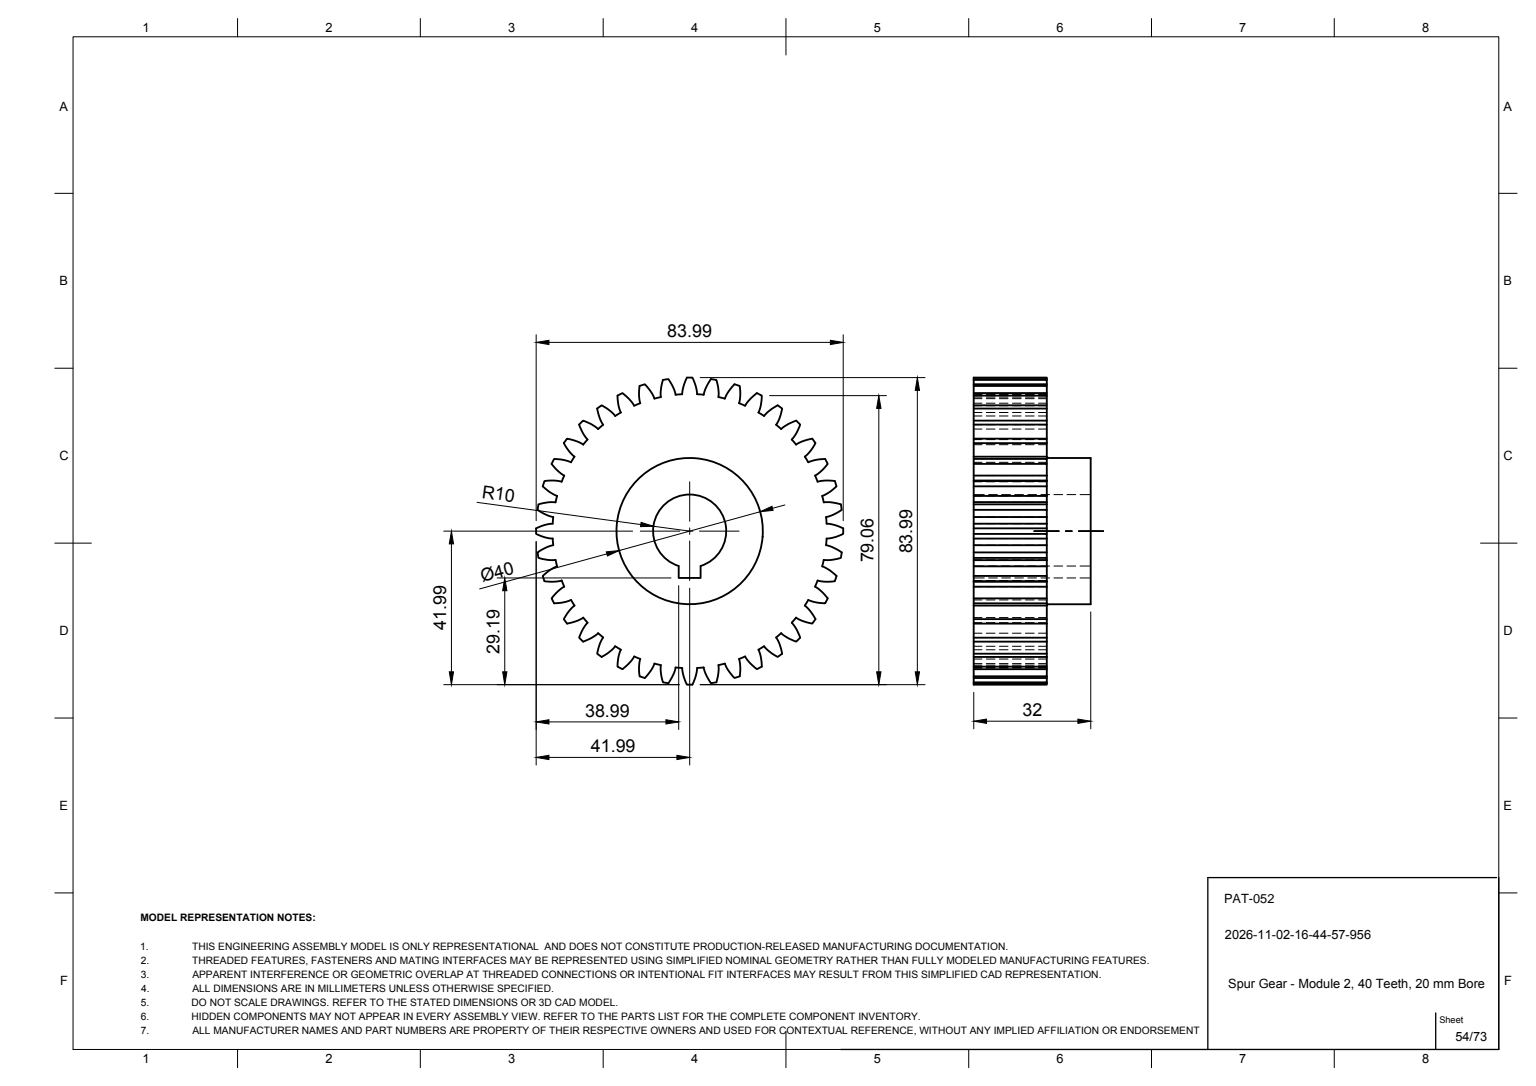
ISO-10303-21;
HEADER;
/* Generated by software containing ST-Developer
 * from STEP Tools, Inc. (www.steptools.com) 
 */

FILE_DESCRIPTION(
/* description */ ('Hand-crank gear train demonstrator'),
/* implementation_level */ '2;1');

FILE_NAME(
/* name */ 'Spur Gear - Module 2, 40 Teeth, 20 mm Bore.step',
/* time_stamp */ '2026-10-28T03:22:13-07:00',
/* author */ (''),
/* organization */ (''),
/* preprocessor_version */ 'ST-DEVELOPER v20.2',
/* originating_system */ 'Autodesk Translation Framework v15.17.0.0',
/* authorisation */ '');

FILE_SCHEMA (('AUTOMOTIVE_DESIGN { 1 0 10303 214 3 1 1 }'));
ENDSEC;

DATA;
#10=MECHANICAL_DESIGN_GEOMETRIC_PRESENTATION_REPRESENTATION('',(#1263),#62758);
#51=(
BOUNDED_SURFACE()
B_SPLINE_SURFACE(5,1,((#44627,#44628),(#44629,#44630),(#44631,#44632),(#44633,
#44634),(#44635,#44636),(#44637,#44638),(#44639,#44640),(#44641,#44642),
(#44643,#44644),(#44645,#44646),(#44647,#44648),(#44649,#44650),(#44651,
#44652),(#44653,#44654),(#44655,#44656),(#44657,#44658),(#44659,#44660),
(#44661,#44662),(#44663,#44664),(#44665,#44666),(#44667,#44668),(#44669,
#44670),(#44671,#44672),(#44673,#44674),(#44675,#44676),(#44677,#44678),
(#44679,#44680),(#44681,#44682),(#44683,#44684),(#44685,#44686),(#44687,
#44688),(#44689,#44690),(#44691,#44692),(#44693,#44694),(#44695,#44696),
(#44697,#44698),(#44699,#44700),(#44701,#44702),(#44703,#44704),(#44705,
#44706),(#44707,#44708),(#44709,#44710),(#44711,#44712),(#44713,#44714),
(#44715,#44716),(#44717,#44718),(#44719,#44720),(#44721,#44722),(#44723,
#44724),(#44725,#44726),(#44727,#44728),(#44729,#44730),(#44731,#44732),
(#44733,#44734),(#44735,#44736),(#44737,#44738),(#44739,#44740),(#44741,
#44742),(#44743,#44744),(#44745,#44746),(#44747,#44748),(#44749,#44750),
(#44751,#44752),(#44753,#44754),(#44755,#44756),(#44757,#44758),(#44759,
#44760),(#44761,#44762),(#44763,#44764),(#44765,#44766)),.UNSPECIFIED.,
 .F.,.F.,.F.)
B_SPLINE_SURFACE_WITH_KNOTS((6,1,1,1,1,1,1,1,1,1,1,1,1,1,1,1,1,1,1,1,1,
1,1,1,1,1,1,1,1,1,1,1,1,1,1,1,1,1,1,1,1,1,1,1,1,1,1,1,1,1,1,1,1,1,1,1,1,
1,1,1,1,1,1,1,1,6),(2,2),(-1.,-0.984615384615383,-0.969230769230768,-0.953846153846152,
-0.938461538461537,-0.923076923076922,-0.907692307692306,-0.892307692307691,
-0.876923076923076,-0.86153846153846,-0.846153846153845,-0.83076923076923,
-0.815384615384614,-0.799999999999999,-0.784615384615384,-0.769230769230768,
-0.753846153846153,-0.738461538461538,-0.723076923076922,-0.707692307692307,
-0.692307692307692,-0.676923076923076,-0.661538461538461,-0.646153846153846,
-0.63076923076923,-0.615384615384615,-0.6,-0.584615384615384,-0.569230769230769,
-0.553846153846154,-0.538461538461538,-0.523076923076923,-0.507692307692308,
-0.492307692307692,-0.476923076923077,-0.461538461538462,-0.446153846153846,
-0.430769230769231,-0.415384615384615,-0.4,-0.384615384615385,-0.369230769230769,
-0.353846153846154,-0.338461538461538,-0.323076923076923,-0.307692307692308,
-0.292307692307692,-0.276923076923077,-0.261538461538462,-0.246153846153846,
-0.230769230769231,-0.215384615384615,-0.2,-0.184615384615385,-0.169230769230769,
-0.153846153846154,-0.138461538461538,-0.123076923076923,-0.107692307692308,
-0.0923076923076923,-0.0769230769230769,-0.0615384615384615,-0.0461538461538462,
-0.0307692307692308,-0.0153846153846154,0.),(-1.,1.),.UNSPECIFIED.)
GEOMETRIC_REPRESENTATION_ITEM()
RATIONAL_B_SPLINE_SURFACE(((1.,1.),(1.,1.),(1.,1.),(1.,1.),(1.,1.),(1.,
1.),(1.,1.),(1.,1.),(1.,1.),(1.,1.),(1.,1.),(1.,1.),(1.,1.),(1.,1.),(1.,
1.),(1.,1.),(1.,1.),(1.,1.),(1.,1.),(1.,1.),(1.,1.),(1.,1.),(1.,1.),(1.,
1.),(1.,1.),(1.,1.),(1.,1.),(1.,1.),(1.,1.),(1.,1.),(1.,1.),(1.,1.),(1.,
1.),(1.,1.),(1.,1.),(1.,1.),(1.,1.),(1.,1.),(1.,1.),(1.,1.),(1.,1.),(1.,
1.),(1.,1.),(1.,1.),(1.,1.),(1.,1.),(1.,1.),(1.,1.),(1.,1.),(1.,1.),(1.,
1.),(1.,1.),(1.,1.),(1.,1.),(1.,1.),(1.,1.),(1.,1.),(1.,1.),(1.,1.),(1.,
1.),(1.,1.),(1.,1.),(1.,1.),(1.,1.),(1.,1.),(1.,1.),(1.,1.),(1.,1.),(1.,
1.),(1.,1.)))
REPRESENTATION_ITEM('')
SURFACE()
);
#52=(
BOUNDED_SURFACE()
B_SPLINE_SURFACE(5,1,((#44846,#44847),(#44848,#44849),(#44850,#44851),(#44852,
#44853),(#44854,#44855),(#44856,#44857),(#44858,#44859),(#44860,#44861),
(#44862,#44863),(#44864,#44865),(#44866,#44867),(#44868,#44869),(#44870,
#44871),(#44872,#44873),(#44874,#44875),(#44876,#44877),(#44878,#44879),
(#44880,#44881),(#44882,#44883),(#44884,#44885),(#44886,#44887),(#44888,
#44889),(#44890,#44891),(#44892,#44893),(#44894,#44895),(#44896,#44897),
(#44898,#44899),(#44900,#44901),(#44902,#44903),(#44904,#44905),(#44906,
#44907),(#44908,#44909),(#44910,#44911),(#44912,#44913),(#44914,#44915),
(#44916,#44917),(#44918,#44919),(#44920,#44921),(#44922,#44923),(#44924,
#44925),(#44926,#44927),(#44928,#44929),(#44930,#44931),(#44932,#44933),
(#44934,#44935),(#44936,#44937),(#44938,#44939),(#44940,#44941),(#44942,
#44943),(#44944,#44945),(#44946,#44947),(#44948,#44949),(#44950,#44951),
(#44952,#44953),(#44954,#44955),(#44956,#44957),(#44958,#44959),(#44960,
#44961),(#44962,#44963),(#44964,#44965),(#44966,#44967),(#44968,#44969),
(#44970,#44971),(#44972,#44973),(#44974,#44975),(#44976,#44977),(#44978,
#44979),(#44980,#44981),(#44982,#44983),(#44984,#44985)),.UNSPECIFIED.,
 .F.,.F.,.F.)
B_SPLINE_SURFACE_WITH_KNOTS((6,1,1,1,1,1,1,1,1,1,1,1,1,1,1,1,1,1,1,1,1,
1,1,1,1,1,1,1,1,1,1,1,1,1,1,1,1,1,1,1,1,1,1,1,1,1,1,1,1,1,1,1,1,1,1,1,1,
1,1,1,1,1,1,1,1,6),(2,2),(-1.,-0.984615384615383,-0.969230769230768,-0.953846153846152,
-0.938461538461537,-0.923076923076922,-0.907692307692306,-0.892307692307691,
-0.876923076923076,-0.86153846153846,-0.846153846153845,-0.83076923076923,
-0.815384615384614,-0.799999999999999,-0.784615384615384,-0.769230769230768,
-0.753846153846153,-0.738461538461538,-0.723076923076922,-0.707692307692307,
-0.692307692307692,-0.676923076923076,-0.661538461538461,-0.646153846153846,
-0.63076923076923,-0.615384615384615,-0.6,-0.584615384615384,-0.569230769230769,
-0.553846153846154,-0.538461538461538,-0.523076923076923,-0.507692307692308,
-0.492307692307692,-0.476923076923077,-0.461538461538462,-0.446153846153846,
-0.430769230769231,-0.415384615384615,-0.4,-0.384615384615385,-0.369230769230769,
-0.353846153846154,-0.338461538461538,-0.323076923076923,-0.307692307692308,
-0.292307692307692,-0.276923076923077,-0.261538461538462,-0.246153846153846,
-0.230769230769231,-0.215384615384615,-0.2,-0.184615384615385,-0.169230769230769,
-0.153846153846154,-0.138461538461538,-0.123076923076923,-0.107692307692308,
-0.0923076923076923,-0.0769230769230769,-0.0615384615384615,-0.0461538461538462,
-0.0307692307692308,-0.0153846153846154,0.),(-1.,1.),.UNSPECIFIED.)
GEOMETRIC_REPRESENTATION_ITEM()
RATIONAL_B_SPLINE_SURFACE(((1.,1.),(1.,1.),(1.,1.),(1.,1.),(1.,1.),(1.,
1.),(1.,1.),(1.,1.),(1.,1.),(1.,1.),(1.,1.),(1.,1.),(1.,1.),(1.,1.),(1.,
1.),(1.,1.),(1.,1.),(1.,1.),(1.,1.),(1.,1.),(1.,1.),(1.,1.),(1.,1.),(1.,
1.),(1.,1.),(1.,1.),(1.,1.),(1.,1.),(1.,1.),(1.,1.),(1.,1.),(1.,1.),(1.,
1.),(1.,1.),(1.,1.),(1.,1.),(1.,1.),(1.,1.),(1.,1.),(1.,1.),(1.,1.),(1.,
1.),(1.,1.),(1.,1.),(1.,1.),(1.,1.),(1.,1.),(1.,1.),(1.,1.),(1.,1.),(1.,
1.),(1.,1.),(1.,1.),(1.,1.),(1.,1.),(1.,1.),(1.,1.),(1.,1.),(1.,1.),(1.,
1.),(1.,1.),(1.,1.),(1.,1.),(1.,1.),(1.,1.),(1.,1.),(1.,1.),(1.,1.),(1.,
1.),(1.,1.)))
REPRESENTATION_ITEM('')
SURFACE()
);
#53=(
BOUNDED_SURFACE()
B_SPLINE_SURFACE(5,1,((#45076,#45077),(#45078,#45079),(#45080,#45081),(#45082,
#45083),(#45084,#45085),(#45086,#45087),(#45088,#45089),(#45090,#45091),
(#45092,#45093),(#45094,#45095),(#45096,#45097),(#45098,#45099),(#45100,
#45101),(#45102,#45103),(#45104,#45105),(#45106,#45107),(#45108,#45109),
(#45110,#45111),(#45112,#45113),(#45114,#45115),(#45116,#45117),(#45118,
#45119),(#45120,#45121),(#45122,#45123),(#45124,#45125),(#45126,#45127),
(#45128,#45129),(#45130,#45131),(#45132,#45133),(#45134,#45135),(#45136,
#45137),(#45138,#45139),(#45140,#45141),(#45142,#45143),(#45144,#45145),
(#45146,#45147),(#45148,#45149),(#45150,#45151),(#45152,#45153),(#45154,
#45155),(#45156,#45157),(#45158,#45159),(#45160,#45161),(#45162,#45163),
(#45164,#45165),(#45166,#45167),(#45168,#45169),(#45170,#45171),(#45172,
#45173),(#45174,#45175),(#45176,#45177),(#45178,#45179),(#45180,#45181),
(#45182,#45183),(#45184,#45185),(#45186,#45187),(#45188,#45189),(#45190,
#45191),(#45192,#45193),(#45194,#45195),(#45196,#45197),(#45198,#45199),
(#45200,#45201),(#45202,#45203),(#45204,#45205),(#45206,#45207),(#45208,
#45209),(#45210,#45211),(#45212,#45213),(#45214,#45215)),.UNSPECIFIED.,
 .F.,.F.,.F.)
B_SPLINE_SURFACE_WITH_KNOTS((6,1,1,1,1,1,1,1,1,1,1,1,1,1,1,1,1,1,1,1,1,
1,1,1,1,1,1,1,1,1,1,1,1,1,1,1,1,1,1,1,1,1,1,1,1,1,1,1,1,1,1,1,1,1,1,1,1,
1,1,1,1,1,1,1,1,6),(2,2),(-1.,-0.984615384615383,-0.969230769230768,-0.953846153846152,
-0.938461538461537,-0.923076923076922,-0.907692307692306,-0.892307692307691,
-0.876923076923076,-0.86153846153846,-0.846153846153845,-0.83076923076923,
-0.815384615384614,-0.799999999999999,-0.784615384615384,-0.769230769230768,
-0.753846153846153,-0.738461538461538,-0.723076923076922,-0.707692307692307,
-0.692307692307692,-0.676923076923076,-0.661538461538461,-0.646153846153846,
-0.63076923076923,-0.615384615384615,-0.6,-0.584615384615384,-0.569230769230769,
-0.553846153846154,-0.538461538461538,-0.523076923076923,-0.507692307692308,
-0.492307692307692,-0.476923076923077,-0.461538461538462,-0.446153846153846,
-0.430769230769231,-0.415384615384615,-0.4,-0.384615384615385,-0.369230769230769,
-0.353846153846154,-0.338461538461538,-0.323076923076923,-0.307692307692308,
-0.292307692307692,-0.276923076923077,-0.261538461538462,-0.246153846153846,
-0.230769230769231,-0.215384615384615,-0.2,-0.184615384615385,-0.169230769230769,
-0.153846153846154,-0.138461538461538,-0.123076923076923,-0.107692307692308,
-0.0923076923076923,-0.0769230769230769,-0.0615384615384615,-0.0461538461538462,
-0.0307692307692308,-0.0153846153846154,0.),(-1.,1.),.UNSPECIFIED.)
GEOMETRIC_REPRESENTATION_ITEM()
RATIONAL_B_SPLINE_SURFACE(((1.,1.),(1.,1.),(1.,1.),(1.,1.),(1.,1.),(1.,
1.),(1.,1.),(1.,1.),(1.,1.),(1.,1.),(1.,1.),(1.,1.),(1.,1.),(1.,1.),(1.,
1.),(1.,1.),(1.,1.),(1.,1.),(1.,1.),(1.,1.),(1.,1.),(1.,1.),(1.,1.),(1.,
1.),(1.,1.),(1.,1.),(1.,1.),(1.,1.),(1.,1.),(1.,1.),(1.,1.),(1.,1.),(1.,
1.),(1.,1.),(1.,1.),(1.,1.),(1.,1.),(1.,1.),(1.,1.),(1.,1.),(1.,1.),(1.,
1.),(1.,1.),(1.,1.),(1.,1.),(1.,1.),(1.,1.),(1.,1.),(1.,1.),(1.,1.),(1.,
1.),(1.,1.),(1.,1.),(1.,1.),(1.,1.),(1.,1.),(1.,1.),(1.,1.),(1.,1.),(1.,
1.),(1.,1.),(1.,1.),(1.,1.),(1.,1.),(1.,1.),(1.,1.),(1.,1.),(1.,1.),(1.,
1.),(1.,1.)))
REPRESENTATION_ITEM('')
SURFACE()
);
#54=(
BOUNDED_SURFACE()
B_SPLINE_SURFACE(5,1,((#45288,#45289),(#45290,#45291),(#45292,#45293),(#45294,
#45295),(#45296,#45297),(#45298,#45299),(#45300,#45301),(#45302,#45303),
(#45304,#45305),(#45306,#45307),(#45308,#45309),(#45310,#45311),(#45312,
#45313),(#45314,#45315),(#45316,#45317),(#45318,#45319),(#45320,#45321),
(#45322,#45323),(#45324,#45325),(#45326,#45327),(#45328,#45329),(#45330,
#45331),(#45332,#45333),(#45334,#45335),(#45336,#45337),(#45338,#45339),
(#45340,#45341),(#45342,#45343),(#45344,#45345),(#45346,#45347),(#45348,
#45349),(#45350,#45351),(#45352,#45353),(#45354,#45355),(#45356,#45357),
(#45358,#45359),(#45360,#45361),(#45362,#45363),(#45364,#45365),(#45366,
#45367),(#45368,#45369),(#45370,#45371),(#45372,#45373),(#45374,#45375),
(#45376,#45377),(#45378,#45379),(#45380,#45381),(#45382,#45383),(#45384,
#45385),(#45386,#45387),(#45388,#45389),(#45390,#45391),(#45392,#45393),
(#45394,#45395),(#45396,#45397),(#45398,#45399),(#45400,#45401),(#45402,
#45403),(#45404,#45405),(#45406,#45407),(#45408,#45409),(#45410,#45411),
(#45412,#45413),(#45414,#45415),(#45416,#45417),(#45418,#45419),(#45420,
#45421),(#45422,#45423),(#45424,#45425),(#45426,#45427)),.UNSPECIFIED.,
 .F.,.F.,.F.)
B_SPLINE_SURFACE_WITH_KNOTS((6,1,1,1,1,1,1,1,1,1,1,1,1,1,1,1,1,1,1,1,1,
1,1,1,1,1,1,1,1,1,1,1,1,1,1,1,1,1,1,1,1,1,1,1,1,1,1,1,1,1,1,1,1,1,1,1,1,
1,1,1,1,1,1,1,1,6),(2,2),(-1.,-0.984615384615383,-0.969230769230768,-0.953846153846152,
-0.938461538461537,-0.923076923076922,-0.907692307692306,-0.892307692307691,
-0.876923076923076,-0.86153846153846,-0.846153846153845,-0.83076923076923,
-0.815384615384614,-0.799999999999999,-0.784615384615384,-0.769230769230768,
-0.753846153846153,-0.738461538461538,-0.723076923076922,-0.707692307692307,
-0.692307692307692,-0.676923076923076,-0.661538461538461,-0.646153846153846,
-0.63076923076923,-0.615384615384615,-0.6,-0.584615384615384,-0.569230769230769,
-0.553846153846154,-0.538461538461538,-0.523076923076923,-0.507692307692308,
-0.492307692307692,-0.476923076923077,-0.461538461538462,-0.446153846153846,
-0.430769230769231,-0.415384615384615,-0.4,-0.384615384615385,-0.369230769230769,
-0.353846153846154,-0.338461538461538,-0.323076923076923,-0.307692307692308,
-0.292307692307692,-0.276923076923077,-0.261538461538462,-0.246153846153846,
-0.230769230769231,-0.215384615384615,-0.2,-0.184615384615385,-0.169230769230769,
-0.153846153846154,-0.138461538461538,-0.123076923076923,-0.107692307692308,
-0.0923076923076923,-0.0769230769230769,-0.0615384615384615,-0.0461538461538462,
-0.0307692307692308,-0.0153846153846154,0.),(-1.,1.),.UNSPECIFIED.)
GEOMETRIC_REPRESENTATION_ITEM()
RATIONAL_B_SPLINE_SURFACE(((1.,1.),(1.,1.),(1.,1.),(1.,1.),(1.,1.),(1.,
1.),(1.,1.),(1.,1.),(1.,1.),(1.,1.),(1.,1.),(1.,1.),(1.,1.),(1.,1.),(1.,
1.),(1.,1.),(1.,1.),(1.,1.),(1.,1.),(1.,1.),(1.,1.),(1.,1.),(1.,1.),(1.,
1.),(1.,1.),(1.,1.),(1.,1.),(1.,1.),(1.,1.),(1.,1.),(1.,1.),(1.,1.),(1.,
1.),(1.,1.),(1.,1.),(1.,1.),(1.,1.),(1.,1.),(1.,1.),(1.,1.),(1.,1.),(1.,
1.),(1.,1.),(1.,1.),(1.,1.),(1.,1.),(1.,1.),(1.,1.),(1.,1.),(1.,1.),(1.,
1.),(1.,1.),(1.,1.),(1.,1.),(1.,1.),(1.,1.),(1.,1.),(1.,1.),(1.,1.),(1.,
1.),(1.,1.),(1.,1.),(1.,1.),(1.,1.),(1.,1.),(1.,1.),(1.,1.),(1.,1.),(1.,
1.),(1.,1.)))
REPRESENTATION_ITEM('')
SURFACE()
);
#55=(
BOUNDED_SURFACE()
B_SPLINE_SURFACE(5,1,((#45518,#45519),(#45520,#45521),(#45522,#45523),(#45524,
#45525),(#45526,#45527),(#45528,#45529),(#45530,#45531),(#45532,#45533),
(#45534,#45535),(#45536,#45537),(#45538,#45539),(#45540,#45541),(#45542,
#45543),(#45544,#45545),(#45546,#45547),(#45548,#45549),(#45550,#45551),
(#45552,#45553),(#45554,#45555),(#45556,#45557),(#45558,#45559),(#45560,
#45561),(#45562,#45563),(#45564,#45565),(#45566,#45567),(#45568,#45569),
(#45570,#45571),(#45572,#45573),(#45574,#45575),(#45576,#45577),(#45578,
#45579),(#45580,#45581),(#45582,#45583),(#45584,#45585),(#45586,#45587),
(#45588,#45589),(#45590,#45591),(#45592,#45593),(#45594,#45595),(#45596,
#45597),(#45598,#45599),(#45600,#45601),(#45602,#45603),(#45604,#45605),
(#45606,#45607),(#45608,#45609),(#45610,#45611),(#45612,#45613),(#45614,
#45615),(#45616,#45617),(#45618,#45619),(#45620,#45621),(#45622,#45623),
(#45624,#45625),(#45626,#45627),(#45628,#45629),(#45630,#45631),(#45632,
#45633),(#45634,#45635),(#45636,#45637),(#45638,#45639),(#45640,#45641),
(#45642,#45643),(#45644,#45645),(#45646,#45647),(#45648,#45649),(#45650,
#45651),(#45652,#45653),(#45654,#45655),(#45656,#45657)),.UNSPECIFIED.,
 .F.,.F.,.F.)
B_SPLINE_SURFACE_WITH_KNOTS((6,1,1,1,1,1,1,1,1,1,1,1,1,1,1,1,1,1,1,1,1,
1,1,1,1,1,1,1,1,1,1,1,1,1,1,1,1,1,1,1,1,1,1,1,1,1,1,1,1,1,1,1,1,1,1,1,1,
1,1,1,1,1,1,1,1,6),(2,2),(-1.,-0.984615384615383,-0.969230769230768,-0.953846153846152,
-0.938461538461537,-0.923076923076922,-0.907692307692306,-0.892307692307691,
-0.876923076923076,-0.86153846153846,-0.846153846153845,-0.83076923076923,
-0.815384615384614,-0.799999999999999,-0.784615384615384,-0.769230769230768,
-0.753846153846153,-0.738461538461538,-0.723076923076922,-0.707692307692307,
-0.692307692307692,-0.676923076923076,-0.661538461538461,-0.646153846153846,
-0.63076923076923,-0.615384615384615,-0.6,-0.584615384615384,-0.569230769230769,
-0.553846153846154,-0.538461538461538,-0.523076923076923,-0.507692307692308,
-0.492307692307692,-0.476923076923077,-0.461538461538462,-0.446153846153846,
-0.430769230769231,-0.415384615384615,-0.4,-0.384615384615385,-0.369230769230769,
-0.353846153846154,-0.338461538461538,-0.323076923076923,-0.307692307692308,
-0.292307692307692,-0.276923076923077,-0.261538461538462,-0.246153846153846,
-0.230769230769231,-0.215384615384615,-0.2,-0.184615384615385,-0.169230769230769,
-0.153846153846154,-0.138461538461538,-0.123076923076923,-0.107692307692308,
-0.0923076923076923,-0.0769230769230769,-0.0615384615384615,-0.0461538461538462,
-0.0307692307692308,-0.0153846153846154,0.),(-1.,1.),.UNSPECIFIED.)
GEOMETRIC_REPRESENTATION_ITEM()
RATIONAL_B_SPLINE_SURFACE(((1.,1.),(1.,1.),(1.,1.),(1.,1.),(1.,1.),(1.,
1.),(1.,1.),(1.,1.),(1.,1.),(1.,1.),(1.,1.),(1.,1.),(1.,1.),(1.,1.),(1.,
1.),(1.,1.),(1.,1.),(1.,1.),(1.,1.),(1.,1.),(1.,1.),(1.,1.),(1.,1.),(1.,
1.),(1.,1.),(1.,1.),(1.,1.),(1.,1.),(1.,1.),(1.,1.),(1.,1.),(1.,1.),(1.,
1.),(1.,1.),(1.,1.),(1.,1.),(1.,1.),(1.,1.),(1.,1.),(1.,1.),(1.,1.),(1.,
1.),(1.,1.),(1.,1.),(1.,1.),(1.,1.),(1.,1.),(1.,1.),(1.,1.),(1.,1.),(1.,
1.),(1.,1.),(1.,1.),(1.,1.),(1.,1.),(1.,1.),(1.,1.),(1.,1.),(1.,1.),(1.,
1.),(1.,1.),(1.,1.),(1.,1.),(1.,1.),(1.,1.),(1.,1.),(1.,1.),(1.,1.),(1.,
1.),(1.,1.)))
REPRESENTATION_ITEM('')
SURFACE()
);
#56=(
BOUNDED_SURFACE()
B_SPLINE_SURFACE(5,1,((#45730,#45731),(#45732,#45733),(#45734,#45735),(#45736,
#45737),(#45738,#45739),(#45740,#45741),(#45742,#45743),(#45744,#45745),
(#45746,#45747),(#45748,#45749),(#45750,#45751),(#45752,#45753),(#45754,
#45755),(#45756,#45757),(#45758,#45759),(#45760,#45761),(#45762,#45763),
(#45764,#45765),(#45766,#45767),(#45768,#45769),(#45770,#45771),(#45772,
#45773),(#45774,#45775),(#45776,#45777),(#45778,#45779),(#45780,#45781),
(#45782,#45783),(#45784,#45785),(#45786,#45787),(#45788,#45789),(#45790,
#45791),(#45792,#45793),(#45794,#45795),(#45796,#45797),(#45798,#45799),
(#45800,#45801),(#45802,#45803),(#45804,#45805),(#45806,#45807),(#45808,
#45809),(#45810,#45811),(#45812,#45813),(#45814,#45815),(#45816,#45817),
(#45818,#45819),(#45820,#45821),(#45822,#45823),(#45824,#45825),(#45826,
#45827),(#45828,#45829),(#45830,#45831),(#45832,#45833),(#45834,#45835),
(#45836,#45837),(#45838,#45839),(#45840,#45841),(#45842,#45843),(#45844,
#45845),(#45846,#45847),(#45848,#45849),(#45850,#45851),(#45852,#45853),
(#45854,#45855),(#45856,#45857),(#45858,#45859),(#45860,#45861),(#45862,
#45863),(#45864,#45865),(#45866,#45867),(#45868,#45869)),.UNSPECIFIED.,
 .F.,.F.,.F.)
B_SPLINE_SURFACE_WITH_KNOTS((6,1,1,1,1,1,1,1,1,1,1,1,1,1,1,1,1,1,1,1,1,
1,1,1,1,1,1,1,1,1,1,1,1,1,1,1,1,1,1,1,1,1,1,1,1,1,1,1,1,1,1,1,1,1,1,1,1,
1,1,1,1,1,1,1,1,6),(2,2),(-1.,-0.984615384615383,-0.969230769230768,-0.953846153846152,
-0.938461538461537,-0.923076923076922,-0.907692307692306,-0.892307692307691,
-0.876923076923076,-0.86153846153846,-0.846153846153845,-0.83076923076923,
-0.815384615384614,-0.799999999999999,-0.784615384615384,-0.769230769230768,
-0.753846153846153,-0.738461538461538,-0.723076923076922,-0.707692307692307,
-0.692307692307692,-0.676923076923076,-0.661538461538461,-0.646153846153846,
-0.63076923076923,-0.615384615384615,-0.6,-0.584615384615384,-0.569230769230769,
-0.553846153846154,-0.538461538461538,-0.523076923076923,-0.507692307692308,
-0.492307692307692,-0.476923076923077,-0.461538461538462,-0.446153846153846,
-0.430769230769231,-0.415384615384615,-0.4,-0.384615384615385,-0.369230769230769,
-0.353846153846154,-0.338461538461538,-0.323076923076923,-0.307692307692308,
-0.292307692307692,-0.276923076923077,-0.261538461538462,-0.246153846153846,
-0.230769230769231,-0.215384615384615,-0.2,-0.184615384615385,-0.169230769230769,
-0.153846153846154,-0.138461538461538,-0.123076923076923,-0.107692307692308,
-0.0923076923076923,-0.0769230769230769,-0.0615384615384615,-0.0461538461538462,
-0.0307692307692308,-0.0153846153846154,0.),(-1.,1.),.UNSPECIFIED.)
GEOMETRIC_REPRESENTATION_ITEM()
RATIONAL_B_SPLINE_SURFACE(((1.,1.),(1.,1.),(1.,1.),(1.,1.),(1.,1.),(1.,
1.),(1.,1.),(1.,1.),(1.,1.),(1.,1.),(1.,1.),(1.,1.),(1.,1.),(1.,1.),(1.,
1.),(1.,1.),(1.,1.),(1.,1.),(1.,1.),(1.,1.),(1.,1.),(1.,1.),(1.,1.),(1.,
1.),(1.,1.),(1.,1.),(1.,1.),(1.,1.),(1.,1.),(1.,1.),(1.,1.),(1.,1.),(1.,
1.),(1.,1.),(1.,1.),(1.,1.),(1.,1.),(1.,1.),(1.,1.),(1.,1.),(1.,1.),(1.,
1.),(1.,1.),(1.,1.),(1.,1.),(1.,1.),(1.,1.),(1.,1.),(1.,1.),(1.,1.),(1.,
1.),(1.,1.),(1.,1.),(1.,1.),(1.,1.),(1.,1.),(1.,1.),(1.,1.),(1.,1.),(1.,
1.),(1.,1.),(1.,1.),(1.,1.),(1.,1.),(1.,1.),(1.,1.),(1.,1.),(1.,1.),(1.,
1.),(1.,1.)))
REPRESENTATION_ITEM('')
SURFACE()
);
#57=(
BOUNDED_SURFACE()
B_SPLINE_SURFACE(5,1,((#45960,#45961),(#45962,#45963),(#45964,#45965),(#45966,
#45967),(#45968,#45969),(#45970,#45971),(#45972,#45973),(#45974,#45975),
(#45976,#45977),(#45978,#45979),(#45980,#45981),(#45982,#45983),(#45984,
#45985),(#45986,#45987),(#45988,#45989),(#45990,#45991),(#45992,#45993),
(#45994,#45995),(#45996,#45997),(#45998,#45999),(#46000,#46001),(#46002,
#46003),(#46004,#46005),(#46006,#46007),(#46008,#46009),(#46010,#46011),
(#46012,#46013),(#46014,#46015),(#46016,#46017),(#46018,#46019),(#46020,
#46021),(#46022,#46023),(#46024,#46025),(#46026,#46027),(#46028,#46029),
(#46030,#46031),(#46032,#46033),(#46034,#46035),(#46036,#46037),(#46038,
#46039),(#46040,#46041),(#46042,#46043),(#46044,#46045),(#46046,#46047),
(#46048,#46049),(#46050,#46051),(#46052,#46053),(#46054,#46055),(#46056,
#46057),(#46058,#46059),(#46060,#46061),(#46062,#46063),(#46064,#46065),
(#46066,#46067),(#46068,#46069),(#46070,#46071),(#46072,#46073),(#46074,
#46075),(#46076,#46077),(#46078,#46079),(#46080,#46081),(#46082,#46083),
(#46084,#46085),(#46086,#46087),(#46088,#46089),(#46090,#46091),(#46092,
#46093),(#46094,#46095),(#46096,#46097),(#46098,#46099)),.UNSPECIFIED.,
 .F.,.F.,.F.)
B_SPLINE_SURFACE_WITH_KNOTS((6,1,1,1,1,1,1,1,1,1,1,1,1,1,1,1,1,1,1,1,1,
1,1,1,1,1,1,1,1,1,1,1,1,1,1,1,1,1,1,1,1,1,1,1,1,1,1,1,1,1,1,1,1,1,1,1,1,
1,1,1,1,1,1,1,1,6),(2,2),(-1.,-0.984615384615383,-0.969230769230768,-0.953846153846152,
-0.938461538461537,-0.923076923076922,-0.907692307692306,-0.892307692307691,
-0.876923076923076,-0.86153846153846,-0.846153846153845,-0.83076923076923,
-0.815384615384614,-0.799999999999999,-0.784615384615384,-0.769230769230768,
-0.753846153846153,-0.738461538461538,-0.723076923076922,-0.707692307692307,
-0.692307692307692,-0.676923076923076,-0.661538461538461,-0.646153846153846,
-0.63076923076923,-0.615384615384615,-0.6,-0.584615384615384,-0.569230769230769,
-0.553846153846154,-0.538461538461538,-0.523076923076923,-0.507692307692308,
-0.492307692307692,-0.476923076923077,-0.461538461538462,-0.446153846153846,
-0.430769230769231,-0.415384615384615,-0.4,-0.384615384615385,-0.369230769230769,
-0.353846153846154,-0.338461538461538,-0.323076923076923,-0.307692307692308,
-0.292307692307692,-0.276923076923077,-0.261538461538462,-0.246153846153846,
-0.230769230769231,-0.215384615384615,-0.2,-0.184615384615385,-0.169230769230769,
-0.153846153846154,-0.138461538461538,-0.123076923076923,-0.107692307692308,
-0.0923076923076923,-0.0769230769230769,-0.0615384615384615,-0.0461538461538462,
-0.0307692307692308,-0.0153846153846154,0.),(-1.,1.),.UNSPECIFIED.)
GEOMETRIC_REPRESENTATION_ITEM()
RATIONAL_B_SPLINE_SURFACE(((1.,1.),(1.,1.),(1.,1.),(1.,1.),(1.,1.),(1.,
1.),(1.,1.),(1.,1.),(1.,1.),(1.,1.),(1.,1.),(1.,1.),(1.,1.),(1.,1.),(1.,
1.),(1.,1.),(1.,1.),(1.,1.),(1.,1.),(1.,1.),(1.,1.),(1.,1.),(1.,1.),(1.,
1.),(1.,1.),(1.,1.),(1.,1.),(1.,1.),(1.,1.),(1.,1.),(1.,1.),(1.,1.),(1.,
1.),(1.,1.),(1.,1.),(1.,1.),(1.,1.),(1.,1.),(1.,1.),(1.,1.),(1.,1.),(1.,
1.),(1.,1.),(1.,1.),(1.,1.),(1.,1.),(1.,1.),(1.,1.),(1.,1.),(1.,1.),(1.,
1.),(1.,1.),(1.,1.),(1.,1.),(1.,1.),(1.,1.),(1.,1.),(1.,1.),(1.,1.),(1.,
1.),(1.,1.),(1.,1.),(1.,1.),(1.,1.),(1.,1.),(1.,1.),(1.,1.),(1.,1.),(1.,
1.),(1.,1.)))
REPRESENTATION_ITEM('')
SURFACE()
);
#58=(
BOUNDED_SURFACE()
B_SPLINE_SURFACE(5,1,((#46172,#46173),(#46174,#46175),(#46176,#46177),(#46178,
#46179),(#46180,#46181),(#46182,#46183),(#46184,#46185),(#46186,#46187),
(#46188,#46189),(#46190,#46191),(#46192,#46193),(#46194,#46195),(#46196,
#46197),(#46198,#46199),(#46200,#46201),(#46202,#46203),(#46204,#46205),
(#46206,#46207),(#46208,#46209),(#46210,#46211),(#46212,#46213),(#46214,
#46215),(#46216,#46217),(#46218,#46219),(#46220,#46221),(#46222,#46223),
(#46224,#46225),(#46226,#46227),(#46228,#46229),(#46230,#46231),(#46232,
#46233),(#46234,#46235),(#46236,#46237),(#46238,#46239),(#46240,#46241),
(#46242,#46243),(#46244,#46245),(#46246,#46247),(#46248,#46249),(#46250,
#46251),(#46252,#46253),(#46254,#46255),(#46256,#46257),(#46258,#46259),
(#46260,#46261),(#46262,#46263),(#46264,#46265),(#46266,#46267),(#46268,
#46269),(#46270,#46271),(#46272,#46273),(#46274,#46275),(#46276,#46277),
(#46278,#46279),(#46280,#46281),(#46282,#46283),(#46284,#46285),(#46286,
#46287),(#46288,#46289),(#46290,#46291),(#46292,#46293),(#46294,#46295),
(#46296,#46297),(#46298,#46299),(#46300,#46301),(#46302,#46303),(#46304,
#46305),(#46306,#46307),(#46308,#46309),(#46310,#46311)),.UNSPECIFIED.,
 .F.,.F.,.F.)
B_SPLINE_SURFACE_WITH_KNOTS((6,1,1,1,1,1,1,1,1,1,1,1,1,1,1,1,1,1,1,1,1,
1,1,1,1,1,1,1,1,1,1,1,1,1,1,1,1,1,1,1,1,1,1,1,1,1,1,1,1,1,1,1,1,1,1,1,1,
1,1,1,1,1,1,1,1,6),(2,2),(-1.,-0.984615384615383,-0.969230769230768,-0.953846153846152,
-0.938461538461537,-0.923076923076922,-0.907692307692306,-0.892307692307691,
-0.876923076923076,-0.86153846153846,-0.846153846153845,-0.83076923076923,
-0.815384615384614,-0.799999999999999,-0.784615384615384,-0.769230769230768,
-0.753846153846153,-0.738461538461538,-0.723076923076922,-0.707692307692307,
-0.692307692307692,-0.676923076923076,-0.661538461538461,-0.646153846153846,
-0.63076923076923,-0.615384615384615,-0.6,-0.584615384615384,-0.569230769230769,
-0.553846153846154,-0.538461538461538,-0.523076923076923,-0.507692307692308,
-0.492307692307692,-0.476923076923077,-0.461538461538462,-0.446153846153846,
-0.430769230769231,-0.415384615384615,-0.4,-0.384615384615385,-0.369230769230769,
-0.353846153846154,-0.338461538461538,-0.323076923076923,-0.307692307692308,
-0.292307692307692,-0.276923076923077,-0.261538461538462,-0.246153846153846,
-0.230769230769231,-0.215384615384615,-0.2,-0.184615384615385,-0.169230769230769,
-0.153846153846154,-0.138461538461538,-0.123076923076923,-0.107692307692308,
-0.0923076923076923,-0.0769230769230769,-0.0615384615384615,-0.0461538461538462,
-0.0307692307692308,-0.0153846153846154,0.),(-1.,1.),.UNSPECIFIED.)
GEOMETRIC_REPRESENTATION_ITEM()
RATIONAL_B_SPLINE_SURFACE(((1.,1.),(1.,1.),(1.,1.),(1.,1.),(1.,1.),(1.,
1.),(1.,1.),(1.,1.),(1.,1.),(1.,1.),(1.,1.),(1.,1.),(1.,1.),(1.,1.),(1.,
1.),(1.,1.),(1.,1.),(1.,1.),(1.,1.),(1.,1.),(1.,1.),(1.,1.),(1.,1.),(1.,
1.),(1.,1.),(1.,1.),(1.,1.),(1.,1.),(1.,1.),(1.,1.),(1.,1.),(1.,1.),(1.,
1.),(1.,1.),(1.,1.),(1.,1.),(1.,1.),(1.,1.),(1.,1.),(1.,1.),(1.,1.),(1.,
1.),(1.,1.),(1.,1.),(1.,1.),(1.,1.),(1.,1.),(1.,1.),(1.,1.),(1.,1.),(1.,
1.),(1.,1.),(1.,1.),(1.,1.),(1.,1.),(1.,1.),(1.,1.),(1.,1.),(1.,1.),(1.,
1.),(1.,1.),(1.,1.),(1.,1.),(1.,1.),(1.,1.),(1.,1.),(1.,1.),(1.,1.),(1.,
1.),(1.,1.)))
REPRESENTATION_ITEM('')
SURFACE()
);
#59=(
BOUNDED_SURFACE()
B_SPLINE_SURFACE(5,1,((#46402,#46403),(#46404,#46405),(#46406,#46407),(#46408,
#46409),(#46410,#46411),(#46412,#46413),(#46414,#46415),(#46416,#46417),
(#46418,#46419),(#46420,#46421),(#46422,#46423),(#46424,#46425),(#46426,
#46427),(#46428,#46429),(#46430,#46431),(#46432,#46433),(#46434,#46435),
(#46436,#46437),(#46438,#46439),(#46440,#46441),(#46442,#46443),(#46444,
#46445),(#46446,#46447),(#46448,#46449),(#46450,#46451),(#46452,#46453),
(#46454,#46455),(#46456,#46457),(#46458,#46459),(#46460,#46461),(#46462,
#46463),(#46464,#46465),(#46466,#46467),(#46468,#46469),(#46470,#46471),
(#46472,#46473),(#46474,#46475),(#46476,#46477),(#46478,#46479),(#46480,
#46481),(#46482,#46483),(#46484,#46485),(#46486,#46487),(#46488,#46489),
(#46490,#46491),(#46492,#46493),(#46494,#46495),(#46496,#46497),(#46498,
#46499),(#46500,#46501),(#46502,#46503),(#46504,#46505),(#46506,#46507),
(#46508,#46509),(#46510,#46511),(#46512,#46513),(#46514,#46515),(#46516,
#46517),(#46518,#46519),(#46520,#46521),(#46522,#46523),(#46524,#46525),
(#46526,#46527),(#46528,#46529),(#46530,#46531),(#46532,#46533),(#46534,
#46535),(#46536,#46537),(#46538,#46539),(#46540,#46541)),.UNSPECIFIED.,
 .F.,.F.,.F.)
B_SPLINE_SURFACE_WITH_KNOTS((6,1,1,1,1,1,1,1,1,1,1,1,1,1,1,1,1,1,1,1,1,
1,1,1,1,1,1,1,1,1,1,1,1,1,1,1,1,1,1,1,1,1,1,1,1,1,1,1,1,1,1,1,1,1,1,1,1,
1,1,1,1,1,1,1,1,6),(2,2),(-1.,-0.984615384615383,-0.969230769230768,-0.953846153846152,
-0.938461538461537,-0.923076923076922,-0.907692307692306,-0.892307692307691,
-0.876923076923076,-0.86153846153846,-0.846153846153845,-0.83076923076923,
-0.815384615384614,-0.799999999999999,-0.784615384615384,-0.769230769230768,
-0.753846153846153,-0.738461538461538,-0.723076923076922,-0.707692307692307,
-0.692307692307692,-0.676923076923076,-0.661538461538461,-0.646153846153846,
-0.63076923076923,-0.615384615384615,-0.6,-0.584615384615384,-0.569230769230769,
-0.553846153846154,-0.538461538461538,-0.523076923076923,-0.507692307692308,
-0.492307692307692,-0.476923076923077,-0.461538461538462,-0.446153846153846,
-0.430769230769231,-0.415384615384615,-0.4,-0.384615384615385,-0.369230769230769,
-0.353846153846154,-0.338461538461538,-0.323076923076923,-0.307692307692308,
-0.292307692307692,-0.276923076923077,-0.261538461538462,-0.246153846153846,
-0.230769230769231,-0.215384615384615,-0.2,-0.184615384615385,-0.169230769230769,
-0.153846153846154,-0.138461538461538,-0.123076923076923,-0.107692307692308,
-0.0923076923076923,-0.0769230769230769,-0.0615384615384615,-0.0461538461538462,
-0.0307692307692308,-0.0153846153846154,0.),(-1.,1.),.UNSPECIFIED.)
GEOMETRIC_REPRESENTATION_ITEM()
RATIONAL_B_SPLINE_SURFACE(((1.,1.),(1.,1.),(1.,1.),(1.,1.),(1.,1.),(1.,
1.),(1.,1.),(1.,1.),(1.,1.),(1.,1.),(1.,1.),(1.,1.),(1.,1.),(1.,1.),(1.,
1.),(1.,1.),(1.,1.),(1.,1.),(1.,1.),(1.,1.),(1.,1.),(1.,1.),(1.,1.),(1.,
1.),(1.,1.),(1.,1.),(1.,1.),(1.,1.),(1.,1.),(1.,1.),(1.,1.),(1.,1.),(1.,
1.),(1.,1.),(1.,1.),(1.,1.),(1.,1.),(1.,1.),(1.,1.),(1.,1.),(1.,1.),(1.,
1.),(1.,1.),(1.,1.),(1.,1.),(1.,1.),(1.,1.),(1.,1.),(1.,1.),(1.,1.),(1.,
1.),(1.,1.),(1.,1.),(1.,1.),(1.,1.),(1.,1.),(1.,1.),(1.,1.),(1.,1.),(1.,
1.),(1.,1.),(1.,1.),(1.,1.),(1.,1.),(1.,1.),(1.,1.),(1.,1.),(1.,1.),(1.,
1.),(1.,1.)))
REPRESENTATION_ITEM('')
SURFACE()
);
#60=(
BOUNDED_SURFACE()
B_SPLINE_SURFACE(5,1,((#46614,#46615),(#46616,#46617),(#46618,#46619),(#46620,
#46621),(#46622,#46623),(#46624,#46625),(#46626,#46627),(#46628,#46629),
(#46630,#46631),(#46632,#46633),(#46634,#46635),(#46636,#46637),(#46638,
#46639),(#46640,#46641),(#46642,#46643),(#46644,#46645),(#46646,#46647),
(#46648,#46649),(#46650,#46651),(#46652,#46653),(#46654,#46655),(#46656,
#46657),(#46658,#46659),(#46660,#46661),(#46662,#46663),(#46664,#46665),
(#46666,#46667),(#46668,#46669),(#46670,#46671),(#46672,#46673),(#46674,
#46675),(#46676,#46677),(#46678,#46679),(#46680,#46681),(#46682,#46683),
(#46684,#46685),(#46686,#46687),(#46688,#46689),(#46690,#46691),(#46692,
#46693),(#46694,#46695),(#46696,#46697),(#46698,#46699),(#46700,#46701),
(#46702,#46703),(#46704,#46705),(#46706,#46707),(#46708,#46709),(#46710,
#46711),(#46712,#46713),(#46714,#46715),(#46716,#46717),(#46718,#46719),
(#46720,#46721),(#46722,#46723),(#46724,#46725),(#46726,#46727),(#46728,
#46729),(#46730,#46731),(#46732,#46733),(#46734,#46735),(#46736,#46737),
(#46738,#46739),(#46740,#46741),(#46742,#46743),(#46744,#46745),(#46746,
#46747),(#46748,#46749),(#46750,#46751),(#46752,#46753)),.UNSPECIFIED.,
 .F.,.F.,.F.)
B_SPLINE_SURFACE_WITH_KNOTS((6,1,1,1,1,1,1,1,1,1,1,1,1,1,1,1,1,1,1,1,1,
1,1,1,1,1,1,1,1,1,1,1,1,1,1,1,1,1,1,1,1,1,1,1,1,1,1,1,1,1,1,1,1,1,1,1,1,
1,1,1,1,1,1,1,1,6),(2,2),(-1.,-0.984615384615383,-0.969230769230768,-0.953846153846152,
-0.938461538461537,-0.923076923076922,-0.907692307692306,-0.892307692307691,
-0.876923076923076,-0.86153846153846,-0.846153846153845,-0.83076923076923,
-0.815384615384614,-0.799999999999999,-0.784615384615384,-0.769230769230768,
-0.753846153846153,-0.738461538461538,-0.723076923076922,-0.707692307692307,
-0.692307692307692,-0.676923076923076,-0.661538461538461,-0.646153846153846,
-0.63076923076923,-0.615384615384615,-0.6,-0.584615384615384,-0.569230769230769,
-0.553846153846154,-0.538461538461538,-0.523076923076923,-0.507692307692308,
-0.492307692307692,-0.476923076923077,-0.461538461538462,-0.446153846153846,
-0.430769230769231,-0.415384615384615,-0.4,-0.384615384615385,-0.369230769230769,
-0.353846153846154,-0.338461538461538,-0.323076923076923,-0.307692307692308,
-0.292307692307692,-0.276923076923077,-0.261538461538462,-0.246153846153846,
-0.230769230769231,-0.215384615384615,-0.2,-0.184615384615385,-0.169230769230769,
-0.153846153846154,-0.138461538461538,-0.123076923076923,-0.107692307692308,
-0.0923076923076923,-0.0769230769230769,-0.0615384615384615,-0.0461538461538462,
-0.0307692307692308,-0.0153846153846154,0.),(-1.,1.),.UNSPECIFIED.)
GEOMETRIC_REPRESENTATION_ITEM()
RATIONAL_B_SPLINE_SURFACE(((1.,1.),(1.,1.),(1.,1.),(1.,1.),(1.,1.),(1.,
1.),(1.,1.),(1.,1.),(1.,1.),(1.,1.),(1.,1.),(1.,1.),(1.,1.),(1.,1.),(1.,
1.),(1.,1.),(1.,1.),(1.,1.),(1.,1.),(1.,1.),(1.,1.),(1.,1.),(1.,1.),(1.,
1.),(1.,1.),(1.,1.),(1.,1.),(1.,1.),(1.,1.),(1.,1.),(1.,1.),(1.,1.),(1.,
1.),(1.,1.),(1.,1.),(1.,1.),(1.,1.),(1.,1.),(1.,1.),(1.,1.),(1.,1.),(1.,
1.),(1.,1.),(1.,1.),(1.,1.),(1.,1.),(1.,1.),(1.,1.),(1.,1.),(1.,1.),(1.,
1.),(1.,1.),(1.,1.),(1.,1.),(1.,1.),(1.,1.),(1.,1.),(1.,1.),(1.,1.),(1.,
1.),(1.,1.),(1.,1.),(1.,1.),(1.,1.),(1.,1.),(1.,1.),(1.,1.),(1.,1.),(1.,
1.),(1.,1.)))
REPRESENTATION_ITEM('')
SURFACE()
);
#61=(
BOUNDED_SURFACE()
B_SPLINE_SURFACE(5,1,((#46844,#46845),(#46846,#46847),(#46848,#46849),(#46850,
#46851),(#46852,#46853),(#46854,#46855),(#46856,#46857),(#46858,#46859),
(#46860,#46861),(#46862,#46863),(#46864,#46865),(#46866,#46867),(#46868,
#46869),(#46870,#46871),(#46872,#46873),(#46874,#46875),(#46876,#46877),
(#46878,#46879),(#46880,#46881),(#46882,#46883),(#46884,#46885),(#46886,
#46887),(#46888,#46889),(#46890,#46891),(#46892,#46893),(#46894,#46895),
(#46896,#46897),(#46898,#46899),(#46900,#46901),(#46902,#46903),(#46904,
#46905),(#46906,#46907),(#46908,#46909),(#46910,#46911),(#46912,#46913),
(#46914,#46915),(#46916,#46917),(#46918,#46919),(#46920,#46921),(#46922,
#46923),(#46924,#46925),(#46926,#46927),(#46928,#46929),(#46930,#46931),
(#46932,#46933),(#46934,#46935),(#46936,#46937),(#46938,#46939),(#46940,
#46941),(#46942,#46943),(#46944,#46945),(#46946,#46947),(#46948,#46949),
(#46950,#46951),(#46952,#46953),(#46954,#46955),(#46956,#46957),(#46958,
#46959),(#46960,#46961),(#46962,#46963),(#46964,#46965),(#46966,#46967),
(#46968,#46969),(#46970,#46971),(#46972,#46973),(#46974,#46975),(#46976,
#46977),(#46978,#46979),(#46980,#46981),(#46982,#46983)),.UNSPECIFIED.,
 .F.,.F.,.F.)
B_SPLINE_SURFACE_WITH_KNOTS((6,1,1,1,1,1,1,1,1,1,1,1,1,1,1,1,1,1,1,1,1,
1,1,1,1,1,1,1,1,1,1,1,1,1,1,1,1,1,1,1,1,1,1,1,1,1,1,1,1,1,1,1,1,1,1,1,1,
1,1,1,1,1,1,1,1,6),(2,2),(-1.,-0.984615384615383,-0.969230769230768,-0.953846153846152,
-0.938461538461537,-0.923076923076922,-0.907692307692306,-0.892307692307691,
-0.876923076923076,-0.86153846153846,-0.846153846153845,-0.83076923076923,
-0.815384615384614,-0.799999999999999,-0.784615384615384,-0.769230769230768,
-0.753846153846153,-0.738461538461538,-0.723076923076922,-0.707692307692307,
-0.692307692307692,-0.676923076923076,-0.661538461538461,-0.646153846153846,
-0.63076923076923,-0.615384615384615,-0.6,-0.584615384615384,-0.569230769230769,
-0.553846153846154,-0.538461538461538,-0.523076923076923,-0.507692307692308,
-0.492307692307692,-0.476923076923077,-0.461538461538462,-0.446153846153846,
-0.430769230769231,-0.415384615384615,-0.4,-0.384615384615385,-0.369230769230769,
-0.353846153846154,-0.338461538461538,-0.323076923076923,-0.307692307692308,
-0.292307692307692,-0.276923076923077,-0.261538461538462,-0.246153846153846,
-0.230769230769231,-0.215384615384615,-0.2,-0.184615384615385,-0.169230769230769,
-0.153846153846154,-0.138461538461538,-0.123076923076923,-0.107692307692308,
-0.0923076923076923,-0.0769230769230769,-0.0615384615384615,-0.0461538461538462,
-0.0307692307692308,-0.0153846153846154,0.),(-1.,1.),.UNSPECIFIED.)
GEOMETRIC_REPRESENTATION_ITEM()
RATIONAL_B_SPLINE_SURFACE(((1.,1.),(1.,1.),(1.,1.),(1.,1.),(1.,1.),(1.,
1.),(1.,1.),(1.,1.),(1.,1.),(1.,1.),(1.,1.),(1.,1.),(1.,1.),(1.,1.),(1.,
1.),(1.,1.),(1.,1.),(1.,1.),(1.,1.),(1.,1.),(1.,1.),(1.,1.),(1.,1.),(1.,
1.),(1.,1.),(1.,1.),(1.,1.),(1.,1.),(1.,1.),(1.,1.),(1.,1.),(1.,1.),(1.,
1.),(1.,1.),(1.,1.),(1.,1.),(1.,1.),(1.,1.),(1.,1.),(1.,1.),(1.,1.),(1.,
1.),(1.,1.),(1.,1.),(1.,1.),(1.,1.),(1.,1.),(1.,1.),(1.,1.),(1.,1.),(1.,
1.),(1.,1.),(1.,1.),(1.,1.),(1.,1.),(1.,1.),(1.,1.),(1.,1.),(1.,1.),(1.,
1.),(1.,1.),(1.,1.),(1.,1.),(1.,1.),(1.,1.),(1.,1.),(1.,1.),(1.,1.),(1.,
1.),(1.,1.)))
REPRESENTATION_ITEM('')
SURFACE()
);
#62=(
BOUNDED_SURFACE()
B_SPLINE_SURFACE(5,1,((#47056,#47057),(#47058,#47059),(#47060,#47061),(#47062,
#47063),(#47064,#47065),(#47066,#47067),(#47068,#47069),(#47070,#47071),
(#47072,#47073),(#47074,#47075),(#47076,#47077),(#47078,#47079),(#47080,
#47081),(#47082,#47083),(#47084,#47085),(#47086,#47087),(#47088,#47089),
(#47090,#47091),(#47092,#47093),(#47094,#47095),(#47096,#47097),(#47098,
#47099),(#47100,#47101),(#47102,#47103),(#47104,#47105),(#47106,#47107),
(#47108,#47109),(#47110,#47111),(#47112,#47113),(#47114,#47115),(#47116,
#47117),(#47118,#47119),(#47120,#47121),(#47122,#47123),(#47124,#47125),
(#47126,#47127),(#47128,#47129),(#47130,#47131),(#47132,#47133),(#47134,
#47135),(#47136,#47137),(#47138,#47139),(#47140,#47141),(#47142,#47143),
(#47144,#47145),(#47146,#47147),(#47148,#47149),(#47150,#47151),(#47152,
#47153),(#47154,#47155),(#47156,#47157),(#47158,#47159),(#47160,#47161),
(#47162,#47163),(#47164,#47165),(#47166,#47167),(#47168,#47169),(#47170,
#47171),(#47172,#47173),(#47174,#47175),(#47176,#47177),(#47178,#47179),
(#47180,#47181),(#47182,#47183),(#47184,#47185),(#47186,#47187),(#47188,
#47189),(#47190,#47191),(#47192,#47193),(#47194,#47195)),.UNSPECIFIED.,
 .F.,.F.,.F.)
B_SPLINE_SURFACE_WITH_KNOTS((6,1,1,1,1,1,1,1,1,1,1,1,1,1,1,1,1,1,1,1,1,
1,1,1,1,1,1,1,1,1,1,1,1,1,1,1,1,1,1,1,1,1,1,1,1,1,1,1,1,1,1,1,1,1,1,1,1,
1,1,1,1,1,1,1,1,6),(2,2),(-1.,-0.984615384615383,-0.969230769230768,-0.953846153846152,
-0.938461538461537,-0.923076923076922,-0.907692307692306,-0.892307692307691,
-0.876923076923076,-0.86153846153846,-0.846153846153845,-0.83076923076923,
-0.815384615384614,-0.799999999999999,-0.784615384615384,-0.769230769230768,
-0.753846153846153,-0.738461538461538,-0.723076923076922,-0.707692307692307,
-0.692307692307692,-0.676923076923076,-0.661538461538461,-0.646153846153846,
-0.63076923076923,-0.615384615384615,-0.6,-0.584615384615384,-0.569230769230769,
-0.553846153846154,-0.538461538461538,-0.523076923076923,-0.507692307692308,
-0.492307692307692,-0.476923076923077,-0.461538461538462,-0.446153846153846,
-0.430769230769231,-0.415384615384615,-0.4,-0.384615384615385,-0.369230769230769,
-0.353846153846154,-0.338461538461538,-0.323076923076923,-0.307692307692308,
-0.292307692307692,-0.276923076923077,-0.261538461538462,-0.246153846153846,
-0.230769230769231,-0.215384615384615,-0.2,-0.184615384615385,-0.169230769230769,
-0.153846153846154,-0.138461538461538,-0.123076923076923,-0.107692307692308,
-0.0923076923076923,-0.0769230769230769,-0.0615384615384615,-0.0461538461538462,
-0.0307692307692308,-0.0153846153846154,0.),(-1.,1.),.UNSPECIFIED.)
GEOMETRIC_REPRESENTATION_ITEM()
RATIONAL_B_SPLINE_SURFACE(((1.,1.),(1.,1.),(1.,1.),(1.,1.),(1.,1.),(1.,
1.),(1.,1.),(1.,1.),(1.,1.),(1.,1.),(1.,1.),(1.,1.),(1.,1.),(1.,1.),(1.,
1.),(1.,1.),(1.,1.),(1.,1.),(1.,1.),(1.,1.),(1.,1.),(1.,1.),(1.,1.),(1.,
1.),(1.,1.),(1.,1.),(1.,1.),(1.,1.),(1.,1.),(1.,1.),(1.,1.),(1.,1.),(1.,
1.),(1.,1.),(1.,1.),(1.,1.),(1.,1.),(1.,1.),(1.,1.),(1.,1.),(1.,1.),(1.,
1.),(1.,1.),(1.,1.),(1.,1.),(1.,1.),(1.,1.),(1.,1.),(1.,1.),(1.,1.),(1.,
1.),(1.,1.),(1.,1.),(1.,1.),(1.,1.),(1.,1.),(1.,1.),(1.,1.),(1.,1.),(1.,
1.),(1.,1.),(1.,1.),(1.,1.),(1.,1.),(1.,1.),(1.,1.),(1.,1.),(1.,1.),(1.,
1.),(1.,1.)))
REPRESENTATION_ITEM('')
SURFACE()
);
#63=(
BOUNDED_SURFACE()
B_SPLINE_SURFACE(5,1,((#47286,#47287),(#47288,#47289),(#47290,#47291),(#47292,
#47293),(#47294,#47295),(#47296,#47297),(#47298,#47299),(#47300,#47301),
(#47302,#47303),(#47304,#47305),(#47306,#47307),(#47308,#47309),(#47310,
#47311),(#47312,#47313),(#47314,#47315),(#47316,#47317),(#47318,#47319),
(#47320,#47321),(#47322,#47323),(#47324,#47325),(#47326,#47327),(#47328,
#47329),(#47330,#47331),(#47332,#47333),(#47334,#47335),(#47336,#47337),
(#47338,#47339),(#47340,#47341),(#47342,#47343),(#47344,#47345),(#47346,
#47347),(#47348,#47349),(#47350,#47351),(#47352,#47353),(#47354,#47355),
(#47356,#47357),(#47358,#47359),(#47360,#47361),(#47362,#47363),(#47364,
#47365),(#47366,#47367),(#47368,#47369),(#47370,#47371),(#47372,#47373),
(#47374,#47375),(#47376,#47377),(#47378,#47379),(#47380,#47381),(#47382,
#47383),(#47384,#47385),(#47386,#47387),(#47388,#47389),(#47390,#47391),
(#47392,#47393),(#47394,#47395),(#47396,#47397),(#47398,#47399),(#47400,
#47401),(#47402,#47403),(#47404,#47405),(#47406,#47407),(#47408,#47409),
(#47410,#47411),(#47412,#47413),(#47414,#47415),(#47416,#47417),(#47418,
#47419),(#47420,#47421),(#47422,#47423),(#47424,#47425)),.UNSPECIFIED.,
 .F.,.F.,.F.)
B_SPLINE_SURFACE_WITH_KNOTS((6,1,1,1,1,1,1,1,1,1,1,1,1,1,1,1,1,1,1,1,1,
1,1,1,1,1,1,1,1,1,1,1,1,1,1,1,1,1,1,1,1,1,1,1,1,1,1,1,1,1,1,1,1,1,1,1,1,
1,1,1,1,1,1,1,1,6),(2,2),(-1.,-0.984615384615383,-0.969230769230768,-0.953846153846152,
-0.938461538461537,-0.923076923076922,-0.907692307692306,-0.892307692307691,
-0.876923076923076,-0.86153846153846,-0.846153846153845,-0.83076923076923,
-0.815384615384614,-0.799999999999999,-0.784615384615384,-0.769230769230768,
-0.753846153846153,-0.738461538461538,-0.723076923076922,-0.707692307692307,
-0.692307692307692,-0.676923076923076,-0.661538461538461,-0.646153846153846,
-0.63076923076923,-0.615384615384615,-0.6,-0.584615384615384,-0.569230769230769,
-0.553846153846154,-0.538461538461538,-0.523076923076923,-0.507692307692308,
-0.492307692307692,-0.476923076923077,-0.461538461538462,-0.446153846153846,
-0.430769230769231,-0.415384615384615,-0.4,-0.384615384615385,-0.369230769230769,
-0.353846153846154,-0.338461538461538,-0.323076923076923,-0.307692307692308,
-0.292307692307692,-0.276923076923077,-0.261538461538462,-0.246153846153846,
-0.230769230769231,-0.215384615384615,-0.2,-0.184615384615385,-0.169230769230769,
-0.153846153846154,-0.138461538461538,-0.123076923076923,-0.107692307692308,
-0.0923076923076923,-0.0769230769230769,-0.0615384615384615,-0.0461538461538462,
-0.0307692307692308,-0.0153846153846154,0.),(-1.,1.),.UNSPECIFIED.)
GEOMETRIC_REPRESENTATION_ITEM()
RATIONAL_B_SPLINE_SURFACE(((1.,1.),(1.,1.),(1.,1.),(1.,1.),(1.,1.),(1.,
1.),(1.,1.),(1.,1.),(1.,1.),(1.,1.),(1.,1.),(1.,1.),(1.,1.),(1.,1.),(1.,
1.),(1.,1.),(1.,1.),(1.,1.),(1.,1.),(1.,1.),(1.,1.),(1.,1.),(1.,1.),(1.,
1.),(1.,1.),(1.,1.),(1.,1.),(1.,1.),(1.,1.),(1.,1.),(1.,1.),(1.,1.),(1.,
1.),(1.,1.),(1.,1.),(1.,1.),(1.,1.),(1.,1.),(1.,1.),(1.,1.),(1.,1.),(1.,
1.),(1.,1.),(1.,1.),(1.,1.),(1.,1.),(1.,1.),(1.,1.),(1.,1.),(1.,1.),(1.,
1.),(1.,1.),(1.,1.),(1.,1.),(1.,1.),(1.,1.),(1.,1.),(1.,1.),(1.,1.),(1.,
1.),(1.,1.),(1.,1.),(1.,1.),(1.,1.),(1.,1.),(1.,1.),(1.,1.),(1.,1.),(1.,
1.),(1.,1.)))
REPRESENTATION_ITEM('')
SURFACE()
);
#64=(
BOUNDED_SURFACE()
B_SPLINE_SURFACE(5,1,((#47498,#47499),(#47500,#47501),(#47502,#47503),(#47504,
#47505),(#47506,#47507),(#47508,#47509),(#47510,#47511),(#47512,#47513),
(#47514,#47515),(#47516,#47517),(#47518,#47519),(#47520,#47521),(#47522,
#47523),(#47524,#47525),(#47526,#47527),(#47528,#47529),(#47530,#47531),
(#47532,#47533),(#47534,#47535),(#47536,#47537),(#47538,#47539),(#47540,
#47541),(#47542,#47543),(#47544,#47545),(#47546,#47547),(#47548,#47549),
(#47550,#47551),(#47552,#47553),(#47554,#47555),(#47556,#47557),(#47558,
#47559),(#47560,#47561),(#47562,#47563),(#47564,#47565),(#47566,#47567),
(#47568,#47569),(#47570,#47571),(#47572,#47573),(#47574,#47575),(#47576,
#47577),(#47578,#47579),(#47580,#47581),(#47582,#47583),(#47584,#47585),
(#47586,#47587),(#47588,#47589),(#47590,#47591),(#47592,#47593),(#47594,
#47595),(#47596,#47597),(#47598,#47599),(#47600,#47601),(#47602,#47603),
(#47604,#47605),(#47606,#47607),(#47608,#47609),(#47610,#47611),(#47612,
#47613),(#47614,#47615),(#47616,#47617),(#47618,#47619),(#47620,#47621),
(#47622,#47623),(#47624,#47625),(#47626,#47627),(#47628,#47629),(#47630,
#47631),(#47632,#47633),(#47634,#47635),(#47636,#47637)),.UNSPECIFIED.,
 .F.,.F.,.F.)
B_SPLINE_SURFACE_WITH_KNOTS((6,1,1,1,1,1,1,1,1,1,1,1,1,1,1,1,1,1,1,1,1,
1,1,1,1,1,1,1,1,1,1,1,1,1,1,1,1,1,1,1,1,1,1,1,1,1,1,1,1,1,1,1,1,1,1,1,1,
1,1,1,1,1,1,1,1,6),(2,2),(-1.,-0.984615384615383,-0.969230769230768,-0.953846153846152,
-0.938461538461537,-0.923076923076922,-0.907692307692306,-0.892307692307691,
-0.876923076923076,-0.86153846153846,-0.846153846153845,-0.83076923076923,
-0.815384615384614,-0.799999999999999,-0.784615384615384,-0.769230769230768,
-0.753846153846153,-0.738461538461538,-0.723076923076922,-0.707692307692307,
-0.692307692307692,-0.676923076923076,-0.661538461538461,-0.646153846153846,
-0.63076923076923,-0.615384615384615,-0.6,-0.584615384615384,-0.569230769230769,
-0.553846153846154,-0.538461538461538,-0.523076923076923,-0.507692307692308,
-0.492307692307692,-0.476923076923077,-0.461538461538462,-0.446153846153846,
-0.430769230769231,-0.415384615384615,-0.4,-0.384615384615385,-0.369230769230769,
-0.353846153846154,-0.338461538461538,-0.323076923076923,-0.307692307692308,
-0.292307692307692,-0.276923076923077,-0.261538461538462,-0.246153846153846,
-0.230769230769231,-0.215384615384615,-0.2,-0.184615384615385,-0.169230769230769,
-0.153846153846154,-0.138461538461538,-0.123076923076923,-0.107692307692308,
-0.0923076923076923,-0.0769230769230769,-0.0615384615384615,-0.0461538461538462,
-0.0307692307692308,-0.0153846153846154,0.),(-1.,1.),.UNSPECIFIED.)
GEOMETRIC_REPRESENTATION_ITEM()
RATIONAL_B_SPLINE_SURFACE(((1.,1.),(1.,1.),(1.,1.),(1.,1.),(1.,1.),(1.,
1.),(1.,1.),(1.,1.),(1.,1.),(1.,1.),(1.,1.),(1.,1.),(1.,1.),(1.,1.),(1.,
1.),(1.,1.),(1.,1.),(1.,1.),(1.,1.),(1.,1.),(1.,1.),(1.,1.),(1.,1.),(1.,
1.),(1.,1.),(1.,1.),(1.,1.),(1.,1.),(1.,1.),(1.,1.),(1.,1.),(1.,1.),(1.,
1.),(1.,1.),(1.,1.),(1.,1.),(1.,1.),(1.,1.),(1.,1.),(1.,1.),(1.,1.),(1.,
1.),(1.,1.),(1.,1.),(1.,1.),(1.,1.),(1.,1.),(1.,1.),(1.,1.),(1.,1.),(1.,
1.),(1.,1.),(1.,1.),(1.,1.),(1.,1.),(1.,1.),(1.,1.),(1.,1.),(1.,1.),(1.,
1.),(1.,1.),(1.,1.),(1.,1.),(1.,1.),(1.,1.),(1.,1.),(1.,1.),(1.,1.),(1.,
1.),(1.,1.)))
REPRESENTATION_ITEM('')
SURFACE()
);
#65=(
BOUNDED_SURFACE()
B_SPLINE_SURFACE(5,1,((#47728,#47729),(#47730,#47731),(#47732,#47733),(#47734,
#47735),(#47736,#47737),(#47738,#47739),(#47740,#47741),(#47742,#47743),
(#47744,#47745),(#47746,#47747),(#47748,#47749),(#47750,#47751),(#47752,
#47753),(#47754,#47755),(#47756,#47757),(#47758,#47759),(#47760,#47761),
(#47762,#47763),(#47764,#47765),(#47766,#47767),(#47768,#47769),(#47770,
#47771),(#47772,#47773),(#47774,#47775),(#47776,#47777),(#47778,#47779),
(#47780,#47781),(#47782,#47783),(#47784,#47785),(#47786,#47787),(#47788,
#47789),(#47790,#47791),(#47792,#47793),(#47794,#47795),(#47796,#47797),
(#47798,#47799),(#47800,#47801),(#47802,#47803),(#47804,#47805),(#47806,
#47807),(#47808,#47809),(#47810,#47811),(#47812,#47813),(#47814,#47815),
(#47816,#47817),(#47818,#47819),(#47820,#47821),(#47822,#47823),(#47824,
#47825),(#47826,#47827),(#47828,#47829),(#47830,#47831),(#47832,#47833),
(#47834,#47835),(#47836,#47837),(#47838,#47839),(#47840,#47841),(#47842,
#47843),(#47844,#47845),(#47846,#47847),(#47848,#47849),(#47850,#47851),
(#47852,#47853),(#47854,#47855),(#47856,#47857),(#47858,#47859),(#47860,
#47861),(#47862,#47863),(#47864,#47865),(#47866,#47867)),.UNSPECIFIED.,
 .F.,.F.,.F.)
B_SPLINE_SURFACE_WITH_KNOTS((6,1,1,1,1,1,1,1,1,1,1,1,1,1,1,1,1,1,1,1,1,
1,1,1,1,1,1,1,1,1,1,1,1,1,1,1,1,1,1,1,1,1,1,1,1,1,1,1,1,1,1,1,1,1,1,1,1,
1,1,1,1,1,1,1,1,6),(2,2),(-1.,-0.984615384615383,-0.969230769230768,-0.953846153846152,
-0.938461538461537,-0.923076923076922,-0.907692307692306,-0.892307692307691,
-0.876923076923076,-0.86153846153846,-0.846153846153845,-0.83076923076923,
-0.815384615384614,-0.799999999999999,-0.784615384615384,-0.769230769230768,
-0.753846153846153,-0.738461538461538,-0.723076923076922,-0.707692307692307,
-0.692307692307692,-0.676923076923076,-0.661538461538461,-0.646153846153846,
-0.63076923076923,-0.615384615384615,-0.6,-0.584615384615384,-0.569230769230769,
-0.553846153846154,-0.538461538461538,-0.523076923076923,-0.507692307692308,
-0.492307692307692,-0.476923076923077,-0.461538461538462,-0.446153846153846,
-0.430769230769231,-0.415384615384615,-0.4,-0.384615384615385,-0.369230769230769,
-0.353846153846154,-0.338461538461538,-0.323076923076923,-0.307692307692308,
-0.292307692307692,-0.276923076923077,-0.261538461538462,-0.246153846153846,
-0.230769230769231,-0.215384615384615,-0.2,-0.184615384615385,-0.169230769230769,
-0.153846153846154,-0.138461538461538,-0.123076923076923,-0.107692307692308,
-0.0923076923076923,-0.0769230769230769,-0.0615384615384615,-0.0461538461538462,
-0.0307692307692308,-0.0153846153846154,0.),(-1.,1.),.UNSPECIFIED.)
GEOMETRIC_REPRESENTATION_ITEM()
RATIONAL_B_SPLINE_SURFACE(((1.,1.),(1.,1.),(1.,1.),(1.,1.),(1.,1.),(1.,
1.),(1.,1.),(1.,1.),(1.,1.),(1.,1.),(1.,1.),(1.,1.),(1.,1.),(1.,1.),(1.,
1.),(1.,1.),(1.,1.),(1.,1.),(1.,1.),(1.,1.),(1.,1.),(1.,1.),(1.,1.),(1.,
1.),(1.,1.),(1.,1.),(1.,1.),(1.,1.),(1.,1.),(1.,1.),(1.,1.),(1.,1.),(1.,
1.),(1.,1.),(1.,1.),(1.,1.),(1.,1.),(1.,1.),(1.,1.),(1.,1.),(1.,1.),(1.,
1.),(1.,1.),(1.,1.),(1.,1.),(1.,1.),(1.,1.),(1.,1.),(1.,1.),(1.,1.),(1.,
1.),(1.,1.),(1.,1.),(1.,1.),(1.,1.),(1.,1.),(1.,1.),(1.,1.),(1.,1.),(1.,
1.),(1.,1.),(1.,1.),(1.,1.),(1.,1.),(1.,1.),(1.,1.),(1.,1.),(1.,1.),(1.,
1.),(1.,1.)))
REPRESENTATION_ITEM('')
SURFACE()
);
#66=(
BOUNDED_SURFACE()
B_SPLINE_SURFACE(5,1,((#47940,#47941),(#47942,#47943),(#47944,#47945),(#47946,
#47947),(#47948,#47949),(#47950,#47951),(#47952,#47953),(#47954,#47955),
(#47956,#47957),(#47958,#47959),(#47960,#47961),(#47962,#47963),(#47964,
#47965),(#47966,#47967),(#47968,#47969),(#47970,#47971),(#47972,#47973),
(#47974,#47975),(#47976,#47977),(#47978,#47979),(#47980,#47981),(#47982,
#47983),(#47984,#47985),(#47986,#47987),(#47988,#47989),(#47990,#47991),
(#47992,#47993),(#47994,#47995),(#47996,#47997),(#47998,#47999),(#48000,
#48001),(#48002,#48003),(#48004,#48005),(#48006,#48007),(#48008,#48009),
(#48010,#48011),(#48012,#48013),(#48014,#48015),(#48016,#48017),(#48018,
#48019),(#48020,#48021),(#48022,#48023),(#48024,#48025),(#48026,#48027),
(#48028,#48029),(#48030,#48031),(#48032,#48033),(#48034,#48035),(#48036,
#48037),(#48038,#48039),(#48040,#48041),(#48042,#48043),(#48044,#48045),
(#48046,#48047),(#48048,#48049),(#48050,#48051),(#48052,#48053),(#48054,
#48055),(#48056,#48057),(#48058,#48059),(#48060,#48061),(#48062,#48063),
(#48064,#48065),(#48066,#48067),(#48068,#48069),(#48070,#48071),(#48072,
#48073),(#48074,#48075),(#48076,#48077),(#48078,#48079)),.UNSPECIFIED.,
 .F.,.F.,.F.)
B_SPLINE_SURFACE_WITH_KNOTS((6,1,1,1,1,1,1,1,1,1,1,1,1,1,1,1,1,1,1,1,1,
1,1,1,1,1,1,1,1,1,1,1,1,1,1,1,1,1,1,1,1,1,1,1,1,1,1,1,1,1,1,1,1,1,1,1,1,
1,1,1,1,1,1,1,1,6),(2,2),(-1.,-0.984615384615383,-0.969230769230768,-0.953846153846152,
-0.938461538461537,-0.923076923076922,-0.907692307692306,-0.892307692307691,
-0.876923076923076,-0.86153846153846,-0.846153846153845,-0.83076923076923,
-0.815384615384614,-0.799999999999999,-0.784615384615384,-0.769230769230768,
-0.753846153846153,-0.738461538461538,-0.723076923076922,-0.707692307692307,
-0.692307692307692,-0.676923076923076,-0.661538461538461,-0.646153846153846,
-0.63076923076923,-0.615384615384615,-0.6,-0.584615384615384,-0.569230769230769,
-0.553846153846154,-0.538461538461538,-0.523076923076923,-0.507692307692308,
-0.492307692307692,-0.476923076923077,-0.461538461538462,-0.446153846153846,
-0.430769230769231,-0.415384615384615,-0.4,-0.384615384615385,-0.369230769230769,
-0.353846153846154,-0.338461538461538,-0.323076923076923,-0.307692307692308,
-0.292307692307692,-0.276923076923077,-0.261538461538462,-0.246153846153846,
-0.230769230769231,-0.215384615384615,-0.2,-0.184615384615385,-0.169230769230769,
-0.153846153846154,-0.138461538461538,-0.123076923076923,-0.107692307692308,
-0.0923076923076923,-0.0769230769230769,-0.0615384615384615,-0.0461538461538462,
-0.0307692307692308,-0.0153846153846154,0.),(-1.,1.),.UNSPECIFIED.)
GEOMETRIC_REPRESENTATION_ITEM()
RATIONAL_B_SPLINE_SURFACE(((1.,1.),(1.,1.),(1.,1.),(1.,1.),(1.,1.),(1.,
1.),(1.,1.),(1.,1.),(1.,1.),(1.,1.),(1.,1.),(1.,1.),(1.,1.),(1.,1.),(1.,
1.),(1.,1.),(1.,1.),(1.,1.),(1.,1.),(1.,1.),(1.,1.),(1.,1.),(1.,1.),(1.,
1.),(1.,1.),(1.,1.),(1.,1.),(1.,1.),(1.,1.),(1.,1.),(1.,1.),(1.,1.),(1.,
1.),(1.,1.),(1.,1.),(1.,1.),(1.,1.),(1.,1.),(1.,1.),(1.,1.),(1.,1.),(1.,
1.),(1.,1.),(1.,1.),(1.,1.),(1.,1.),(1.,1.),(1.,1.),(1.,1.),(1.,1.),(1.,
1.),(1.,1.),(1.,1.),(1.,1.),(1.,1.),(1.,1.),(1.,1.),(1.,1.),(1.,1.),(1.,
1.),(1.,1.),(1.,1.),(1.,1.),(1.,1.),(1.,1.),(1.,1.),(1.,1.),(1.,1.),(1.,
1.),(1.,1.)))
REPRESENTATION_ITEM('')
SURFACE()
);
#67=(
BOUNDED_SURFACE()
B_SPLINE_SURFACE(5,1,((#48170,#48171),(#48172,#48173),(#48174,#48175),(#48176,
#48177),(#48178,#48179),(#48180,#48181),(#48182,#48183),(#48184,#48185),
(#48186,#48187),(#48188,#48189),(#48190,#48191),(#48192,#48193),(#48194,
#48195),(#48196,#48197),(#48198,#48199),(#48200,#48201),(#48202,#48203),
(#48204,#48205),(#48206,#48207),(#48208,#48209),(#48210,#48211),(#48212,
#48213),(#48214,#48215),(#48216,#48217),(#48218,#48219),(#48220,#48221),
(#48222,#48223),(#48224,#48225),(#48226,#48227),(#48228,#48229),(#48230,
#48231),(#48232,#48233),(#48234,#48235),(#48236,#48237),(#48238,#48239),
(#48240,#48241),(#48242,#48243),(#48244,#48245),(#48246,#48247),(#48248,
#48249),(#48250,#48251),(#48252,#48253),(#48254,#48255),(#48256,#48257),
(#48258,#48259),(#48260,#48261),(#48262,#48263),(#48264,#48265),(#48266,
#48267),(#48268,#48269),(#48270,#48271),(#48272,#48273),(#48274,#48275),
(#48276,#48277),(#48278,#48279),(#48280,#48281),(#48282,#48283),(#48284,
#48285),(#48286,#48287),(#48288,#48289),(#48290,#48291),(#48292,#48293),
(#48294,#48295),(#48296,#48297),(#48298,#48299),(#48300,#48301),(#48302,
#48303),(#48304,#48305),(#48306,#48307),(#48308,#48309)),.UNSPECIFIED.,
 .F.,.F.,.F.)
B_SPLINE_SURFACE_WITH_KNOTS((6,1,1,1,1,1,1,1,1,1,1,1,1,1,1,1,1,1,1,1,1,
1,1,1,1,1,1,1,1,1,1,1,1,1,1,1,1,1,1,1,1,1,1,1,1,1,1,1,1,1,1,1,1,1,1,1,1,
1,1,1,1,1,1,1,1,6),(2,2),(-1.,-0.984615384615383,-0.969230769230768,-0.953846153846152,
-0.938461538461537,-0.923076923076922,-0.907692307692306,-0.892307692307691,
-0.876923076923076,-0.86153846153846,-0.846153846153845,-0.83076923076923,
-0.815384615384614,-0.799999999999999,-0.784615384615384,-0.769230769230768,
-0.753846153846153,-0.738461538461538,-0.723076923076922,-0.707692307692307,
-0.692307692307692,-0.676923076923076,-0.661538461538461,-0.646153846153846,
-0.63076923076923,-0.615384615384615,-0.6,-0.584615384615384,-0.569230769230769,
-0.553846153846154,-0.538461538461538,-0.523076923076923,-0.507692307692308,
-0.492307692307692,-0.476923076923077,-0.461538461538462,-0.446153846153846,
-0.430769230769231,-0.415384615384615,-0.4,-0.384615384615385,-0.369230769230769,
-0.353846153846154,-0.338461538461538,-0.323076923076923,-0.307692307692308,
-0.292307692307692,-0.276923076923077,-0.261538461538462,-0.246153846153846,
-0.230769230769231,-0.215384615384615,-0.2,-0.184615384615385,-0.169230769230769,
-0.153846153846154,-0.138461538461538,-0.123076923076923,-0.107692307692308,
-0.0923076923076923,-0.0769230769230769,-0.0615384615384615,-0.0461538461538462,
-0.0307692307692308,-0.0153846153846154,0.),(-1.,1.),.UNSPECIFIED.)
GEOMETRIC_REPRESENTATION_ITEM()
RATIONAL_B_SPLINE_SURFACE(((1.,1.),(1.,1.),(1.,1.),(1.,1.),(1.,1.),(1.,
1.),(1.,1.),(1.,1.),(1.,1.),(1.,1.),(1.,1.),(1.,1.),(1.,1.),(1.,1.),(1.,
1.),(1.,1.),(1.,1.),(1.,1.),(1.,1.),(1.,1.),(1.,1.),(1.,1.),(1.,1.),(1.,
1.),(1.,1.),(1.,1.),(1.,1.),(1.,1.),(1.,1.),(1.,1.),(1.,1.),(1.,1.),(1.,
1.),(1.,1.),(1.,1.),(1.,1.),(1.,1.),(1.,1.),(1.,1.),(1.,1.),(1.,1.),(1.,
1.),(1.,1.),(1.,1.),(1.,1.),(1.,1.),(1.,1.),(1.,1.),(1.,1.),(1.,1.),(1.,
1.),(1.,1.),(1.,1.),(1.,1.),(1.,1.),(1.,1.),(1.,1.),(1.,1.),(1.,1.),(1.,
1.),(1.,1.),(1.,1.),(1.,1.),(1.,1.),(1.,1.),(1.,1.),(1.,1.),(1.,1.),(1.,
1.),(1.,1.)))
REPRESENTATION_ITEM('')
SURFACE()
);
#68=(
BOUNDED_SURFACE()
B_SPLINE_SURFACE(5,1,((#48382,#48383),(#48384,#48385),(#48386,#48387),(#48388,
#48389),(#48390,#48391),(#48392,#48393),(#48394,#48395),(#48396,#48397),
(#48398,#48399),(#48400,#48401),(#48402,#48403),(#48404,#48405),(#48406,
#48407),(#48408,#48409),(#48410,#48411),(#48412,#48413),(#48414,#48415),
(#48416,#48417),(#48418,#48419),(#48420,#48421),(#48422,#48423),(#48424,
#48425),(#48426,#48427),(#48428,#48429),(#48430,#48431),(#48432,#48433),
(#48434,#48435),(#48436,#48437),(#48438,#48439),(#48440,#48441),(#48442,
#48443),(#48444,#48445),(#48446,#48447),(#48448,#48449),(#48450,#48451),
(#48452,#48453),(#48454,#48455),(#48456,#48457),(#48458,#48459),(#48460,
#48461),(#48462,#48463),(#48464,#48465),(#48466,#48467),(#48468,#48469),
(#48470,#48471),(#48472,#48473),(#48474,#48475),(#48476,#48477),(#48478,
#48479),(#48480,#48481),(#48482,#48483),(#48484,#48485),(#48486,#48487),
(#48488,#48489),(#48490,#48491),(#48492,#48493),(#48494,#48495),(#48496,
#48497),(#48498,#48499),(#48500,#48501),(#48502,#48503),(#48504,#48505),
(#48506,#48507),(#48508,#48509),(#48510,#48511),(#48512,#48513),(#48514,
#48515),(#48516,#48517),(#48518,#48519),(#48520,#48521)),.UNSPECIFIED.,
 .F.,.F.,.F.)
B_SPLINE_SURFACE_WITH_KNOTS((6,1,1,1,1,1,1,1,1,1,1,1,1,1,1,1,1,1,1,1,1,
1,1,1,1,1,1,1,1,1,1,1,1,1,1,1,1,1,1,1,1,1,1,1,1,1,1,1,1,1,1,1,1,1,1,1,1,
1,1,1,1,1,1,1,1,6),(2,2),(-1.,-0.984615384615383,-0.969230769230768,-0.953846153846152,
-0.938461538461537,-0.923076923076922,-0.907692307692306,-0.892307692307691,
-0.876923076923076,-0.86153846153846,-0.846153846153845,-0.83076923076923,
-0.815384615384614,-0.799999999999999,-0.784615384615384,-0.769230769230768,
-0.753846153846153,-0.738461538461538,-0.723076923076922,-0.707692307692307,
-0.692307692307692,-0.676923076923076,-0.661538461538461,-0.646153846153846,
-0.63076923076923,-0.615384615384615,-0.6,-0.584615384615384,-0.569230769230769,
-0.553846153846154,-0.538461538461538,-0.523076923076923,-0.507692307692308,
-0.492307692307692,-0.476923076923077,-0.461538461538462,-0.446153846153846,
-0.430769230769231,-0.415384615384615,-0.4,-0.384615384615385,-0.369230769230769,
-0.353846153846154,-0.338461538461538,-0.323076923076923,-0.307692307692308,
-0.292307692307692,-0.276923076923077,-0.261538461538462,-0.246153846153846,
-0.230769230769231,-0.215384615384615,-0.2,-0.184615384615385,-0.169230769230769,
-0.153846153846154,-0.138461538461538,-0.123076923076923,-0.107692307692308,
-0.0923076923076923,-0.0769230769230769,-0.0615384615384615,-0.0461538461538462,
-0.0307692307692308,-0.0153846153846154,0.),(-1.,1.),.UNSPECIFIED.)
GEOMETRIC_REPRESENTATION_ITEM()
RATIONAL_B_SPLINE_SURFACE(((1.,1.),(1.,1.),(1.,1.),(1.,1.),(1.,1.),(1.,
1.),(1.,1.),(1.,1.),(1.,1.),(1.,1.),(1.,1.),(1.,1.),(1.,1.),(1.,1.),(1.,
1.),(1.,1.),(1.,1.),(1.,1.),(1.,1.),(1.,1.),(1.,1.),(1.,1.),(1.,1.),(1.,
1.),(1.,1.),(1.,1.),(1.,1.),(1.,1.),(1.,1.),(1.,1.),(1.,1.),(1.,1.),(1.,
1.),(1.,1.),(1.,1.),(1.,1.),(1.,1.),(1.,1.),(1.,1.),(1.,1.),(1.,1.),(1.,
1.),(1.,1.),(1.,1.),(1.,1.),(1.,1.),(1.,1.),(1.,1.),(1.,1.),(1.,1.),(1.,
1.),(1.,1.),(1.,1.),(1.,1.),(1.,1.),(1.,1.),(1.,1.),(1.,1.),(1.,1.),(1.,
1.),(1.,1.),(1.,1.),(1.,1.),(1.,1.),(1.,1.),(1.,1.),(1.,1.),(1.,1.),(1.,
1.),(1.,1.)))
REPRESENTATION_ITEM('')
SURFACE()
);
#69=(
BOUNDED_SURFACE()
B_SPLINE_SURFACE(5,1,((#48612,#48613),(#48614,#48615),(#48616,#48617),(#48618,
#48619),(#48620,#48621),(#48622,#48623),(#48624,#48625),(#48626,#48627),
(#48628,#48629),(#48630,#48631),(#48632,#48633),(#48634,#48635),(#48636,
#48637),(#48638,#48639),(#48640,#48641),(#48642,#48643),(#48644,#48645),
(#48646,#48647),(#48648,#48649),(#48650,#48651),(#48652,#48653),(#48654,
#48655),(#48656,#48657),(#48658,#48659),(#48660,#48661),(#48662,#48663),
(#48664,#48665),(#48666,#48667),(#48668,#48669),(#48670,#48671),(#48672,
#48673),(#48674,#48675),(#48676,#48677),(#48678,#48679),(#48680,#48681),
(#48682,#48683),(#48684,#48685),(#48686,#48687),(#48688,#48689),(#48690,
#48691),(#48692,#48693),(#48694,#48695),(#48696,#48697),(#48698,#48699),
(#48700,#48701),(#48702,#48703),(#48704,#48705),(#48706,#48707),(#48708,
#48709),(#48710,#48711),(#48712,#48713),(#48714,#48715),(#48716,#48717),
(#48718,#48719),(#48720,#48721),(#48722,#48723),(#48724,#48725),(#48726,
#48727),(#48728,#48729),(#48730,#48731),(#48732,#48733),(#48734,#48735),
(#48736,#48737),(#48738,#48739),(#48740,#48741),(#48742,#48743),(#48744,
#48745),(#48746,#48747),(#48748,#48749),(#48750,#48751)),.UNSPECIFIED.,
 .F.,.F.,.F.)
B_SPLINE_SURFACE_WITH_KNOTS((6,1,1,1,1,1,1,1,1,1,1,1,1,1,1,1,1,1,1,1,1,
1,1,1,1,1,1,1,1,1,1,1,1,1,1,1,1,1,1,1,1,1,1,1,1,1,1,1,1,1,1,1,1,1,1,1,1,
1,1,1,1,1,1,1,1,6),(2,2),(-1.,-0.984615384615383,-0.969230769230768,-0.953846153846152,
-0.938461538461537,-0.923076923076922,-0.907692307692306,-0.892307692307691,
-0.876923076923076,-0.86153846153846,-0.846153846153845,-0.83076923076923,
-0.815384615384614,-0.799999999999999,-0.784615384615384,-0.769230769230768,
-0.753846153846153,-0.738461538461538,-0.723076923076922,-0.707692307692307,
-0.692307692307692,-0.676923076923076,-0.661538461538461,-0.646153846153846,
-0.63076923076923,-0.615384615384615,-0.6,-0.584615384615384,-0.569230769230769,
-0.553846153846154,-0.538461538461538,-0.523076923076923,-0.507692307692308,
-0.492307692307692,-0.476923076923077,-0.461538461538462,-0.446153846153846,
-0.430769230769231,-0.415384615384615,-0.4,-0.384615384615385,-0.369230769230769,
-0.353846153846154,-0.338461538461538,-0.323076923076923,-0.307692307692308,
-0.292307692307692,-0.276923076923077,-0.261538461538462,-0.246153846153846,
-0.230769230769231,-0.215384615384615,-0.2,-0.184615384615385,-0.169230769230769,
-0.153846153846154,-0.138461538461538,-0.123076923076923,-0.107692307692308,
-0.0923076923076923,-0.0769230769230769,-0.0615384615384615,-0.0461538461538462,
-0.0307692307692308,-0.0153846153846154,0.),(-1.,1.),.UNSPECIFIED.)
GEOMETRIC_REPRESENTATION_ITEM()
RATIONAL_B_SPLINE_SURFACE(((1.,1.),(1.,1.),(1.,1.),(1.,1.),(1.,1.),(1.,
1.),(1.,1.),(1.,1.),(1.,1.),(1.,1.),(1.,1.),(1.,1.),(1.,1.),(1.,1.),(1.,
1.),(1.,1.),(1.,1.),(1.,1.),(1.,1.),(1.,1.),(1.,1.),(1.,1.),(1.,1.),(1.,
1.),(1.,1.),(1.,1.),(1.,1.),(1.,1.),(1.,1.),(1.,1.),(1.,1.),(1.,1.),(1.,
1.),(1.,1.),(1.,1.),(1.,1.),(1.,1.),(1.,1.),(1.,1.),(1.,1.),(1.,1.),(1.,
1.),(1.,1.),(1.,1.),(1.,1.),(1.,1.),(1.,1.),(1.,1.),(1.,1.),(1.,1.),(1.,
1.),(1.,1.),(1.,1.),(1.,1.),(1.,1.),(1.,1.),(1.,1.),(1.,1.),(1.,1.),(1.,
1.),(1.,1.),(1.,1.),(1.,1.),(1.,1.),(1.,1.),(1.,1.),(1.,1.),(1.,1.),(1.,
1.),(1.,1.)))
REPRESENTATION_ITEM('')
SURFACE()
);
#70=(
BOUNDED_SURFACE()
B_SPLINE_SURFACE(5,1,((#48824,#48825),(#48826,#48827),(#48828,#48829),(#48830,
#48831),(#48832,#48833),(#48834,#48835),(#48836,#48837),(#48838,#48839),
(#48840,#48841),(#48842,#48843),(#48844,#48845),(#48846,#48847),(#48848,
#48849),(#48850,#48851),(#48852,#48853),(#48854,#48855),(#48856,#48857),
(#48858,#48859),(#48860,#48861),(#48862,#48863),(#48864,#48865),(#48866,
#48867),(#48868,#48869),(#48870,#48871),(#48872,#48873),(#48874,#48875),
(#48876,#48877),(#48878,#48879),(#48880,#48881),(#48882,#48883),(#48884,
#48885),(#48886,#48887),(#48888,#48889),(#48890,#48891),(#48892,#48893),
(#48894,#48895),(#48896,#48897),(#48898,#48899),(#48900,#48901),(#48902,
#48903),(#48904,#48905),(#48906,#48907),(#48908,#48909),(#48910,#48911),
(#48912,#48913),(#48914,#48915),(#48916,#48917),(#48918,#48919),(#48920,
#48921),(#48922,#48923),(#48924,#48925),(#48926,#48927),(#48928,#48929),
(#48930,#48931),(#48932,#48933),(#48934,#48935),(#48936,#48937),(#48938,
#48939),(#48940,#48941),(#48942,#48943),(#48944,#48945),(#48946,#48947),
(#48948,#48949),(#48950,#48951),(#48952,#48953),(#48954,#48955),(#48956,
#48957),(#48958,#48959),(#48960,#48961),(#48962,#48963)),.UNSPECIFIED.,
 .F.,.F.,.F.)
B_SPLINE_SURFACE_WITH_KNOTS((6,1,1,1,1,1,1,1,1,1,1,1,1,1,1,1,1,1,1,1,1,
1,1,1,1,1,1,1,1,1,1,1,1,1,1,1,1,1,1,1,1,1,1,1,1,1,1,1,1,1,1,1,1,1,1,1,1,
1,1,1,1,1,1,1,1,6),(2,2),(-1.,-0.984615384615383,-0.969230769230768,-0.953846153846152,
-0.938461538461537,-0.923076923076922,-0.907692307692306,-0.892307692307691,
-0.876923076923076,-0.86153846153846,-0.846153846153845,-0.83076923076923,
-0.815384615384614,-0.799999999999999,-0.784615384615384,-0.769230769230768,
-0.753846153846153,-0.738461538461538,-0.723076923076922,-0.707692307692307,
-0.692307692307692,-0.676923076923076,-0.661538461538461,-0.646153846153846,
-0.63076923076923,-0.615384615384615,-0.6,-0.584615384615384,-0.569230769230769,
-0.553846153846154,-0.538461538461538,-0.523076923076923,-0.507692307692308,
-0.492307692307692,-0.476923076923077,-0.461538461538462,-0.446153846153846,
-0.430769230769231,-0.415384615384615,-0.4,-0.384615384615385,-0.369230769230769,
-0.353846153846154,-0.338461538461538,-0.323076923076923,-0.307692307692308,
-0.292307692307692,-0.276923076923077,-0.261538461538462,-0.246153846153846,
-0.230769230769231,-0.215384615384615,-0.2,-0.184615384615385,-0.169230769230769,
-0.153846153846154,-0.138461538461538,-0.123076923076923,-0.107692307692308,
-0.0923076923076923,-0.0769230769230769,-0.0615384615384615,-0.0461538461538462,
-0.0307692307692308,-0.0153846153846154,0.),(-1.,1.),.UNSPECIFIED.)
GEOMETRIC_REPRESENTATION_ITEM()
RATIONAL_B_SPLINE_SURFACE(((1.,1.),(1.,1.),(1.,1.),(1.,1.),(1.,1.),(1.,
1.),(1.,1.),(1.,1.),(1.,1.),(1.,1.),(1.,1.),(1.,1.),(1.,1.),(1.,1.),(1.,
1.),(1.,1.),(1.,1.),(1.,1.),(1.,1.),(1.,1.),(1.,1.),(1.,1.),(1.,1.),(1.,
1.),(1.,1.),(1.,1.),(1.,1.),(1.,1.),(1.,1.),(1.,1.),(1.,1.),(1.,1.),(1.,
1.),(1.,1.),(1.,1.),(1.,1.),(1.,1.),(1.,1.),(1.,1.),(1.,1.),(1.,1.),(1.,
1.),(1.,1.),(1.,1.),(1.,1.),(1.,1.),(1.,1.),(1.,1.),(1.,1.),(1.,1.),(1.,
1.),(1.,1.),(1.,1.),(1.,1.),(1.,1.),(1.,1.),(1.,1.),(1.,1.),(1.,1.),(1.,
1.),(1.,1.),(1.,1.),(1.,1.),(1.,1.),(1.,1.),(1.,1.),(1.,1.),(1.,1.),(1.,
1.),(1.,1.)))
REPRESENTATION_ITEM('')
SURFACE()
);
#71=(
BOUNDED_SURFACE()
B_SPLINE_SURFACE(5,1,((#49054,#49055),(#49056,#49057),(#49058,#49059),(#49060,
#49061),(#49062,#49063),(#49064,#49065),(#49066,#49067),(#49068,#49069),
(#49070,#49071),(#49072,#49073),(#49074,#49075),(#49076,#49077),(#49078,
#49079),(#49080,#49081),(#49082,#49083),(#49084,#49085),(#49086,#49087),
(#49088,#49089),(#49090,#49091),(#49092,#49093),(#49094,#49095),(#49096,
#49097),(#49098,#49099),(#49100,#49101),(#49102,#49103),(#49104,#49105),
(#49106,#49107),(#49108,#49109),(#49110,#49111),(#49112,#49113),(#49114,
#49115),(#49116,#49117),(#49118,#49119),(#49120,#49121),(#49122,#49123),
(#49124,#49125),(#49126,#49127),(#49128,#49129),(#49130,#49131),(#49132,
#49133),(#49134,#49135),(#49136,#49137),(#49138,#49139),(#49140,#49141),
(#49142,#49143),(#49144,#49145),(#49146,#49147),(#49148,#49149),(#49150,
#49151),(#49152,#49153),(#49154,#49155),(#49156,#49157),(#49158,#49159),
(#49160,#49161),(#49162,#49163),(#49164,#49165),(#49166,#49167),(#49168,
#49169),(#49170,#49171),(#49172,#49173),(#49174,#49175),(#49176,#49177),
(#49178,#49179),(#49180,#49181),(#49182,#49183),(#49184,#49185),(#49186,
#49187),(#49188,#49189),(#49190,#49191),(#49192,#49193)),.UNSPECIFIED.,
 .F.,.F.,.F.)
B_SPLINE_SURFACE_WITH_KNOTS((6,1,1,1,1,1,1,1,1,1,1,1,1,1,1,1,1,1,1,1,1,
1,1,1,1,1,1,1,1,1,1,1,1,1,1,1,1,1,1,1,1,1,1,1,1,1,1,1,1,1,1,1,1,1,1,1,1,
1,1,1,1,1,1,1,1,6),(2,2),(-1.,-0.984615384615383,-0.969230769230768,-0.953846153846152,
-0.938461538461537,-0.923076923076922,-0.907692307692306,-0.892307692307691,
-0.876923076923076,-0.86153846153846,-0.846153846153845,-0.83076923076923,
-0.815384615384614,-0.799999999999999,-0.784615384615384,-0.769230769230768,
-0.753846153846153,-0.738461538461538,-0.723076923076922,-0.707692307692307,
-0.692307692307692,-0.676923076923076,-0.661538461538461,-0.646153846153846,
-0.63076923076923,-0.615384615384615,-0.6,-0.584615384615384,-0.569230769230769,
-0.553846153846154,-0.538461538461538,-0.523076923076923,-0.507692307692308,
-0.492307692307692,-0.476923076923077,-0.461538461538462,-0.446153846153846,
-0.430769230769231,-0.415384615384615,-0.4,-0.384615384615385,-0.369230769230769,
-0.353846153846154,-0.338461538461538,-0.323076923076923,-0.307692307692308,
-0.292307692307692,-0.276923076923077,-0.261538461538462,-0.246153846153846,
-0.230769230769231,-0.215384615384615,-0.2,-0.184615384615385,-0.169230769230769,
-0.153846153846154,-0.138461538461538,-0.123076923076923,-0.107692307692308,
-0.0923076923076923,-0.0769230769230769,-0.0615384615384615,-0.0461538461538462,
-0.0307692307692308,-0.0153846153846154,0.),(-1.,1.),.UNSPECIFIED.)
GEOMETRIC_REPRESENTATION_ITEM()
RATIONAL_B_SPLINE_SURFACE(((1.,1.),(1.,1.),(1.,1.),(1.,1.),(1.,1.),(1.,
1.),(1.,1.),(1.,1.),(1.,1.),(1.,1.),(1.,1.),(1.,1.),(1.,1.),(1.,1.),(1.,
1.),(1.,1.),(1.,1.),(1.,1.),(1.,1.),(1.,1.),(1.,1.),(1.,1.),(1.,1.),(1.,
1.),(1.,1.),(1.,1.),(1.,1.),(1.,1.),(1.,1.),(1.,1.),(1.,1.),(1.,1.),(1.,
1.),(1.,1.),(1.,1.),(1.,1.),(1.,1.),(1.,1.),(1.,1.),(1.,1.),(1.,1.),(1.,
1.),(1.,1.),(1.,1.),(1.,1.),(1.,1.),(1.,1.),(1.,1.),(1.,1.),(1.,1.),(1.,
1.),(1.,1.),(1.,1.),(1.,1.),(1.,1.),(1.,1.),(1.,1.),(1.,1.),(1.,1.),(1.,
1.),(1.,1.),(1.,1.),(1.,1.),(1.,1.),(1.,1.),(1.,1.),(1.,1.),(1.,1.),(1.,
1.),(1.,1.)))
REPRESENTATION_ITEM('')
SURFACE()
);
#72=(
BOUNDED_SURFACE()
B_SPLINE_SURFACE(5,1,((#49266,#49267),(#49268,#49269),(#49270,#49271),(#49272,
#49273),(#49274,#49275),(#49276,#49277),(#49278,#49279),(#49280,#49281),
(#49282,#49283),(#49284,#49285),(#49286,#49287),(#49288,#49289),(#49290,
#49291),(#49292,#49293),(#49294,#49295),(#49296,#49297),(#49298,#49299),
(#49300,#49301),(#49302,#49303),(#49304,#49305),(#49306,#49307),(#49308,
#49309),(#49310,#49311),(#49312,#49313),(#49314,#49315),(#49316,#49317),
(#49318,#49319),(#49320,#49321),(#49322,#49323),(#49324,#49325),(#49326,
#49327),(#49328,#49329),(#49330,#49331),(#49332,#49333),(#49334,#49335),
(#49336,#49337),(#49338,#49339),(#49340,#49341),(#49342,#49343),(#49344,
#49345),(#49346,#49347),(#49348,#49349),(#49350,#49351),(#49352,#49353),
(#49354,#49355),(#49356,#49357),(#49358,#49359),(#49360,#49361),(#49362,
#49363),(#49364,#49365),(#49366,#49367),(#49368,#49369),(#49370,#49371),
(#49372,#49373),(#49374,#49375),(#49376,#49377),(#49378,#49379),(#49380,
#49381),(#49382,#49383),(#49384,#49385),(#49386,#49387),(#49388,#49389),
(#49390,#49391),(#49392,#49393),(#49394,#49395),(#49396,#49397),(#49398,
#49399),(#49400,#49401),(#49402,#49403),(#49404,#49405)),.UNSPECIFIED.,
 .F.,.F.,.F.)
B_SPLINE_SURFACE_WITH_KNOTS((6,1,1,1,1,1,1,1,1,1,1,1,1,1,1,1,1,1,1,1,1,
1,1,1,1,1,1,1,1,1,1,1,1,1,1,1,1,1,1,1,1,1,1,1,1,1,1,1,1,1,1,1,1,1,1,1,1,
1,1,1,1,1,1,1,1,6),(2,2),(-1.,-0.984615384615383,-0.969230769230768,-0.953846153846152,
-0.938461538461537,-0.923076923076922,-0.907692307692306,-0.892307692307691,
-0.876923076923076,-0.86153846153846,-0.846153846153845,-0.83076923076923,
-0.815384615384614,-0.799999999999999,-0.784615384615384,-0.769230769230768,
-0.753846153846153,-0.738461538461538,-0.723076923076922,-0.707692307692307,
-0.692307692307692,-0.676923076923076,-0.661538461538461,-0.646153846153846,
-0.63076923076923,-0.615384615384615,-0.6,-0.584615384615384,-0.569230769230769,
-0.553846153846154,-0.538461538461538,-0.523076923076923,-0.507692307692308,
-0.492307692307692,-0.476923076923077,-0.461538461538462,-0.446153846153846,
-0.430769230769231,-0.415384615384615,-0.4,-0.384615384615385,-0.369230769230769,
-0.353846153846154,-0.338461538461538,-0.323076923076923,-0.307692307692308,
-0.292307692307692,-0.276923076923077,-0.261538461538462,-0.246153846153846,
-0.230769230769231,-0.215384615384615,-0.2,-0.184615384615385,-0.169230769230769,
-0.153846153846154,-0.138461538461538,-0.123076923076923,-0.107692307692308,
-0.0923076923076923,-0.0769230769230769,-0.0615384615384615,-0.0461538461538462,
-0.0307692307692308,-0.0153846153846154,0.),(-1.,1.),.UNSPECIFIED.)
GEOMETRIC_REPRESENTATION_ITEM()
RATIONAL_B_SPLINE_SURFACE(((1.,1.),(1.,1.),(1.,1.),(1.,1.),(1.,1.),(1.,
1.),(1.,1.),(1.,1.),(1.,1.),(1.,1.),(1.,1.),(1.,1.),(1.,1.),(1.,1.),(1.,
1.),(1.,1.),(1.,1.),(1.,1.),(1.,1.),(1.,1.),(1.,1.),(1.,1.),(1.,1.),(1.,
1.),(1.,1.),(1.,1.),(1.,1.),(1.,1.),(1.,1.),(1.,1.),(1.,1.),(1.,1.),(1.,
1.),(1.,1.),(1.,1.),(1.,1.),(1.,1.),(1.,1.),(1.,1.),(1.,1.),(1.,1.),(1.,
1.),(1.,1.),(1.,1.),(1.,1.),(1.,1.),(1.,1.),(1.,1.),(1.,1.),(1.,1.),(1.,
1.),(1.,1.),(1.,1.),(1.,1.),(1.,1.),(1.,1.),(1.,1.),(1.,1.),(1.,1.),(1.,
1.),(1.,1.),(1.,1.),(1.,1.),(1.,1.),(1.,1.),(1.,1.),(1.,1.),(1.,1.),(1.,
1.),(1.,1.)))
REPRESENTATION_ITEM('')
SURFACE()
);
#73=(
BOUNDED_SURFACE()
B_SPLINE_SURFACE(5,1,((#49496,#49497),(#49498,#49499),(#49500,#49501),(#49502,
#49503),(#49504,#49505),(#49506,#49507),(#49508,#49509),(#49510,#49511),
(#49512,#49513),(#49514,#49515),(#49516,#49517),(#49518,#49519),(#49520,
#49521),(#49522,#49523),(#49524,#49525),(#49526,#49527),(#49528,#49529),
(#49530,#49531),(#49532,#49533),(#49534,#49535),(#49536,#49537),(#49538,
#49539),(#49540,#49541),(#49542,#49543),(#49544,#49545),(#49546,#49547),
(#49548,#49549),(#49550,#49551),(#49552,#49553),(#49554,#49555),(#49556,
#49557),(#49558,#49559),(#49560,#49561),(#49562,#49563),(#49564,#49565),
(#49566,#49567),(#49568,#49569),(#49570,#49571),(#49572,#49573),(#49574,
#49575),(#49576,#49577),(#49578,#49579),(#49580,#49581),(#49582,#49583),
(#49584,#49585),(#49586,#49587),(#49588,#49589),(#49590,#49591),(#49592,
#49593),(#49594,#49595),(#49596,#49597),(#49598,#49599),(#49600,#49601),
(#49602,#49603),(#49604,#49605),(#49606,#49607),(#49608,#49609),(#49610,
#49611),(#49612,#49613),(#49614,#49615),(#49616,#49617),(#49618,#49619),
(#49620,#49621),(#49622,#49623),(#49624,#49625),(#49626,#49627),(#49628,
#49629),(#49630,#49631),(#49632,#49633),(#49634,#49635)),.UNSPECIFIED.,
 .F.,.F.,.F.)
B_SPLINE_SURFACE_WITH_KNOTS((6,1,1,1,1,1,1,1,1,1,1,1,1,1,1,1,1,1,1,1,1,
1,1,1,1,1,1,1,1,1,1,1,1,1,1,1,1,1,1,1,1,1,1,1,1,1,1,1,1,1,1,1,1,1,1,1,1,
1,1,1,1,1,1,1,1,6),(2,2),(-1.,-0.984615384615383,-0.969230769230768,-0.953846153846152,
-0.938461538461537,-0.923076923076922,-0.907692307692306,-0.892307692307691,
-0.876923076923076,-0.86153846153846,-0.846153846153845,-0.83076923076923,
-0.815384615384614,-0.799999999999999,-0.784615384615384,-0.769230769230768,
-0.753846153846153,-0.738461538461538,-0.723076923076922,-0.707692307692307,
-0.692307692307692,-0.676923076923076,-0.661538461538461,-0.646153846153846,
-0.63076923076923,-0.615384615384615,-0.6,-0.584615384615384,-0.569230769230769,
-0.553846153846154,-0.538461538461538,-0.523076923076923,-0.507692307692308,
-0.492307692307692,-0.476923076923077,-0.461538461538462,-0.446153846153846,
-0.430769230769231,-0.415384615384615,-0.4,-0.384615384615385,-0.369230769230769,
-0.353846153846154,-0.338461538461538,-0.323076923076923,-0.307692307692308,
-0.292307692307692,-0.276923076923077,-0.261538461538462,-0.246153846153846,
-0.230769230769231,-0.215384615384615,-0.2,-0.184615384615385,-0.169230769230769,
-0.153846153846154,-0.138461538461538,-0.123076923076923,-0.107692307692308,
-0.0923076923076923,-0.0769230769230769,-0.0615384615384615,-0.0461538461538462,
-0.0307692307692308,-0.0153846153846154,0.),(-1.,1.),.UNSPECIFIED.)
GEOMETRIC_REPRESENTATION_ITEM()
RATIONAL_B_SPLINE_SURFACE(((1.,1.),(1.,1.),(1.,1.),(1.,1.),(1.,1.),(1.,
1.),(1.,1.),(1.,1.),(1.,1.),(1.,1.),(1.,1.),(1.,1.),(1.,1.),(1.,1.),(1.,
1.),(1.,1.),(1.,1.),(1.,1.),(1.,1.),(1.,1.),(1.,1.),(1.,1.),(1.,1.),(1.,
1.),(1.,1.),(1.,1.),(1.,1.),(1.,1.),(1.,1.),(1.,1.),(1.,1.),(1.,1.),(1.,
1.),(1.,1.),(1.,1.),(1.,1.),(1.,1.),(1.,1.),(1.,1.),(1.,1.),(1.,1.),(1.,
1.),(1.,1.),(1.,1.),(1.,1.),(1.,1.),(1.,1.),(1.,1.),(1.,1.),(1.,1.),(1.,
1.),(1.,1.),(1.,1.),(1.,1.),(1.,1.),(1.,1.),(1.,1.),(1.,1.),(1.,1.),(1.,
1.),(1.,1.),(1.,1.),(1.,1.),(1.,1.),(1.,1.),(1.,1.),(1.,1.),(1.,1.),(1.,
1.),(1.,1.)))
REPRESENTATION_ITEM('')
SURFACE()
);
#74=(
BOUNDED_SURFACE()
B_SPLINE_SURFACE(5,1,((#49708,#49709),(#49710,#49711),(#49712,#49713),(#49714,
#49715),(#49716,#49717),(#49718,#49719),(#49720,#49721),(#49722,#49723),
(#49724,#49725),(#49726,#49727),(#49728,#49729),(#49730,#49731),(#49732,
#49733),(#49734,#49735),(#49736,#49737),(#49738,#49739),(#49740,#49741),
(#49742,#49743),(#49744,#49745),(#49746,#49747),(#49748,#49749),(#49750,
#49751),(#49752,#49753),(#49754,#49755),(#49756,#49757),(#49758,#49759),
(#49760,#49761),(#49762,#49763),(#49764,#49765),(#49766,#49767),(#49768,
#49769),(#49770,#49771),(#49772,#49773),(#49774,#49775),(#49776,#49777),
(#49778,#49779),(#49780,#49781),(#49782,#49783),(#49784,#49785),(#49786,
#49787),(#49788,#49789),(#49790,#49791),(#49792,#49793),(#49794,#49795),
(#49796,#49797),(#49798,#49799),(#49800,#49801),(#49802,#49803),(#49804,
#49805),(#49806,#49807),(#49808,#49809),(#49810,#49811),(#49812,#49813),
(#49814,#49815),(#49816,#49817),(#49818,#49819),(#49820,#49821),(#49822,
#49823),(#49824,#49825),(#49826,#49827),(#49828,#49829),(#49830,#49831),
(#49832,#49833),(#49834,#49835),(#49836,#49837),(#49838,#49839),(#49840,
#49841),(#49842,#49843),(#49844,#49845),(#49846,#49847)),.UNSPECIFIED.,
 .F.,.F.,.F.)
B_SPLINE_SURFACE_WITH_KNOTS((6,1,1,1,1,1,1,1,1,1,1,1,1,1,1,1,1,1,1,1,1,
1,1,1,1,1,1,1,1,1,1,1,1,1,1,1,1,1,1,1,1,1,1,1,1,1,1,1,1,1,1,1,1,1,1,1,1,
1,1,1,1,1,1,1,1,6),(2,2),(-1.,-0.984615384615383,-0.969230769230768,-0.953846153846152,
-0.938461538461537,-0.923076923076922,-0.907692307692306,-0.892307692307691,
-0.876923076923076,-0.86153846153846,-0.846153846153845,-0.83076923076923,
-0.815384615384614,-0.799999999999999,-0.784615384615384,-0.769230769230768,
-0.753846153846153,-0.738461538461538,-0.723076923076922,-0.707692307692307,
-0.692307692307692,-0.676923076923076,-0.661538461538461,-0.646153846153846,
-0.63076923076923,-0.615384615384615,-0.6,-0.584615384615384,-0.569230769230769,
-0.553846153846154,-0.538461538461538,-0.523076923076923,-0.507692307692308,
-0.492307692307692,-0.476923076923077,-0.461538461538462,-0.446153846153846,
-0.430769230769231,-0.415384615384615,-0.4,-0.384615384615385,-0.369230769230769,
-0.353846153846154,-0.338461538461538,-0.323076923076923,-0.307692307692308,
-0.292307692307692,-0.276923076923077,-0.261538461538462,-0.246153846153846,
-0.230769230769231,-0.215384615384615,-0.2,-0.184615384615385,-0.169230769230769,
-0.153846153846154,-0.138461538461538,-0.123076923076923,-0.107692307692308,
-0.0923076923076923,-0.0769230769230769,-0.0615384615384615,-0.0461538461538462,
-0.0307692307692308,-0.0153846153846154,0.),(-1.,1.),.UNSPECIFIED.)
GEOMETRIC_REPRESENTATION_ITEM()
RATIONAL_B_SPLINE_SURFACE(((1.,1.),(1.,1.),(1.,1.),(1.,1.),(1.,1.),(1.,
1.),(1.,1.),(1.,1.),(1.,1.),(1.,1.),(1.,1.),(1.,1.),(1.,1.),(1.,1.),(1.,
1.),(1.,1.),(1.,1.),(1.,1.),(1.,1.),(1.,1.),(1.,1.),(1.,1.),(1.,1.),(1.,
1.),(1.,1.),(1.,1.),(1.,1.),(1.,1.),(1.,1.),(1.,1.),(1.,1.),(1.,1.),(1.,
1.),(1.,1.),(1.,1.),(1.,1.),(1.,1.),(1.,1.),(1.,1.),(1.,1.),(1.,1.),(1.,
1.),(1.,1.),(1.,1.),(1.,1.),(1.,1.),(1.,1.),(1.,1.),(1.,1.),(1.,1.),(1.,
1.),(1.,1.),(1.,1.),(1.,1.),(1.,1.),(1.,1.),(1.,1.),(1.,1.),(1.,1.),(1.,
1.),(1.,1.),(1.,1.),(1.,1.),(1.,1.),(1.,1.),(1.,1.),(1.,1.),(1.,1.),(1.,
1.),(1.,1.)))
REPRESENTATION_ITEM('')
SURFACE()
);
#75=(
BOUNDED_SURFACE()
B_SPLINE_SURFACE(5,1,((#49938,#49939),(#49940,#49941),(#49942,#49943),(#49944,
#49945),(#49946,#49947),(#49948,#49949),(#49950,#49951),(#49952,#49953),
(#49954,#49955),(#49956,#49957),(#49958,#49959),(#49960,#49961),(#49962,
#49963),(#49964,#49965),(#49966,#49967),(#49968,#49969),(#49970,#49971),
(#49972,#49973),(#49974,#49975),(#49976,#49977),(#49978,#49979),(#49980,
#49981),(#49982,#49983),(#49984,#49985),(#49986,#49987),(#49988,#49989),
(#49990,#49991),(#49992,#49993),(#49994,#49995),(#49996,#49997),(#49998,
#49999),(#50000,#50001),(#50002,#50003),(#50004,#50005),(#50006,#50007),
(#50008,#50009),(#50010,#50011),(#50012,#50013),(#50014,#50015),(#50016,
#50017),(#50018,#50019),(#50020,#50021),(#50022,#50023),(#50024,#50025),
(#50026,#50027),(#50028,#50029),(#50030,#50031),(#50032,#50033),(#50034,
#50035),(#50036,#50037),(#50038,#50039),(#50040,#50041),(#50042,#50043),
(#50044,#50045),(#50046,#50047),(#50048,#50049),(#50050,#50051),(#50052,
#50053),(#50054,#50055),(#50056,#50057),(#50058,#50059),(#50060,#50061),
(#50062,#50063),(#50064,#50065),(#50066,#50067),(#50068,#50069),(#50070,
#50071),(#50072,#50073),(#50074,#50075),(#50076,#50077)),.UNSPECIFIED.,
 .F.,.F.,.F.)
B_SPLINE_SURFACE_WITH_KNOTS((6,1,1,1,1,1,1,1,1,1,1,1,1,1,1,1,1,1,1,1,1,
1,1,1,1,1,1,1,1,1,1,1,1,1,1,1,1,1,1,1,1,1,1,1,1,1,1,1,1,1,1,1,1,1,1,1,1,
1,1,1,1,1,1,1,1,6),(2,2),(-1.,-0.984615384615383,-0.969230769230768,-0.953846153846152,
-0.938461538461537,-0.923076923076922,-0.907692307692306,-0.892307692307691,
-0.876923076923076,-0.86153846153846,-0.846153846153845,-0.83076923076923,
-0.815384615384614,-0.799999999999999,-0.784615384615384,-0.769230769230768,
-0.753846153846153,-0.738461538461538,-0.723076923076922,-0.707692307692307,
-0.692307692307692,-0.676923076923076,-0.661538461538461,-0.646153846153846,
-0.63076923076923,-0.615384615384615,-0.6,-0.584615384615384,-0.569230769230769,
-0.553846153846154,-0.538461538461538,-0.523076923076923,-0.507692307692308,
-0.492307692307692,-0.476923076923077,-0.461538461538462,-0.446153846153846,
-0.430769230769231,-0.415384615384615,-0.4,-0.384615384615385,-0.369230769230769,
-0.353846153846154,-0.338461538461538,-0.323076923076923,-0.307692307692308,
-0.292307692307692,-0.276923076923077,-0.261538461538462,-0.246153846153846,
-0.230769230769231,-0.215384615384615,-0.2,-0.184615384615385,-0.169230769230769,
-0.153846153846154,-0.138461538461538,-0.123076923076923,-0.107692307692308,
-0.0923076923076923,-0.0769230769230769,-0.0615384615384615,-0.0461538461538462,
-0.0307692307692308,-0.0153846153846154,0.),(-1.,1.),.UNSPECIFIED.)
GEOMETRIC_REPRESENTATION_ITEM()
RATIONAL_B_SPLINE_SURFACE(((1.,1.),(1.,1.),(1.,1.),(1.,1.),(1.,1.),(1.,
1.),(1.,1.),(1.,1.),(1.,1.),(1.,1.),(1.,1.),(1.,1.),(1.,1.),(1.,1.),(1.,
1.),(1.,1.),(1.,1.),(1.,1.),(1.,1.),(1.,1.),(1.,1.),(1.,1.),(1.,1.),(1.,
1.),(1.,1.),(1.,1.),(1.,1.),(1.,1.),(1.,1.),(1.,1.),(1.,1.),(1.,1.),(1.,
1.),(1.,1.),(1.,1.),(1.,1.),(1.,1.),(1.,1.),(1.,1.),(1.,1.),(1.,1.),(1.,
1.),(1.,1.),(1.,1.),(1.,1.),(1.,1.),(1.,1.),(1.,1.),(1.,1.),(1.,1.),(1.,
1.),(1.,1.),(1.,1.),(1.,1.),(1.,1.),(1.,1.),(1.,1.),(1.,1.),(1.,1.),(1.,
1.),(1.,1.),(1.,1.),(1.,1.),(1.,1.),(1.,1.),(1.,1.),(1.,1.),(1.,1.),(1.,
1.),(1.,1.)))
REPRESENTATION_ITEM('')
SURFACE()
);
#76=(
BOUNDED_SURFACE()
B_SPLINE_SURFACE(5,1,((#50150,#50151),(#50152,#50153),(#50154,#50155),(#50156,
#50157),(#50158,#50159),(#50160,#50161),(#50162,#50163),(#50164,#50165),
(#50166,#50167),(#50168,#50169),(#50170,#50171),(#50172,#50173),(#50174,
#50175),(#50176,#50177),(#50178,#50179),(#50180,#50181),(#50182,#50183),
(#50184,#50185),(#50186,#50187),(#50188,#50189),(#50190,#50191),(#50192,
#50193),(#50194,#50195),(#50196,#50197),(#50198,#50199),(#50200,#50201),
(#50202,#50203),(#50204,#50205),(#50206,#50207),(#50208,#50209),(#50210,
#50211),(#50212,#50213),(#50214,#50215),(#50216,#50217),(#50218,#50219),
(#50220,#50221),(#50222,#50223),(#50224,#50225),(#50226,#50227),(#50228,
#50229),(#50230,#50231),(#50232,#50233),(#50234,#50235),(#50236,#50237),
(#50238,#50239),(#50240,#50241),(#50242,#50243),(#50244,#50245),(#50246,
#50247),(#50248,#50249),(#50250,#50251),(#50252,#50253),(#50254,#50255),
(#50256,#50257),(#50258,#50259),(#50260,#50261),(#50262,#50263),(#50264,
#50265),(#50266,#50267),(#50268,#50269),(#50270,#50271),(#50272,#50273),
(#50274,#50275),(#50276,#50277),(#50278,#50279),(#50280,#50281),(#50282,
#50283),(#50284,#50285),(#50286,#50287),(#50288,#50289)),.UNSPECIFIED.,
 .F.,.F.,.F.)
B_SPLINE_SURFACE_WITH_KNOTS((6,1,1,1,1,1,1,1,1,1,1,1,1,1,1,1,1,1,1,1,1,
1,1,1,1,1,1,1,1,1,1,1,1,1,1,1,1,1,1,1,1,1,1,1,1,1,1,1,1,1,1,1,1,1,1,1,1,
1,1,1,1,1,1,1,1,6),(2,2),(-1.,-0.984615384615383,-0.969230769230768,-0.953846153846152,
-0.938461538461537,-0.923076923076922,-0.907692307692306,-0.892307692307691,
-0.876923076923076,-0.86153846153846,-0.846153846153845,-0.83076923076923,
-0.815384615384614,-0.799999999999999,-0.784615384615384,-0.769230769230768,
-0.753846153846153,-0.738461538461538,-0.723076923076922,-0.707692307692307,
-0.692307692307692,-0.676923076923076,-0.661538461538461,-0.646153846153846,
-0.63076923076923,-0.615384615384615,-0.6,-0.584615384615384,-0.569230769230769,
-0.553846153846154,-0.538461538461538,-0.523076923076923,-0.507692307692308,
-0.492307692307692,-0.476923076923077,-0.461538461538462,-0.446153846153846,
-0.430769230769231,-0.415384615384615,-0.4,-0.384615384615385,-0.369230769230769,
-0.353846153846154,-0.338461538461538,-0.323076923076923,-0.307692307692308,
-0.292307692307692,-0.276923076923077,-0.261538461538462,-0.246153846153846,
-0.230769230769231,-0.215384615384615,-0.2,-0.184615384615385,-0.169230769230769,
-0.153846153846154,-0.138461538461538,-0.123076923076923,-0.107692307692308,
-0.0923076923076923,-0.0769230769230769,-0.0615384615384615,-0.0461538461538462,
-0.0307692307692308,-0.0153846153846154,0.),(-1.,1.),.UNSPECIFIED.)
GEOMETRIC_REPRESENTATION_ITEM()
RATIONAL_B_SPLINE_SURFACE(((1.,1.),(1.,1.),(1.,1.),(1.,1.),(1.,1.),(1.,
1.),(1.,1.),(1.,1.),(1.,1.),(1.,1.),(1.,1.),(1.,1.),(1.,1.),(1.,1.),(1.,
1.),(1.,1.),(1.,1.),(1.,1.),(1.,1.),(1.,1.),(1.,1.),(1.,1.),(1.,1.),(1.,
1.),(1.,1.),(1.,1.),(1.,1.),(1.,1.),(1.,1.),(1.,1.),(1.,1.),(1.,1.),(1.,
1.),(1.,1.),(1.,1.),(1.,1.),(1.,1.),(1.,1.),(1.,1.),(1.,1.),(1.,1.),(1.,
1.),(1.,1.),(1.,1.),(1.,1.),(1.,1.),(1.,1.),(1.,1.),(1.,1.),(1.,1.),(1.,
1.),(1.,1.),(1.,1.),(1.,1.),(1.,1.),(1.,1.),(1.,1.),(1.,1.),(1.,1.),(1.,
1.),(1.,1.),(1.,1.),(1.,1.),(1.,1.),(1.,1.),(1.,1.),(1.,1.),(1.,1.),(1.,
1.),(1.,1.)))
REPRESENTATION_ITEM('')
SURFACE()
);
#77=(
BOUNDED_SURFACE()
B_SPLINE_SURFACE(5,1,((#50380,#50381),(#50382,#50383),(#50384,#50385),(#50386,
#50387),(#50388,#50389),(#50390,#50391),(#50392,#50393),(#50394,#50395),
(#50396,#50397),(#50398,#50399),(#50400,#50401),(#50402,#50403),(#50404,
#50405),(#50406,#50407),(#50408,#50409),(#50410,#50411),(#50412,#50413),
(#50414,#50415),(#50416,#50417),(#50418,#50419),(#50420,#50421),(#50422,
#50423),(#50424,#50425),(#50426,#50427),(#50428,#50429),(#50430,#50431),
(#50432,#50433),(#50434,#50435),(#50436,#50437),(#50438,#50439),(#50440,
#50441),(#50442,#50443),(#50444,#50445),(#50446,#50447),(#50448,#50449),
(#50450,#50451),(#50452,#50453),(#50454,#50455),(#50456,#50457),(#50458,
#50459),(#50460,#50461),(#50462,#50463),(#50464,#50465),(#50466,#50467),
(#50468,#50469),(#50470,#50471),(#50472,#50473),(#50474,#50475),(#50476,
#50477),(#50478,#50479),(#50480,#50481),(#50482,#50483),(#50484,#50485),
(#50486,#50487),(#50488,#50489),(#50490,#50491),(#50492,#50493),(#50494,
#50495),(#50496,#50497),(#50498,#50499),(#50500,#50501),(#50502,#50503),
(#50504,#50505),(#50506,#50507),(#50508,#50509),(#50510,#50511),(#50512,
#50513),(#50514,#50515),(#50516,#50517),(#50518,#50519)),.UNSPECIFIED.,
 .F.,.F.,.F.)
B_SPLINE_SURFACE_WITH_KNOTS((6,1,1,1,1,1,1,1,1,1,1,1,1,1,1,1,1,1,1,1,1,
1,1,1,1,1,1,1,1,1,1,1,1,1,1,1,1,1,1,1,1,1,1,1,1,1,1,1,1,1,1,1,1,1,1,1,1,
1,1,1,1,1,1,1,1,6),(2,2),(-1.,-0.984615384615383,-0.969230769230768,-0.953846153846152,
-0.938461538461537,-0.923076923076922,-0.907692307692306,-0.892307692307691,
-0.876923076923076,-0.86153846153846,-0.846153846153845,-0.83076923076923,
-0.815384615384614,-0.799999999999999,-0.784615384615384,-0.769230769230768,
-0.753846153846153,-0.738461538461538,-0.723076923076922,-0.707692307692307,
-0.692307692307692,-0.676923076923076,-0.661538461538461,-0.646153846153846,
-0.63076923076923,-0.615384615384615,-0.6,-0.584615384615384,-0.569230769230769,
-0.553846153846154,-0.538461538461538,-0.523076923076923,-0.507692307692308,
-0.492307692307692,-0.476923076923077,-0.461538461538462,-0.446153846153846,
-0.430769230769231,-0.415384615384615,-0.4,-0.384615384615385,-0.369230769230769,
-0.353846153846154,-0.338461538461538,-0.323076923076923,-0.307692307692308,
-0.292307692307692,-0.276923076923077,-0.261538461538462,-0.246153846153846,
-0.230769230769231,-0.215384615384615,-0.2,-0.184615384615385,-0.169230769230769,
-0.153846153846154,-0.138461538461538,-0.123076923076923,-0.107692307692308,
-0.0923076923076923,-0.0769230769230769,-0.0615384615384615,-0.0461538461538462,
-0.0307692307692308,-0.0153846153846154,0.),(-1.,1.),.UNSPECIFIED.)
GEOMETRIC_REPRESENTATION_ITEM()
RATIONAL_B_SPLINE_SURFACE(((1.,1.),(1.,1.),(1.,1.),(1.,1.),(1.,1.),(1.,
1.),(1.,1.),(1.,1.),(1.,1.),(1.,1.),(1.,1.),(1.,1.),(1.,1.),(1.,1.),(1.,
1.),(1.,1.),(1.,1.),(1.,1.),(1.,1.),(1.,1.),(1.,1.),(1.,1.),(1.,1.),(1.,
1.),(1.,1.),(1.,1.),(1.,1.),(1.,1.),(1.,1.),(1.,1.),(1.,1.),(1.,1.),(1.,
1.),(1.,1.),(1.,1.),(1.,1.),(1.,1.),(1.,1.),(1.,1.),(1.,1.),(1.,1.),(1.,
1.),(1.,1.),(1.,1.),(1.,1.),(1.,1.),(1.,1.),(1.,1.),(1.,1.),(1.,1.),(1.,
1.),(1.,1.),(1.,1.),(1.,1.),(1.,1.),(1.,1.),(1.,1.),(1.,1.),(1.,1.),(1.,
1.),(1.,1.),(1.,1.),(1.,1.),(1.,1.),(1.,1.),(1.,1.),(1.,1.),(1.,1.),(1.,
1.),(1.,1.)))
REPRESENTATION_ITEM('')
SURFACE()
);
#78=(
BOUNDED_SURFACE()
B_SPLINE_SURFACE(5,1,((#50592,#50593),(#50594,#50595),(#50596,#50597),(#50598,
#50599),(#50600,#50601),(#50602,#50603),(#50604,#50605),(#50606,#50607),
(#50608,#50609),(#50610,#50611),(#50612,#50613),(#50614,#50615),(#50616,
#50617),(#50618,#50619),(#50620,#50621),(#50622,#50623),(#50624,#50625),
(#50626,#50627),(#50628,#50629),(#50630,#50631),(#50632,#50633),(#50634,
#50635),(#50636,#50637),(#50638,#50639),(#50640,#50641),(#50642,#50643),
(#50644,#50645),(#50646,#50647),(#50648,#50649),(#50650,#50651),(#50652,
#50653),(#50654,#50655),(#50656,#50657),(#50658,#50659),(#50660,#50661),
(#50662,#50663),(#50664,#50665),(#50666,#50667),(#50668,#50669),(#50670,
#50671),(#50672,#50673),(#50674,#50675),(#50676,#50677),(#50678,#50679),
(#50680,#50681),(#50682,#50683),(#50684,#50685),(#50686,#50687),(#50688,
#50689),(#50690,#50691),(#50692,#50693),(#50694,#50695),(#50696,#50697),
(#50698,#50699),(#50700,#50701),(#50702,#50703),(#50704,#50705),(#50706,
#50707),(#50708,#50709),(#50710,#50711),(#50712,#50713),(#50714,#50715),
(#50716,#50717),(#50718,#50719),(#50720,#50721),(#50722,#50723),(#50724,
#50725),(#50726,#50727),(#50728,#50729),(#50730,#50731)),.UNSPECIFIED.,
 .F.,.F.,.F.)
B_SPLINE_SURFACE_WITH_KNOTS((6,1,1,1,1,1,1,1,1,1,1,1,1,1,1,1,1,1,1,1,1,
1,1,1,1,1,1,1,1,1,1,1,1,1,1,1,1,1,1,1,1,1,1,1,1,1,1,1,1,1,1,1,1,1,1,1,1,
1,1,1,1,1,1,1,1,6),(2,2),(-1.,-0.984615384615383,-0.969230769230768,-0.953846153846152,
-0.938461538461537,-0.923076923076922,-0.907692307692306,-0.892307692307691,
-0.876923076923076,-0.86153846153846,-0.846153846153845,-0.83076923076923,
-0.815384615384614,-0.799999999999999,-0.784615384615384,-0.769230769230768,
-0.753846153846153,-0.738461538461538,-0.723076923076922,-0.707692307692307,
-0.692307692307692,-0.676923076923076,-0.661538461538461,-0.646153846153846,
-0.63076923076923,-0.615384615384615,-0.6,-0.584615384615384,-0.569230769230769,
-0.553846153846154,-0.538461538461538,-0.523076923076923,-0.507692307692308,
-0.492307692307692,-0.476923076923077,-0.461538461538462,-0.446153846153846,
-0.430769230769231,-0.415384615384615,-0.4,-0.384615384615385,-0.369230769230769,
-0.353846153846154,-0.338461538461538,-0.323076923076923,-0.307692307692308,
-0.292307692307692,-0.276923076923077,-0.261538461538462,-0.246153846153846,
-0.230769230769231,-0.215384615384615,-0.2,-0.184615384615385,-0.169230769230769,
-0.153846153846154,-0.138461538461538,-0.123076923076923,-0.107692307692308,
-0.0923076923076923,-0.0769230769230769,-0.0615384615384615,-0.0461538461538462,
-0.0307692307692308,-0.0153846153846154,0.),(-1.,1.),.UNSPECIFIED.)
GEOMETRIC_REPRESENTATION_ITEM()
RATIONAL_B_SPLINE_SURFACE(((1.,1.),(1.,1.),(1.,1.),(1.,1.),(1.,1.),(1.,
1.),(1.,1.),(1.,1.),(1.,1.),(1.,1.),(1.,1.),(1.,1.),(1.,1.),(1.,1.),(1.,
1.),(1.,1.),(1.,1.),(1.,1.),(1.,1.),(1.,1.),(1.,1.),(1.,1.),(1.,1.),(1.,
1.),(1.,1.),(1.,1.),(1.,1.),(1.,1.),(1.,1.),(1.,1.),(1.,1.),(1.,1.),(1.,
1.),(1.,1.),(1.,1.),(1.,1.),(1.,1.),(1.,1.),(1.,1.),(1.,1.),(1.,1.),(1.,
1.),(1.,1.),(1.,1.),(1.,1.),(1.,1.),(1.,1.),(1.,1.),(1.,1.),(1.,1.),(1.,
1.),(1.,1.),(1.,1.),(1.,1.),(1.,1.),(1.,1.),(1.,1.),(1.,1.),(1.,1.),(1.,
1.),(1.,1.),(1.,1.),(1.,1.),(1.,1.),(1.,1.),(1.,1.),(1.,1.),(1.,1.),(1.,
1.),(1.,1.)))
REPRESENTATION_ITEM('')
SURFACE()
);
#79=(
BOUNDED_SURFACE()
B_SPLINE_SURFACE(5,1,((#50822,#50823),(#50824,#50825),(#50826,#50827),(#50828,
#50829),(#50830,#50831),(#50832,#50833),(#50834,#50835),(#50836,#50837),
(#50838,#50839),(#50840,#50841),(#50842,#50843),(#50844,#50845),(#50846,
#50847),(#50848,#50849),(#50850,#50851),(#50852,#50853),(#50854,#50855),
(#50856,#50857),(#50858,#50859),(#50860,#50861),(#50862,#50863),(#50864,
#50865),(#50866,#50867),(#50868,#50869),(#50870,#50871),(#50872,#50873),
(#50874,#50875),(#50876,#50877),(#50878,#50879),(#50880,#50881),(#50882,
#50883),(#50884,#50885),(#50886,#50887),(#50888,#50889),(#50890,#50891),
(#50892,#50893),(#50894,#50895),(#50896,#50897),(#50898,#50899),(#50900,
#50901),(#50902,#50903),(#50904,#50905),(#50906,#50907),(#50908,#50909),
(#50910,#50911),(#50912,#50913),(#50914,#50915),(#50916,#50917),(#50918,
#50919),(#50920,#50921),(#50922,#50923),(#50924,#50925),(#50926,#50927),
(#50928,#50929),(#50930,#50931),(#50932,#50933),(#50934,#50935),(#50936,
#50937),(#50938,#50939),(#50940,#50941),(#50942,#50943),(#50944,#50945),
(#50946,#50947),(#50948,#50949),(#50950,#50951),(#50952,#50953),(#50954,
#50955),(#50956,#50957),(#50958,#50959),(#50960,#50961)),.UNSPECIFIED.,
 .F.,.F.,.F.)
B_SPLINE_SURFACE_WITH_KNOTS((6,1,1,1,1,1,1,1,1,1,1,1,1,1,1,1,1,1,1,1,1,
1,1,1,1,1,1,1,1,1,1,1,1,1,1,1,1,1,1,1,1,1,1,1,1,1,1,1,1,1,1,1,1,1,1,1,1,
1,1,1,1,1,1,1,1,6),(2,2),(-1.,-0.984615384615383,-0.969230769230768,-0.953846153846152,
-0.938461538461537,-0.923076923076922,-0.907692307692306,-0.892307692307691,
-0.876923076923076,-0.86153846153846,-0.846153846153845,-0.83076923076923,
-0.815384615384614,-0.799999999999999,-0.784615384615384,-0.769230769230768,
-0.753846153846153,-0.738461538461538,-0.723076923076922,-0.707692307692307,
-0.692307692307692,-0.676923076923076,-0.661538461538461,-0.646153846153846,
-0.63076923076923,-0.615384615384615,-0.6,-0.584615384615384,-0.569230769230769,
-0.553846153846154,-0.538461538461538,-0.523076923076923,-0.507692307692308,
-0.492307692307692,-0.476923076923077,-0.461538461538462,-0.446153846153846,
-0.430769230769231,-0.415384615384615,-0.4,-0.384615384615385,-0.369230769230769,
-0.353846153846154,-0.338461538461538,-0.323076923076923,-0.307692307692308,
-0.292307692307692,-0.276923076923077,-0.261538461538462,-0.246153846153846,
-0.230769230769231,-0.215384615384615,-0.2,-0.184615384615385,-0.169230769230769,
-0.153846153846154,-0.138461538461538,-0.123076923076923,-0.107692307692308,
-0.0923076923076923,-0.0769230769230769,-0.0615384615384615,-0.0461538461538462,
-0.0307692307692308,-0.0153846153846154,0.),(-1.,1.),.UNSPECIFIED.)
GEOMETRIC_REPRESENTATION_ITEM()
RATIONAL_B_SPLINE_SURFACE(((1.,1.),(1.,1.),(1.,1.),(1.,1.),(1.,1.),(1.,
1.),(1.,1.),(1.,1.),(1.,1.),(1.,1.),(1.,1.),(1.,1.),(1.,1.),(1.,1.),(1.,
1.),(1.,1.),(1.,1.),(1.,1.),(1.,1.),(1.,1.),(1.,1.),(1.,1.),(1.,1.),(1.,
1.),(1.,1.),(1.,1.),(1.,1.),(1.,1.),(1.,1.),(1.,1.),(1.,1.),(1.,1.),(1.,
1.),(1.,1.),(1.,1.),(1.,1.),(1.,1.),(1.,1.),(1.,1.),(1.,1.),(1.,1.),(1.,
1.),(1.,1.),(1.,1.),(1.,1.),(1.,1.),(1.,1.),(1.,1.),(1.,1.),(1.,1.),(1.,
1.),(1.,1.),(1.,1.),(1.,1.),(1.,1.),(1.,1.),(1.,1.),(1.,1.),(1.,1.),(1.,
1.),(1.,1.),(1.,1.),(1.,1.),(1.,1.),(1.,1.),(1.,1.),(1.,1.),(1.,1.),(1.,
1.),(1.,1.)))
REPRESENTATION_ITEM('')
SURFACE()
);
#80=(
BOUNDED_SURFACE()
B_SPLINE_SURFACE(5,1,((#51034,#51035),(#51036,#51037),(#51038,#51039),(#51040,
#51041),(#51042,#51043),(#51044,#51045),(#51046,#51047),(#51048,#51049),
(#51050,#51051),(#51052,#51053),(#51054,#51055),(#51056,#51057),(#51058,
#51059),(#51060,#51061),(#51062,#51063),(#51064,#51065),(#51066,#51067),
(#51068,#51069),(#51070,#51071),(#51072,#51073),(#51074,#51075),(#51076,
#51077),(#51078,#51079),(#51080,#51081),(#51082,#51083),(#51084,#51085),
(#51086,#51087),(#51088,#51089),(#51090,#51091),(#51092,#51093),(#51094,
#51095),(#51096,#51097),(#51098,#51099),(#51100,#51101),(#51102,#51103),
(#51104,#51105),(#51106,#51107),(#51108,#51109),(#51110,#51111),(#51112,
#51113),(#51114,#51115),(#51116,#51117),(#51118,#51119),(#51120,#51121),
(#51122,#51123),(#51124,#51125),(#51126,#51127),(#51128,#51129),(#51130,
#51131),(#51132,#51133),(#51134,#51135),(#51136,#51137),(#51138,#51139),
(#51140,#51141),(#51142,#51143),(#51144,#51145),(#51146,#51147),(#51148,
#51149),(#51150,#51151),(#51152,#51153),(#51154,#51155),(#51156,#51157),
(#51158,#51159),(#51160,#51161),(#51162,#51163),(#51164,#51165),(#51166,
#51167),(#51168,#51169),(#51170,#51171),(#51172,#51173)),.UNSPECIFIED.,
 .F.,.F.,.F.)
B_SPLINE_SURFACE_WITH_KNOTS((6,1,1,1,1,1,1,1,1,1,1,1,1,1,1,1,1,1,1,1,1,
1,1,1,1,1,1,1,1,1,1,1,1,1,1,1,1,1,1,1,1,1,1,1,1,1,1,1,1,1,1,1,1,1,1,1,1,
1,1,1,1,1,1,1,1,6),(2,2),(-1.,-0.984615384615383,-0.969230769230768,-0.953846153846152,
-0.938461538461537,-0.923076923076922,-0.907692307692306,-0.892307692307691,
-0.876923076923076,-0.86153846153846,-0.846153846153845,-0.83076923076923,
-0.815384615384614,-0.799999999999999,-0.784615384615384,-0.769230769230768,
-0.753846153846153,-0.738461538461538,-0.723076923076922,-0.707692307692307,
-0.692307692307692,-0.676923076923076,-0.661538461538461,-0.646153846153846,
-0.63076923076923,-0.615384615384615,-0.6,-0.584615384615384,-0.569230769230769,
-0.553846153846154,-0.538461538461538,-0.523076923076923,-0.507692307692308,
-0.492307692307692,-0.476923076923077,-0.461538461538462,-0.446153846153846,
-0.430769230769231,-0.415384615384615,-0.4,-0.384615384615385,-0.369230769230769,
-0.353846153846154,-0.338461538461538,-0.323076923076923,-0.307692307692308,
-0.292307692307692,-0.276923076923077,-0.261538461538462,-0.246153846153846,
-0.230769230769231,-0.215384615384615,-0.2,-0.184615384615385,-0.169230769230769,
-0.153846153846154,-0.138461538461538,-0.123076923076923,-0.107692307692308,
-0.0923076923076923,-0.0769230769230769,-0.0615384615384615,-0.0461538461538462,
-0.0307692307692308,-0.0153846153846154,0.),(-1.,1.),.UNSPECIFIED.)
GEOMETRIC_REPRESENTATION_ITEM()
RATIONAL_B_SPLINE_SURFACE(((1.,1.),(1.,1.),(1.,1.),(1.,1.),(1.,1.),(1.,
1.),(1.,1.),(1.,1.),(1.,1.),(1.,1.),(1.,1.),(1.,1.),(1.,1.),(1.,1.),(1.,
1.),(1.,1.),(1.,1.),(1.,1.),(1.,1.),(1.,1.),(1.,1.),(1.,1.),(1.,1.),(1.,
1.),(1.,1.),(1.,1.),(1.,1.),(1.,1.),(1.,1.),(1.,1.),(1.,1.),(1.,1.),(1.,
1.),(1.,1.),(1.,1.),(1.,1.),(1.,1.),(1.,1.),(1.,1.),(1.,1.),(1.,1.),(1.,
1.),(1.,1.),(1.,1.),(1.,1.),(1.,1.),(1.,1.),(1.,1.),(1.,1.),(1.,1.),(1.,
1.),(1.,1.),(1.,1.),(1.,1.),(1.,1.),(1.,1.),(1.,1.),(1.,1.),(1.,1.),(1.,
1.),(1.,1.),(1.,1.),(1.,1.),(1.,1.),(1.,1.),(1.,1.),(1.,1.),(1.,1.),(1.,
1.),(1.,1.)))
REPRESENTATION_ITEM('')
SURFACE()
);
#81=(
BOUNDED_SURFACE()
B_SPLINE_SURFACE(5,1,((#51264,#51265),(#51266,#51267),(#51268,#51269),(#51270,
#51271),(#51272,#51273),(#51274,#51275),(#51276,#51277),(#51278,#51279),
(#51280,#51281),(#51282,#51283),(#51284,#51285),(#51286,#51287),(#51288,
#51289),(#51290,#51291),(#51292,#51293),(#51294,#51295),(#51296,#51297),
(#51298,#51299),(#51300,#51301),(#51302,#51303),(#51304,#51305),(#51306,
#51307),(#51308,#51309),(#51310,#51311),(#51312,#51313),(#51314,#51315),
(#51316,#51317),(#51318,#51319),(#51320,#51321),(#51322,#51323),(#51324,
#51325),(#51326,#51327),(#51328,#51329),(#51330,#51331),(#51332,#51333),
(#51334,#51335),(#51336,#51337),(#51338,#51339),(#51340,#51341),(#51342,
#51343),(#51344,#51345),(#51346,#51347),(#51348,#51349),(#51350,#51351),
(#51352,#51353),(#51354,#51355),(#51356,#51357),(#51358,#51359),(#51360,
#51361),(#51362,#51363),(#51364,#51365),(#51366,#51367),(#51368,#51369),
(#51370,#51371),(#51372,#51373),(#51374,#51375),(#51376,#51377),(#51378,
#51379),(#51380,#51381),(#51382,#51383),(#51384,#51385),(#51386,#51387),
(#51388,#51389),(#51390,#51391),(#51392,#51393),(#51394,#51395),(#51396,
#51397),(#51398,#51399),(#51400,#51401),(#51402,#51403)),.UNSPECIFIED.,
 .F.,.F.,.F.)
B_SPLINE_SURFACE_WITH_KNOTS((6,1,1,1,1,1,1,1,1,1,1,1,1,1,1,1,1,1,1,1,1,
1,1,1,1,1,1,1,1,1,1,1,1,1,1,1,1,1,1,1,1,1,1,1,1,1,1,1,1,1,1,1,1,1,1,1,1,
1,1,1,1,1,1,1,1,6),(2,2),(-1.,-0.984615384615383,-0.969230769230768,-0.953846153846152,
-0.938461538461537,-0.923076923076922,-0.907692307692306,-0.892307692307691,
-0.876923076923076,-0.86153846153846,-0.846153846153845,-0.83076923076923,
-0.815384615384614,-0.799999999999999,-0.784615384615384,-0.769230769230768,
-0.753846153846153,-0.738461538461538,-0.723076923076922,-0.707692307692307,
-0.692307692307692,-0.676923076923076,-0.661538461538461,-0.646153846153846,
-0.63076923076923,-0.615384615384615,-0.6,-0.584615384615384,-0.569230769230769,
-0.553846153846154,-0.538461538461538,-0.523076923076923,-0.507692307692308,
-0.492307692307692,-0.476923076923077,-0.461538461538462,-0.446153846153846,
-0.430769230769231,-0.415384615384615,-0.4,-0.384615384615385,-0.369230769230769,
-0.353846153846154,-0.338461538461538,-0.323076923076923,-0.307692307692308,
-0.292307692307692,-0.276923076923077,-0.261538461538462,-0.246153846153846,
-0.230769230769231,-0.215384615384615,-0.2,-0.184615384615385,-0.169230769230769,
-0.153846153846154,-0.138461538461538,-0.123076923076923,-0.107692307692308,
-0.0923076923076923,-0.0769230769230769,-0.0615384615384615,-0.0461538461538462,
-0.0307692307692308,-0.0153846153846154,0.),(-1.,1.),.UNSPECIFIED.)
GEOMETRIC_REPRESENTATION_ITEM()
RATIONAL_B_SPLINE_SURFACE(((1.,1.),(1.,1.),(1.,1.),(1.,1.),(1.,1.),(1.,
1.),(1.,1.),(1.,1.),(1.,1.),(1.,1.),(1.,1.),(1.,1.),(1.,1.),(1.,1.),(1.,
1.),(1.,1.),(1.,1.),(1.,1.),(1.,1.),(1.,1.),(1.,1.),(1.,1.),(1.,1.),(1.,
1.),(1.,1.),(1.,1.),(1.,1.),(1.,1.),(1.,1.),(1.,1.),(1.,1.),(1.,1.),(1.,
1.),(1.,1.),(1.,1.),(1.,1.),(1.,1.),(1.,1.),(1.,1.),(1.,1.),(1.,1.),(1.,
1.),(1.,1.),(1.,1.),(1.,1.),(1.,1.),(1.,1.),(1.,1.),(1.,1.),(1.,1.),(1.,
1.),(1.,1.),(1.,1.),(1.,1.),(1.,1.),(1.,1.),(1.,1.),(1.,1.),(1.,1.),(1.,
1.),(1.,1.),(1.,1.),(1.,1.),(1.,1.),(1.,1.),(1.,1.),(1.,1.),(1.,1.),(1.,
1.),(1.,1.)))
REPRESENTATION_ITEM('')
SURFACE()
);
#82=(
BOUNDED_SURFACE()
B_SPLINE_SURFACE(5,1,((#51476,#51477),(#51478,#51479),(#51480,#51481),(#51482,
#51483),(#51484,#51485),(#51486,#51487),(#51488,#51489),(#51490,#51491),
(#51492,#51493),(#51494,#51495),(#51496,#51497),(#51498,#51499),(#51500,
#51501),(#51502,#51503),(#51504,#51505),(#51506,#51507),(#51508,#51509),
(#51510,#51511),(#51512,#51513),(#51514,#51515),(#51516,#51517),(#51518,
#51519),(#51520,#51521),(#51522,#51523),(#51524,#51525),(#51526,#51527),
(#51528,#51529),(#51530,#51531),(#51532,#51533),(#51534,#51535),(#51536,
#51537),(#51538,#51539),(#51540,#51541),(#51542,#51543),(#51544,#51545),
(#51546,#51547),(#51548,#51549),(#51550,#51551),(#51552,#51553),(#51554,
#51555),(#51556,#51557),(#51558,#51559),(#51560,#51561),(#51562,#51563),
(#51564,#51565),(#51566,#51567),(#51568,#51569),(#51570,#51571),(#51572,
#51573),(#51574,#51575),(#51576,#51577),(#51578,#51579),(#51580,#51581),
(#51582,#51583),(#51584,#51585),(#51586,#51587),(#51588,#51589),(#51590,
#51591),(#51592,#51593),(#51594,#51595),(#51596,#51597),(#51598,#51599),
(#51600,#51601),(#51602,#51603),(#51604,#51605),(#51606,#51607),(#51608,
#51609),(#51610,#51611),(#51612,#51613),(#51614,#51615)),.UNSPECIFIED.,
 .F.,.F.,.F.)
B_SPLINE_SURFACE_WITH_KNOTS((6,1,1,1,1,1,1,1,1,1,1,1,1,1,1,1,1,1,1,1,1,
1,1,1,1,1,1,1,1,1,1,1,1,1,1,1,1,1,1,1,1,1,1,1,1,1,1,1,1,1,1,1,1,1,1,1,1,
1,1,1,1,1,1,1,1,6),(2,2),(-1.,-0.984615384615383,-0.969230769230768,-0.953846153846152,
-0.938461538461537,-0.923076923076922,-0.907692307692306,-0.892307692307691,
-0.876923076923076,-0.86153846153846,-0.846153846153845,-0.83076923076923,
-0.815384615384614,-0.799999999999999,-0.784615384615384,-0.769230769230768,
-0.753846153846153,-0.738461538461538,-0.723076923076922,-0.707692307692307,
-0.692307692307692,-0.676923076923076,-0.661538461538461,-0.646153846153846,
-0.63076923076923,-0.615384615384615,-0.6,-0.584615384615384,-0.569230769230769,
-0.553846153846154,-0.538461538461538,-0.523076923076923,-0.507692307692308,
-0.492307692307692,-0.476923076923077,-0.461538461538462,-0.446153846153846,
-0.430769230769231,-0.415384615384615,-0.4,-0.384615384615385,-0.369230769230769,
-0.353846153846154,-0.338461538461538,-0.323076923076923,-0.307692307692308,
-0.292307692307692,-0.276923076923077,-0.261538461538462,-0.246153846153846,
-0.230769230769231,-0.215384615384615,-0.2,-0.184615384615385,-0.169230769230769,
-0.153846153846154,-0.138461538461538,-0.123076923076923,-0.107692307692308,
-0.0923076923076923,-0.0769230769230769,-0.0615384615384615,-0.0461538461538462,
-0.0307692307692308,-0.0153846153846154,0.),(-1.,1.),.UNSPECIFIED.)
GEOMETRIC_REPRESENTATION_ITEM()
RATIONAL_B_SPLINE_SURFACE(((1.,1.),(1.,1.),(1.,1.),(1.,1.),(1.,1.),(1.,
1.),(1.,1.),(1.,1.),(1.,1.),(1.,1.),(1.,1.),(1.,1.),(1.,1.),(1.,1.),(1.,
1.),(1.,1.),(1.,1.),(1.,1.),(1.,1.),(1.,1.),(1.,1.),(1.,1.),(1.,1.),(1.,
1.),(1.,1.),(1.,1.),(1.,1.),(1.,1.),(1.,1.),(1.,1.),(1.,1.),(1.,1.),(1.,
1.),(1.,1.),(1.,1.),(1.,1.),(1.,1.),(1.,1.),(1.,1.),(1.,1.),(1.,1.),(1.,
1.),(1.,1.),(1.,1.),(1.,1.),(1.,1.),(1.,1.),(1.,1.),(1.,1.),(1.,1.),(1.,
1.),(1.,1.),(1.,1.),(1.,1.),(1.,1.),(1.,1.),(1.,1.),(1.,1.),(1.,1.),(1.,
1.),(1.,1.),(1.,1.),(1.,1.),(1.,1.),(1.,1.),(1.,1.),(1.,1.),(1.,1.),(1.,
1.),(1.,1.)))
REPRESENTATION_ITEM('')
SURFACE()
);
#83=(
BOUNDED_SURFACE()
B_SPLINE_SURFACE(5,1,((#51706,#51707),(#51708,#51709),(#51710,#51711),(#51712,
#51713),(#51714,#51715),(#51716,#51717),(#51718,#51719),(#51720,#51721),
(#51722,#51723),(#51724,#51725),(#51726,#51727),(#51728,#51729),(#51730,
#51731),(#51732,#51733),(#51734,#51735),(#51736,#51737),(#51738,#51739),
(#51740,#51741),(#51742,#51743),(#51744,#51745),(#51746,#51747),(#51748,
#51749),(#51750,#51751),(#51752,#51753),(#51754,#51755),(#51756,#51757),
(#51758,#51759),(#51760,#51761),(#51762,#51763),(#51764,#51765),(#51766,
#51767),(#51768,#51769),(#51770,#51771),(#51772,#51773),(#51774,#51775),
(#51776,#51777),(#51778,#51779),(#51780,#51781),(#51782,#51783),(#51784,
#51785),(#51786,#51787),(#51788,#51789),(#51790,#51791),(#51792,#51793),
(#51794,#51795),(#51796,#51797),(#51798,#51799),(#51800,#51801),(#51802,
#51803),(#51804,#51805),(#51806,#51807),(#51808,#51809),(#51810,#51811),
(#51812,#51813),(#51814,#51815),(#51816,#51817),(#51818,#51819),(#51820,
#51821),(#51822,#51823),(#51824,#51825),(#51826,#51827),(#51828,#51829),
(#51830,#51831),(#51832,#51833),(#51834,#51835),(#51836,#51837),(#51838,
#51839),(#51840,#51841),(#51842,#51843),(#51844,#51845)),.UNSPECIFIED.,
 .F.,.F.,.F.)
B_SPLINE_SURFACE_WITH_KNOTS((6,1,1,1,1,1,1,1,1,1,1,1,1,1,1,1,1,1,1,1,1,
1,1,1,1,1,1,1,1,1,1,1,1,1,1,1,1,1,1,1,1,1,1,1,1,1,1,1,1,1,1,1,1,1,1,1,1,
1,1,1,1,1,1,1,1,6),(2,2),(-1.,-0.984615384615383,-0.969230769230768,-0.953846153846152,
-0.938461538461537,-0.923076923076922,-0.907692307692306,-0.892307692307691,
-0.876923076923076,-0.86153846153846,-0.846153846153845,-0.83076923076923,
-0.815384615384614,-0.799999999999999,-0.784615384615384,-0.769230769230768,
-0.753846153846153,-0.738461538461538,-0.723076923076922,-0.707692307692307,
-0.692307692307692,-0.676923076923076,-0.661538461538461,-0.646153846153846,
-0.63076923076923,-0.615384615384615,-0.6,-0.584615384615384,-0.569230769230769,
-0.553846153846154,-0.538461538461538,-0.523076923076923,-0.507692307692308,
-0.492307692307692,-0.476923076923077,-0.461538461538462,-0.446153846153846,
-0.430769230769231,-0.415384615384615,-0.4,-0.384615384615385,-0.369230769230769,
-0.353846153846154,-0.338461538461538,-0.323076923076923,-0.307692307692308,
-0.292307692307692,-0.276923076923077,-0.261538461538462,-0.246153846153846,
-0.230769230769231,-0.215384615384615,-0.2,-0.184615384615385,-0.169230769230769,
-0.153846153846154,-0.138461538461538,-0.123076923076923,-0.107692307692308,
-0.0923076923076923,-0.0769230769230769,-0.0615384615384615,-0.0461538461538462,
-0.0307692307692308,-0.0153846153846154,0.),(-1.,1.),.UNSPECIFIED.)
GEOMETRIC_REPRESENTATION_ITEM()
RATIONAL_B_SPLINE_SURFACE(((1.,1.),(1.,1.),(1.,1.),(1.,1.),(1.,1.),(1.,
1.),(1.,1.),(1.,1.),(1.,1.),(1.,1.),(1.,1.),(1.,1.),(1.,1.),(1.,1.),(1.,
1.),(1.,1.),(1.,1.),(1.,1.),(1.,1.),(1.,1.),(1.,1.),(1.,1.),(1.,1.),(1.,
1.),(1.,1.),(1.,1.),(1.,1.),(1.,1.),(1.,1.),(1.,1.),(1.,1.),(1.,1.),(1.,
1.),(1.,1.),(1.,1.),(1.,1.),(1.,1.),(1.,1.),(1.,1.),(1.,1.),(1.,1.),(1.,
1.),(1.,1.),(1.,1.),(1.,1.),(1.,1.),(1.,1.),(1.,1.),(1.,1.),(1.,1.),(1.,
1.),(1.,1.),(1.,1.),(1.,1.),(1.,1.),(1.,1.),(1.,1.),(1.,1.),(1.,1.),(1.,
1.),(1.,1.),(1.,1.),(1.,1.),(1.,1.),(1.,1.),(1.,1.),(1.,1.),(1.,1.),(1.,
1.),(1.,1.)))
REPRESENTATION_ITEM('')
SURFACE()
);
#84=(
BOUNDED_SURFACE()
B_SPLINE_SURFACE(5,1,((#51918,#51919),(#51920,#51921),(#51922,#51923),(#51924,
#51925),(#51926,#51927),(#51928,#51929),(#51930,#51931),(#51932,#51933),
(#51934,#51935),(#51936,#51937),(#51938,#51939),(#51940,#51941),(#51942,
#51943),(#51944,#51945),(#51946,#51947),(#51948,#51949),(#51950,#51951),
(#51952,#51953),(#51954,#51955),(#51956,#51957),(#51958,#51959),(#51960,
#51961),(#51962,#51963),(#51964,#51965),(#51966,#51967),(#51968,#51969),
(#51970,#51971),(#51972,#51973),(#51974,#51975),(#51976,#51977),(#51978,
#51979),(#51980,#51981),(#51982,#51983),(#51984,#51985),(#51986,#51987),
(#51988,#51989),(#51990,#51991),(#51992,#51993),(#51994,#51995),(#51996,
#51997),(#51998,#51999),(#52000,#52001),(#52002,#52003),(#52004,#52005),
(#52006,#52007),(#52008,#52009),(#52010,#52011),(#52012,#52013),(#52014,
#52015),(#52016,#52017),(#52018,#52019),(#52020,#52021),(#52022,#52023),
(#52024,#52025),(#52026,#52027),(#52028,#52029),(#52030,#52031),(#52032,
#52033),(#52034,#52035),(#52036,#52037),(#52038,#52039),(#52040,#52041),
(#52042,#52043),(#52044,#52045),(#52046,#52047),(#52048,#52049),(#52050,
#52051),(#52052,#52053),(#52054,#52055),(#52056,#52057)),.UNSPECIFIED.,
 .F.,.F.,.F.)
B_SPLINE_SURFACE_WITH_KNOTS((6,1,1,1,1,1,1,1,1,1,1,1,1,1,1,1,1,1,1,1,1,
1,1,1,1,1,1,1,1,1,1,1,1,1,1,1,1,1,1,1,1,1,1,1,1,1,1,1,1,1,1,1,1,1,1,1,1,
1,1,1,1,1,1,1,1,6),(2,2),(-1.,-0.984615384615383,-0.969230769230768,-0.953846153846152,
-0.938461538461537,-0.923076923076922,-0.907692307692306,-0.892307692307691,
-0.876923076923076,-0.86153846153846,-0.846153846153845,-0.83076923076923,
-0.815384615384614,-0.799999999999999,-0.784615384615384,-0.769230769230768,
-0.753846153846153,-0.738461538461538,-0.723076923076922,-0.707692307692307,
-0.692307692307692,-0.676923076923076,-0.661538461538461,-0.646153846153846,
-0.63076923076923,-0.615384615384615,-0.6,-0.584615384615384,-0.569230769230769,
-0.553846153846154,-0.538461538461538,-0.523076923076923,-0.507692307692308,
-0.492307692307692,-0.476923076923077,-0.461538461538462,-0.446153846153846,
-0.430769230769231,-0.415384615384615,-0.4,-0.384615384615385,-0.369230769230769,
-0.353846153846154,-0.338461538461538,-0.323076923076923,-0.307692307692308,
-0.292307692307692,-0.276923076923077,-0.261538461538462,-0.246153846153846,
-0.230769230769231,-0.215384615384615,-0.2,-0.184615384615385,-0.169230769230769,
-0.153846153846154,-0.138461538461538,-0.123076923076923,-0.107692307692308,
-0.0923076923076923,-0.0769230769230769,-0.0615384615384615,-0.0461538461538462,
-0.0307692307692308,-0.0153846153846154,0.),(-1.,1.),.UNSPECIFIED.)
GEOMETRIC_REPRESENTATION_ITEM()
RATIONAL_B_SPLINE_SURFACE(((1.,1.),(1.,1.),(1.,1.),(1.,1.),(1.,1.),(1.,
1.),(1.,1.),(1.,1.),(1.,1.),(1.,1.),(1.,1.),(1.,1.),(1.,1.),(1.,1.),(1.,
1.),(1.,1.),(1.,1.),(1.,1.),(1.,1.),(1.,1.),(1.,1.),(1.,1.),(1.,1.),(1.,
1.),(1.,1.),(1.,1.),(1.,1.),(1.,1.),(1.,1.),(1.,1.),(1.,1.),(1.,1.),(1.,
1.),(1.,1.),(1.,1.),(1.,1.),(1.,1.),(1.,1.),(1.,1.),(1.,1.),(1.,1.),(1.,
1.),(1.,1.),(1.,1.),(1.,1.),(1.,1.),(1.,1.),(1.,1.),(1.,1.),(1.,1.),(1.,
1.),(1.,1.),(1.,1.),(1.,1.),(1.,1.),(1.,1.),(1.,1.),(1.,1.),(1.,1.),(1.,
1.),(1.,1.),(1.,1.),(1.,1.),(1.,1.),(1.,1.),(1.,1.),(1.,1.),(1.,1.),(1.,
1.),(1.,1.)))
REPRESENTATION_ITEM('')
SURFACE()
);
#85=(
BOUNDED_SURFACE()
B_SPLINE_SURFACE(5,1,((#52148,#52149),(#52150,#52151),(#52152,#52153),(#52154,
#52155),(#52156,#52157),(#52158,#52159),(#52160,#52161),(#52162,#52163),
(#52164,#52165),(#52166,#52167),(#52168,#52169),(#52170,#52171),(#52172,
#52173),(#52174,#52175),(#52176,#52177),(#52178,#52179),(#52180,#52181),
(#52182,#52183),(#52184,#52185),(#52186,#52187),(#52188,#52189),(#52190,
#52191),(#52192,#52193),(#52194,#52195),(#52196,#52197),(#52198,#52199),
(#52200,#52201),(#52202,#52203),(#52204,#52205),(#52206,#52207),(#52208,
#52209),(#52210,#52211),(#52212,#52213),(#52214,#52215),(#52216,#52217),
(#52218,#52219),(#52220,#52221),(#52222,#52223),(#52224,#52225),(#52226,
#52227),(#52228,#52229),(#52230,#52231),(#52232,#52233),(#52234,#52235),
(#52236,#52237),(#52238,#52239),(#52240,#52241),(#52242,#52243),(#52244,
#52245),(#52246,#52247),(#52248,#52249),(#52250,#52251),(#52252,#52253),
(#52254,#52255),(#52256,#52257),(#52258,#52259),(#52260,#52261),(#52262,
#52263),(#52264,#52265),(#52266,#52267),(#52268,#52269),(#52270,#52271),
(#52272,#52273),(#52274,#52275),(#52276,#52277),(#52278,#52279),(#52280,
#52281),(#52282,#52283),(#52284,#52285),(#52286,#52287)),.UNSPECIFIED.,
 .F.,.F.,.F.)
B_SPLINE_SURFACE_WITH_KNOTS((6,1,1,1,1,1,1,1,1,1,1,1,1,1,1,1,1,1,1,1,1,
1,1,1,1,1,1,1,1,1,1,1,1,1,1,1,1,1,1,1,1,1,1,1,1,1,1,1,1,1,1,1,1,1,1,1,1,
1,1,1,1,1,1,1,1,6),(2,2),(-1.,-0.984615384615383,-0.969230769230768,-0.953846153846152,
-0.938461538461537,-0.923076923076922,-0.907692307692306,-0.892307692307691,
-0.876923076923076,-0.86153846153846,-0.846153846153845,-0.83076923076923,
-0.815384615384614,-0.799999999999999,-0.784615384615384,-0.769230769230768,
-0.753846153846153,-0.738461538461538,-0.723076923076922,-0.707692307692307,
-0.692307692307692,-0.676923076923076,-0.661538461538461,-0.646153846153846,
-0.63076923076923,-0.615384615384615,-0.6,-0.584615384615384,-0.569230769230769,
-0.553846153846154,-0.538461538461538,-0.523076923076923,-0.507692307692308,
-0.492307692307692,-0.476923076923077,-0.461538461538462,-0.446153846153846,
-0.430769230769231,-0.415384615384615,-0.4,-0.384615384615385,-0.369230769230769,
-0.353846153846154,-0.338461538461538,-0.323076923076923,-0.307692307692308,
-0.292307692307692,-0.276923076923077,-0.261538461538462,-0.246153846153846,
-0.230769230769231,-0.215384615384615,-0.2,-0.184615384615385,-0.169230769230769,
-0.153846153846154,-0.138461538461538,-0.123076923076923,-0.107692307692308,
-0.0923076923076923,-0.0769230769230769,-0.0615384615384615,-0.0461538461538462,
-0.0307692307692308,-0.0153846153846154,0.),(-1.,1.),.UNSPECIFIED.)
GEOMETRIC_REPRESENTATION_ITEM()
RATIONAL_B_SPLINE_SURFACE(((1.,1.),(1.,1.),(1.,1.),(1.,1.),(1.,1.),(1.,
1.),(1.,1.),(1.,1.),(1.,1.),(1.,1.),(1.,1.),(1.,1.),(1.,1.),(1.,1.),(1.,
1.),(1.,1.),(1.,1.),(1.,1.),(1.,1.),(1.,1.),(1.,1.),(1.,1.),(1.,1.),(1.,
1.),(1.,1.),(1.,1.),(1.,1.),(1.,1.),(1.,1.),(1.,1.),(1.,1.),(1.,1.),(1.,
1.),(1.,1.),(1.,1.),(1.,1.),(1.,1.),(1.,1.),(1.,1.),(1.,1.),(1.,1.),(1.,
1.),(1.,1.),(1.,1.),(1.,1.),(1.,1.),(1.,1.),(1.,1.),(1.,1.),(1.,1.),(1.,
1.),(1.,1.),(1.,1.),(1.,1.),(1.,1.),(1.,1.),(1.,1.),(1.,1.),(1.,1.),(1.,
1.),(1.,1.),(1.,1.),(1.,1.),(1.,1.),(1.,1.),(1.,1.),(1.,1.),(1.,1.),(1.,
1.),(1.,1.)))
REPRESENTATION_ITEM('')
SURFACE()
);
#86=(
BOUNDED_SURFACE()
B_SPLINE_SURFACE(5,1,((#52360,#52361),(#52362,#52363),(#52364,#52365),(#52366,
#52367),(#52368,#52369),(#52370,#52371),(#52372,#52373),(#52374,#52375),
(#52376,#52377),(#52378,#52379),(#52380,#52381),(#52382,#52383),(#52384,
#52385),(#52386,#52387),(#52388,#52389),(#52390,#52391),(#52392,#52393),
(#52394,#52395),(#52396,#52397),(#52398,#52399),(#52400,#52401),(#52402,
#52403),(#52404,#52405),(#52406,#52407),(#52408,#52409),(#52410,#52411),
(#52412,#52413),(#52414,#52415),(#52416,#52417),(#52418,#52419),(#52420,
#52421),(#52422,#52423),(#52424,#52425),(#52426,#52427),(#52428,#52429),
(#52430,#52431),(#52432,#52433),(#52434,#52435),(#52436,#52437),(#52438,
#52439),(#52440,#52441),(#52442,#52443),(#52444,#52445),(#52446,#52447),
(#52448,#52449),(#52450,#52451),(#52452,#52453),(#52454,#52455),(#52456,
#52457),(#52458,#52459),(#52460,#52461),(#52462,#52463),(#52464,#52465),
(#52466,#52467),(#52468,#52469),(#52470,#52471),(#52472,#52473),(#52474,
#52475),(#52476,#52477),(#52478,#52479),(#52480,#52481),(#52482,#52483),
(#52484,#52485),(#52486,#52487),(#52488,#52489),(#52490,#52491),(#52492,
#52493),(#52494,#52495),(#52496,#52497),(#52498,#52499)),.UNSPECIFIED.,
 .F.,.F.,.F.)
B_SPLINE_SURFACE_WITH_KNOTS((6,1,1,1,1,1,1,1,1,1,1,1,1,1,1,1,1,1,1,1,1,
1,1,1,1,1,1,1,1,1,1,1,1,1,1,1,1,1,1,1,1,1,1,1,1,1,1,1,1,1,1,1,1,1,1,1,1,
1,1,1,1,1,1,1,1,6),(2,2),(-1.,-0.984615384615383,-0.969230769230768,-0.953846153846152,
-0.938461538461537,-0.923076923076922,-0.907692307692306,-0.892307692307691,
-0.876923076923076,-0.86153846153846,-0.846153846153845,-0.83076923076923,
-0.815384615384614,-0.799999999999999,-0.784615384615384,-0.769230769230768,
-0.753846153846153,-0.738461538461538,-0.723076923076922,-0.707692307692307,
-0.692307692307692,-0.676923076923076,-0.661538461538461,-0.646153846153846,
-0.63076923076923,-0.615384615384615,-0.6,-0.584615384615384,-0.569230769230769,
-0.553846153846154,-0.538461538461538,-0.523076923076923,-0.507692307692308,
-0.492307692307692,-0.476923076923077,-0.461538461538462,-0.446153846153846,
-0.430769230769231,-0.415384615384615,-0.4,-0.384615384615385,-0.369230769230769,
-0.353846153846154,-0.338461538461538,-0.323076923076923,-0.307692307692308,
-0.292307692307692,-0.276923076923077,-0.261538461538462,-0.246153846153846,
-0.230769230769231,-0.215384615384615,-0.2,-0.184615384615385,-0.169230769230769,
-0.153846153846154,-0.138461538461538,-0.123076923076923,-0.107692307692308,
-0.0923076923076923,-0.0769230769230769,-0.0615384615384615,-0.0461538461538462,
-0.0307692307692308,-0.0153846153846154,0.),(-1.,1.),.UNSPECIFIED.)
GEOMETRIC_REPRESENTATION_ITEM()
RATIONAL_B_SPLINE_SURFACE(((1.,1.),(1.,1.),(1.,1.),(1.,1.),(1.,1.),(1.,
1.),(1.,1.),(1.,1.),(1.,1.),(1.,1.),(1.,1.),(1.,1.),(1.,1.),(1.,1.),(1.,
1.),(1.,1.),(1.,1.),(1.,1.),(1.,1.),(1.,1.),(1.,1.),(1.,1.),(1.,1.),(1.,
1.),(1.,1.),(1.,1.),(1.,1.),(1.,1.),(1.,1.),(1.,1.),(1.,1.),(1.,1.),(1.,
1.),(1.,1.),(1.,1.),(1.,1.),(1.,1.),(1.,1.),(1.,1.),(1.,1.),(1.,1.),(1.,
1.),(1.,1.),(1.,1.),(1.,1.),(1.,1.),(1.,1.),(1.,1.),(1.,1.),(1.,1.),(1.,
1.),(1.,1.),(1.,1.),(1.,1.),(1.,1.),(1.,1.),(1.,1.),(1.,1.),(1.,1.),(1.,
1.),(1.,1.),(1.,1.),(1.,1.),(1.,1.),(1.,1.),(1.,1.),(1.,1.),(1.,1.),(1.,
1.),(1.,1.)))
REPRESENTATION_ITEM('')
SURFACE()
);
#87=(
BOUNDED_SURFACE()
B_SPLINE_SURFACE(5,1,((#52590,#52591),(#52592,#52593),(#52594,#52595),(#52596,
#52597),(#52598,#52599),(#52600,#52601),(#52602,#52603),(#52604,#52605),
(#52606,#52607),(#52608,#52609),(#52610,#52611),(#52612,#52613),(#52614,
#52615),(#52616,#52617),(#52618,#52619),(#52620,#52621),(#52622,#52623),
(#52624,#52625),(#52626,#52627),(#52628,#52629),(#52630,#52631),(#52632,
#52633),(#52634,#52635),(#52636,#52637),(#52638,#52639),(#52640,#52641),
(#52642,#52643),(#52644,#52645),(#52646,#52647),(#52648,#52649),(#52650,
#52651),(#52652,#52653),(#52654,#52655),(#52656,#52657),(#52658,#52659),
(#52660,#52661),(#52662,#52663),(#52664,#52665),(#52666,#52667),(#52668,
#52669),(#52670,#52671),(#52672,#52673),(#52674,#52675),(#52676,#52677),
(#52678,#52679),(#52680,#52681),(#52682,#52683),(#52684,#52685),(#52686,
#52687),(#52688,#52689),(#52690,#52691),(#52692,#52693),(#52694,#52695),
(#52696,#52697),(#52698,#52699),(#52700,#52701),(#52702,#52703),(#52704,
#52705),(#52706,#52707),(#52708,#52709),(#52710,#52711),(#52712,#52713),
(#52714,#52715),(#52716,#52717),(#52718,#52719),(#52720,#52721),(#52722,
#52723),(#52724,#52725),(#52726,#52727),(#52728,#52729)),.UNSPECIFIED.,
 .F.,.F.,.F.)
B_SPLINE_SURFACE_WITH_KNOTS((6,1,1,1,1,1,1,1,1,1,1,1,1,1,1,1,1,1,1,1,1,
1,1,1,1,1,1,1,1,1,1,1,1,1,1,1,1,1,1,1,1,1,1,1,1,1,1,1,1,1,1,1,1,1,1,1,1,
1,1,1,1,1,1,1,1,6),(2,2),(-1.,-0.984615384615383,-0.969230769230768,-0.953846153846152,
-0.938461538461537,-0.923076923076922,-0.907692307692306,-0.892307692307691,
-0.876923076923076,-0.86153846153846,-0.846153846153845,-0.83076923076923,
-0.815384615384614,-0.799999999999999,-0.784615384615384,-0.769230769230768,
-0.753846153846153,-0.738461538461538,-0.723076923076922,-0.707692307692307,
-0.692307692307692,-0.676923076923076,-0.661538461538461,-0.646153846153846,
-0.63076923076923,-0.615384615384615,-0.6,-0.584615384615384,-0.569230769230769,
-0.553846153846154,-0.538461538461538,-0.523076923076923,-0.507692307692308,
-0.492307692307692,-0.476923076923077,-0.461538461538462,-0.446153846153846,
-0.430769230769231,-0.415384615384615,-0.4,-0.384615384615385,-0.369230769230769,
-0.353846153846154,-0.338461538461538,-0.323076923076923,-0.307692307692308,
-0.292307692307692,-0.276923076923077,-0.261538461538462,-0.246153846153846,
-0.230769230769231,-0.215384615384615,-0.2,-0.184615384615385,-0.169230769230769,
-0.153846153846154,-0.138461538461538,-0.123076923076923,-0.107692307692308,
-0.0923076923076923,-0.0769230769230769,-0.0615384615384615,-0.0461538461538462,
-0.0307692307692308,-0.0153846153846154,0.),(-1.,1.),.UNSPECIFIED.)
GEOMETRIC_REPRESENTATION_ITEM()
RATIONAL_B_SPLINE_SURFACE(((1.,1.),(1.,1.),(1.,1.),(1.,1.),(1.,1.),(1.,
1.),(1.,1.),(1.,1.),(1.,1.),(1.,1.),(1.,1.),(1.,1.),(1.,1.),(1.,1.),(1.,
1.),(1.,1.),(1.,1.),(1.,1.),(1.,1.),(1.,1.),(1.,1.),(1.,1.),(1.,1.),(1.,
1.),(1.,1.),(1.,1.),(1.,1.),(1.,1.),(1.,1.),(1.,1.),(1.,1.),(1.,1.),(1.,
1.),(1.,1.),(1.,1.),(1.,1.),(1.,1.),(1.,1.),(1.,1.),(1.,1.),(1.,1.),(1.,
1.),(1.,1.),(1.,1.),(1.,1.),(1.,1.),(1.,1.),(1.,1.),(1.,1.),(1.,1.),(1.,
1.),(1.,1.),(1.,1.),(1.,1.),(1.,1.),(1.,1.),(1.,1.),(1.,1.),(1.,1.),(1.,
1.),(1.,1.),(1.,1.),(1.,1.),(1.,1.),(1.,1.),(1.,1.),(1.,1.),(1.,1.),(1.,
1.),(1.,1.)))
REPRESENTATION_ITEM('')
SURFACE()
);
#88=(
BOUNDED_SURFACE()
B_SPLINE_SURFACE(5,1,((#52802,#52803),(#52804,#52805),(#52806,#52807),(#52808,
#52809),(#52810,#52811),(#52812,#52813),(#52814,#52815),(#52816,#52817),
(#52818,#52819),(#52820,#52821),(#52822,#52823),(#52824,#52825),(#52826,
#52827),(#52828,#52829),(#52830,#52831),(#52832,#52833),(#52834,#52835),
(#52836,#52837),(#52838,#52839),(#52840,#52841),(#52842,#52843),(#52844,
#52845),(#52846,#52847),(#52848,#52849),(#52850,#52851),(#52852,#52853),
(#52854,#52855),(#52856,#52857),(#52858,#52859),(#52860,#52861),(#52862,
#52863),(#52864,#52865),(#52866,#52867),(#52868,#52869),(#52870,#52871),
(#52872,#52873),(#52874,#52875),(#52876,#52877),(#52878,#52879),(#52880,
#52881),(#52882,#52883),(#52884,#52885),(#52886,#52887),(#52888,#52889),
(#52890,#52891),(#52892,#52893),(#52894,#52895),(#52896,#52897),(#52898,
#52899),(#52900,#52901),(#52902,#52903),(#52904,#52905),(#52906,#52907),
(#52908,#52909),(#52910,#52911),(#52912,#52913),(#52914,#52915),(#52916,
#52917),(#52918,#52919),(#52920,#52921),(#52922,#52923),(#52924,#52925),
(#52926,#52927),(#52928,#52929),(#52930,#52931),(#52932,#52933),(#52934,
#52935),(#52936,#52937),(#52938,#52939),(#52940,#52941)),.UNSPECIFIED.,
 .F.,.F.,.F.)
B_SPLINE_SURFACE_WITH_KNOTS((6,1,1,1,1,1,1,1,1,1,1,1,1,1,1,1,1,1,1,1,1,
1,1,1,1,1,1,1,1,1,1,1,1,1,1,1,1,1,1,1,1,1,1,1,1,1,1,1,1,1,1,1,1,1,1,1,1,
1,1,1,1,1,1,1,1,6),(2,2),(-1.,-0.984615384615383,-0.969230769230768,-0.953846153846152,
-0.938461538461537,-0.923076923076922,-0.907692307692306,-0.892307692307691,
-0.876923076923076,-0.86153846153846,-0.846153846153845,-0.83076923076923,
-0.815384615384614,-0.799999999999999,-0.784615384615384,-0.769230769230768,
-0.753846153846153,-0.738461538461538,-0.723076923076922,-0.707692307692307,
-0.692307692307692,-0.676923076923076,-0.661538461538461,-0.646153846153846,
-0.63076923076923,-0.615384615384615,-0.6,-0.584615384615384,-0.569230769230769,
-0.553846153846154,-0.538461538461538,-0.523076923076923,-0.507692307692308,
-0.492307692307692,-0.476923076923077,-0.461538461538462,-0.446153846153846,
-0.430769230769231,-0.415384615384615,-0.4,-0.384615384615385,-0.369230769230769,
-0.353846153846154,-0.338461538461538,-0.323076923076923,-0.307692307692308,
-0.292307692307692,-0.276923076923077,-0.261538461538462,-0.246153846153846,
-0.230769230769231,-0.215384615384615,-0.2,-0.184615384615385,-0.169230769230769,
-0.153846153846154,-0.138461538461538,-0.123076923076923,-0.107692307692308,
-0.0923076923076923,-0.0769230769230769,-0.0615384615384615,-0.0461538461538462,
-0.0307692307692308,-0.0153846153846154,0.),(-1.,1.),.UNSPECIFIED.)
GEOMETRIC_REPRESENTATION_ITEM()
RATIONAL_B_SPLINE_SURFACE(((1.,1.),(1.,1.),(1.,1.),(1.,1.),(1.,1.),(1.,
1.),(1.,1.),(1.,1.),(1.,1.),(1.,1.),(1.,1.),(1.,1.),(1.,1.),(1.,1.),(1.,
1.),(1.,1.),(1.,1.),(1.,1.),(1.,1.),(1.,1.),(1.,1.),(1.,1.),(1.,1.),(1.,
1.),(1.,1.),(1.,1.),(1.,1.),(1.,1.),(1.,1.),(1.,1.),(1.,1.),(1.,1.),(1.,
1.),(1.,1.),(1.,1.),(1.,1.),(1.,1.),(1.,1.),(1.,1.),(1.,1.),(1.,1.),(1.,
1.),(1.,1.),(1.,1.),(1.,1.),(1.,1.),(1.,1.),(1.,1.),(1.,1.),(1.,1.),(1.,
1.),(1.,1.),(1.,1.),(1.,1.),(1.,1.),(1.,1.),(1.,1.),(1.,1.),(1.,1.),(1.,
1.),(1.,1.),(1.,1.),(1.,1.),(1.,1.),(1.,1.),(1.,1.),(1.,1.),(1.,1.),(1.,
1.),(1.,1.)))
REPRESENTATION_ITEM('')
SURFACE()
);
#89=(
BOUNDED_SURFACE()
B_SPLINE_SURFACE(5,1,((#53032,#53033),(#53034,#53035),(#53036,#53037),(#53038,
#53039),(#53040,#53041),(#53042,#53043),(#53044,#53045),(#53046,#53047),
(#53048,#53049),(#53050,#53051),(#53052,#53053),(#53054,#53055),(#53056,
#53057),(#53058,#53059),(#53060,#53061),(#53062,#53063),(#53064,#53065),
(#53066,#53067),(#53068,#53069),(#53070,#53071),(#53072,#53073),(#53074,
#53075),(#53076,#53077),(#53078,#53079),(#53080,#53081),(#53082,#53083),
(#53084,#53085),(#53086,#53087),(#53088,#53089),(#53090,#53091),(#53092,
#53093),(#53094,#53095),(#53096,#53097),(#53098,#53099),(#53100,#53101),
(#53102,#53103),(#53104,#53105),(#53106,#53107),(#53108,#53109),(#53110,
#53111),(#53112,#53113),(#53114,#53115),(#53116,#53117),(#53118,#53119),
(#53120,#53121),(#53122,#53123),(#53124,#53125),(#53126,#53127),(#53128,
#53129),(#53130,#53131),(#53132,#53133),(#53134,#53135),(#53136,#53137),
(#53138,#53139),(#53140,#53141),(#53142,#53143),(#53144,#53145),(#53146,
#53147),(#53148,#53149),(#53150,#53151),(#53152,#53153),(#53154,#53155),
(#53156,#53157),(#53158,#53159),(#53160,#53161),(#53162,#53163),(#53164,
#53165),(#53166,#53167),(#53168,#53169),(#53170,#53171)),.UNSPECIFIED.,
 .F.,.F.,.F.)
B_SPLINE_SURFACE_WITH_KNOTS((6,1,1,1,1,1,1,1,1,1,1,1,1,1,1,1,1,1,1,1,1,
1,1,1,1,1,1,1,1,1,1,1,1,1,1,1,1,1,1,1,1,1,1,1,1,1,1,1,1,1,1,1,1,1,1,1,1,
1,1,1,1,1,1,1,1,6),(2,2),(-1.,-0.984615384615383,-0.969230769230768,-0.953846153846152,
-0.938461538461537,-0.923076923076922,-0.907692307692306,-0.892307692307691,
-0.876923076923076,-0.86153846153846,-0.846153846153845,-0.83076923076923,
-0.815384615384614,-0.799999999999999,-0.784615384615384,-0.769230769230768,
-0.753846153846153,-0.738461538461538,-0.723076923076922,-0.707692307692307,
-0.692307692307692,-0.676923076923076,-0.661538461538461,-0.646153846153846,
-0.63076923076923,-0.615384615384615,-0.6,-0.584615384615384,-0.569230769230769,
-0.553846153846154,-0.538461538461538,-0.523076923076923,-0.507692307692308,
-0.492307692307692,-0.476923076923077,-0.461538461538462,-0.446153846153846,
-0.430769230769231,-0.415384615384615,-0.4,-0.384615384615385,-0.369230769230769,
-0.353846153846154,-0.338461538461538,-0.323076923076923,-0.307692307692308,
-0.292307692307692,-0.276923076923077,-0.261538461538462,-0.246153846153846,
-0.230769230769231,-0.215384615384615,-0.2,-0.184615384615385,-0.169230769230769,
-0.153846153846154,-0.138461538461538,-0.123076923076923,-0.107692307692308,
-0.0923076923076923,-0.0769230769230769,-0.0615384615384615,-0.0461538461538462,
-0.0307692307692308,-0.0153846153846154,0.),(-1.,1.),.UNSPECIFIED.)
GEOMETRIC_REPRESENTATION_ITEM()
RATIONAL_B_SPLINE_SURFACE(((1.,1.),(1.,1.),(1.,1.),(1.,1.),(1.,1.),(1.,
1.),(1.,1.),(1.,1.),(1.,1.),(1.,1.),(1.,1.),(1.,1.),(1.,1.),(1.,1.),(1.,
1.),(1.,1.),(1.,1.),(1.,1.),(1.,1.),(1.,1.),(1.,1.),(1.,1.),(1.,1.),(1.,
1.),(1.,1.),(1.,1.),(1.,1.),(1.,1.),(1.,1.),(1.,1.),(1.,1.),(1.,1.),(1.,
1.),(1.,1.),(1.,1.),(1.,1.),(1.,1.),(1.,1.),(1.,1.),(1.,1.),(1.,1.),(1.,
1.),(1.,1.),(1.,1.),(1.,1.),(1.,1.),(1.,1.),(1.,1.),(1.,1.),(1.,1.),(1.,
1.),(1.,1.),(1.,1.),(1.,1.),(1.,1.),(1.,1.),(1.,1.),(1.,1.),(1.,1.),(1.,
1.),(1.,1.),(1.,1.),(1.,1.),(1.,1.),(1.,1.),(1.,1.),(1.,1.),(1.,1.),(1.,
1.),(1.,1.)))
REPRESENTATION_ITEM('')
SURFACE()
);
#90=(
BOUNDED_SURFACE()
B_SPLINE_SURFACE(5,1,((#53244,#53245),(#53246,#53247),(#53248,#53249),(#53250,
#53251),(#53252,#53253),(#53254,#53255),(#53256,#53257),(#53258,#53259),
(#53260,#53261),(#53262,#53263),(#53264,#53265),(#53266,#53267),(#53268,
#53269),(#53270,#53271),(#53272,#53273),(#53274,#53275),(#53276,#53277),
(#53278,#53279),(#53280,#53281),(#53282,#53283),(#53284,#53285),(#53286,
#53287),(#53288,#53289),(#53290,#53291),(#53292,#53293),(#53294,#53295),
(#53296,#53297),(#53298,#53299),(#53300,#53301),(#53302,#53303),(#53304,
#53305),(#53306,#53307),(#53308,#53309),(#53310,#53311),(#53312,#53313),
(#53314,#53315),(#53316,#53317),(#53318,#53319),(#53320,#53321),(#53322,
#53323),(#53324,#53325),(#53326,#53327),(#53328,#53329),(#53330,#53331),
(#53332,#53333),(#53334,#53335),(#53336,#53337),(#53338,#53339),(#53340,
#53341),(#53342,#53343),(#53344,#53345),(#53346,#53347),(#53348,#53349),
(#53350,#53351),(#53352,#53353),(#53354,#53355),(#53356,#53357),(#53358,
#53359),(#53360,#53361),(#53362,#53363),(#53364,#53365),(#53366,#53367),
(#53368,#53369),(#53370,#53371),(#53372,#53373),(#53374,#53375),(#53376,
#53377),(#53378,#53379),(#53380,#53381),(#53382,#53383)),.UNSPECIFIED.,
 .F.,.F.,.F.)
B_SPLINE_SURFACE_WITH_KNOTS((6,1,1,1,1,1,1,1,1,1,1,1,1,1,1,1,1,1,1,1,1,
1,1,1,1,1,1,1,1,1,1,1,1,1,1,1,1,1,1,1,1,1,1,1,1,1,1,1,1,1,1,1,1,1,1,1,1,
1,1,1,1,1,1,1,1,6),(2,2),(-1.,-0.984615384615383,-0.969230769230768,-0.953846153846152,
-0.938461538461537,-0.923076923076922,-0.907692307692306,-0.892307692307691,
-0.876923076923076,-0.86153846153846,-0.846153846153845,-0.83076923076923,
-0.815384615384614,-0.799999999999999,-0.784615384615384,-0.769230769230768,
-0.753846153846153,-0.738461538461538,-0.723076923076922,-0.707692307692307,
-0.692307692307692,-0.676923076923076,-0.661538461538461,-0.646153846153846,
-0.63076923076923,-0.615384615384615,-0.6,-0.584615384615384,-0.569230769230769,
-0.553846153846154,-0.538461538461538,-0.523076923076923,-0.507692307692308,
-0.492307692307692,-0.476923076923077,-0.461538461538462,-0.446153846153846,
-0.430769230769231,-0.415384615384615,-0.4,-0.384615384615385,-0.369230769230769,
-0.353846153846154,-0.338461538461538,-0.323076923076923,-0.307692307692308,
-0.292307692307692,-0.276923076923077,-0.261538461538462,-0.246153846153846,
-0.230769230769231,-0.215384615384615,-0.2,-0.184615384615385,-0.169230769230769,
-0.153846153846154,-0.138461538461538,-0.123076923076923,-0.107692307692308,
-0.0923076923076923,-0.0769230769230769,-0.0615384615384615,-0.0461538461538462,
-0.0307692307692308,-0.0153846153846154,0.),(-1.,1.),.UNSPECIFIED.)
GEOMETRIC_REPRESENTATION_ITEM()
RATIONAL_B_SPLINE_SURFACE(((1.,1.),(1.,1.),(1.,1.),(1.,1.),(1.,1.),(1.,
1.),(1.,1.),(1.,1.),(1.,1.),(1.,1.),(1.,1.),(1.,1.),(1.,1.),(1.,1.),(1.,
1.),(1.,1.),(1.,1.),(1.,1.),(1.,1.),(1.,1.),(1.,1.),(1.,1.),(1.,1.),(1.,
1.),(1.,1.),(1.,1.),(1.,1.),(1.,1.),(1.,1.),(1.,1.),(1.,1.),(1.,1.),(1.,
1.),(1.,1.),(1.,1.),(1.,1.),(1.,1.),(1.,1.),(1.,1.),(1.,1.),(1.,1.),(1.,
1.),(1.,1.),(1.,1.),(1.,1.),(1.,1.),(1.,1.),(1.,1.),(1.,1.),(1.,1.),(1.,
1.),(1.,1.),(1.,1.),(1.,1.),(1.,1.),(1.,1.),(1.,1.),(1.,1.),(1.,1.),(1.,
1.),(1.,1.),(1.,1.),(1.,1.),(1.,1.),(1.,1.),(1.,1.),(1.,1.),(1.,1.),(1.,
1.),(1.,1.)))
REPRESENTATION_ITEM('')
SURFACE()
);
#91=(
BOUNDED_SURFACE()
B_SPLINE_SURFACE(5,1,((#53474,#53475),(#53476,#53477),(#53478,#53479),(#53480,
#53481),(#53482,#53483),(#53484,#53485),(#53486,#53487),(#53488,#53489),
(#53490,#53491),(#53492,#53493),(#53494,#53495),(#53496,#53497),(#53498,
#53499),(#53500,#53501),(#53502,#53503),(#53504,#53505),(#53506,#53507),
(#53508,#53509),(#53510,#53511),(#53512,#53513),(#53514,#53515),(#53516,
#53517),(#53518,#53519),(#53520,#53521),(#53522,#53523),(#53524,#53525),
(#53526,#53527),(#53528,#53529),(#53530,#53531),(#53532,#53533),(#53534,
#53535),(#53536,#53537),(#53538,#53539),(#53540,#53541),(#53542,#53543),
(#53544,#53545),(#53546,#53547),(#53548,#53549),(#53550,#53551),(#53552,
#53553),(#53554,#53555),(#53556,#53557),(#53558,#53559),(#53560,#53561),
(#53562,#53563),(#53564,#53565),(#53566,#53567),(#53568,#53569),(#53570,
#53571),(#53572,#53573),(#53574,#53575),(#53576,#53577),(#53578,#53579),
(#53580,#53581),(#53582,#53583),(#53584,#53585),(#53586,#53587),(#53588,
#53589),(#53590,#53591),(#53592,#53593),(#53594,#53595),(#53596,#53597),
(#53598,#53599),(#53600,#53601),(#53602,#53603),(#53604,#53605),(#53606,
#53607),(#53608,#53609),(#53610,#53611),(#53612,#53613)),.UNSPECIFIED.,
 .F.,.F.,.F.)
B_SPLINE_SURFACE_WITH_KNOTS((6,1,1,1,1,1,1,1,1,1,1,1,1,1,1,1,1,1,1,1,1,
1,1,1,1,1,1,1,1,1,1,1,1,1,1,1,1,1,1,1,1,1,1,1,1,1,1,1,1,1,1,1,1,1,1,1,1,
1,1,1,1,1,1,1,1,6),(2,2),(-1.,-0.984615384615383,-0.969230769230768,-0.953846153846152,
-0.938461538461537,-0.923076923076922,-0.907692307692306,-0.892307692307691,
-0.876923076923076,-0.86153846153846,-0.846153846153845,-0.83076923076923,
-0.815384615384614,-0.799999999999999,-0.784615384615384,-0.769230769230768,
-0.753846153846153,-0.738461538461538,-0.723076923076922,-0.707692307692307,
-0.692307692307692,-0.676923076923076,-0.661538461538461,-0.646153846153846,
-0.63076923076923,-0.615384615384615,-0.6,-0.584615384615384,-0.569230769230769,
-0.553846153846154,-0.538461538461538,-0.523076923076923,-0.507692307692308,
-0.492307692307692,-0.476923076923077,-0.461538461538462,-0.446153846153846,
-0.430769230769231,-0.415384615384615,-0.4,-0.384615384615385,-0.369230769230769,
-0.353846153846154,-0.338461538461538,-0.323076923076923,-0.307692307692308,
-0.292307692307692,-0.276923076923077,-0.261538461538462,-0.246153846153846,
-0.230769230769231,-0.215384615384615,-0.2,-0.184615384615385,-0.169230769230769,
-0.153846153846154,-0.138461538461538,-0.123076923076923,-0.107692307692308,
-0.0923076923076923,-0.0769230769230769,-0.0615384615384615,-0.0461538461538462,
-0.0307692307692308,-0.0153846153846154,0.),(-1.,1.),.UNSPECIFIED.)
GEOMETRIC_REPRESENTATION_ITEM()
RATIONAL_B_SPLINE_SURFACE(((1.,1.),(1.,1.),(1.,1.),(1.,1.),(1.,1.),(1.,
1.),(1.,1.),(1.,1.),(1.,1.),(1.,1.),(1.,1.),(1.,1.),(1.,1.),(1.,1.),(1.,
1.),(1.,1.),(1.,1.),(1.,1.),(1.,1.),(1.,1.),(1.,1.),(1.,1.),(1.,1.),(1.,
1.),(1.,1.),(1.,1.),(1.,1.),(1.,1.),(1.,1.),(1.,1.),(1.,1.),(1.,1.),(1.,
1.),(1.,1.),(1.,1.),(1.,1.),(1.,1.),(1.,1.),(1.,1.),(1.,1.),(1.,1.),(1.,
1.),(1.,1.),(1.,1.),(1.,1.),(1.,1.),(1.,1.),(1.,1.),(1.,1.),(1.,1.),(1.,
1.),(1.,1.),(1.,1.),(1.,1.),(1.,1.),(1.,1.),(1.,1.),(1.,1.),(1.,1.),(1.,
1.),(1.,1.),(1.,1.),(1.,1.),(1.,1.),(1.,1.),(1.,1.),(1.,1.),(1.,1.),(1.,
1.),(1.,1.)))
REPRESENTATION_ITEM('')
SURFACE()
);
#92=(
BOUNDED_SURFACE()
B_SPLINE_SURFACE(5,1,((#53686,#53687),(#53688,#53689),(#53690,#53691),(#53692,
#53693),(#53694,#53695),(#53696,#53697),(#53698,#53699),(#53700,#53701),
(#53702,#53703),(#53704,#53705),(#53706,#53707),(#53708,#53709),(#53710,
#53711),(#53712,#53713),(#53714,#53715),(#53716,#53717),(#53718,#53719),
(#53720,#53721),(#53722,#53723),(#53724,#53725),(#53726,#53727),(#53728,
#53729),(#53730,#53731),(#53732,#53733),(#53734,#53735),(#53736,#53737),
(#53738,#53739),(#53740,#53741),(#53742,#53743),(#53744,#53745),(#53746,
#53747),(#53748,#53749),(#53750,#53751),(#53752,#53753),(#53754,#53755),
(#53756,#53757),(#53758,#53759),(#53760,#53761),(#53762,#53763),(#53764,
#53765),(#53766,#53767),(#53768,#53769),(#53770,#53771),(#53772,#53773),
(#53774,#53775),(#53776,#53777),(#53778,#53779),(#53780,#53781),(#53782,
#53783),(#53784,#53785),(#53786,#53787),(#53788,#53789),(#53790,#53791),
(#53792,#53793),(#53794,#53795),(#53796,#53797),(#53798,#53799),(#53800,
#53801),(#53802,#53803),(#53804,#53805),(#53806,#53807),(#53808,#53809),
(#53810,#53811),(#53812,#53813),(#53814,#53815),(#53816,#53817),(#53818,
#53819),(#53820,#53821),(#53822,#53823),(#53824,#53825)),.UNSPECIFIED.,
 .F.,.F.,.F.)
B_SPLINE_SURFACE_WITH_KNOTS((6,1,1,1,1,1,1,1,1,1,1,1,1,1,1,1,1,1,1,1,1,
1,1,1,1,1,1,1,1,1,1,1,1,1,1,1,1,1,1,1,1,1,1,1,1,1,1,1,1,1,1,1,1,1,1,1,1,
1,1,1,1,1,1,1,1,6),(2,2),(-1.,-0.984615384615383,-0.969230769230768,-0.953846153846152,
-0.938461538461537,-0.923076923076922,-0.907692307692306,-0.892307692307691,
-0.876923076923076,-0.86153846153846,-0.846153846153845,-0.83076923076923,
-0.815384615384614,-0.799999999999999,-0.784615384615384,-0.769230769230768,
-0.753846153846153,-0.738461538461538,-0.723076923076922,-0.707692307692307,
-0.692307692307692,-0.676923076923076,-0.661538461538461,-0.646153846153846,
-0.63076923076923,-0.615384615384615,-0.6,-0.584615384615384,-0.569230769230769,
-0.553846153846154,-0.538461538461538,-0.523076923076923,-0.507692307692308,
-0.492307692307692,-0.476923076923077,-0.461538461538462,-0.446153846153846,
-0.430769230769231,-0.415384615384615,-0.4,-0.384615384615385,-0.369230769230769,
-0.353846153846154,-0.338461538461538,-0.323076923076923,-0.307692307692308,
-0.292307692307692,-0.276923076923077,-0.261538461538462,-0.246153846153846,
-0.230769230769231,-0.215384615384615,-0.2,-0.184615384615385,-0.169230769230769,
-0.153846153846154,-0.138461538461538,-0.123076923076923,-0.107692307692308,
-0.0923076923076923,-0.0769230769230769,-0.0615384615384615,-0.0461538461538462,
-0.0307692307692308,-0.0153846153846154,0.),(-1.,1.),.UNSPECIFIED.)
GEOMETRIC_REPRESENTATION_ITEM()
RATIONAL_B_SPLINE_SURFACE(((1.,1.),(1.,1.),(1.,1.),(1.,1.),(1.,1.),(1.,
1.),(1.,1.),(1.,1.),(1.,1.),(1.,1.),(1.,1.),(1.,1.),(1.,1.),(1.,1.),(1.,
1.),(1.,1.),(1.,1.),(1.,1.),(1.,1.),(1.,1.),(1.,1.),(1.,1.),(1.,1.),(1.,
1.),(1.,1.),(1.,1.),(1.,1.),(1.,1.),(1.,1.),(1.,1.),(1.,1.),(1.,1.),(1.,
1.),(1.,1.),(1.,1.),(1.,1.),(1.,1.),(1.,1.),(1.,1.),(1.,1.),(1.,1.),(1.,
1.),(1.,1.),(1.,1.),(1.,1.),(1.,1.),(1.,1.),(1.,1.),(1.,1.),(1.,1.),(1.,
1.),(1.,1.),(1.,1.),(1.,1.),(1.,1.),(1.,1.),(1.,1.),(1.,1.),(1.,1.),(1.,
1.),(1.,1.),(1.,1.),(1.,1.),(1.,1.),(1.,1.),(1.,1.),(1.,1.),(1.,1.),(1.,
1.),(1.,1.)))
REPRESENTATION_ITEM('')
SURFACE()
);
#93=(
BOUNDED_SURFACE()
B_SPLINE_SURFACE(5,1,((#53916,#53917),(#53918,#53919),(#53920,#53921),(#53922,
#53923),(#53924,#53925),(#53926,#53927),(#53928,#53929),(#53930,#53931),
(#53932,#53933),(#53934,#53935),(#53936,#53937),(#53938,#53939),(#53940,
#53941),(#53942,#53943),(#53944,#53945),(#53946,#53947),(#53948,#53949),
(#53950,#53951),(#53952,#53953),(#53954,#53955),(#53956,#53957),(#53958,
#53959),(#53960,#53961),(#53962,#53963),(#53964,#53965),(#53966,#53967),
(#53968,#53969),(#53970,#53971),(#53972,#53973),(#53974,#53975),(#53976,
#53977),(#53978,#53979),(#53980,#53981),(#53982,#53983),(#53984,#53985),
(#53986,#53987),(#53988,#53989),(#53990,#53991),(#53992,#53993),(#53994,
#53995),(#53996,#53997),(#53998,#53999),(#54000,#54001),(#54002,#54003),
(#54004,#54005),(#54006,#54007),(#54008,#54009),(#54010,#54011),(#54012,
#54013),(#54014,#54015),(#54016,#54017),(#54018,#54019),(#54020,#54021),
(#54022,#54023),(#54024,#54025),(#54026,#54027),(#54028,#54029),(#54030,
#54031),(#54032,#54033),(#54034,#54035),(#54036,#54037),(#54038,#54039),
(#54040,#54041),(#54042,#54043),(#54044,#54045),(#54046,#54047),(#54048,
#54049),(#54050,#54051),(#54052,#54053),(#54054,#54055)),.UNSPECIFIED.,
 .F.,.F.,.F.)
B_SPLINE_SURFACE_WITH_KNOTS((6,1,1,1,1,1,1,1,1,1,1,1,1,1,1,1,1,1,1,1,1,
1,1,1,1,1,1,1,1,1,1,1,1,1,1,1,1,1,1,1,1,1,1,1,1,1,1,1,1,1,1,1,1,1,1,1,1,
1,1,1,1,1,1,1,1,6),(2,2),(-1.,-0.984615384615383,-0.969230769230768,-0.953846153846152,
-0.938461538461537,-0.923076923076922,-0.907692307692306,-0.892307692307691,
-0.876923076923076,-0.86153846153846,-0.846153846153845,-0.83076923076923,
-0.815384615384614,-0.799999999999999,-0.784615384615384,-0.769230769230768,
-0.753846153846153,-0.738461538461538,-0.723076923076922,-0.707692307692307,
-0.692307692307692,-0.676923076923076,-0.661538461538461,-0.646153846153846,
-0.63076923076923,-0.615384615384615,-0.6,-0.584615384615384,-0.569230769230769,
-0.553846153846154,-0.538461538461538,-0.523076923076923,-0.507692307692308,
-0.492307692307692,-0.476923076923077,-0.461538461538462,-0.446153846153846,
-0.430769230769231,-0.415384615384615,-0.4,-0.384615384615385,-0.369230769230769,
-0.353846153846154,-0.338461538461538,-0.323076923076923,-0.307692307692308,
-0.292307692307692,-0.276923076923077,-0.261538461538462,-0.246153846153846,
-0.230769230769231,-0.215384615384615,-0.2,-0.184615384615385,-0.169230769230769,
-0.153846153846154,-0.138461538461538,-0.123076923076923,-0.107692307692308,
-0.0923076923076923,-0.0769230769230769,-0.0615384615384615,-0.0461538461538462,
-0.0307692307692308,-0.0153846153846154,0.),(-1.,1.),.UNSPECIFIED.)
GEOMETRIC_REPRESENTATION_ITEM()
RATIONAL_B_SPLINE_SURFACE(((1.,1.),(1.,1.),(1.,1.),(1.,1.),(1.,1.),(1.,
1.),(1.,1.),(1.,1.),(1.,1.),(1.,1.),(1.,1.),(1.,1.),(1.,1.),(1.,1.),(1.,
1.),(1.,1.),(1.,1.),(1.,1.),(1.,1.),(1.,1.),(1.,1.),(1.,1.),(1.,1.),(1.,
1.),(1.,1.),(1.,1.),(1.,1.),(1.,1.),(1.,1.),(1.,1.),(1.,1.),(1.,1.),(1.,
1.),(1.,1.),(1.,1.),(1.,1.),(1.,1.),(1.,1.),(1.,1.),(1.,1.),(1.,1.),(1.,
1.),(1.,1.),(1.,1.),(1.,1.),(1.,1.),(1.,1.),(1.,1.),(1.,1.),(1.,1.),(1.,
1.),(1.,1.),(1.,1.),(1.,1.),(1.,1.),(1.,1.),(1.,1.),(1.,1.),(1.,1.),(1.,
1.),(1.,1.),(1.,1.),(1.,1.),(1.,1.),(1.,1.),(1.,1.),(1.,1.),(1.,1.),(1.,
1.),(1.,1.)))
REPRESENTATION_ITEM('')
SURFACE()
);
#94=(
BOUNDED_SURFACE()
B_SPLINE_SURFACE(5,1,((#54128,#54129),(#54130,#54131),(#54132,#54133),(#54134,
#54135),(#54136,#54137),(#54138,#54139),(#54140,#54141),(#54142,#54143),
(#54144,#54145),(#54146,#54147),(#54148,#54149),(#54150,#54151),(#54152,
#54153),(#54154,#54155),(#54156,#54157),(#54158,#54159),(#54160,#54161),
(#54162,#54163),(#54164,#54165),(#54166,#54167),(#54168,#54169),(#54170,
#54171),(#54172,#54173),(#54174,#54175),(#54176,#54177),(#54178,#54179),
(#54180,#54181),(#54182,#54183),(#54184,#54185),(#54186,#54187),(#54188,
#54189),(#54190,#54191),(#54192,#54193),(#54194,#54195),(#54196,#54197),
(#54198,#54199),(#54200,#54201),(#54202,#54203),(#54204,#54205),(#54206,
#54207),(#54208,#54209),(#54210,#54211),(#54212,#54213),(#54214,#54215),
(#54216,#54217),(#54218,#54219),(#54220,#54221),(#54222,#54223),(#54224,
#54225),(#54226,#54227),(#54228,#54229),(#54230,#54231),(#54232,#54233),
(#54234,#54235),(#54236,#54237),(#54238,#54239),(#54240,#54241),(#54242,
#54243),(#54244,#54245),(#54246,#54247),(#54248,#54249),(#54250,#54251),
(#54252,#54253),(#54254,#54255),(#54256,#54257),(#54258,#54259),(#54260,
#54261),(#54262,#54263),(#54264,#54265),(#54266,#54267)),.UNSPECIFIED.,
 .F.,.F.,.F.)
B_SPLINE_SURFACE_WITH_KNOTS((6,1,1,1,1,1,1,1,1,1,1,1,1,1,1,1,1,1,1,1,1,
1,1,1,1,1,1,1,1,1,1,1,1,1,1,1,1,1,1,1,1,1,1,1,1,1,1,1,1,1,1,1,1,1,1,1,1,
1,1,1,1,1,1,1,1,6),(2,2),(-1.,-0.984615384615383,-0.969230769230768,-0.953846153846152,
-0.938461538461537,-0.923076923076922,-0.907692307692306,-0.892307692307691,
-0.876923076923076,-0.86153846153846,-0.846153846153845,-0.83076923076923,
-0.815384615384614,-0.799999999999999,-0.784615384615384,-0.769230769230768,
-0.753846153846153,-0.738461538461538,-0.723076923076922,-0.707692307692307,
-0.692307692307692,-0.676923076923076,-0.661538461538461,-0.646153846153846,
-0.63076923076923,-0.615384615384615,-0.6,-0.584615384615384,-0.569230769230769,
-0.553846153846154,-0.538461538461538,-0.523076923076923,-0.507692307692308,
-0.492307692307692,-0.476923076923077,-0.461538461538462,-0.446153846153846,
-0.430769230769231,-0.415384615384615,-0.4,-0.384615384615385,-0.369230769230769,
-0.353846153846154,-0.338461538461538,-0.323076923076923,-0.307692307692308,
-0.292307692307692,-0.276923076923077,-0.261538461538462,-0.246153846153846,
-0.230769230769231,-0.215384615384615,-0.2,-0.184615384615385,-0.169230769230769,
-0.153846153846154,-0.138461538461538,-0.123076923076923,-0.107692307692308,
-0.0923076923076923,-0.0769230769230769,-0.0615384615384615,-0.0461538461538462,
-0.0307692307692308,-0.0153846153846154,0.),(-1.,1.),.UNSPECIFIED.)
GEOMETRIC_REPRESENTATION_ITEM()
RATIONAL_B_SPLINE_SURFACE(((1.,1.),(1.,1.),(1.,1.),(1.,1.),(1.,1.),(1.,
1.),(1.,1.),(1.,1.),(1.,1.),(1.,1.),(1.,1.),(1.,1.),(1.,1.),(1.,1.),(1.,
1.),(1.,1.),(1.,1.),(1.,1.),(1.,1.),(1.,1.),(1.,1.),(1.,1.),(1.,1.),(1.,
1.),(1.,1.),(1.,1.),(1.,1.),(1.,1.),(1.,1.),(1.,1.),(1.,1.),(1.,1.),(1.,
1.),(1.,1.),(1.,1.),(1.,1.),(1.,1.),(1.,1.),(1.,1.),(1.,1.),(1.,1.),(1.,
1.),(1.,1.),(1.,1.),(1.,1.),(1.,1.),(1.,1.),(1.,1.),(1.,1.),(1.,1.),(1.,
1.),(1.,1.),(1.,1.),(1.,1.),(1.,1.),(1.,1.),(1.,1.),(1.,1.),(1.,1.),(1.,
1.),(1.,1.),(1.,1.),(1.,1.),(1.,1.),(1.,1.),(1.,1.),(1.,1.),(1.,1.),(1.,
1.),(1.,1.)))
REPRESENTATION_ITEM('')
SURFACE()
);
#95=(
BOUNDED_SURFACE()
B_SPLINE_SURFACE(5,1,((#54358,#54359),(#54360,#54361),(#54362,#54363),(#54364,
#54365),(#54366,#54367),(#54368,#54369),(#54370,#54371),(#54372,#54373),
(#54374,#54375),(#54376,#54377),(#54378,#54379),(#54380,#54381),(#54382,
#54383),(#54384,#54385),(#54386,#54387),(#54388,#54389),(#54390,#54391),
(#54392,#54393),(#54394,#54395),(#54396,#54397),(#54398,#54399),(#54400,
#54401),(#54402,#54403),(#54404,#54405),(#54406,#54407),(#54408,#54409),
(#54410,#54411),(#54412,#54413),(#54414,#54415),(#54416,#54417),(#54418,
#54419),(#54420,#54421),(#54422,#54423),(#54424,#54425),(#54426,#54427),
(#54428,#54429),(#54430,#54431),(#54432,#54433),(#54434,#54435),(#54436,
#54437),(#54438,#54439),(#54440,#54441),(#54442,#54443),(#54444,#54445),
(#54446,#54447),(#54448,#54449),(#54450,#54451),(#54452,#54453),(#54454,
#54455),(#54456,#54457),(#54458,#54459),(#54460,#54461),(#54462,#54463),
(#54464,#54465),(#54466,#54467),(#54468,#54469),(#54470,#54471),(#54472,
#54473),(#54474,#54475),(#54476,#54477),(#54478,#54479),(#54480,#54481),
(#54482,#54483),(#54484,#54485),(#54486,#54487),(#54488,#54489),(#54490,
#54491),(#54492,#54493),(#54494,#54495),(#54496,#54497)),.UNSPECIFIED.,
 .F.,.F.,.F.)
B_SPLINE_SURFACE_WITH_KNOTS((6,1,1,1,1,1,1,1,1,1,1,1,1,1,1,1,1,1,1,1,1,
1,1,1,1,1,1,1,1,1,1,1,1,1,1,1,1,1,1,1,1,1,1,1,1,1,1,1,1,1,1,1,1,1,1,1,1,
1,1,1,1,1,1,1,1,6),(2,2),(-1.,-0.984615384615383,-0.969230769230768,-0.953846153846152,
-0.938461538461537,-0.923076923076922,-0.907692307692306,-0.892307692307691,
-0.876923076923076,-0.86153846153846,-0.846153846153845,-0.83076923076923,
-0.815384615384614,-0.799999999999999,-0.784615384615384,-0.769230769230768,
-0.753846153846153,-0.738461538461538,-0.723076923076922,-0.707692307692307,
-0.692307692307692,-0.676923076923076,-0.661538461538461,-0.646153846153846,
-0.63076923076923,-0.615384615384615,-0.6,-0.584615384615384,-0.569230769230769,
-0.553846153846154,-0.538461538461538,-0.523076923076923,-0.507692307692308,
-0.492307692307692,-0.476923076923077,-0.461538461538462,-0.446153846153846,
-0.430769230769231,-0.415384615384615,-0.4,-0.384615384615385,-0.369230769230769,
-0.353846153846154,-0.338461538461538,-0.323076923076923,-0.307692307692308,
-0.292307692307692,-0.276923076923077,-0.261538461538462,-0.246153846153846,
-0.230769230769231,-0.215384615384615,-0.2,-0.184615384615385,-0.169230769230769,
-0.153846153846154,-0.138461538461538,-0.123076923076923,-0.107692307692308,
-0.0923076923076923,-0.0769230769230769,-0.0615384615384615,-0.0461538461538462,
-0.0307692307692308,-0.0153846153846154,0.),(-1.,1.),.UNSPECIFIED.)
GEOMETRIC_REPRESENTATION_ITEM()
RATIONAL_B_SPLINE_SURFACE(((1.,1.),(1.,1.),(1.,1.),(1.,1.),(1.,1.),(1.,
1.),(1.,1.),(1.,1.),(1.,1.),(1.,1.),(1.,1.),(1.,1.),(1.,1.),(1.,1.),(1.,
1.),(1.,1.),(1.,1.),(1.,1.),(1.,1.),(1.,1.),(1.,1.),(1.,1.),(1.,1.),(1.,
1.),(1.,1.),(1.,1.),(1.,1.),(1.,1.),(1.,1.),(1.,1.),(1.,1.),(1.,1.),(1.,
1.),(1.,1.),(1.,1.),(1.,1.),(1.,1.),(1.,1.),(1.,1.),(1.,1.),(1.,1.),(1.,
1.),(1.,1.),(1.,1.),(1.,1.),(1.,1.),(1.,1.),(1.,1.),(1.,1.),(1.,1.),(1.,
1.),(1.,1.),(1.,1.),(1.,1.),(1.,1.),(1.,1.),(1.,1.),(1.,1.),(1.,1.),(1.,
1.),(1.,1.),(1.,1.),(1.,1.),(1.,1.),(1.,1.),(1.,1.),(1.,1.),(1.,1.),(1.,
1.),(1.,1.)))
REPRESENTATION_ITEM('')
SURFACE()
);
#96=(
BOUNDED_SURFACE()
B_SPLINE_SURFACE(5,1,((#54570,#54571),(#54572,#54573),(#54574,#54575),(#54576,
#54577),(#54578,#54579),(#54580,#54581),(#54582,#54583),(#54584,#54585),
(#54586,#54587),(#54588,#54589),(#54590,#54591),(#54592,#54593),(#54594,
#54595),(#54596,#54597),(#54598,#54599),(#54600,#54601),(#54602,#54603),
(#54604,#54605),(#54606,#54607),(#54608,#54609),(#54610,#54611),(#54612,
#54613),(#54614,#54615),(#54616,#54617),(#54618,#54619),(#54620,#54621),
(#54622,#54623),(#54624,#54625),(#54626,#54627),(#54628,#54629),(#54630,
#54631),(#54632,#54633),(#54634,#54635),(#54636,#54637),(#54638,#54639),
(#54640,#54641),(#54642,#54643),(#54644,#54645),(#54646,#54647),(#54648,
#54649),(#54650,#54651),(#54652,#54653),(#54654,#54655),(#54656,#54657),
(#54658,#54659),(#54660,#54661),(#54662,#54663),(#54664,#54665),(#54666,
#54667),(#54668,#54669),(#54670,#54671),(#54672,#54673),(#54674,#54675),
(#54676,#54677),(#54678,#54679),(#54680,#54681),(#54682,#54683),(#54684,
#54685),(#54686,#54687),(#54688,#54689),(#54690,#54691),(#54692,#54693),
(#54694,#54695),(#54696,#54697),(#54698,#54699),(#54700,#54701),(#54702,
#54703),(#54704,#54705),(#54706,#54707),(#54708,#54709)),.UNSPECIFIED.,
 .F.,.F.,.F.)
B_SPLINE_SURFACE_WITH_KNOTS((6,1,1,1,1,1,1,1,1,1,1,1,1,1,1,1,1,1,1,1,1,
1,1,1,1,1,1,1,1,1,1,1,1,1,1,1,1,1,1,1,1,1,1,1,1,1,1,1,1,1,1,1,1,1,1,1,1,
1,1,1,1,1,1,1,1,6),(2,2),(-1.,-0.984615384615383,-0.969230769230768,-0.953846153846152,
-0.938461538461537,-0.923076923076922,-0.907692307692306,-0.892307692307691,
-0.876923076923076,-0.86153846153846,-0.846153846153845,-0.83076923076923,
-0.815384615384614,-0.799999999999999,-0.784615384615384,-0.769230769230768,
-0.753846153846153,-0.738461538461538,-0.723076923076922,-0.707692307692307,
-0.692307692307692,-0.676923076923076,-0.661538461538461,-0.646153846153846,
-0.63076923076923,-0.615384615384615,-0.6,-0.584615384615384,-0.569230769230769,
-0.553846153846154,-0.538461538461538,-0.523076923076923,-0.507692307692308,
-0.492307692307692,-0.476923076923077,-0.461538461538462,-0.446153846153846,
-0.430769230769231,-0.415384615384615,-0.4,-0.384615384615385,-0.369230769230769,
-0.353846153846154,-0.338461538461538,-0.323076923076923,-0.307692307692308,
-0.292307692307692,-0.276923076923077,-0.261538461538462,-0.246153846153846,
-0.230769230769231,-0.215384615384615,-0.2,-0.184615384615385,-0.169230769230769,
-0.153846153846154,-0.138461538461538,-0.123076923076923,-0.107692307692308,
-0.0923076923076923,-0.0769230769230769,-0.0615384615384615,-0.0461538461538462,
-0.0307692307692308,-0.0153846153846154,0.),(-1.,1.),.UNSPECIFIED.)
GEOMETRIC_REPRESENTATION_ITEM()
RATIONAL_B_SPLINE_SURFACE(((1.,1.),(1.,1.),(1.,1.),(1.,1.),(1.,1.),(1.,
1.),(1.,1.),(1.,1.),(1.,1.),(1.,1.),(1.,1.),(1.,1.),(1.,1.),(1.,1.),(1.,
1.),(1.,1.),(1.,1.),(1.,1.),(1.,1.),(1.,1.),(1.,1.),(1.,1.),(1.,1.),(1.,
1.),(1.,1.),(1.,1.),(1.,1.),(1.,1.),(1.,1.),(1.,1.),(1.,1.),(1.,1.),(1.,
1.),(1.,1.),(1.,1.),(1.,1.),(1.,1.),(1.,1.),(1.,1.),(1.,1.),(1.,1.),(1.,
1.),(1.,1.),(1.,1.),(1.,1.),(1.,1.),(1.,1.),(1.,1.),(1.,1.),(1.,1.),(1.,
1.),(1.,1.),(1.,1.),(1.,1.),(1.,1.),(1.,1.),(1.,1.),(1.,1.),(1.,1.),(1.,
1.),(1.,1.),(1.,1.),(1.,1.),(1.,1.),(1.,1.),(1.,1.),(1.,1.),(1.,1.),(1.,
1.),(1.,1.)))
REPRESENTATION_ITEM('')
SURFACE()
);
#97=(
BOUNDED_SURFACE()
B_SPLINE_SURFACE(5,1,((#54800,#54801),(#54802,#54803),(#54804,#54805),(#54806,
#54807),(#54808,#54809),(#54810,#54811),(#54812,#54813),(#54814,#54815),
(#54816,#54817),(#54818,#54819),(#54820,#54821),(#54822,#54823),(#54824,
#54825),(#54826,#54827),(#54828,#54829),(#54830,#54831),(#54832,#54833),
(#54834,#54835),(#54836,#54837),(#54838,#54839),(#54840,#54841),(#54842,
#54843),(#54844,#54845),(#54846,#54847),(#54848,#54849),(#54850,#54851),
(#54852,#54853),(#54854,#54855),(#54856,#54857),(#54858,#54859),(#54860,
#54861),(#54862,#54863),(#54864,#54865),(#54866,#54867),(#54868,#54869),
(#54870,#54871),(#54872,#54873),(#54874,#54875),(#54876,#54877),(#54878,
#54879),(#54880,#54881),(#54882,#54883),(#54884,#54885),(#54886,#54887),
(#54888,#54889),(#54890,#54891),(#54892,#54893),(#54894,#54895),(#54896,
#54897),(#54898,#54899),(#54900,#54901),(#54902,#54903),(#54904,#54905),
(#54906,#54907),(#54908,#54909),(#54910,#54911),(#54912,#54913),(#54914,
#54915),(#54916,#54917),(#54918,#54919),(#54920,#54921),(#54922,#54923),
(#54924,#54925),(#54926,#54927),(#54928,#54929),(#54930,#54931),(#54932,
#54933),(#54934,#54935),(#54936,#54937),(#54938,#54939)),.UNSPECIFIED.,
 .F.,.F.,.F.)
B_SPLINE_SURFACE_WITH_KNOTS((6,1,1,1,1,1,1,1,1,1,1,1,1,1,1,1,1,1,1,1,1,
1,1,1,1,1,1,1,1,1,1,1,1,1,1,1,1,1,1,1,1,1,1,1,1,1,1,1,1,1,1,1,1,1,1,1,1,
1,1,1,1,1,1,1,1,6),(2,2),(-1.,-0.984615384615383,-0.969230769230768,-0.953846153846152,
-0.938461538461537,-0.923076923076922,-0.907692307692306,-0.892307692307691,
-0.876923076923076,-0.86153846153846,-0.846153846153845,-0.83076923076923,
-0.815384615384614,-0.799999999999999,-0.784615384615384,-0.769230769230768,
-0.753846153846153,-0.738461538461538,-0.723076923076922,-0.707692307692307,
-0.692307692307692,-0.676923076923076,-0.661538461538461,-0.646153846153846,
-0.63076923076923,-0.615384615384615,-0.6,-0.584615384615384,-0.569230769230769,
-0.553846153846154,-0.538461538461538,-0.523076923076923,-0.507692307692308,
-0.492307692307692,-0.476923076923077,-0.461538461538462,-0.446153846153846,
-0.430769230769231,-0.415384615384615,-0.4,-0.384615384615385,-0.369230769230769,
-0.353846153846154,-0.338461538461538,-0.323076923076923,-0.307692307692308,
-0.292307692307692,-0.276923076923077,-0.261538461538462,-0.246153846153846,
-0.230769230769231,-0.215384615384615,-0.2,-0.184615384615385,-0.169230769230769,
-0.153846153846154,-0.138461538461538,-0.123076923076923,-0.107692307692308,
-0.0923076923076923,-0.0769230769230769,-0.0615384615384615,-0.0461538461538462,
-0.0307692307692308,-0.0153846153846154,0.),(-1.,1.),.UNSPECIFIED.)
GEOMETRIC_REPRESENTATION_ITEM()
RATIONAL_B_SPLINE_SURFACE(((1.,1.),(1.,1.),(1.,1.),(1.,1.),(1.,1.),(1.,
1.),(1.,1.),(1.,1.),(1.,1.),(1.,1.),(1.,1.),(1.,1.),(1.,1.),(1.,1.),(1.,
1.),(1.,1.),(1.,1.),(1.,1.),(1.,1.),(1.,1.),(1.,1.),(1.,1.),(1.,1.),(1.,
1.),(1.,1.),(1.,1.),(1.,1.),(1.,1.),(1.,1.),(1.,1.),(1.,1.),(1.,1.),(1.,
1.),(1.,1.),(1.,1.),(1.,1.),(1.,1.),(1.,1.),(1.,1.),(1.,1.),(1.,1.),(1.,
1.),(1.,1.),(1.,1.),(1.,1.),(1.,1.),(1.,1.),(1.,1.),(1.,1.),(1.,1.),(1.,
1.),(1.,1.),(1.,1.),(1.,1.),(1.,1.),(1.,1.),(1.,1.),(1.,1.),(1.,1.),(1.,
1.),(1.,1.),(1.,1.),(1.,1.),(1.,1.),(1.,1.),(1.,1.),(1.,1.),(1.,1.),(1.,
1.),(1.,1.)))
REPRESENTATION_ITEM('')
SURFACE()
);
#98=(
BOUNDED_SURFACE()
B_SPLINE_SURFACE(5,1,((#55012,#55013),(#55014,#55015),(#55016,#55017),(#55018,
#55019),(#55020,#55021),(#55022,#55023),(#55024,#55025),(#55026,#55027),
(#55028,#55029),(#55030,#55031),(#55032,#55033),(#55034,#55035),(#55036,
#55037),(#55038,#55039),(#55040,#55041),(#55042,#55043),(#55044,#55045),
(#55046,#55047),(#55048,#55049),(#55050,#55051),(#55052,#55053),(#55054,
#55055),(#55056,#55057),(#55058,#55059),(#55060,#55061),(#55062,#55063),
(#55064,#55065),(#55066,#55067),(#55068,#55069),(#55070,#55071),(#55072,
#55073),(#55074,#55075),(#55076,#55077),(#55078,#55079),(#55080,#55081),
(#55082,#55083),(#55084,#55085),(#55086,#55087),(#55088,#55089),(#55090,
#55091),(#55092,#55093),(#55094,#55095),(#55096,#55097),(#55098,#55099),
(#55100,#55101),(#55102,#55103),(#55104,#55105),(#55106,#55107),(#55108,
#55109),(#55110,#55111),(#55112,#55113),(#55114,#55115),(#55116,#55117),
(#55118,#55119),(#55120,#55121),(#55122,#55123),(#55124,#55125),(#55126,
#55127),(#55128,#55129),(#55130,#55131),(#55132,#55133),(#55134,#55135),
(#55136,#55137),(#55138,#55139),(#55140,#55141),(#55142,#55143),(#55144,
#55145),(#55146,#55147),(#55148,#55149),(#55150,#55151)),.UNSPECIFIED.,
 .F.,.F.,.F.)
B_SPLINE_SURFACE_WITH_KNOTS((6,1,1,1,1,1,1,1,1,1,1,1,1,1,1,1,1,1,1,1,1,
1,1,1,1,1,1,1,1,1,1,1,1,1,1,1,1,1,1,1,1,1,1,1,1,1,1,1,1,1,1,1,1,1,1,1,1,
1,1,1,1,1,1,1,1,6),(2,2),(-1.,-0.984615384615383,-0.969230769230768,-0.953846153846152,
-0.938461538461537,-0.923076923076922,-0.907692307692306,-0.892307692307691,
-0.876923076923076,-0.86153846153846,-0.846153846153845,-0.83076923076923,
-0.815384615384614,-0.799999999999999,-0.784615384615384,-0.769230769230768,
-0.753846153846153,-0.738461538461538,-0.723076923076922,-0.707692307692307,
-0.692307692307692,-0.676923076923076,-0.661538461538461,-0.646153846153846,
-0.63076923076923,-0.615384615384615,-0.6,-0.584615384615384,-0.569230769230769,
-0.553846153846154,-0.538461538461538,-0.523076923076923,-0.507692307692308,
-0.492307692307692,-0.476923076923077,-0.461538461538462,-0.446153846153846,
-0.430769230769231,-0.415384615384615,-0.4,-0.384615384615385,-0.369230769230769,
-0.353846153846154,-0.338461538461538,-0.323076923076923,-0.307692307692308,
-0.292307692307692,-0.276923076923077,-0.261538461538462,-0.246153846153846,
-0.230769230769231,-0.215384615384615,-0.2,-0.184615384615385,-0.169230769230769,
-0.153846153846154,-0.138461538461538,-0.123076923076923,-0.107692307692308,
-0.0923076923076923,-0.0769230769230769,-0.0615384615384615,-0.0461538461538462,
-0.0307692307692308,-0.0153846153846154,0.),(-1.,1.),.UNSPECIFIED.)
GEOMETRIC_REPRESENTATION_ITEM()
RATIONAL_B_SPLINE_SURFACE(((1.,1.),(1.,1.),(1.,1.),(1.,1.),(1.,1.),(1.,
1.),(1.,1.),(1.,1.),(1.,1.),(1.,1.),(1.,1.),(1.,1.),(1.,1.),(1.,1.),(1.,
1.),(1.,1.),(1.,1.),(1.,1.),(1.,1.),(1.,1.),(1.,1.),(1.,1.),(1.,1.),(1.,
1.),(1.,1.),(1.,1.),(1.,1.),(1.,1.),(1.,1.),(1.,1.),(1.,1.),(1.,1.),(1.,
1.),(1.,1.),(1.,1.),(1.,1.),(1.,1.),(1.,1.),(1.,1.),(1.,1.),(1.,1.),(1.,
1.),(1.,1.),(1.,1.),(1.,1.),(1.,1.),(1.,1.),(1.,1.),(1.,1.),(1.,1.),(1.,
1.),(1.,1.),(1.,1.),(1.,1.),(1.,1.),(1.,1.),(1.,1.),(1.,1.),(1.,1.),(1.,
1.),(1.,1.),(1.,1.),(1.,1.),(1.,1.),(1.,1.),(1.,1.),(1.,1.),(1.,1.),(1.,
1.),(1.,1.)))
REPRESENTATION_ITEM('')
SURFACE()
);
#99=(
BOUNDED_SURFACE()
B_SPLINE_SURFACE(5,1,((#55242,#55243),(#55244,#55245),(#55246,#55247),(#55248,
#55249),(#55250,#55251),(#55252,#55253),(#55254,#55255),(#55256,#55257),
(#55258,#55259),(#55260,#55261),(#55262,#55263),(#55264,#55265),(#55266,
#55267),(#55268,#55269),(#55270,#55271),(#55272,#55273),(#55274,#55275),
(#55276,#55277),(#55278,#55279),(#55280,#55281),(#55282,#55283),(#55284,
#55285),(#55286,#55287),(#55288,#55289),(#55290,#55291),(#55292,#55293),
(#55294,#55295),(#55296,#55297),(#55298,#55299),(#55300,#55301),(#55302,
#55303),(#55304,#55305),(#55306,#55307),(#55308,#55309),(#55310,#55311),
(#55312,#55313),(#55314,#55315),(#55316,#55317),(#55318,#55319),(#55320,
#55321),(#55322,#55323),(#55324,#55325),(#55326,#55327),(#55328,#55329),
(#55330,#55331),(#55332,#55333),(#55334,#55335),(#55336,#55337),(#55338,
#55339),(#55340,#55341),(#55342,#55343),(#55344,#55345),(#55346,#55347),
(#55348,#55349),(#55350,#55351),(#55352,#55353),(#55354,#55355),(#55356,
#55357),(#55358,#55359),(#55360,#55361),(#55362,#55363),(#55364,#55365),
(#55366,#55367),(#55368,#55369),(#55370,#55371),(#55372,#55373),(#55374,
#55375),(#55376,#55377),(#55378,#55379),(#55380,#55381)),.UNSPECIFIED.,
 .F.,.F.,.F.)
B_SPLINE_SURFACE_WITH_KNOTS((6,1,1,1,1,1,1,1,1,1,1,1,1,1,1,1,1,1,1,1,1,
1,1,1,1,1,1,1,1,1,1,1,1,1,1,1,1,1,1,1,1,1,1,1,1,1,1,1,1,1,1,1,1,1,1,1,1,
1,1,1,1,1,1,1,1,6),(2,2),(-1.,-0.984615384615383,-0.969230769230768,-0.953846153846152,
-0.938461538461537,-0.923076923076922,-0.907692307692306,-0.892307692307691,
-0.876923076923076,-0.86153846153846,-0.846153846153845,-0.83076923076923,
-0.815384615384614,-0.799999999999999,-0.784615384615384,-0.769230769230768,
-0.753846153846153,-0.738461538461538,-0.723076923076922,-0.707692307692307,
-0.692307692307692,-0.676923076923076,-0.661538461538461,-0.646153846153846,
-0.63076923076923,-0.615384615384615,-0.6,-0.584615384615384,-0.569230769230769,
-0.553846153846154,-0.538461538461538,-0.523076923076923,-0.507692307692308,
-0.492307692307692,-0.476923076923077,-0.461538461538462,-0.446153846153846,
-0.430769230769231,-0.415384615384615,-0.4,-0.384615384615385,-0.369230769230769,
-0.353846153846154,-0.338461538461538,-0.323076923076923,-0.307692307692308,
-0.292307692307692,-0.276923076923077,-0.261538461538462,-0.246153846153846,
-0.230769230769231,-0.215384615384615,-0.2,-0.184615384615385,-0.169230769230769,
-0.153846153846154,-0.138461538461538,-0.123076923076923,-0.107692307692308,
-0.0923076923076923,-0.0769230769230769,-0.0615384615384615,-0.0461538461538462,
-0.0307692307692308,-0.0153846153846154,0.),(-1.,1.),.UNSPECIFIED.)
GEOMETRIC_REPRESENTATION_ITEM()
RATIONAL_B_SPLINE_SURFACE(((1.,1.),(1.,1.),(1.,1.),(1.,1.),(1.,1.),(1.,
1.),(1.,1.),(1.,1.),(1.,1.),(1.,1.),(1.,1.),(1.,1.),(1.,1.),(1.,1.),(1.,
1.),(1.,1.),(1.,1.),(1.,1.),(1.,1.),(1.,1.),(1.,1.),(1.,1.),(1.,1.),(1.,
1.),(1.,1.),(1.,1.),(1.,1.),(1.,1.),(1.,1.),(1.,1.),(1.,1.),(1.,1.),(1.,
1.),(1.,1.),(1.,1.),(1.,1.),(1.,1.),(1.,1.),(1.,1.),(1.,1.),(1.,1.),(1.,
1.),(1.,1.),(1.,1.),(1.,1.),(1.,1.),(1.,1.),(1.,1.),(1.,1.),(1.,1.),(1.,
1.),(1.,1.),(1.,1.),(1.,1.),(1.,1.),(1.,1.),(1.,1.),(1.,1.),(1.,1.),(1.,
1.),(1.,1.),(1.,1.),(1.,1.),(1.,1.),(1.,1.),(1.,1.),(1.,1.),(1.,1.),(1.,
1.),(1.,1.)))
REPRESENTATION_ITEM('')
SURFACE()
);
#100=(
BOUNDED_SURFACE()
B_SPLINE_SURFACE(5,1,((#55454,#55455),(#55456,#55457),(#55458,#55459),(#55460,
#55461),(#55462,#55463),(#55464,#55465),(#55466,#55467),(#55468,#55469),
(#55470,#55471),(#55472,#55473),(#55474,#55475),(#55476,#55477),(#55478,
#55479),(#55480,#55481),(#55482,#55483),(#55484,#55485),(#55486,#55487),
(#55488,#55489),(#55490,#55491),(#55492,#55493),(#55494,#55495),(#55496,
#55497),(#55498,#55499),(#55500,#55501),(#55502,#55503),(#55504,#55505),
(#55506,#55507),(#55508,#55509),(#55510,#55511),(#55512,#55513),(#55514,
#55515),(#55516,#55517),(#55518,#55519),(#55520,#55521),(#55522,#55523),
(#55524,#55525),(#55526,#55527),(#55528,#55529),(#55530,#55531),(#55532,
#55533),(#55534,#55535),(#55536,#55537),(#55538,#55539),(#55540,#55541),
(#55542,#55543),(#55544,#55545),(#55546,#55547),(#55548,#55549),(#55550,
#55551),(#55552,#55553),(#55554,#55555),(#55556,#55557),(#55558,#55559),
(#55560,#55561),(#55562,#55563),(#55564,#55565),(#55566,#55567),(#55568,
#55569),(#55570,#55571),(#55572,#55573),(#55574,#55575),(#55576,#55577),
(#55578,#55579),(#55580,#55581),(#55582,#55583),(#55584,#55585),(#55586,
#55587),(#55588,#55589),(#55590,#55591),(#55592,#55593)),.UNSPECIFIED.,
 .F.,.F.,.F.)
B_SPLINE_SURFACE_WITH_KNOTS((6,1,1,1,1,1,1,1,1,1,1,1,1,1,1,1,1,1,1,1,1,
1,1,1,1,1,1,1,1,1,1,1,1,1,1,1,1,1,1,1,1,1,1,1,1,1,1,1,1,1,1,1,1,1,1,1,1,
1,1,1,1,1,1,1,1,6),(2,2),(-1.,-0.984615384615383,-0.969230769230768,-0.953846153846152,
-0.938461538461537,-0.923076923076922,-0.907692307692306,-0.892307692307691,
-0.876923076923076,-0.86153846153846,-0.846153846153845,-0.83076923076923,
-0.815384615384614,-0.799999999999999,-0.784615384615384,-0.769230769230768,
-0.753846153846153,-0.738461538461538,-0.723076923076922,-0.707692307692307,
-0.692307692307692,-0.676923076923076,-0.661538461538461,-0.646153846153846,
-0.63076923076923,-0.615384615384615,-0.6,-0.584615384615384,-0.569230769230769,
-0.553846153846154,-0.538461538461538,-0.523076923076923,-0.507692307692308,
-0.492307692307692,-0.476923076923077,-0.461538461538462,-0.446153846153846,
-0.430769230769231,-0.415384615384615,-0.4,-0.384615384615385,-0.369230769230769,
-0.353846153846154,-0.338461538461538,-0.323076923076923,-0.307692307692308,
-0.292307692307692,-0.276923076923077,-0.261538461538462,-0.246153846153846,
-0.230769230769231,-0.215384615384615,-0.2,-0.184615384615385,-0.169230769230769,
-0.153846153846154,-0.138461538461538,-0.123076923076923,-0.107692307692308,
-0.0923076923076923,-0.0769230769230769,-0.0615384615384615,-0.0461538461538462,
-0.0307692307692308,-0.0153846153846154,0.),(-1.,1.),.UNSPECIFIED.)
GEOMETRIC_REPRESENTATION_ITEM()
RATIONAL_B_SPLINE_SURFACE(((1.,1.),(1.,1.),(1.,1.),(1.,1.),(1.,1.),(1.,
1.),(1.,1.),(1.,1.),(1.,1.),(1.,1.),(1.,1.),(1.,1.),(1.,1.),(1.,1.),(1.,
1.),(1.,1.),(1.,1.),(1.,1.),(1.,1.),(1.,1.),(1.,1.),(1.,1.),(1.,1.),(1.,
1.),(1.,1.),(1.,1.),(1.,1.),(1.,1.),(1.,1.),(1.,1.),(1.,1.),(1.,1.),(1.,
1.),(1.,1.),(1.,1.),(1.,1.),(1.,1.),(1.,1.),(1.,1.),(1.,1.),(1.,1.),(1.,
1.),(1.,1.),(1.,1.),(1.,1.),(1.,1.),(1.,1.),(1.,1.),(1.,1.),(1.,1.),(1.,
1.),(1.,1.),(1.,1.),(1.,1.),(1.,1.),(1.,1.),(1.,1.),(1.,1.),(1.,1.),(1.,
1.),(1.,1.),(1.,1.),(1.,1.),(1.,1.),(1.,1.),(1.,1.),(1.,1.),(1.,1.),(1.,
1.),(1.,1.)))
REPRESENTATION_ITEM('')
SURFACE()
);
#101=(
BOUNDED_SURFACE()
B_SPLINE_SURFACE(5,1,((#55684,#55685),(#55686,#55687),(#55688,#55689),(#55690,
#55691),(#55692,#55693),(#55694,#55695),(#55696,#55697),(#55698,#55699),
(#55700,#55701),(#55702,#55703),(#55704,#55705),(#55706,#55707),(#55708,
#55709),(#55710,#55711),(#55712,#55713),(#55714,#55715),(#55716,#55717),
(#55718,#55719),(#55720,#55721),(#55722,#55723),(#55724,#55725),(#55726,
#55727),(#55728,#55729),(#55730,#55731),(#55732,#55733),(#55734,#55735),
(#55736,#55737),(#55738,#55739),(#55740,#55741),(#55742,#55743),(#55744,
#55745),(#55746,#55747),(#55748,#55749),(#55750,#55751),(#55752,#55753),
(#55754,#55755),(#55756,#55757),(#55758,#55759),(#55760,#55761),(#55762,
#55763),(#55764,#55765),(#55766,#55767),(#55768,#55769),(#55770,#55771),
(#55772,#55773),(#55774,#55775),(#55776,#55777),(#55778,#55779),(#55780,
#55781),(#55782,#55783),(#55784,#55785),(#55786,#55787),(#55788,#55789),
(#55790,#55791),(#55792,#55793),(#55794,#55795),(#55796,#55797),(#55798,
#55799),(#55800,#55801),(#55802,#55803),(#55804,#55805),(#55806,#55807),
(#55808,#55809),(#55810,#55811),(#55812,#55813),(#55814,#55815),(#55816,
#55817),(#55818,#55819),(#55820,#55821),(#55822,#55823)),.UNSPECIFIED.,
 .F.,.F.,.F.)
B_SPLINE_SURFACE_WITH_KNOTS((6,1,1,1,1,1,1,1,1,1,1,1,1,1,1,1,1,1,1,1,1,
1,1,1,1,1,1,1,1,1,1,1,1,1,1,1,1,1,1,1,1,1,1,1,1,1,1,1,1,1,1,1,1,1,1,1,1,
1,1,1,1,1,1,1,1,6),(2,2),(-1.,-0.984615384615383,-0.969230769230768,-0.953846153846152,
-0.938461538461537,-0.923076923076922,-0.907692307692306,-0.892307692307691,
-0.876923076923076,-0.86153846153846,-0.846153846153845,-0.83076923076923,
-0.815384615384614,-0.799999999999999,-0.784615384615384,-0.769230769230768,
-0.753846153846153,-0.738461538461538,-0.723076923076922,-0.707692307692307,
-0.692307692307692,-0.676923076923076,-0.661538461538461,-0.646153846153846,
-0.63076923076923,-0.615384615384615,-0.6,-0.584615384615384,-0.569230769230769,
-0.553846153846154,-0.538461538461538,-0.523076923076923,-0.507692307692308,
-0.492307692307692,-0.476923076923077,-0.461538461538462,-0.446153846153846,
-0.430769230769231,-0.415384615384615,-0.4,-0.384615384615385,-0.369230769230769,
-0.353846153846154,-0.338461538461538,-0.323076923076923,-0.307692307692308,
-0.292307692307692,-0.276923076923077,-0.261538461538462,-0.246153846153846,
-0.230769230769231,-0.215384615384615,-0.2,-0.184615384615385,-0.169230769230769,
-0.153846153846154,-0.138461538461538,-0.123076923076923,-0.107692307692308,
-0.0923076923076923,-0.0769230769230769,-0.0615384615384615,-0.0461538461538462,
-0.0307692307692308,-0.0153846153846154,0.),(-1.,1.),.UNSPECIFIED.)
GEOMETRIC_REPRESENTATION_ITEM()
RATIONAL_B_SPLINE_SURFACE(((1.,1.),(1.,1.),(1.,1.),(1.,1.),(1.,1.),(1.,
1.),(1.,1.),(1.,1.),(1.,1.),(1.,1.),(1.,1.),(1.,1.),(1.,1.),(1.,1.),(1.,
1.),(1.,1.),(1.,1.),(1.,1.),(1.,1.),(1.,1.),(1.,1.),(1.,1.),(1.,1.),(1.,
1.),(1.,1.),(1.,1.),(1.,1.),(1.,1.),(1.,1.),(1.,1.),(1.,1.),(1.,1.),(1.,
1.),(1.,1.),(1.,1.),(1.,1.),(1.,1.),(1.,1.),(1.,1.),(1.,1.),(1.,1.),(1.,
1.),(1.,1.),(1.,1.),(1.,1.),(1.,1.),(1.,1.),(1.,1.),(1.,1.),(1.,1.),(1.,
1.),(1.,1.),(1.,1.),(1.,1.),(1.,1.),(1.,1.),(1.,1.),(1.,1.),(1.,1.),(1.,
1.),(1.,1.),(1.,1.),(1.,1.),(1.,1.),(1.,1.),(1.,1.),(1.,1.),(1.,1.),(1.,
1.),(1.,1.)))
REPRESENTATION_ITEM('')
SURFACE()
);
#102=(
BOUNDED_SURFACE()
B_SPLINE_SURFACE(5,1,((#55896,#55897),(#55898,#55899),(#55900,#55901),(#55902,
#55903),(#55904,#55905),(#55906,#55907),(#55908,#55909),(#55910,#55911),
(#55912,#55913),(#55914,#55915),(#55916,#55917),(#55918,#55919),(#55920,
#55921),(#55922,#55923),(#55924,#55925),(#55926,#55927),(#55928,#55929),
(#55930,#55931),(#55932,#55933),(#55934,#55935),(#55936,#55937),(#55938,
#55939),(#55940,#55941),(#55942,#55943),(#55944,#55945),(#55946,#55947),
(#55948,#55949),(#55950,#55951),(#55952,#55953),(#55954,#55955),(#55956,
#55957),(#55958,#55959),(#55960,#55961),(#55962,#55963),(#55964,#55965),
(#55966,#55967),(#55968,#55969),(#55970,#55971),(#55972,#55973),(#55974,
#55975),(#55976,#55977),(#55978,#55979),(#55980,#55981),(#55982,#55983),
(#55984,#55985),(#55986,#55987),(#55988,#55989),(#55990,#55991),(#55992,
#55993),(#55994,#55995),(#55996,#55997),(#55998,#55999),(#56000,#56001),
(#56002,#56003),(#56004,#56005),(#56006,#56007),(#56008,#56009),(#56010,
#56011),(#56012,#56013),(#56014,#56015),(#56016,#56017),(#56018,#56019),
(#56020,#56021),(#56022,#56023),(#56024,#56025),(#56026,#56027),(#56028,
#56029),(#56030,#56031),(#56032,#56033),(#56034,#56035)),.UNSPECIFIED.,
 .F.,.F.,.F.)
B_SPLINE_SURFACE_WITH_KNOTS((6,1,1,1,1,1,1,1,1,1,1,1,1,1,1,1,1,1,1,1,1,
1,1,1,1,1,1,1,1,1,1,1,1,1,1,1,1,1,1,1,1,1,1,1,1,1,1,1,1,1,1,1,1,1,1,1,1,
1,1,1,1,1,1,1,1,6),(2,2),(-1.,-0.984615384615383,-0.969230769230768,-0.953846153846152,
-0.938461538461537,-0.923076923076922,-0.907692307692306,-0.892307692307691,
-0.876923076923076,-0.86153846153846,-0.846153846153845,-0.83076923076923,
-0.815384615384614,-0.799999999999999,-0.784615384615384,-0.769230769230768,
-0.753846153846153,-0.738461538461538,-0.723076923076922,-0.707692307692307,
-0.692307692307692,-0.676923076923076,-0.661538461538461,-0.646153846153846,
-0.63076923076923,-0.615384615384615,-0.6,-0.584615384615384,-0.569230769230769,
-0.553846153846154,-0.538461538461538,-0.523076923076923,-0.507692307692308,
-0.492307692307692,-0.476923076923077,-0.461538461538462,-0.446153846153846,
-0.430769230769231,-0.415384615384615,-0.4,-0.384615384615385,-0.369230769230769,
-0.353846153846154,-0.338461538461538,-0.323076923076923,-0.307692307692308,
-0.292307692307692,-0.276923076923077,-0.261538461538462,-0.246153846153846,
-0.230769230769231,-0.215384615384615,-0.2,-0.184615384615385,-0.169230769230769,
-0.153846153846154,-0.138461538461538,-0.123076923076923,-0.107692307692308,
-0.0923076923076923,-0.0769230769230769,-0.0615384615384615,-0.0461538461538462,
-0.0307692307692308,-0.0153846153846154,0.),(-1.,1.),.UNSPECIFIED.)
GEOMETRIC_REPRESENTATION_ITEM()
RATIONAL_B_SPLINE_SURFACE(((1.,1.),(1.,1.),(1.,1.),(1.,1.),(1.,1.),(1.,
1.),(1.,1.),(1.,1.),(1.,1.),(1.,1.),(1.,1.),(1.,1.),(1.,1.),(1.,1.),(1.,
1.),(1.,1.),(1.,1.),(1.,1.),(1.,1.),(1.,1.),(1.,1.),(1.,1.),(1.,1.),(1.,
1.),(1.,1.),(1.,1.),(1.,1.),(1.,1.),(1.,1.),(1.,1.),(1.,1.),(1.,1.),(1.,
1.),(1.,1.),(1.,1.),(1.,1.),(1.,1.),(1.,1.),(1.,1.),(1.,1.),(1.,1.),(1.,
1.),(1.,1.),(1.,1.),(1.,1.),(1.,1.),(1.,1.),(1.,1.),(1.,1.),(1.,1.),(1.,
1.),(1.,1.),(1.,1.),(1.,1.),(1.,1.),(1.,1.),(1.,1.),(1.,1.),(1.,1.),(1.,
1.),(1.,1.),(1.,1.),(1.,1.),(1.,1.),(1.,1.),(1.,1.),(1.,1.),(1.,1.),(1.,
1.),(1.,1.)))
REPRESENTATION_ITEM('')
SURFACE()
);
#103=(
BOUNDED_SURFACE()
B_SPLINE_SURFACE(5,1,((#56126,#56127),(#56128,#56129),(#56130,#56131),(#56132,
#56133),(#56134,#56135),(#56136,#56137),(#56138,#56139),(#56140,#56141),
(#56142,#56143),(#56144,#56145),(#56146,#56147),(#56148,#56149),(#56150,
#56151),(#56152,#56153),(#56154,#56155),(#56156,#56157),(#56158,#56159),
(#56160,#56161),(#56162,#56163),(#56164,#56165),(#56166,#56167),(#56168,
#56169),(#56170,#56171),(#56172,#56173),(#56174,#56175),(#56176,#56177),
(#56178,#56179),(#56180,#56181),(#56182,#56183),(#56184,#56185),(#56186,
#56187),(#56188,#56189),(#56190,#56191),(#56192,#56193),(#56194,#56195),
(#56196,#56197),(#56198,#56199),(#56200,#56201),(#56202,#56203),(#56204,
#56205),(#56206,#56207),(#56208,#56209),(#56210,#56211),(#56212,#56213),
(#56214,#56215),(#56216,#56217),(#56218,#56219),(#56220,#56221),(#56222,
#56223),(#56224,#56225),(#56226,#56227),(#56228,#56229),(#56230,#56231),
(#56232,#56233),(#56234,#56235),(#56236,#56237),(#56238,#56239),(#56240,
#56241),(#56242,#56243),(#56244,#56245),(#56246,#56247),(#56248,#56249),
(#56250,#56251),(#56252,#56253),(#56254,#56255),(#56256,#56257),(#56258,
#56259),(#56260,#56261),(#56262,#56263),(#56264,#56265)),.UNSPECIFIED.,
 .F.,.F.,.F.)
B_SPLINE_SURFACE_WITH_KNOTS((6,1,1,1,1,1,1,1,1,1,1,1,1,1,1,1,1,1,1,1,1,
1,1,1,1,1,1,1,1,1,1,1,1,1,1,1,1,1,1,1,1,1,1,1,1,1,1,1,1,1,1,1,1,1,1,1,1,
1,1,1,1,1,1,1,1,6),(2,2),(-1.,-0.984615384615383,-0.969230769230768,-0.953846153846152,
-0.938461538461537,-0.923076923076922,-0.907692307692306,-0.892307692307691,
-0.876923076923076,-0.86153846153846,-0.846153846153845,-0.83076923076923,
-0.815384615384614,-0.799999999999999,-0.784615384615384,-0.769230769230768,
-0.753846153846153,-0.738461538461538,-0.723076923076922,-0.707692307692307,
-0.692307692307692,-0.676923076923076,-0.661538461538461,-0.646153846153846,
-0.63076923076923,-0.615384615384615,-0.6,-0.584615384615384,-0.569230769230769,
-0.553846153846154,-0.538461538461538,-0.523076923076923,-0.507692307692308,
-0.492307692307692,-0.476923076923077,-0.461538461538462,-0.446153846153846,
-0.430769230769231,-0.415384615384615,-0.4,-0.384615384615385,-0.369230769230769,
-0.353846153846154,-0.338461538461538,-0.323076923076923,-0.307692307692308,
-0.292307692307692,-0.276923076923077,-0.261538461538462,-0.246153846153846,
-0.230769230769231,-0.215384615384615,-0.2,-0.184615384615385,-0.169230769230769,
-0.153846153846154,-0.138461538461538,-0.123076923076923,-0.107692307692308,
-0.0923076923076923,-0.0769230769230769,-0.0615384615384615,-0.0461538461538462,
-0.0307692307692308,-0.0153846153846154,0.),(-1.,1.),.UNSPECIFIED.)
GEOMETRIC_REPRESENTATION_ITEM()
RATIONAL_B_SPLINE_SURFACE(((1.,1.),(1.,1.),(1.,1.),(1.,1.),(1.,1.),(1.,
1.),(1.,1.),(1.,1.),(1.,1.),(1.,1.),(1.,1.),(1.,1.),(1.,1.),(1.,1.),(1.,
1.),(1.,1.),(1.,1.),(1.,1.),(1.,1.),(1.,1.),(1.,1.),(1.,1.),(1.,1.),(1.,
1.),(1.,1.),(1.,1.),(1.,1.),(1.,1.),(1.,1.),(1.,1.),(1.,1.),(1.,1.),(1.,
1.),(1.,1.),(1.,1.),(1.,1.),(1.,1.),(1.,1.),(1.,1.),(1.,1.),(1.,1.),(1.,
1.),(1.,1.),(1.,1.),(1.,1.),(1.,1.),(1.,1.),(1.,1.),(1.,1.),(1.,1.),(1.,
1.),(1.,1.),(1.,1.),(1.,1.),(1.,1.),(1.,1.),(1.,1.),(1.,1.),(1.,1.),(1.,
1.),(1.,1.),(1.,1.),(1.,1.),(1.,1.),(1.,1.),(1.,1.),(1.,1.),(1.,1.),(1.,
1.),(1.,1.)))
REPRESENTATION_ITEM('')
SURFACE()
);
#104=(
BOUNDED_SURFACE()
B_SPLINE_SURFACE(5,1,((#56338,#56339),(#56340,#56341),(#56342,#56343),(#56344,
#56345),(#56346,#56347),(#56348,#56349),(#56350,#56351),(#56352,#56353),
(#56354,#56355),(#56356,#56357),(#56358,#56359),(#56360,#56361),(#56362,
#56363),(#56364,#56365),(#56366,#56367),(#56368,#56369),(#56370,#56371),
(#56372,#56373),(#56374,#56375),(#56376,#56377),(#56378,#56379),(#56380,
#56381),(#56382,#56383),(#56384,#56385),(#56386,#56387),(#56388,#56389),
(#56390,#56391),(#56392,#56393),(#56394,#56395),(#56396,#56397),(#56398,
#56399),(#56400,#56401),(#56402,#56403),(#56404,#56405),(#56406,#56407),
(#56408,#56409),(#56410,#56411),(#56412,#56413),(#56414,#56415),(#56416,
#56417),(#56418,#56419),(#56420,#56421),(#56422,#56423),(#56424,#56425),
(#56426,#56427),(#56428,#56429),(#56430,#56431),(#56432,#56433),(#56434,
#56435),(#56436,#56437),(#56438,#56439),(#56440,#56441),(#56442,#56443),
(#56444,#56445),(#56446,#56447),(#56448,#56449),(#56450,#56451),(#56452,
#56453),(#56454,#56455),(#56456,#56457),(#56458,#56459),(#56460,#56461),
(#56462,#56463),(#56464,#56465),(#56466,#56467),(#56468,#56469),(#56470,
#56471),(#56472,#56473),(#56474,#56475),(#56476,#56477)),.UNSPECIFIED.,
 .F.,.F.,.F.)
B_SPLINE_SURFACE_WITH_KNOTS((6,1,1,1,1,1,1,1,1,1,1,1,1,1,1,1,1,1,1,1,1,
1,1,1,1,1,1,1,1,1,1,1,1,1,1,1,1,1,1,1,1,1,1,1,1,1,1,1,1,1,1,1,1,1,1,1,1,
1,1,1,1,1,1,1,1,6),(2,2),(-1.,-0.984615384615383,-0.969230769230768,-0.953846153846152,
-0.938461538461537,-0.923076923076922,-0.907692307692306,-0.892307692307691,
-0.876923076923076,-0.86153846153846,-0.846153846153845,-0.83076923076923,
-0.815384615384614,-0.799999999999999,-0.784615384615384,-0.769230769230768,
-0.753846153846153,-0.738461538461538,-0.723076923076922,-0.707692307692307,
-0.692307692307692,-0.676923076923076,-0.661538461538461,-0.646153846153846,
-0.63076923076923,-0.615384615384615,-0.6,-0.584615384615384,-0.569230769230769,
-0.553846153846154,-0.538461538461538,-0.523076923076923,-0.507692307692308,
-0.492307692307692,-0.476923076923077,-0.461538461538462,-0.446153846153846,
-0.430769230769231,-0.415384615384615,-0.4,-0.384615384615385,-0.369230769230769,
-0.353846153846154,-0.338461538461538,-0.323076923076923,-0.307692307692308,
-0.292307692307692,-0.276923076923077,-0.261538461538462,-0.246153846153846,
-0.230769230769231,-0.215384615384615,-0.2,-0.184615384615385,-0.169230769230769,
-0.153846153846154,-0.138461538461538,-0.123076923076923,-0.107692307692308,
-0.0923076923076923,-0.0769230769230769,-0.0615384615384615,-0.0461538461538462,
-0.0307692307692308,-0.0153846153846154,0.),(-1.,1.),.UNSPECIFIED.)
GEOMETRIC_REPRESENTATION_ITEM()
RATIONAL_B_SPLINE_SURFACE(((1.,1.),(1.,1.),(1.,1.),(1.,1.),(1.,1.),(1.,
1.),(1.,1.),(1.,1.),(1.,1.),(1.,1.),(1.,1.),(1.,1.),(1.,1.),(1.,1.),(1.,
1.),(1.,1.),(1.,1.),(1.,1.),(1.,1.),(1.,1.),(1.,1.),(1.,1.),(1.,1.),(1.,
1.),(1.,1.),(1.,1.),(1.,1.),(1.,1.),(1.,1.),(1.,1.),(1.,1.),(1.,1.),(1.,
1.),(1.,1.),(1.,1.),(1.,1.),(1.,1.),(1.,1.),(1.,1.),(1.,1.),(1.,1.),(1.,
1.),(1.,1.),(1.,1.),(1.,1.),(1.,1.),(1.,1.),(1.,1.),(1.,1.),(1.,1.),(1.,
1.),(1.,1.),(1.,1.),(1.,1.),(1.,1.),(1.,1.),(1.,1.),(1.,1.),(1.,1.),(1.,
1.),(1.,1.),(1.,1.),(1.,1.),(1.,1.),(1.,1.),(1.,1.),(1.,1.),(1.,1.),(1.,
1.),(1.,1.)))
REPRESENTATION_ITEM('')
SURFACE()
);
#105=(
BOUNDED_SURFACE()
B_SPLINE_SURFACE(5,1,((#56568,#56569),(#56570,#56571),(#56572,#56573),(#56574,
#56575),(#56576,#56577),(#56578,#56579),(#56580,#56581),(#56582,#56583),
(#56584,#56585),(#56586,#56587),(#56588,#56589),(#56590,#56591),(#56592,
#56593),(#56594,#56595),(#56596,#56597),(#56598,#56599),(#56600,#56601),
(#56602,#56603),(#56604,#56605),(#56606,#56607),(#56608,#56609),(#56610,
#56611),(#56612,#56613),(#56614,#56615),(#56616,#56617),(#56618,#56619),
(#56620,#56621),(#56622,#56623),(#56624,#56625),(#56626,#56627),(#56628,
#56629),(#56630,#56631),(#56632,#56633),(#56634,#56635),(#56636,#56637),
(#56638,#56639),(#56640,#56641),(#56642,#56643),(#56644,#56645),(#56646,
#56647),(#56648,#56649),(#56650,#56651),(#56652,#56653),(#56654,#56655),
(#56656,#56657),(#56658,#56659),(#56660,#56661),(#56662,#56663),(#56664,
#56665),(#56666,#56667),(#56668,#56669),(#56670,#56671),(#56672,#56673),
(#56674,#56675),(#56676,#56677),(#56678,#56679),(#56680,#56681),(#56682,
#56683),(#56684,#56685),(#56686,#56687),(#56688,#56689),(#56690,#56691),
(#56692,#56693),(#56694,#56695),(#56696,#56697),(#56698,#56699),(#56700,
#56701),(#56702,#56703),(#56704,#56705),(#56706,#56707)),.UNSPECIFIED.,
 .F.,.F.,.F.)
B_SPLINE_SURFACE_WITH_KNOTS((6,1,1,1,1,1,1,1,1,1,1,1,1,1,1,1,1,1,1,1,1,
1,1,1,1,1,1,1,1,1,1,1,1,1,1,1,1,1,1,1,1,1,1,1,1,1,1,1,1,1,1,1,1,1,1,1,1,
1,1,1,1,1,1,1,1,6),(2,2),(-1.,-0.984615384615383,-0.969230769230768,-0.953846153846152,
-0.938461538461537,-0.923076923076922,-0.907692307692306,-0.892307692307691,
-0.876923076923076,-0.86153846153846,-0.846153846153845,-0.83076923076923,
-0.815384615384614,-0.799999999999999,-0.784615384615384,-0.769230769230768,
-0.753846153846153,-0.738461538461538,-0.723076923076922,-0.707692307692307,
-0.692307692307692,-0.676923076923076,-0.661538461538461,-0.646153846153846,
-0.63076923076923,-0.615384615384615,-0.6,-0.584615384615384,-0.569230769230769,
-0.553846153846154,-0.538461538461538,-0.523076923076923,-0.507692307692308,
-0.492307692307692,-0.476923076923077,-0.461538461538462,-0.446153846153846,
-0.430769230769231,-0.415384615384615,-0.4,-0.384615384615385,-0.369230769230769,
-0.353846153846154,-0.338461538461538,-0.323076923076923,-0.307692307692308,
-0.292307692307692,-0.276923076923077,-0.261538461538462,-0.246153846153846,
-0.230769230769231,-0.215384615384615,-0.2,-0.184615384615385,-0.169230769230769,
-0.153846153846154,-0.138461538461538,-0.123076923076923,-0.107692307692308,
-0.0923076923076923,-0.0769230769230769,-0.0615384615384615,-0.0461538461538462,
-0.0307692307692308,-0.0153846153846154,0.),(-1.,1.),.UNSPECIFIED.)
GEOMETRIC_REPRESENTATION_ITEM()
RATIONAL_B_SPLINE_SURFACE(((1.,1.),(1.,1.),(1.,1.),(1.,1.),(1.,1.),(1.,
1.),(1.,1.),(1.,1.),(1.,1.),(1.,1.),(1.,1.),(1.,1.),(1.,1.),(1.,1.),(1.,
1.),(1.,1.),(1.,1.),(1.,1.),(1.,1.),(1.,1.),(1.,1.),(1.,1.),(1.,1.),(1.,
1.),(1.,1.),(1.,1.),(1.,1.),(1.,1.),(1.,1.),(1.,1.),(1.,1.),(1.,1.),(1.,
1.),(1.,1.),(1.,1.),(1.,1.),(1.,1.),(1.,1.),(1.,1.),(1.,1.),(1.,1.),(1.,
1.),(1.,1.),(1.,1.),(1.,1.),(1.,1.),(1.,1.),(1.,1.),(1.,1.),(1.,1.),(1.,
1.),(1.,1.),(1.,1.),(1.,1.),(1.,1.),(1.,1.),(1.,1.),(1.,1.),(1.,1.),(1.,
1.),(1.,1.),(1.,1.),(1.,1.),(1.,1.),(1.,1.),(1.,1.),(1.,1.),(1.,1.),(1.,
1.),(1.,1.)))
REPRESENTATION_ITEM('')
SURFACE()
);
#106=(
BOUNDED_SURFACE()
B_SPLINE_SURFACE(5,1,((#56780,#56781),(#56782,#56783),(#56784,#56785),(#56786,
#56787),(#56788,#56789),(#56790,#56791),(#56792,#56793),(#56794,#56795),
(#56796,#56797),(#56798,#56799),(#56800,#56801),(#56802,#56803),(#56804,
#56805),(#56806,#56807),(#56808,#56809),(#56810,#56811),(#56812,#56813),
(#56814,#56815),(#56816,#56817),(#56818,#56819),(#56820,#56821),(#56822,
#56823),(#56824,#56825),(#56826,#56827),(#56828,#56829),(#56830,#56831),
(#56832,#56833),(#56834,#56835),(#56836,#56837),(#56838,#56839),(#56840,
#56841),(#56842,#56843),(#56844,#56845),(#56846,#56847),(#56848,#56849),
(#56850,#56851),(#56852,#56853),(#56854,#56855),(#56856,#56857),(#56858,
#56859),(#56860,#56861),(#56862,#56863),(#56864,#56865),(#56866,#56867),
(#56868,#56869),(#56870,#56871),(#56872,#56873),(#56874,#56875),(#56876,
#56877),(#56878,#56879),(#56880,#56881),(#56882,#56883),(#56884,#56885),
(#56886,#56887),(#56888,#56889),(#56890,#56891),(#56892,#56893),(#56894,
#56895),(#56896,#56897),(#56898,#56899),(#56900,#56901),(#56902,#56903),
(#56904,#56905),(#56906,#56907),(#56908,#56909),(#56910,#56911),(#56912,
#56913),(#56914,#56915),(#56916,#56917),(#56918,#56919)),.UNSPECIFIED.,
 .F.,.F.,.F.)
B_SPLINE_SURFACE_WITH_KNOTS((6,1,1,1,1,1,1,1,1,1,1,1,1,1,1,1,1,1,1,1,1,
1,1,1,1,1,1,1,1,1,1,1,1,1,1,1,1,1,1,1,1,1,1,1,1,1,1,1,1,1,1,1,1,1,1,1,1,
1,1,1,1,1,1,1,1,6),(2,2),(-1.,-0.984615384615383,-0.969230769230768,-0.953846153846152,
-0.938461538461537,-0.923076923076922,-0.907692307692306,-0.892307692307691,
-0.876923076923076,-0.86153846153846,-0.846153846153845,-0.83076923076923,
-0.815384615384614,-0.799999999999999,-0.784615384615384,-0.769230769230768,
-0.753846153846153,-0.738461538461538,-0.723076923076922,-0.707692307692307,
-0.692307692307692,-0.676923076923076,-0.661538461538461,-0.646153846153846,
-0.63076923076923,-0.615384615384615,-0.6,-0.584615384615384,-0.569230769230769,
-0.553846153846154,-0.538461538461538,-0.523076923076923,-0.507692307692308,
-0.492307692307692,-0.476923076923077,-0.461538461538462,-0.446153846153846,
-0.430769230769231,-0.415384615384615,-0.4,-0.384615384615385,-0.369230769230769,
-0.353846153846154,-0.338461538461538,-0.323076923076923,-0.307692307692308,
-0.292307692307692,-0.276923076923077,-0.261538461538462,-0.246153846153846,
-0.230769230769231,-0.215384615384615,-0.2,-0.184615384615385,-0.169230769230769,
-0.153846153846154,-0.138461538461538,-0.123076923076923,-0.107692307692308,
-0.0923076923076923,-0.0769230769230769,-0.0615384615384615,-0.0461538461538462,
-0.0307692307692308,-0.0153846153846154,0.),(-1.,1.),.UNSPECIFIED.)
GEOMETRIC_REPRESENTATION_ITEM()
RATIONAL_B_SPLINE_SURFACE(((1.,1.),(1.,1.),(1.,1.),(1.,1.),(1.,1.),(1.,
1.),(1.,1.),(1.,1.),(1.,1.),(1.,1.),(1.,1.),(1.,1.),(1.,1.),(1.,1.),(1.,
1.),(1.,1.),(1.,1.),(1.,1.),(1.,1.),(1.,1.),(1.,1.),(1.,1.),(1.,1.),(1.,
1.),(1.,1.),(1.,1.),(1.,1.),(1.,1.),(1.,1.),(1.,1.),(1.,1.),(1.,1.),(1.,
1.),(1.,1.),(1.,1.),(1.,1.),(1.,1.),(1.,1.),(1.,1.),(1.,1.),(1.,1.),(1.,
1.),(1.,1.),(1.,1.),(1.,1.),(1.,1.),(1.,1.),(1.,1.),(1.,1.),(1.,1.),(1.,
1.),(1.,1.),(1.,1.),(1.,1.),(1.,1.),(1.,1.),(1.,1.),(1.,1.),(1.,1.),(1.,
1.),(1.,1.),(1.,1.),(1.,1.),(1.,1.),(1.,1.),(1.,1.),(1.,1.),(1.,1.),(1.,
1.),(1.,1.)))
REPRESENTATION_ITEM('')
SURFACE()
);
#107=(
BOUNDED_SURFACE()
B_SPLINE_SURFACE(5,1,((#57010,#57011),(#57012,#57013),(#57014,#57015),(#57016,
#57017),(#57018,#57019),(#57020,#57021),(#57022,#57023),(#57024,#57025),
(#57026,#57027),(#57028,#57029),(#57030,#57031),(#57032,#57033),(#57034,
#57035),(#57036,#57037),(#57038,#57039),(#57040,#57041),(#57042,#57043),
(#57044,#57045),(#57046,#57047),(#57048,#57049),(#57050,#57051),(#57052,
#57053),(#57054,#57055),(#57056,#57057),(#57058,#57059),(#57060,#57061),
(#57062,#57063),(#57064,#57065),(#57066,#57067),(#57068,#57069),(#57070,
#57071),(#57072,#57073),(#57074,#57075),(#57076,#57077),(#57078,#57079),
(#57080,#57081),(#57082,#57083),(#57084,#57085),(#57086,#57087),(#57088,
#57089),(#57090,#57091),(#57092,#57093),(#57094,#57095),(#57096,#57097),
(#57098,#57099),(#57100,#57101),(#57102,#57103),(#57104,#57105),(#57106,
#57107),(#57108,#57109),(#57110,#57111),(#57112,#57113),(#57114,#57115),
(#57116,#57117),(#57118,#57119),(#57120,#57121),(#57122,#57123),(#57124,
#57125),(#57126,#57127),(#57128,#57129),(#57130,#57131),(#57132,#57133),
(#57134,#57135),(#57136,#57137),(#57138,#57139),(#57140,#57141),(#57142,
#57143),(#57144,#57145),(#57146,#57147),(#57148,#57149)),.UNSPECIFIED.,
 .F.,.F.,.F.)
B_SPLINE_SURFACE_WITH_KNOTS((6,1,1,1,1,1,1,1,1,1,1,1,1,1,1,1,1,1,1,1,1,
1,1,1,1,1,1,1,1,1,1,1,1,1,1,1,1,1,1,1,1,1,1,1,1,1,1,1,1,1,1,1,1,1,1,1,1,
1,1,1,1,1,1,1,1,6),(2,2),(-1.,-0.984615384615383,-0.969230769230768,-0.953846153846152,
-0.938461538461537,-0.923076923076922,-0.907692307692306,-0.892307692307691,
-0.876923076923076,-0.86153846153846,-0.846153846153845,-0.83076923076923,
-0.815384615384614,-0.799999999999999,-0.784615384615384,-0.769230769230768,
-0.753846153846153,-0.738461538461538,-0.723076923076922,-0.707692307692307,
-0.692307692307692,-0.676923076923076,-0.661538461538461,-0.646153846153846,
-0.63076923076923,-0.615384615384615,-0.6,-0.584615384615384,-0.569230769230769,
-0.553846153846154,-0.538461538461538,-0.523076923076923,-0.507692307692308,
-0.492307692307692,-0.476923076923077,-0.461538461538462,-0.446153846153846,
-0.430769230769231,-0.415384615384615,-0.4,-0.384615384615385,-0.369230769230769,
-0.353846153846154,-0.338461538461538,-0.323076923076923,-0.307692307692308,
-0.292307692307692,-0.276923076923077,-0.261538461538462,-0.246153846153846,
-0.230769230769231,-0.215384615384615,-0.2,-0.184615384615385,-0.169230769230769,
-0.153846153846154,-0.138461538461538,-0.123076923076923,-0.107692307692308,
-0.0923076923076923,-0.0769230769230769,-0.0615384615384615,-0.0461538461538462,
-0.0307692307692308,-0.0153846153846154,0.),(-1.,1.),.UNSPECIFIED.)
GEOMETRIC_REPRESENTATION_ITEM()
RATIONAL_B_SPLINE_SURFACE(((1.,1.),(1.,1.),(1.,1.),(1.,1.),(1.,1.),(1.,
1.),(1.,1.),(1.,1.),(1.,1.),(1.,1.),(1.,1.),(1.,1.),(1.,1.),(1.,1.),(1.,
1.),(1.,1.),(1.,1.),(1.,1.),(1.,1.),(1.,1.),(1.,1.),(1.,1.),(1.,1.),(1.,
1.),(1.,1.),(1.,1.),(1.,1.),(1.,1.),(1.,1.),(1.,1.),(1.,1.),(1.,1.),(1.,
1.),(1.,1.),(1.,1.),(1.,1.),(1.,1.),(1.,1.),(1.,1.),(1.,1.),(1.,1.),(1.,
1.),(1.,1.),(1.,1.),(1.,1.),(1.,1.),(1.,1.),(1.,1.),(1.,1.),(1.,1.),(1.,
1.),(1.,1.),(1.,1.),(1.,1.),(1.,1.),(1.,1.),(1.,1.),(1.,1.),(1.,1.),(1.,
1.),(1.,1.),(1.,1.),(1.,1.),(1.,1.),(1.,1.),(1.,1.),(1.,1.),(1.,1.),(1.,
1.),(1.,1.)))
REPRESENTATION_ITEM('')
SURFACE()
);
#108=(
BOUNDED_SURFACE()
B_SPLINE_SURFACE(5,1,((#57222,#57223),(#57224,#57225),(#57226,#57227),(#57228,
#57229),(#57230,#57231),(#57232,#57233),(#57234,#57235),(#57236,#57237),
(#57238,#57239),(#57240,#57241),(#57242,#57243),(#57244,#57245),(#57246,
#57247),(#57248,#57249),(#57250,#57251),(#57252,#57253),(#57254,#57255),
(#57256,#57257),(#57258,#57259),(#57260,#57261),(#57262,#57263),(#57264,
#57265),(#57266,#57267),(#57268,#57269),(#57270,#57271),(#57272,#57273),
(#57274,#57275),(#57276,#57277),(#57278,#57279),(#57280,#57281),(#57282,
#57283),(#57284,#57285),(#57286,#57287),(#57288,#57289),(#57290,#57291),
(#57292,#57293),(#57294,#57295),(#57296,#57297),(#57298,#57299),(#57300,
#57301),(#57302,#57303),(#57304,#57305),(#57306,#57307),(#57308,#57309),
(#57310,#57311),(#57312,#57313),(#57314,#57315),(#57316,#57317),(#57318,
#57319),(#57320,#57321),(#57322,#57323),(#57324,#57325),(#57326,#57327),
(#57328,#57329),(#57330,#57331),(#57332,#57333),(#57334,#57335),(#57336,
#57337),(#57338,#57339),(#57340,#57341),(#57342,#57343),(#57344,#57345),
(#57346,#57347),(#57348,#57349),(#57350,#57351),(#57352,#57353),(#57354,
#57355),(#57356,#57357),(#57358,#57359),(#57360,#57361)),.UNSPECIFIED.,
 .F.,.F.,.F.)
B_SPLINE_SURFACE_WITH_KNOTS((6,1,1,1,1,1,1,1,1,1,1,1,1,1,1,1,1,1,1,1,1,
1,1,1,1,1,1,1,1,1,1,1,1,1,1,1,1,1,1,1,1,1,1,1,1,1,1,1,1,1,1,1,1,1,1,1,1,
1,1,1,1,1,1,1,1,6),(2,2),(-1.,-0.984615384615383,-0.969230769230768,-0.953846153846152,
-0.938461538461537,-0.923076923076922,-0.907692307692306,-0.892307692307691,
-0.876923076923076,-0.86153846153846,-0.846153846153845,-0.83076923076923,
-0.815384615384614,-0.799999999999999,-0.784615384615384,-0.769230769230768,
-0.753846153846153,-0.738461538461538,-0.723076923076922,-0.707692307692307,
-0.692307692307692,-0.676923076923076,-0.661538461538461,-0.646153846153846,
-0.63076923076923,-0.615384615384615,-0.6,-0.584615384615384,-0.569230769230769,
-0.553846153846154,-0.538461538461538,-0.523076923076923,-0.507692307692308,
-0.492307692307692,-0.476923076923077,-0.461538461538462,-0.446153846153846,
-0.430769230769231,-0.415384615384615,-0.4,-0.384615384615385,-0.369230769230769,
-0.353846153846154,-0.338461538461538,-0.323076923076923,-0.307692307692308,
-0.292307692307692,-0.276923076923077,-0.261538461538462,-0.246153846153846,
-0.230769230769231,-0.215384615384615,-0.2,-0.184615384615385,-0.169230769230769,
-0.153846153846154,-0.138461538461538,-0.123076923076923,-0.107692307692308,
-0.0923076923076923,-0.0769230769230769,-0.0615384615384615,-0.0461538461538462,
-0.0307692307692308,-0.0153846153846154,0.),(-1.,1.),.UNSPECIFIED.)
GEOMETRIC_REPRESENTATION_ITEM()
RATIONAL_B_SPLINE_SURFACE(((1.,1.),(1.,1.),(1.,1.),(1.,1.),(1.,1.),(1.,
1.),(1.,1.),(1.,1.),(1.,1.),(1.,1.),(1.,1.),(1.,1.),(1.,1.),(1.,1.),(1.,
1.),(1.,1.),(1.,1.),(1.,1.),(1.,1.),(1.,1.),(1.,1.),(1.,1.),(1.,1.),(1.,
1.),(1.,1.),(1.,1.),(1.,1.),(1.,1.),(1.,1.),(1.,1.),(1.,1.),(1.,1.),(1.,
1.),(1.,1.),(1.,1.),(1.,1.),(1.,1.),(1.,1.),(1.,1.),(1.,1.),(1.,1.),(1.,
1.),(1.,1.),(1.,1.),(1.,1.),(1.,1.),(1.,1.),(1.,1.),(1.,1.),(1.,1.),(1.,
1.),(1.,1.),(1.,1.),(1.,1.),(1.,1.),(1.,1.),(1.,1.),(1.,1.),(1.,1.),(1.,
1.),(1.,1.),(1.,1.),(1.,1.),(1.,1.),(1.,1.),(1.,1.),(1.,1.),(1.,1.),(1.,
1.),(1.,1.)))
REPRESENTATION_ITEM('')
SURFACE()
);
#109=(
BOUNDED_SURFACE()
B_SPLINE_SURFACE(5,1,((#57452,#57453),(#57454,#57455),(#57456,#57457),(#57458,
#57459),(#57460,#57461),(#57462,#57463),(#57464,#57465),(#57466,#57467),
(#57468,#57469),(#57470,#57471),(#57472,#57473),(#57474,#57475),(#57476,
#57477),(#57478,#57479),(#57480,#57481),(#57482,#57483),(#57484,#57485),
(#57486,#57487),(#57488,#57489),(#57490,#57491),(#57492,#57493),(#57494,
#57495),(#57496,#57497),(#57498,#57499),(#57500,#57501),(#57502,#57503),
(#57504,#57505),(#57506,#57507),(#57508,#57509),(#57510,#57511),(#57512,
#57513),(#57514,#57515),(#57516,#57517),(#57518,#57519),(#57520,#57521),
(#57522,#57523),(#57524,#57525),(#57526,#57527),(#57528,#57529),(#57530,
#57531),(#57532,#57533),(#57534,#57535),(#57536,#57537),(#57538,#57539),
(#57540,#57541),(#57542,#57543),(#57544,#57545),(#57546,#57547),(#57548,
#57549),(#57550,#57551),(#57552,#57553),(#57554,#57555),(#57556,#57557),
(#57558,#57559),(#57560,#57561),(#57562,#57563),(#57564,#57565),(#57566,
#57567),(#57568,#57569),(#57570,#57571),(#57572,#57573),(#57574,#57575),
(#57576,#57577),(#57578,#57579),(#57580,#57581),(#57582,#57583),(#57584,
#57585),(#57586,#57587),(#57588,#57589),(#57590,#57591)),.UNSPECIFIED.,
 .F.,.F.,.F.)
B_SPLINE_SURFACE_WITH_KNOTS((6,1,1,1,1,1,1,1,1,1,1,1,1,1,1,1,1,1,1,1,1,
1,1,1,1,1,1,1,1,1,1,1,1,1,1,1,1,1,1,1,1,1,1,1,1,1,1,1,1,1,1,1,1,1,1,1,1,
1,1,1,1,1,1,1,1,6),(2,2),(-1.,-0.984615384615383,-0.969230769230768,-0.953846153846152,
-0.938461538461537,-0.923076923076922,-0.907692307692306,-0.892307692307691,
-0.876923076923076,-0.86153846153846,-0.846153846153845,-0.83076923076923,
-0.815384615384614,-0.799999999999999,-0.784615384615384,-0.769230769230768,
-0.753846153846153,-0.738461538461538,-0.723076923076922,-0.707692307692307,
-0.692307692307692,-0.676923076923076,-0.661538461538461,-0.646153846153846,
-0.63076923076923,-0.615384615384615,-0.6,-0.584615384615384,-0.569230769230769,
-0.553846153846154,-0.538461538461538,-0.523076923076923,-0.507692307692308,
-0.492307692307692,-0.476923076923077,-0.461538461538462,-0.446153846153846,
-0.430769230769231,-0.415384615384615,-0.4,-0.384615384615385,-0.369230769230769,
-0.353846153846154,-0.338461538461538,-0.323076923076923,-0.307692307692308,
-0.292307692307692,-0.276923076923077,-0.261538461538462,-0.246153846153846,
-0.230769230769231,-0.215384615384615,-0.2,-0.184615384615385,-0.169230769230769,
-0.153846153846154,-0.138461538461538,-0.123076923076923,-0.107692307692308,
-0.0923076923076923,-0.0769230769230769,-0.0615384615384615,-0.0461538461538462,
-0.0307692307692308,-0.0153846153846154,0.),(-1.,1.),.UNSPECIFIED.)
GEOMETRIC_REPRESENTATION_ITEM()
RATIONAL_B_SPLINE_SURFACE(((1.,1.),(1.,1.),(1.,1.),(1.,1.),(1.,1.),(1.,
1.),(1.,1.),(1.,1.),(1.,1.),(1.,1.),(1.,1.),(1.,1.),(1.,1.),(1.,1.),(1.,
1.),(1.,1.),(1.,1.),(1.,1.),(1.,1.),(1.,1.),(1.,1.),(1.,1.),(1.,1.),(1.,
1.),(1.,1.),(1.,1.),(1.,1.),(1.,1.),(1.,1.),(1.,1.),(1.,1.),(1.,1.),(1.,
1.),(1.,1.),(1.,1.),(1.,1.),(1.,1.),(1.,1.),(1.,1.),(1.,1.),(1.,1.),(1.,
1.),(1.,1.),(1.,1.),(1.,1.),(1.,1.),(1.,1.),(1.,1.),(1.,1.),(1.,1.),(1.,
1.),(1.,1.),(1.,1.),(1.,1.),(1.,1.),(1.,1.),(1.,1.),(1.,1.),(1.,1.),(1.,
1.),(1.,1.),(1.,1.),(1.,1.),(1.,1.),(1.,1.),(1.,1.),(1.,1.),(1.,1.),(1.,
1.),(1.,1.)))
REPRESENTATION_ITEM('')
SURFACE()
);
#110=(
BOUNDED_SURFACE()
B_SPLINE_SURFACE(5,1,((#57664,#57665),(#57666,#57667),(#57668,#57669),(#57670,
#57671),(#57672,#57673),(#57674,#57675),(#57676,#57677),(#57678,#57679),
(#57680,#57681),(#57682,#57683),(#57684,#57685),(#57686,#57687),(#57688,
#57689),(#57690,#57691),(#57692,#57693),(#57694,#57695),(#57696,#57697),
(#57698,#57699),(#57700,#57701),(#57702,#57703),(#57704,#57705),(#57706,
#57707),(#57708,#57709),(#57710,#57711),(#57712,#57713),(#57714,#57715),
(#57716,#57717),(#57718,#57719),(#57720,#57721),(#57722,#57723),(#57724,
#57725),(#57726,#57727),(#57728,#57729),(#57730,#57731),(#57732,#57733),
(#57734,#57735),(#57736,#57737),(#57738,#57739),(#57740,#57741),(#57742,
#57743),(#57744,#57745),(#57746,#57747),(#57748,#57749),(#57750,#57751),
(#57752,#57753),(#57754,#57755),(#57756,#57757),(#57758,#57759),(#57760,
#57761),(#57762,#57763),(#57764,#57765),(#57766,#57767),(#57768,#57769),
(#57770,#57771),(#57772,#57773),(#57774,#57775),(#57776,#57777),(#57778,
#57779),(#57780,#57781),(#57782,#57783),(#57784,#57785),(#57786,#57787),
(#57788,#57789),(#57790,#57791),(#57792,#57793),(#57794,#57795),(#57796,
#57797),(#57798,#57799),(#57800,#57801),(#57802,#57803)),.UNSPECIFIED.,
 .F.,.F.,.F.)
B_SPLINE_SURFACE_WITH_KNOTS((6,1,1,1,1,1,1,1,1,1,1,1,1,1,1,1,1,1,1,1,1,
1,1,1,1,1,1,1,1,1,1,1,1,1,1,1,1,1,1,1,1,1,1,1,1,1,1,1,1,1,1,1,1,1,1,1,1,
1,1,1,1,1,1,1,1,6),(2,2),(-1.,-0.984615384615383,-0.969230769230768,-0.953846153846152,
-0.938461538461537,-0.923076923076922,-0.907692307692306,-0.892307692307691,
-0.876923076923076,-0.86153846153846,-0.846153846153845,-0.83076923076923,
-0.815384615384614,-0.799999999999999,-0.784615384615384,-0.769230769230768,
-0.753846153846153,-0.738461538461538,-0.723076923076922,-0.707692307692307,
-0.692307692307692,-0.676923076923076,-0.661538461538461,-0.646153846153846,
-0.63076923076923,-0.615384615384615,-0.6,-0.584615384615384,-0.569230769230769,
-0.553846153846154,-0.538461538461538,-0.523076923076923,-0.507692307692308,
-0.492307692307692,-0.476923076923077,-0.461538461538462,-0.446153846153846,
-0.430769230769231,-0.415384615384615,-0.4,-0.384615384615385,-0.369230769230769,
-0.353846153846154,-0.338461538461538,-0.323076923076923,-0.307692307692308,
-0.292307692307692,-0.276923076923077,-0.261538461538462,-0.246153846153846,
-0.230769230769231,-0.215384615384615,-0.2,-0.184615384615385,-0.169230769230769,
-0.153846153846154,-0.138461538461538,-0.123076923076923,-0.107692307692308,
-0.0923076923076923,-0.0769230769230769,-0.0615384615384615,-0.0461538461538462,
-0.0307692307692308,-0.0153846153846154,0.),(-1.,1.),.UNSPECIFIED.)
GEOMETRIC_REPRESENTATION_ITEM()
RATIONAL_B_SPLINE_SURFACE(((1.,1.),(1.,1.),(1.,1.),(1.,1.),(1.,1.),(1.,
1.),(1.,1.),(1.,1.),(1.,1.),(1.,1.),(1.,1.),(1.,1.),(1.,1.),(1.,1.),(1.,
1.),(1.,1.),(1.,1.),(1.,1.),(1.,1.),(1.,1.),(1.,1.),(1.,1.),(1.,1.),(1.,
1.),(1.,1.),(1.,1.),(1.,1.),(1.,1.),(1.,1.),(1.,1.),(1.,1.),(1.,1.),(1.,
1.),(1.,1.),(1.,1.),(1.,1.),(1.,1.),(1.,1.),(1.,1.),(1.,1.),(1.,1.),(1.,
1.),(1.,1.),(1.,1.),(1.,1.),(1.,1.),(1.,1.),(1.,1.),(1.,1.),(1.,1.),(1.,
1.),(1.,1.),(1.,1.),(1.,1.),(1.,1.),(1.,1.),(1.,1.),(1.,1.),(1.,1.),(1.,
1.),(1.,1.),(1.,1.),(1.,1.),(1.,1.),(1.,1.),(1.,1.),(1.,1.),(1.,1.),(1.,
1.),(1.,1.)))
REPRESENTATION_ITEM('')
SURFACE()
);
#111=(
BOUNDED_SURFACE()
B_SPLINE_SURFACE(5,1,((#57894,#57895),(#57896,#57897),(#57898,#57899),(#57900,
#57901),(#57902,#57903),(#57904,#57905),(#57906,#57907),(#57908,#57909),
(#57910,#57911),(#57912,#57913),(#57914,#57915),(#57916,#57917),(#57918,
#57919),(#57920,#57921),(#57922,#57923),(#57924,#57925),(#57926,#57927),
(#57928,#57929),(#57930,#57931),(#57932,#57933),(#57934,#57935),(#57936,
#57937),(#57938,#57939),(#57940,#57941),(#57942,#57943),(#57944,#57945),
(#57946,#57947),(#57948,#57949),(#57950,#57951),(#57952,#57953),(#57954,
#57955),(#57956,#57957),(#57958,#57959),(#57960,#57961),(#57962,#57963),
(#57964,#57965),(#57966,#57967),(#57968,#57969),(#57970,#57971),(#57972,
#57973),(#57974,#57975),(#57976,#57977),(#57978,#57979),(#57980,#57981),
(#57982,#57983),(#57984,#57985),(#57986,#57987),(#57988,#57989),(#57990,
#57991),(#57992,#57993),(#57994,#57995),(#57996,#57997),(#57998,#57999),
(#58000,#58001),(#58002,#58003),(#58004,#58005),(#58006,#58007),(#58008,
#58009),(#58010,#58011),(#58012,#58013),(#58014,#58015),(#58016,#58017),
(#58018,#58019),(#58020,#58021),(#58022,#58023),(#58024,#58025),(#58026,
#58027),(#58028,#58029),(#58030,#58031),(#58032,#58033)),.UNSPECIFIED.,
 .F.,.F.,.F.)
B_SPLINE_SURFACE_WITH_KNOTS((6,1,1,1,1,1,1,1,1,1,1,1,1,1,1,1,1,1,1,1,1,
1,1,1,1,1,1,1,1,1,1,1,1,1,1,1,1,1,1,1,1,1,1,1,1,1,1,1,1,1,1,1,1,1,1,1,1,
1,1,1,1,1,1,1,1,6),(2,2),(-1.,-0.984615384615383,-0.969230769230768,-0.953846153846152,
-0.938461538461537,-0.923076923076922,-0.907692307692306,-0.892307692307691,
-0.876923076923076,-0.86153846153846,-0.846153846153845,-0.83076923076923,
-0.815384615384614,-0.799999999999999,-0.784615384615384,-0.769230769230768,
-0.753846153846153,-0.738461538461538,-0.723076923076922,-0.707692307692307,
-0.692307692307692,-0.676923076923076,-0.661538461538461,-0.646153846153846,
-0.63076923076923,-0.615384615384615,-0.6,-0.584615384615384,-0.569230769230769,
-0.553846153846154,-0.538461538461538,-0.523076923076923,-0.507692307692308,
-0.492307692307692,-0.476923076923077,-0.461538461538462,-0.446153846153846,
-0.430769230769231,-0.415384615384615,-0.4,-0.384615384615385,-0.369230769230769,
-0.353846153846154,-0.338461538461538,-0.323076923076923,-0.307692307692308,
-0.292307692307692,-0.276923076923077,-0.261538461538462,-0.246153846153846,
-0.230769230769231,-0.215384615384615,-0.2,-0.184615384615385,-0.169230769230769,
-0.153846153846154,-0.138461538461538,-0.123076923076923,-0.107692307692308,
-0.0923076923076923,-0.0769230769230769,-0.0615384615384615,-0.0461538461538462,
-0.0307692307692308,-0.0153846153846154,0.),(-1.,1.),.UNSPECIFIED.)
GEOMETRIC_REPRESENTATION_ITEM()
RATIONAL_B_SPLINE_SURFACE(((1.,1.),(1.,1.),(1.,1.),(1.,1.),(1.,1.),(1.,
1.),(1.,1.),(1.,1.),(1.,1.),(1.,1.),(1.,1.),(1.,1.),(1.,1.),(1.,1.),(1.,
1.),(1.,1.),(1.,1.),(1.,1.),(1.,1.),(1.,1.),(1.,1.),(1.,1.),(1.,1.),(1.,
1.),(1.,1.),(1.,1.),(1.,1.),(1.,1.),(1.,1.),(1.,1.),(1.,1.),(1.,1.),(1.,
1.),(1.,1.),(1.,1.),(1.,1.),(1.,1.),(1.,1.),(1.,1.),(1.,1.),(1.,1.),(1.,
1.),(1.,1.),(1.,1.),(1.,1.),(1.,1.),(1.,1.),(1.,1.),(1.,1.),(1.,1.),(1.,
1.),(1.,1.),(1.,1.),(1.,1.),(1.,1.),(1.,1.),(1.,1.),(1.,1.),(1.,1.),(1.,
1.),(1.,1.),(1.,1.),(1.,1.),(1.,1.),(1.,1.),(1.,1.),(1.,1.),(1.,1.),(1.,
1.),(1.,1.)))
REPRESENTATION_ITEM('')
SURFACE()
);
#112=(
BOUNDED_SURFACE()
B_SPLINE_SURFACE(5,1,((#58106,#58107),(#58108,#58109),(#58110,#58111),(#58112,
#58113),(#58114,#58115),(#58116,#58117),(#58118,#58119),(#58120,#58121),
(#58122,#58123),(#58124,#58125),(#58126,#58127),(#58128,#58129),(#58130,
#58131),(#58132,#58133),(#58134,#58135),(#58136,#58137),(#58138,#58139),
(#58140,#58141),(#58142,#58143),(#58144,#58145),(#58146,#58147),(#58148,
#58149),(#58150,#58151),(#58152,#58153),(#58154,#58155),(#58156,#58157),
(#58158,#58159),(#58160,#58161),(#58162,#58163),(#58164,#58165),(#58166,
#58167),(#58168,#58169),(#58170,#58171),(#58172,#58173),(#58174,#58175),
(#58176,#58177),(#58178,#58179),(#58180,#58181),(#58182,#58183),(#58184,
#58185),(#58186,#58187),(#58188,#58189),(#58190,#58191),(#58192,#58193),
(#58194,#58195),(#58196,#58197),(#58198,#58199),(#58200,#58201),(#58202,
#58203),(#58204,#58205),(#58206,#58207),(#58208,#58209),(#58210,#58211),
(#58212,#58213),(#58214,#58215),(#58216,#58217),(#58218,#58219),(#58220,
#58221),(#58222,#58223),(#58224,#58225),(#58226,#58227),(#58228,#58229),
(#58230,#58231),(#58232,#58233),(#58234,#58235),(#58236,#58237),(#58238,
#58239),(#58240,#58241),(#58242,#58243),(#58244,#58245)),.UNSPECIFIED.,
 .F.,.F.,.F.)
B_SPLINE_SURFACE_WITH_KNOTS((6,1,1,1,1,1,1,1,1,1,1,1,1,1,1,1,1,1,1,1,1,
1,1,1,1,1,1,1,1,1,1,1,1,1,1,1,1,1,1,1,1,1,1,1,1,1,1,1,1,1,1,1,1,1,1,1,1,
1,1,1,1,1,1,1,1,6),(2,2),(-1.,-0.984615384615383,-0.969230769230768,-0.953846153846152,
-0.938461538461537,-0.923076923076922,-0.907692307692306,-0.892307692307691,
-0.876923076923076,-0.86153846153846,-0.846153846153845,-0.83076923076923,
-0.815384615384614,-0.799999999999999,-0.784615384615384,-0.769230769230768,
-0.753846153846153,-0.738461538461538,-0.723076923076922,-0.707692307692307,
-0.692307692307692,-0.676923076923076,-0.661538461538461,-0.646153846153846,
-0.63076923076923,-0.615384615384615,-0.6,-0.584615384615384,-0.569230769230769,
-0.553846153846154,-0.538461538461538,-0.523076923076923,-0.507692307692308,
-0.492307692307692,-0.476923076923077,-0.461538461538462,-0.446153846153846,
-0.430769230769231,-0.415384615384615,-0.4,-0.384615384615385,-0.369230769230769,
-0.353846153846154,-0.338461538461538,-0.323076923076923,-0.307692307692308,
-0.292307692307692,-0.276923076923077,-0.261538461538462,-0.246153846153846,
-0.230769230769231,-0.215384615384615,-0.2,-0.184615384615385,-0.169230769230769,
-0.153846153846154,-0.138461538461538,-0.123076923076923,-0.107692307692308,
-0.0923076923076923,-0.0769230769230769,-0.0615384615384615,-0.0461538461538462,
-0.0307692307692308,-0.0153846153846154,0.),(-1.,1.),.UNSPECIFIED.)
GEOMETRIC_REPRESENTATION_ITEM()
RATIONAL_B_SPLINE_SURFACE(((1.,1.),(1.,1.),(1.,1.),(1.,1.),(1.,1.),(1.,
1.),(1.,1.),(1.,1.),(1.,1.),(1.,1.),(1.,1.),(1.,1.),(1.,1.),(1.,1.),(1.,
1.),(1.,1.),(1.,1.),(1.,1.),(1.,1.),(1.,1.),(1.,1.),(1.,1.),(1.,1.),(1.,
1.),(1.,1.),(1.,1.),(1.,1.),(1.,1.),(1.,1.),(1.,1.),(1.,1.),(1.,1.),(1.,
1.),(1.,1.),(1.,1.),(1.,1.),(1.,1.),(1.,1.),(1.,1.),(1.,1.),(1.,1.),(1.,
1.),(1.,1.),(1.,1.),(1.,1.),(1.,1.),(1.,1.),(1.,1.),(1.,1.),(1.,1.),(1.,
1.),(1.,1.),(1.,1.),(1.,1.),(1.,1.),(1.,1.),(1.,1.),(1.,1.),(1.,1.),(1.,
1.),(1.,1.),(1.,1.),(1.,1.),(1.,1.),(1.,1.),(1.,1.),(1.,1.),(1.,1.),(1.,
1.),(1.,1.)))
REPRESENTATION_ITEM('')
SURFACE()
);
#113=(
BOUNDED_SURFACE()
B_SPLINE_SURFACE(5,1,((#58336,#58337),(#58338,#58339),(#58340,#58341),(#58342,
#58343),(#58344,#58345),(#58346,#58347),(#58348,#58349),(#58350,#58351),
(#58352,#58353),(#58354,#58355),(#58356,#58357),(#58358,#58359),(#58360,
#58361),(#58362,#58363),(#58364,#58365),(#58366,#58367),(#58368,#58369),
(#58370,#58371),(#58372,#58373),(#58374,#58375),(#58376,#58377),(#58378,
#58379),(#58380,#58381),(#58382,#58383),(#58384,#58385),(#58386,#58387),
(#58388,#58389),(#58390,#58391),(#58392,#58393),(#58394,#58395),(#58396,
#58397),(#58398,#58399),(#58400,#58401),(#58402,#58403),(#58404,#58405),
(#58406,#58407),(#58408,#58409),(#58410,#58411),(#58412,#58413),(#58414,
#58415),(#58416,#58417),(#58418,#58419),(#58420,#58421),(#58422,#58423),
(#58424,#58425),(#58426,#58427),(#58428,#58429),(#58430,#58431),(#58432,
#58433),(#58434,#58435),(#58436,#58437),(#58438,#58439),(#58440,#58441),
(#58442,#58443),(#58444,#58445),(#58446,#58447),(#58448,#58449),(#58450,
#58451),(#58452,#58453),(#58454,#58455),(#58456,#58457),(#58458,#58459),
(#58460,#58461),(#58462,#58463),(#58464,#58465),(#58466,#58467),(#58468,
#58469),(#58470,#58471),(#58472,#58473),(#58474,#58475)),.UNSPECIFIED.,
 .F.,.F.,.F.)
B_SPLINE_SURFACE_WITH_KNOTS((6,1,1,1,1,1,1,1,1,1,1,1,1,1,1,1,1,1,1,1,1,
1,1,1,1,1,1,1,1,1,1,1,1,1,1,1,1,1,1,1,1,1,1,1,1,1,1,1,1,1,1,1,1,1,1,1,1,
1,1,1,1,1,1,1,1,6),(2,2),(-1.,-0.984615384615383,-0.969230769230768,-0.953846153846152,
-0.938461538461537,-0.923076923076922,-0.907692307692306,-0.892307692307691,
-0.876923076923076,-0.86153846153846,-0.846153846153845,-0.83076923076923,
-0.815384615384614,-0.799999999999999,-0.784615384615384,-0.769230769230768,
-0.753846153846153,-0.738461538461538,-0.723076923076922,-0.707692307692307,
-0.692307692307692,-0.676923076923076,-0.661538461538461,-0.646153846153846,
-0.63076923076923,-0.615384615384615,-0.6,-0.584615384615384,-0.569230769230769,
-0.553846153846154,-0.538461538461538,-0.523076923076923,-0.507692307692308,
-0.492307692307692,-0.476923076923077,-0.461538461538462,-0.446153846153846,
-0.430769230769231,-0.415384615384615,-0.4,-0.384615384615385,-0.369230769230769,
-0.353846153846154,-0.338461538461538,-0.323076923076923,-0.307692307692308,
-0.292307692307692,-0.276923076923077,-0.261538461538462,-0.246153846153846,
-0.230769230769231,-0.215384615384615,-0.2,-0.184615384615385,-0.169230769230769,
-0.153846153846154,-0.138461538461538,-0.123076923076923,-0.107692307692308,
-0.0923076923076923,-0.0769230769230769,-0.0615384615384615,-0.0461538461538462,
-0.0307692307692308,-0.0153846153846154,0.),(-1.,1.),.UNSPECIFIED.)
GEOMETRIC_REPRESENTATION_ITEM()
RATIONAL_B_SPLINE_SURFACE(((1.,1.),(1.,1.),(1.,1.),(1.,1.),(1.,1.),(1.,
1.),(1.,1.),(1.,1.),(1.,1.),(1.,1.),(1.,1.),(1.,1.),(1.,1.),(1.,1.),(1.,
1.),(1.,1.),(1.,1.),(1.,1.),(1.,1.),(1.,1.),(1.,1.),(1.,1.),(1.,1.),(1.,
1.),(1.,1.),(1.,1.),(1.,1.),(1.,1.),(1.,1.),(1.,1.),(1.,1.),(1.,1.),(1.,
1.),(1.,1.),(1.,1.),(1.,1.),(1.,1.),(1.,1.),(1.,1.),(1.,1.),(1.,1.),(1.,
1.),(1.,1.),(1.,1.),(1.,1.),(1.,1.),(1.,1.),(1.,1.),(1.,1.),(1.,1.),(1.,
1.),(1.,1.),(1.,1.),(1.,1.),(1.,1.),(1.,1.),(1.,1.),(1.,1.),(1.,1.),(1.,
1.),(1.,1.),(1.,1.),(1.,1.),(1.,1.),(1.,1.),(1.,1.),(1.,1.),(1.,1.),(1.,
1.),(1.,1.)))
REPRESENTATION_ITEM('')
SURFACE()
);
#114=(
BOUNDED_SURFACE()
B_SPLINE_SURFACE(5,1,((#58548,#58549),(#58550,#58551),(#58552,#58553),(#58554,
#58555),(#58556,#58557),(#58558,#58559),(#58560,#58561),(#58562,#58563),
(#58564,#58565),(#58566,#58567),(#58568,#58569),(#58570,#58571),(#58572,
#58573),(#58574,#58575),(#58576,#58577),(#58578,#58579),(#58580,#58581),
(#58582,#58583),(#58584,#58585),(#58586,#58587),(#58588,#58589),(#58590,
#58591),(#58592,#58593),(#58594,#58595),(#58596,#58597),(#58598,#58599),
(#58600,#58601),(#58602,#58603),(#58604,#58605),(#58606,#58607),(#58608,
#58609),(#58610,#58611),(#58612,#58613),(#58614,#58615),(#58616,#58617),
(#58618,#58619),(#58620,#58621),(#58622,#58623),(#58624,#58625),(#58626,
#58627),(#58628,#58629),(#58630,#58631),(#58632,#58633),(#58634,#58635),
(#58636,#58637),(#58638,#58639),(#58640,#58641),(#58642,#58643),(#58644,
#58645),(#58646,#58647),(#58648,#58649),(#58650,#58651),(#58652,#58653),
(#58654,#58655),(#58656,#58657),(#58658,#58659),(#58660,#58661),(#58662,
#58663),(#58664,#58665),(#58666,#58667),(#58668,#58669),(#58670,#58671),
(#58672,#58673),(#58674,#58675),(#58676,#58677),(#58678,#58679),(#58680,
#58681),(#58682,#58683),(#58684,#58685),(#58686,#58687)),.UNSPECIFIED.,
 .F.,.F.,.F.)
B_SPLINE_SURFACE_WITH_KNOTS((6,1,1,1,1,1,1,1,1,1,1,1,1,1,1,1,1,1,1,1,1,
1,1,1,1,1,1,1,1,1,1,1,1,1,1,1,1,1,1,1,1,1,1,1,1,1,1,1,1,1,1,1,1,1,1,1,1,
1,1,1,1,1,1,1,1,6),(2,2),(-1.,-0.984615384615383,-0.969230769230768,-0.953846153846152,
-0.938461538461537,-0.923076923076922,-0.907692307692306,-0.892307692307691,
-0.876923076923076,-0.86153846153846,-0.846153846153845,-0.83076923076923,
-0.815384615384614,-0.799999999999999,-0.784615384615384,-0.769230769230768,
-0.753846153846153,-0.738461538461538,-0.723076923076922,-0.707692307692307,
-0.692307692307692,-0.676923076923076,-0.661538461538461,-0.646153846153846,
-0.63076923076923,-0.615384615384615,-0.6,-0.584615384615384,-0.569230769230769,
-0.553846153846154,-0.538461538461538,-0.523076923076923,-0.507692307692308,
-0.492307692307692,-0.476923076923077,-0.461538461538462,-0.446153846153846,
-0.430769230769231,-0.415384615384615,-0.4,-0.384615384615385,-0.369230769230769,
-0.353846153846154,-0.338461538461538,-0.323076923076923,-0.307692307692308,
-0.292307692307692,-0.276923076923077,-0.261538461538462,-0.246153846153846,
-0.230769230769231,-0.215384615384615,-0.2,-0.184615384615385,-0.169230769230769,
-0.153846153846154,-0.138461538461538,-0.123076923076923,-0.107692307692308,
-0.0923076923076923,-0.0769230769230769,-0.0615384615384615,-0.0461538461538462,
-0.0307692307692308,-0.0153846153846154,0.),(-1.,1.),.UNSPECIFIED.)
GEOMETRIC_REPRESENTATION_ITEM()
RATIONAL_B_SPLINE_SURFACE(((1.,1.),(1.,1.),(1.,1.),(1.,1.),(1.,1.),(1.,
1.),(1.,1.),(1.,1.),(1.,1.),(1.,1.),(1.,1.),(1.,1.),(1.,1.),(1.,1.),(1.,
1.),(1.,1.),(1.,1.),(1.,1.),(1.,1.),(1.,1.),(1.,1.),(1.,1.),(1.,1.),(1.,
1.),(1.,1.),(1.,1.),(1.,1.),(1.,1.),(1.,1.),(1.,1.),(1.,1.),(1.,1.),(1.,
1.),(1.,1.),(1.,1.),(1.,1.),(1.,1.),(1.,1.),(1.,1.),(1.,1.),(1.,1.),(1.,
1.),(1.,1.),(1.,1.),(1.,1.),(1.,1.),(1.,1.),(1.,1.),(1.,1.),(1.,1.),(1.,
1.),(1.,1.),(1.,1.),(1.,1.),(1.,1.),(1.,1.),(1.,1.),(1.,1.),(1.,1.),(1.,
1.),(1.,1.),(1.,1.),(1.,1.),(1.,1.),(1.,1.),(1.,1.),(1.,1.),(1.,1.),(1.,
1.),(1.,1.)))
REPRESENTATION_ITEM('')
SURFACE()
);
#115=(
BOUNDED_SURFACE()
B_SPLINE_SURFACE(5,1,((#58778,#58779),(#58780,#58781),(#58782,#58783),(#58784,
#58785),(#58786,#58787),(#58788,#58789),(#58790,#58791),(#58792,#58793),
(#58794,#58795),(#58796,#58797),(#58798,#58799),(#58800,#58801),(#58802,
#58803),(#58804,#58805),(#58806,#58807),(#58808,#58809),(#58810,#58811),
(#58812,#58813),(#58814,#58815),(#58816,#58817),(#58818,#58819),(#58820,
#58821),(#58822,#58823),(#58824,#58825),(#58826,#58827),(#58828,#58829),
(#58830,#58831),(#58832,#58833),(#58834,#58835),(#58836,#58837),(#58838,
#58839),(#58840,#58841),(#58842,#58843),(#58844,#58845),(#58846,#58847),
(#58848,#58849),(#58850,#58851),(#58852,#58853),(#58854,#58855),(#58856,
#58857),(#58858,#58859),(#58860,#58861),(#58862,#58863),(#58864,#58865),
(#58866,#58867),(#58868,#58869),(#58870,#58871),(#58872,#58873),(#58874,
#58875),(#58876,#58877),(#58878,#58879),(#58880,#58881),(#58882,#58883),
(#58884,#58885),(#58886,#58887),(#58888,#58889),(#58890,#58891),(#58892,
#58893),(#58894,#58895),(#58896,#58897),(#58898,#58899),(#58900,#58901),
(#58902,#58903),(#58904,#58905),(#58906,#58907),(#58908,#58909),(#58910,
#58911),(#58912,#58913),(#58914,#58915),(#58916,#58917)),.UNSPECIFIED.,
 .F.,.F.,.F.)
B_SPLINE_SURFACE_WITH_KNOTS((6,1,1,1,1,1,1,1,1,1,1,1,1,1,1,1,1,1,1,1,1,
1,1,1,1,1,1,1,1,1,1,1,1,1,1,1,1,1,1,1,1,1,1,1,1,1,1,1,1,1,1,1,1,1,1,1,1,
1,1,1,1,1,1,1,1,6),(2,2),(-1.,-0.984615384615383,-0.969230769230768,-0.953846153846152,
-0.938461538461537,-0.923076923076922,-0.907692307692306,-0.892307692307691,
-0.876923076923076,-0.86153846153846,-0.846153846153845,-0.83076923076923,
-0.815384615384614,-0.799999999999999,-0.784615384615384,-0.769230769230768,
-0.753846153846153,-0.738461538461538,-0.723076923076922,-0.707692307692307,
-0.692307692307692,-0.676923076923076,-0.661538461538461,-0.646153846153846,
-0.63076923076923,-0.615384615384615,-0.6,-0.584615384615384,-0.569230769230769,
-0.553846153846154,-0.538461538461538,-0.523076923076923,-0.507692307692308,
-0.492307692307692,-0.476923076923077,-0.461538461538462,-0.446153846153846,
-0.430769230769231,-0.415384615384615,-0.4,-0.384615384615385,-0.369230769230769,
-0.353846153846154,-0.338461538461538,-0.323076923076923,-0.307692307692308,
-0.292307692307692,-0.276923076923077,-0.261538461538462,-0.246153846153846,
-0.230769230769231,-0.215384615384615,-0.2,-0.184615384615385,-0.169230769230769,
-0.153846153846154,-0.138461538461538,-0.123076923076923,-0.107692307692308,
-0.0923076923076923,-0.0769230769230769,-0.0615384615384615,-0.0461538461538462,
-0.0307692307692308,-0.0153846153846154,0.),(-1.,1.),.UNSPECIFIED.)
GEOMETRIC_REPRESENTATION_ITEM()
RATIONAL_B_SPLINE_SURFACE(((1.,1.),(1.,1.),(1.,1.),(1.,1.),(1.,1.),(1.,
1.),(1.,1.),(1.,1.),(1.,1.),(1.,1.),(1.,1.),(1.,1.),(1.,1.),(1.,1.),(1.,
1.),(1.,1.),(1.,1.),(1.,1.),(1.,1.),(1.,1.),(1.,1.),(1.,1.),(1.,1.),(1.,
1.),(1.,1.),(1.,1.),(1.,1.),(1.,1.),(1.,1.),(1.,1.),(1.,1.),(1.,1.),(1.,
1.),(1.,1.),(1.,1.),(1.,1.),(1.,1.),(1.,1.),(1.,1.),(1.,1.),(1.,1.),(1.,
1.),(1.,1.),(1.,1.),(1.,1.),(1.,1.),(1.,1.),(1.,1.),(1.,1.),(1.,1.),(1.,
1.),(1.,1.),(1.,1.),(1.,1.),(1.,1.),(1.,1.),(1.,1.),(1.,1.),(1.,1.),(1.,
1.),(1.,1.),(1.,1.),(1.,1.),(1.,1.),(1.,1.),(1.,1.),(1.,1.),(1.,1.),(1.,
1.),(1.,1.)))
REPRESENTATION_ITEM('')
SURFACE()
);
#116=(
BOUNDED_SURFACE()
B_SPLINE_SURFACE(5,1,((#58990,#58991),(#58992,#58993),(#58994,#58995),(#58996,
#58997),(#58998,#58999),(#59000,#59001),(#59002,#59003),(#59004,#59005),
(#59006,#59007),(#59008,#59009),(#59010,#59011),(#59012,#59013),(#59014,
#59015),(#59016,#59017),(#59018,#59019),(#59020,#59021),(#59022,#59023),
(#59024,#59025),(#59026,#59027),(#59028,#59029),(#59030,#59031),(#59032,
#59033),(#59034,#59035),(#59036,#59037),(#59038,#59039),(#59040,#59041),
(#59042,#59043),(#59044,#59045),(#59046,#59047),(#59048,#59049),(#59050,
#59051),(#59052,#59053),(#59054,#59055),(#59056,#59057),(#59058,#59059),
(#59060,#59061),(#59062,#59063),(#59064,#59065),(#59066,#59067),(#59068,
#59069),(#59070,#59071),(#59072,#59073),(#59074,#59075),(#59076,#59077),
(#59078,#59079),(#59080,#59081),(#59082,#59083),(#59084,#59085),(#59086,
#59087),(#59088,#59089),(#59090,#59091),(#59092,#59093),(#59094,#59095),
(#59096,#59097),(#59098,#59099),(#59100,#59101),(#59102,#59103),(#59104,
#59105),(#59106,#59107),(#59108,#59109),(#59110,#59111),(#59112,#59113),
(#59114,#59115),(#59116,#59117),(#59118,#59119),(#59120,#59121),(#59122,
#59123),(#59124,#59125),(#59126,#59127),(#59128,#59129)),.UNSPECIFIED.,
 .F.,.F.,.F.)
B_SPLINE_SURFACE_WITH_KNOTS((6,1,1,1,1,1,1,1,1,1,1,1,1,1,1,1,1,1,1,1,1,
1,1,1,1,1,1,1,1,1,1,1,1,1,1,1,1,1,1,1,1,1,1,1,1,1,1,1,1,1,1,1,1,1,1,1,1,
1,1,1,1,1,1,1,1,6),(2,2),(-1.,-0.984615384615383,-0.969230769230768,-0.953846153846152,
-0.938461538461537,-0.923076923076922,-0.907692307692306,-0.892307692307691,
-0.876923076923076,-0.86153846153846,-0.846153846153845,-0.83076923076923,
-0.815384615384614,-0.799999999999999,-0.784615384615384,-0.769230769230768,
-0.753846153846153,-0.738461538461538,-0.723076923076922,-0.707692307692307,
-0.692307692307692,-0.676923076923076,-0.661538461538461,-0.646153846153846,
-0.63076923076923,-0.615384615384615,-0.6,-0.584615384615384,-0.569230769230769,
-0.553846153846154,-0.538461538461538,-0.523076923076923,-0.507692307692308,
-0.492307692307692,-0.476923076923077,-0.461538461538462,-0.446153846153846,
-0.430769230769231,-0.415384615384615,-0.4,-0.384615384615385,-0.369230769230769,
-0.353846153846154,-0.338461538461538,-0.323076923076923,-0.307692307692308,
-0.292307692307692,-0.276923076923077,-0.261538461538462,-0.246153846153846,
-0.230769230769231,-0.215384615384615,-0.2,-0.184615384615385,-0.169230769230769,
-0.153846153846154,-0.138461538461538,-0.123076923076923,-0.107692307692308,
-0.0923076923076923,-0.0769230769230769,-0.0615384615384615,-0.0461538461538462,
-0.0307692307692308,-0.0153846153846154,0.),(-1.,1.),.UNSPECIFIED.)
GEOMETRIC_REPRESENTATION_ITEM()
RATIONAL_B_SPLINE_SURFACE(((1.,1.),(1.,1.),(1.,1.),(1.,1.),(1.,1.),(1.,
1.),(1.,1.),(1.,1.),(1.,1.),(1.,1.),(1.,1.),(1.,1.),(1.,1.),(1.,1.),(1.,
1.),(1.,1.),(1.,1.),(1.,1.),(1.,1.),(1.,1.),(1.,1.),(1.,1.),(1.,1.),(1.,
1.),(1.,1.),(1.,1.),(1.,1.),(1.,1.),(1.,1.),(1.,1.),(1.,1.),(1.,1.),(1.,
1.),(1.,1.),(1.,1.),(1.,1.),(1.,1.),(1.,1.),(1.,1.),(1.,1.),(1.,1.),(1.,
1.),(1.,1.),(1.,1.),(1.,1.),(1.,1.),(1.,1.),(1.,1.),(1.,1.),(1.,1.),(1.,
1.),(1.,1.),(1.,1.),(1.,1.),(1.,1.),(1.,1.),(1.,1.),(1.,1.),(1.,1.),(1.,
1.),(1.,1.),(1.,1.),(1.,1.),(1.,1.),(1.,1.),(1.,1.),(1.,1.),(1.,1.),(1.,
1.),(1.,1.)))
REPRESENTATION_ITEM('')
SURFACE()
);
#117=(
BOUNDED_SURFACE()
B_SPLINE_SURFACE(5,1,((#59220,#59221),(#59222,#59223),(#59224,#59225),(#59226,
#59227),(#59228,#59229),(#59230,#59231),(#59232,#59233),(#59234,#59235),
(#59236,#59237),(#59238,#59239),(#59240,#59241),(#59242,#59243),(#59244,
#59245),(#59246,#59247),(#59248,#59249),(#59250,#59251),(#59252,#59253),
(#59254,#59255),(#59256,#59257),(#59258,#59259),(#59260,#59261),(#59262,
#59263),(#59264,#59265),(#59266,#59267),(#59268,#59269),(#59270,#59271),
(#59272,#59273),(#59274,#59275),(#59276,#59277),(#59278,#59279),(#59280,
#59281),(#59282,#59283),(#59284,#59285),(#59286,#59287),(#59288,#59289),
(#59290,#59291),(#59292,#59293),(#59294,#59295),(#59296,#59297),(#59298,
#59299),(#59300,#59301),(#59302,#59303),(#59304,#59305),(#59306,#59307),
(#59308,#59309),(#59310,#59311),(#59312,#59313),(#59314,#59315),(#59316,
#59317),(#59318,#59319),(#59320,#59321),(#59322,#59323),(#59324,#59325),
(#59326,#59327),(#59328,#59329),(#59330,#59331),(#59332,#59333),(#59334,
#59335),(#59336,#59337),(#59338,#59339),(#59340,#59341),(#59342,#59343),
(#59344,#59345),(#59346,#59347),(#59348,#59349),(#59350,#59351),(#59352,
#59353),(#59354,#59355),(#59356,#59357),(#59358,#59359)),.UNSPECIFIED.,
 .F.,.F.,.F.)
B_SPLINE_SURFACE_WITH_KNOTS((6,1,1,1,1,1,1,1,1,1,1,1,1,1,1,1,1,1,1,1,1,
1,1,1,1,1,1,1,1,1,1,1,1,1,1,1,1,1,1,1,1,1,1,1,1,1,1,1,1,1,1,1,1,1,1,1,1,
1,1,1,1,1,1,1,1,6),(2,2),(-1.,-0.984615384615383,-0.969230769230768,-0.953846153846152,
-0.938461538461537,-0.923076923076922,-0.907692307692306,-0.892307692307691,
-0.876923076923076,-0.86153846153846,-0.846153846153845,-0.83076923076923,
-0.815384615384614,-0.799999999999999,-0.784615384615384,-0.769230769230768,
-0.753846153846153,-0.738461538461538,-0.723076923076922,-0.707692307692307,
-0.692307692307692,-0.676923076923076,-0.661538461538461,-0.646153846153846,
-0.63076923076923,-0.615384615384615,-0.6,-0.584615384615384,-0.569230769230769,
-0.553846153846154,-0.538461538461538,-0.523076923076923,-0.507692307692308,
-0.492307692307692,-0.476923076923077,-0.461538461538462,-0.446153846153846,
-0.430769230769231,-0.415384615384615,-0.4,-0.384615384615385,-0.369230769230769,
-0.353846153846154,-0.338461538461538,-0.323076923076923,-0.307692307692308,
-0.292307692307692,-0.276923076923077,-0.261538461538462,-0.246153846153846,
-0.230769230769231,-0.215384615384615,-0.2,-0.184615384615385,-0.169230769230769,
-0.153846153846154,-0.138461538461538,-0.123076923076923,-0.107692307692308,
-0.0923076923076923,-0.0769230769230769,-0.0615384615384615,-0.0461538461538462,
-0.0307692307692308,-0.0153846153846154,0.),(-1.,1.),.UNSPECIFIED.)
GEOMETRIC_REPRESENTATION_ITEM()
RATIONAL_B_SPLINE_SURFACE(((1.,1.),(1.,1.),(1.,1.),(1.,1.),(1.,1.),(1.,
1.),(1.,1.),(1.,1.),(1.,1.),(1.,1.),(1.,1.),(1.,1.),(1.,1.),(1.,1.),(1.,
1.),(1.,1.),(1.,1.),(1.,1.),(1.,1.),(1.,1.),(1.,1.),(1.,1.),(1.,1.),(1.,
1.),(1.,1.),(1.,1.),(1.,1.),(1.,1.),(1.,1.),(1.,1.),(1.,1.),(1.,1.),(1.,
1.),(1.,1.),(1.,1.),(1.,1.),(1.,1.),(1.,1.),(1.,1.),(1.,1.),(1.,1.),(1.,
1.),(1.,1.),(1.,1.),(1.,1.),(1.,1.),(1.,1.),(1.,1.),(1.,1.),(1.,1.),(1.,
1.),(1.,1.),(1.,1.),(1.,1.),(1.,1.),(1.,1.),(1.,1.),(1.,1.),(1.,1.),(1.,
1.),(1.,1.),(1.,1.),(1.,1.),(1.,1.),(1.,1.),(1.,1.),(1.,1.),(1.,1.),(1.,
1.),(1.,1.)))
REPRESENTATION_ITEM('')
SURFACE()
);
#118=(
BOUNDED_SURFACE()
B_SPLINE_SURFACE(5,1,((#59432,#59433),(#59434,#59435),(#59436,#59437),(#59438,
#59439),(#59440,#59441),(#59442,#59443),(#59444,#59445),(#59446,#59447),
(#59448,#59449),(#59450,#59451),(#59452,#59453),(#59454,#59455),(#59456,
#59457),(#59458,#59459),(#59460,#59461),(#59462,#59463),(#59464,#59465),
(#59466,#59467),(#59468,#59469),(#59470,#59471),(#59472,#59473),(#59474,
#59475),(#59476,#59477),(#59478,#59479),(#59480,#59481),(#59482,#59483),
(#59484,#59485),(#59486,#59487),(#59488,#59489),(#59490,#59491),(#59492,
#59493),(#59494,#59495),(#59496,#59497),(#59498,#59499),(#59500,#59501),
(#59502,#59503),(#59504,#59505),(#59506,#59507),(#59508,#59509),(#59510,
#59511),(#59512,#59513),(#59514,#59515),(#59516,#59517),(#59518,#59519),
(#59520,#59521),(#59522,#59523),(#59524,#59525),(#59526,#59527),(#59528,
#59529),(#59530,#59531),(#59532,#59533),(#59534,#59535),(#59536,#59537),
(#59538,#59539),(#59540,#59541),(#59542,#59543),(#59544,#59545),(#59546,
#59547),(#59548,#59549),(#59550,#59551),(#59552,#59553),(#59554,#59555),
(#59556,#59557),(#59558,#59559),(#59560,#59561),(#59562,#59563),(#59564,
#59565),(#59566,#59567),(#59568,#59569),(#59570,#59571)),.UNSPECIFIED.,
 .F.,.F.,.F.)
B_SPLINE_SURFACE_WITH_KNOTS((6,1,1,1,1,1,1,1,1,1,1,1,1,1,1,1,1,1,1,1,1,
1,1,1,1,1,1,1,1,1,1,1,1,1,1,1,1,1,1,1,1,1,1,1,1,1,1,1,1,1,1,1,1,1,1,1,1,
1,1,1,1,1,1,1,1,6),(2,2),(-1.,-0.984615384615383,-0.969230769230768,-0.953846153846152,
-0.938461538461537,-0.923076923076922,-0.907692307692306,-0.892307692307691,
-0.876923076923076,-0.86153846153846,-0.846153846153845,-0.83076923076923,
-0.815384615384614,-0.799999999999999,-0.784615384615384,-0.769230769230768,
-0.753846153846153,-0.738461538461538,-0.723076923076922,-0.707692307692307,
-0.692307692307692,-0.676923076923076,-0.661538461538461,-0.646153846153846,
-0.63076923076923,-0.615384615384615,-0.6,-0.584615384615384,-0.569230769230769,
-0.553846153846154,-0.538461538461538,-0.523076923076923,-0.507692307692308,
-0.492307692307692,-0.476923076923077,-0.461538461538462,-0.446153846153846,
-0.430769230769231,-0.415384615384615,-0.4,-0.384615384615385,-0.369230769230769,
-0.353846153846154,-0.338461538461538,-0.323076923076923,-0.307692307692308,
-0.292307692307692,-0.276923076923077,-0.261538461538462,-0.246153846153846,
-0.230769230769231,-0.215384615384615,-0.2,-0.184615384615385,-0.169230769230769,
-0.153846153846154,-0.138461538461538,-0.123076923076923,-0.107692307692308,
-0.0923076923076923,-0.0769230769230769,-0.0615384615384615,-0.0461538461538462,
-0.0307692307692308,-0.0153846153846154,0.),(-1.,1.),.UNSPECIFIED.)
GEOMETRIC_REPRESENTATION_ITEM()
RATIONAL_B_SPLINE_SURFACE(((1.,1.),(1.,1.),(1.,1.),(1.,1.),(1.,1.),(1.,
1.),(1.,1.),(1.,1.),(1.,1.),(1.,1.),(1.,1.),(1.,1.),(1.,1.),(1.,1.),(1.,
1.),(1.,1.),(1.,1.),(1.,1.),(1.,1.),(1.,1.),(1.,1.),(1.,1.),(1.,1.),(1.,
1.),(1.,1.),(1.,1.),(1.,1.),(1.,1.),(1.,1.),(1.,1.),(1.,1.),(1.,1.),(1.,
1.),(1.,1.),(1.,1.),(1.,1.),(1.,1.),(1.,1.),(1.,1.),(1.,1.),(1.,1.),(1.,
1.),(1.,1.),(1.,1.),(1.,1.),(1.,1.),(1.,1.),(1.,1.),(1.,1.),(1.,1.),(1.,
1.),(1.,1.),(1.,1.),(1.,1.),(1.,1.),(1.,1.),(1.,1.),(1.,1.),(1.,1.),(1.,
1.),(1.,1.),(1.,1.),(1.,1.),(1.,1.),(1.,1.),(1.,1.),(1.,1.),(1.,1.),(1.,
1.),(1.,1.)))
REPRESENTATION_ITEM('')
SURFACE()
);
#119=(
BOUNDED_SURFACE()
B_SPLINE_SURFACE(5,1,((#59662,#59663),(#59664,#59665),(#59666,#59667),(#59668,
#59669),(#59670,#59671),(#59672,#59673),(#59674,#59675),(#59676,#59677),
(#59678,#59679),(#59680,#59681),(#59682,#59683),(#59684,#59685),(#59686,
#59687),(#59688,#59689),(#59690,#59691),(#59692,#59693),(#59694,#59695),
(#59696,#59697),(#59698,#59699),(#59700,#59701),(#59702,#59703),(#59704,
#59705),(#59706,#59707),(#59708,#59709),(#59710,#59711),(#59712,#59713),
(#59714,#59715),(#59716,#59717),(#59718,#59719),(#59720,#59721),(#59722,
#59723),(#59724,#59725),(#59726,#59727),(#59728,#59729),(#59730,#59731),
(#59732,#59733),(#59734,#59735),(#59736,#59737),(#59738,#59739),(#59740,
#59741),(#59742,#59743),(#59744,#59745),(#59746,#59747),(#59748,#59749),
(#59750,#59751),(#59752,#59753),(#59754,#59755),(#59756,#59757),(#59758,
#59759),(#59760,#59761),(#59762,#59763),(#59764,#59765),(#59766,#59767),
(#59768,#59769),(#59770,#59771),(#59772,#59773),(#59774,#59775),(#59776,
#59777),(#59778,#59779),(#59780,#59781),(#59782,#59783),(#59784,#59785),
(#59786,#59787),(#59788,#59789),(#59790,#59791),(#59792,#59793),(#59794,
#59795),(#59796,#59797),(#59798,#59799),(#59800,#59801)),.UNSPECIFIED.,
 .F.,.F.,.F.)
B_SPLINE_SURFACE_WITH_KNOTS((6,1,1,1,1,1,1,1,1,1,1,1,1,1,1,1,1,1,1,1,1,
1,1,1,1,1,1,1,1,1,1,1,1,1,1,1,1,1,1,1,1,1,1,1,1,1,1,1,1,1,1,1,1,1,1,1,1,
1,1,1,1,1,1,1,1,6),(2,2),(-1.,-0.984615384615383,-0.969230769230768,-0.953846153846152,
-0.938461538461537,-0.923076923076922,-0.907692307692306,-0.892307692307691,
-0.876923076923076,-0.86153846153846,-0.846153846153845,-0.83076923076923,
-0.815384615384614,-0.799999999999999,-0.784615384615384,-0.769230769230768,
-0.753846153846153,-0.738461538461538,-0.723076923076922,-0.707692307692307,
-0.692307692307692,-0.676923076923076,-0.661538461538461,-0.646153846153846,
-0.63076923076923,-0.615384615384615,-0.6,-0.584615384615384,-0.569230769230769,
-0.553846153846154,-0.538461538461538,-0.523076923076923,-0.507692307692308,
-0.492307692307692,-0.476923076923077,-0.461538461538462,-0.446153846153846,
-0.430769230769231,-0.415384615384615,-0.4,-0.384615384615385,-0.369230769230769,
-0.353846153846154,-0.338461538461538,-0.323076923076923,-0.307692307692308,
-0.292307692307692,-0.276923076923077,-0.261538461538462,-0.246153846153846,
-0.230769230769231,-0.215384615384615,-0.2,-0.184615384615385,-0.169230769230769,
-0.153846153846154,-0.138461538461538,-0.123076923076923,-0.107692307692308,
-0.0923076923076923,-0.0769230769230769,-0.0615384615384615,-0.0461538461538462,
-0.0307692307692308,-0.0153846153846154,0.),(-1.,1.),.UNSPECIFIED.)
GEOMETRIC_REPRESENTATION_ITEM()
RATIONAL_B_SPLINE_SURFACE(((1.,1.),(1.,1.),(1.,1.),(1.,1.),(1.,1.),(1.,
1.),(1.,1.),(1.,1.),(1.,1.),(1.,1.),(1.,1.),(1.,1.),(1.,1.),(1.,1.),(1.,
1.),(1.,1.),(1.,1.),(1.,1.),(1.,1.),(1.,1.),(1.,1.),(1.,1.),(1.,1.),(1.,
1.),(1.,1.),(1.,1.),(1.,1.),(1.,1.),(1.,1.),(1.,1.),(1.,1.),(1.,1.),(1.,
1.),(1.,1.),(1.,1.),(1.,1.),(1.,1.),(1.,1.),(1.,1.),(1.,1.),(1.,1.),(1.,
1.),(1.,1.),(1.,1.),(1.,1.),(1.,1.),(1.,1.),(1.,1.),(1.,1.),(1.,1.),(1.,
1.),(1.,1.),(1.,1.),(1.,1.),(1.,1.),(1.,1.),(1.,1.),(1.,1.),(1.,1.),(1.,
1.),(1.,1.),(1.,1.),(1.,1.),(1.,1.),(1.,1.),(1.,1.),(1.,1.),(1.,1.),(1.,
1.),(1.,1.)))
REPRESENTATION_ITEM('')
SURFACE()
);
#120=(
BOUNDED_SURFACE()
B_SPLINE_SURFACE(5,1,((#59874,#59875),(#59876,#59877),(#59878,#59879),(#59880,
#59881),(#59882,#59883),(#59884,#59885),(#59886,#59887),(#59888,#59889),
(#59890,#59891),(#59892,#59893),(#59894,#59895),(#59896,#59897),(#59898,
#59899),(#59900,#59901),(#59902,#59903),(#59904,#59905),(#59906,#59907),
(#59908,#59909),(#59910,#59911),(#59912,#59913),(#59914,#59915),(#59916,
#59917),(#59918,#59919),(#59920,#59921),(#59922,#59923),(#59924,#59925),
(#59926,#59927),(#59928,#59929),(#59930,#59931),(#59932,#59933),(#59934,
#59935),(#59936,#59937),(#59938,#59939),(#59940,#59941),(#59942,#59943),
(#59944,#59945),(#59946,#59947),(#59948,#59949),(#59950,#59951),(#59952,
#59953),(#59954,#59955),(#59956,#59957),(#59958,#59959),(#59960,#59961),
(#59962,#59963),(#59964,#59965),(#59966,#59967),(#59968,#59969),(#59970,
#59971),(#59972,#59973),(#59974,#59975),(#59976,#59977),(#59978,#59979),
(#59980,#59981),(#59982,#59983),(#59984,#59985),(#59986,#59987),(#59988,
#59989),(#59990,#59991),(#59992,#59993),(#59994,#59995),(#59996,#59997),
(#59998,#59999),(#60000,#60001),(#60002,#60003),(#60004,#60005),(#60006,
#60007),(#60008,#60009),(#60010,#60011),(#60012,#60013)),.UNSPECIFIED.,
 .F.,.F.,.F.)
B_SPLINE_SURFACE_WITH_KNOTS((6,1,1,1,1,1,1,1,1,1,1,1,1,1,1,1,1,1,1,1,1,
1,1,1,1,1,1,1,1,1,1,1,1,1,1,1,1,1,1,1,1,1,1,1,1,1,1,1,1,1,1,1,1,1,1,1,1,
1,1,1,1,1,1,1,1,6),(2,2),(-1.,-0.984615384615383,-0.969230769230768,-0.953846153846152,
-0.938461538461537,-0.923076923076922,-0.907692307692306,-0.892307692307691,
-0.876923076923076,-0.86153846153846,-0.846153846153845,-0.83076923076923,
-0.815384615384614,-0.799999999999999,-0.784615384615384,-0.769230769230768,
-0.753846153846153,-0.738461538461538,-0.723076923076922,-0.707692307692307,
-0.692307692307692,-0.676923076923076,-0.661538461538461,-0.646153846153846,
-0.63076923076923,-0.615384615384615,-0.6,-0.584615384615384,-0.569230769230769,
-0.553846153846154,-0.538461538461538,-0.523076923076923,-0.507692307692308,
-0.492307692307692,-0.476923076923077,-0.461538461538462,-0.446153846153846,
-0.430769230769231,-0.415384615384615,-0.4,-0.384615384615385,-0.369230769230769,
-0.353846153846154,-0.338461538461538,-0.323076923076923,-0.307692307692308,
-0.292307692307692,-0.276923076923077,-0.261538461538462,-0.246153846153846,
-0.230769230769231,-0.215384615384615,-0.2,-0.184615384615385,-0.169230769230769,
-0.153846153846154,-0.138461538461538,-0.123076923076923,-0.107692307692308,
-0.0923076923076923,-0.0769230769230769,-0.0615384615384615,-0.0461538461538462,
-0.0307692307692308,-0.0153846153846154,0.),(-1.,1.),.UNSPECIFIED.)
GEOMETRIC_REPRESENTATION_ITEM()
RATIONAL_B_SPLINE_SURFACE(((1.,1.),(1.,1.),(1.,1.),(1.,1.),(1.,1.),(1.,
1.),(1.,1.),(1.,1.),(1.,1.),(1.,1.),(1.,1.),(1.,1.),(1.,1.),(1.,1.),(1.,
1.),(1.,1.),(1.,1.),(1.,1.),(1.,1.),(1.,1.),(1.,1.),(1.,1.),(1.,1.),(1.,
1.),(1.,1.),(1.,1.),(1.,1.),(1.,1.),(1.,1.),(1.,1.),(1.,1.),(1.,1.),(1.,
1.),(1.,1.),(1.,1.),(1.,1.),(1.,1.),(1.,1.),(1.,1.),(1.,1.),(1.,1.),(1.,
1.),(1.,1.),(1.,1.),(1.,1.),(1.,1.),(1.,1.),(1.,1.),(1.,1.),(1.,1.),(1.,
1.),(1.,1.),(1.,1.),(1.,1.),(1.,1.),(1.,1.),(1.,1.),(1.,1.),(1.,1.),(1.,
1.),(1.,1.),(1.,1.),(1.,1.),(1.,1.),(1.,1.),(1.,1.),(1.,1.),(1.,1.),(1.,
1.),(1.,1.)))
REPRESENTATION_ITEM('')
SURFACE()
);
#121=(
BOUNDED_SURFACE()
B_SPLINE_SURFACE(5,1,((#60104,#60105),(#60106,#60107),(#60108,#60109),(#60110,
#60111),(#60112,#60113),(#60114,#60115),(#60116,#60117),(#60118,#60119),
(#60120,#60121),(#60122,#60123),(#60124,#60125),(#60126,#60127),(#60128,
#60129),(#60130,#60131),(#60132,#60133),(#60134,#60135),(#60136,#60137),
(#60138,#60139),(#60140,#60141),(#60142,#60143),(#60144,#60145),(#60146,
#60147),(#60148,#60149),(#60150,#60151),(#60152,#60153),(#60154,#60155),
(#60156,#60157),(#60158,#60159),(#60160,#60161),(#60162,#60163),(#60164,
#60165),(#60166,#60167),(#60168,#60169),(#60170,#60171),(#60172,#60173),
(#60174,#60175),(#60176,#60177),(#60178,#60179),(#60180,#60181),(#60182,
#60183),(#60184,#60185),(#60186,#60187),(#60188,#60189),(#60190,#60191),
(#60192,#60193),(#60194,#60195),(#60196,#60197),(#60198,#60199),(#60200,
#60201),(#60202,#60203),(#60204,#60205),(#60206,#60207),(#60208,#60209),
(#60210,#60211),(#60212,#60213),(#60214,#60215),(#60216,#60217),(#60218,
#60219),(#60220,#60221),(#60222,#60223),(#60224,#60225),(#60226,#60227),
(#60228,#60229),(#60230,#60231),(#60232,#60233),(#60234,#60235),(#60236,
#60237),(#60238,#60239),(#60240,#60241),(#60242,#60243)),.UNSPECIFIED.,
 .F.,.F.,.F.)
B_SPLINE_SURFACE_WITH_KNOTS((6,1,1,1,1,1,1,1,1,1,1,1,1,1,1,1,1,1,1,1,1,
1,1,1,1,1,1,1,1,1,1,1,1,1,1,1,1,1,1,1,1,1,1,1,1,1,1,1,1,1,1,1,1,1,1,1,1,
1,1,1,1,1,1,1,1,6),(2,2),(-1.,-0.984615384615383,-0.969230769230768,-0.953846153846152,
-0.938461538461537,-0.923076923076922,-0.907692307692306,-0.892307692307691,
-0.876923076923076,-0.86153846153846,-0.846153846153845,-0.83076923076923,
-0.815384615384614,-0.799999999999999,-0.784615384615384,-0.769230769230768,
-0.753846153846153,-0.738461538461538,-0.723076923076922,-0.707692307692307,
-0.692307692307692,-0.676923076923076,-0.661538461538461,-0.646153846153846,
-0.63076923076923,-0.615384615384615,-0.6,-0.584615384615384,-0.569230769230769,
-0.553846153846154,-0.538461538461538,-0.523076923076923,-0.507692307692308,
-0.492307692307692,-0.476923076923077,-0.461538461538462,-0.446153846153846,
-0.430769230769231,-0.415384615384615,-0.4,-0.384615384615385,-0.369230769230769,
-0.353846153846154,-0.338461538461538,-0.323076923076923,-0.307692307692308,
-0.292307692307692,-0.276923076923077,-0.261538461538462,-0.246153846153846,
-0.230769230769231,-0.215384615384615,-0.2,-0.184615384615385,-0.169230769230769,
-0.153846153846154,-0.138461538461538,-0.123076923076923,-0.107692307692308,
-0.0923076923076923,-0.0769230769230769,-0.0615384615384615,-0.0461538461538462,
-0.0307692307692308,-0.0153846153846154,0.),(-1.,1.),.UNSPECIFIED.)
GEOMETRIC_REPRESENTATION_ITEM()
RATIONAL_B_SPLINE_SURFACE(((1.,1.),(1.,1.),(1.,1.),(1.,1.),(1.,1.),(1.,
1.),(1.,1.),(1.,1.),(1.,1.),(1.,1.),(1.,1.),(1.,1.),(1.,1.),(1.,1.),(1.,
1.),(1.,1.),(1.,1.),(1.,1.),(1.,1.),(1.,1.),(1.,1.),(1.,1.),(1.,1.),(1.,
1.),(1.,1.),(1.,1.),(1.,1.),(1.,1.),(1.,1.),(1.,1.),(1.,1.),(1.,1.),(1.,
1.),(1.,1.),(1.,1.),(1.,1.),(1.,1.),(1.,1.),(1.,1.),(1.,1.),(1.,1.),(1.,
1.),(1.,1.),(1.,1.),(1.,1.),(1.,1.),(1.,1.),(1.,1.),(1.,1.),(1.,1.),(1.,
1.),(1.,1.),(1.,1.),(1.,1.),(1.,1.),(1.,1.),(1.,1.),(1.,1.),(1.,1.),(1.,
1.),(1.,1.),(1.,1.),(1.,1.),(1.,1.),(1.,1.),(1.,1.),(1.,1.),(1.,1.),(1.,
1.),(1.,1.)))
REPRESENTATION_ITEM('')
SURFACE()
);
#122=(
BOUNDED_SURFACE()
B_SPLINE_SURFACE(5,1,((#60316,#60317),(#60318,#60319),(#60320,#60321),(#60322,
#60323),(#60324,#60325),(#60326,#60327),(#60328,#60329),(#60330,#60331),
(#60332,#60333),(#60334,#60335),(#60336,#60337),(#60338,#60339),(#60340,
#60341),(#60342,#60343),(#60344,#60345),(#60346,#60347),(#60348,#60349),
(#60350,#60351),(#60352,#60353),(#60354,#60355),(#60356,#60357),(#60358,
#60359),(#60360,#60361),(#60362,#60363),(#60364,#60365),(#60366,#60367),
(#60368,#60369),(#60370,#60371),(#60372,#60373),(#60374,#60375),(#60376,
#60377),(#60378,#60379),(#60380,#60381),(#60382,#60383),(#60384,#60385),
(#60386,#60387),(#60388,#60389),(#60390,#60391),(#60392,#60393),(#60394,
#60395),(#60396,#60397),(#60398,#60399),(#60400,#60401),(#60402,#60403),
(#60404,#60405),(#60406,#60407),(#60408,#60409),(#60410,#60411),(#60412,
#60413),(#60414,#60415),(#60416,#60417),(#60418,#60419),(#60420,#60421),
(#60422,#60423),(#60424,#60425),(#60426,#60427),(#60428,#60429),(#60430,
#60431),(#60432,#60433),(#60434,#60435),(#60436,#60437),(#60438,#60439),
(#60440,#60441),(#60442,#60443),(#60444,#60445),(#60446,#60447),(#60448,
#60449),(#60450,#60451),(#60452,#60453),(#60454,#60455)),.UNSPECIFIED.,
 .F.,.F.,.F.)
B_SPLINE_SURFACE_WITH_KNOTS((6,1,1,1,1,1,1,1,1,1,1,1,1,1,1,1,1,1,1,1,1,
1,1,1,1,1,1,1,1,1,1,1,1,1,1,1,1,1,1,1,1,1,1,1,1,1,1,1,1,1,1,1,1,1,1,1,1,
1,1,1,1,1,1,1,1,6),(2,2),(-1.,-0.984615384615383,-0.969230769230768,-0.953846153846152,
-0.938461538461537,-0.923076923076922,-0.907692307692306,-0.892307692307691,
-0.876923076923076,-0.86153846153846,-0.846153846153845,-0.83076923076923,
-0.815384615384614,-0.799999999999999,-0.784615384615384,-0.769230769230768,
-0.753846153846153,-0.738461538461538,-0.723076923076922,-0.707692307692307,
-0.692307692307692,-0.676923076923076,-0.661538461538461,-0.646153846153846,
-0.63076923076923,-0.615384615384615,-0.6,-0.584615384615384,-0.569230769230769,
-0.553846153846154,-0.538461538461538,-0.523076923076923,-0.507692307692308,
-0.492307692307692,-0.476923076923077,-0.461538461538462,-0.446153846153846,
-0.430769230769231,-0.415384615384615,-0.4,-0.384615384615385,-0.369230769230769,
-0.353846153846154,-0.338461538461538,-0.323076923076923,-0.307692307692308,
-0.292307692307692,-0.276923076923077,-0.261538461538462,-0.246153846153846,
-0.230769230769231,-0.215384615384615,-0.2,-0.184615384615385,-0.169230769230769,
-0.153846153846154,-0.138461538461538,-0.123076923076923,-0.107692307692308,
-0.0923076923076923,-0.0769230769230769,-0.0615384615384615,-0.0461538461538462,
-0.0307692307692308,-0.0153846153846154,0.),(-1.,1.),.UNSPECIFIED.)
GEOMETRIC_REPRESENTATION_ITEM()
RATIONAL_B_SPLINE_SURFACE(((1.,1.),(1.,1.),(1.,1.),(1.,1.),(1.,1.),(1.,
1.),(1.,1.),(1.,1.),(1.,1.),(1.,1.),(1.,1.),(1.,1.),(1.,1.),(1.,1.),(1.,
1.),(1.,1.),(1.,1.),(1.,1.),(1.,1.),(1.,1.),(1.,1.),(1.,1.),(1.,1.),(1.,
1.),(1.,1.),(1.,1.),(1.,1.),(1.,1.),(1.,1.),(1.,1.),(1.,1.),(1.,1.),(1.,
1.),(1.,1.),(1.,1.),(1.,1.),(1.,1.),(1.,1.),(1.,1.),(1.,1.),(1.,1.),(1.,
1.),(1.,1.),(1.,1.),(1.,1.),(1.,1.),(1.,1.),(1.,1.),(1.,1.),(1.,1.),(1.,
1.),(1.,1.),(1.,1.),(1.,1.),(1.,1.),(1.,1.),(1.,1.),(1.,1.),(1.,1.),(1.,
1.),(1.,1.),(1.,1.),(1.,1.),(1.,1.),(1.,1.),(1.,1.),(1.,1.),(1.,1.),(1.,
1.),(1.,1.)))
REPRESENTATION_ITEM('')
SURFACE()
);
#123=(
BOUNDED_SURFACE()
B_SPLINE_SURFACE(5,1,((#60546,#60547),(#60548,#60549),(#60550,#60551),(#60552,
#60553),(#60554,#60555),(#60556,#60557),(#60558,#60559),(#60560,#60561),
(#60562,#60563),(#60564,#60565),(#60566,#60567),(#60568,#60569),(#60570,
#60571),(#60572,#60573),(#60574,#60575),(#60576,#60577),(#60578,#60579),
(#60580,#60581),(#60582,#60583),(#60584,#60585),(#60586,#60587),(#60588,
#60589),(#60590,#60591),(#60592,#60593),(#60594,#60595),(#60596,#60597),
(#60598,#60599),(#60600,#60601),(#60602,#60603),(#60604,#60605),(#60606,
#60607),(#60608,#60609),(#60610,#60611),(#60612,#60613),(#60614,#60615),
(#60616,#60617),(#60618,#60619),(#60620,#60621),(#60622,#60623),(#60624,
#60625),(#60626,#60627),(#60628,#60629),(#60630,#60631),(#60632,#60633),
(#60634,#60635),(#60636,#60637),(#60638,#60639),(#60640,#60641),(#60642,
#60643),(#60644,#60645),(#60646,#60647),(#60648,#60649),(#60650,#60651),
(#60652,#60653),(#60654,#60655),(#60656,#60657),(#60658,#60659),(#60660,
#60661),(#60662,#60663),(#60664,#60665),(#60666,#60667),(#60668,#60669),
(#60670,#60671),(#60672,#60673),(#60674,#60675),(#60676,#60677),(#60678,
#60679),(#60680,#60681),(#60682,#60683),(#60684,#60685)),.UNSPECIFIED.,
 .F.,.F.,.F.)
B_SPLINE_SURFACE_WITH_KNOTS((6,1,1,1,1,1,1,1,1,1,1,1,1,1,1,1,1,1,1,1,1,
1,1,1,1,1,1,1,1,1,1,1,1,1,1,1,1,1,1,1,1,1,1,1,1,1,1,1,1,1,1,1,1,1,1,1,1,
1,1,1,1,1,1,1,1,6),(2,2),(-1.,-0.984615384615383,-0.969230769230768,-0.953846153846152,
-0.938461538461537,-0.923076923076922,-0.907692307692306,-0.892307692307691,
-0.876923076923076,-0.86153846153846,-0.846153846153845,-0.83076923076923,
-0.815384615384614,-0.799999999999999,-0.784615384615384,-0.769230769230768,
-0.753846153846153,-0.738461538461538,-0.723076923076922,-0.707692307692307,
-0.692307692307692,-0.676923076923076,-0.661538461538461,-0.646153846153846,
-0.63076923076923,-0.615384615384615,-0.6,-0.584615384615384,-0.569230769230769,
-0.553846153846154,-0.538461538461538,-0.523076923076923,-0.507692307692308,
-0.492307692307692,-0.476923076923077,-0.461538461538462,-0.446153846153846,
-0.430769230769231,-0.415384615384615,-0.4,-0.384615384615385,-0.369230769230769,
-0.353846153846154,-0.338461538461538,-0.323076923076923,-0.307692307692308,
-0.292307692307692,-0.276923076923077,-0.261538461538462,-0.246153846153846,
-0.230769230769231,-0.215384615384615,-0.2,-0.184615384615385,-0.169230769230769,
-0.153846153846154,-0.138461538461538,-0.123076923076923,-0.107692307692308,
-0.0923076923076923,-0.0769230769230769,-0.0615384615384615,-0.0461538461538462,
-0.0307692307692308,-0.0153846153846154,0.),(-1.,1.),.UNSPECIFIED.)
GEOMETRIC_REPRESENTATION_ITEM()
RATIONAL_B_SPLINE_SURFACE(((1.,1.),(1.,1.),(1.,1.),(1.,1.),(1.,1.),(1.,
1.),(1.,1.),(1.,1.),(1.,1.),(1.,1.),(1.,1.),(1.,1.),(1.,1.),(1.,1.),(1.,
1.),(1.,1.),(1.,1.),(1.,1.),(1.,1.),(1.,1.),(1.,1.),(1.,1.),(1.,1.),(1.,
1.),(1.,1.),(1.,1.),(1.,1.),(1.,1.),(1.,1.),(1.,1.),(1.,1.),(1.,1.),(1.,
1.),(1.,1.),(1.,1.),(1.,1.),(1.,1.),(1.,1.),(1.,1.),(1.,1.),(1.,1.),(1.,
1.),(1.,1.),(1.,1.),(1.,1.),(1.,1.),(1.,1.),(1.,1.),(1.,1.),(1.,1.),(1.,
1.),(1.,1.),(1.,1.),(1.,1.),(1.,1.),(1.,1.),(1.,1.),(1.,1.),(1.,1.),(1.,
1.),(1.,1.),(1.,1.),(1.,1.),(1.,1.),(1.,1.),(1.,1.),(1.,1.),(1.,1.),(1.,
1.),(1.,1.)))
REPRESENTATION_ITEM('')
SURFACE()
);
#124=(
BOUNDED_SURFACE()
B_SPLINE_SURFACE(5,1,((#60758,#60759),(#60760,#60761),(#60762,#60763),(#60764,
#60765),(#60766,#60767),(#60768,#60769),(#60770,#60771),(#60772,#60773),
(#60774,#60775),(#60776,#60777),(#60778,#60779),(#60780,#60781),(#60782,
#60783),(#60784,#60785),(#60786,#60787),(#60788,#60789),(#60790,#60791),
(#60792,#60793),(#60794,#60795),(#60796,#60797),(#60798,#60799),(#60800,
#60801),(#60802,#60803),(#60804,#60805),(#60806,#60807),(#60808,#60809),
(#60810,#60811),(#60812,#60813),(#60814,#60815),(#60816,#60817),(#60818,
#60819),(#60820,#60821),(#60822,#60823),(#60824,#60825),(#60826,#60827),
(#60828,#60829),(#60830,#60831),(#60832,#60833),(#60834,#60835),(#60836,
#60837),(#60838,#60839),(#60840,#60841),(#60842,#60843),(#60844,#60845),
(#60846,#60847),(#60848,#60849),(#60850,#60851),(#60852,#60853),(#60854,
#60855),(#60856,#60857),(#60858,#60859),(#60860,#60861),(#60862,#60863),
(#60864,#60865),(#60866,#60867),(#60868,#60869),(#60870,#60871),(#60872,
#60873),(#60874,#60875),(#60876,#60877),(#60878,#60879),(#60880,#60881),
(#60882,#60883),(#60884,#60885),(#60886,#60887),(#60888,#60889),(#60890,
#60891),(#60892,#60893),(#60894,#60895),(#60896,#60897)),.UNSPECIFIED.,
 .F.,.F.,.F.)
B_SPLINE_SURFACE_WITH_KNOTS((6,1,1,1,1,1,1,1,1,1,1,1,1,1,1,1,1,1,1,1,1,
1,1,1,1,1,1,1,1,1,1,1,1,1,1,1,1,1,1,1,1,1,1,1,1,1,1,1,1,1,1,1,1,1,1,1,1,
1,1,1,1,1,1,1,1,6),(2,2),(-1.,-0.984615384615383,-0.969230769230768,-0.953846153846152,
-0.938461538461537,-0.923076923076922,-0.907692307692306,-0.892307692307691,
-0.876923076923076,-0.86153846153846,-0.846153846153845,-0.83076923076923,
-0.815384615384614,-0.799999999999999,-0.784615384615384,-0.769230769230768,
-0.753846153846153,-0.738461538461538,-0.723076923076922,-0.707692307692307,
-0.692307692307692,-0.676923076923076,-0.661538461538461,-0.646153846153846,
-0.63076923076923,-0.615384615384615,-0.6,-0.584615384615384,-0.569230769230769,
-0.553846153846154,-0.538461538461538,-0.523076923076923,-0.507692307692308,
-0.492307692307692,-0.476923076923077,-0.461538461538462,-0.446153846153846,
-0.430769230769231,-0.415384615384615,-0.4,-0.384615384615385,-0.369230769230769,
-0.353846153846154,-0.338461538461538,-0.323076923076923,-0.307692307692308,
-0.292307692307692,-0.276923076923077,-0.261538461538462,-0.246153846153846,
-0.230769230769231,-0.215384615384615,-0.2,-0.184615384615385,-0.169230769230769,
-0.153846153846154,-0.138461538461538,-0.123076923076923,-0.107692307692308,
-0.0923076923076923,-0.0769230769230769,-0.0615384615384615,-0.0461538461538462,
-0.0307692307692308,-0.0153846153846154,0.),(-1.,1.),.UNSPECIFIED.)
GEOMETRIC_REPRESENTATION_ITEM()
RATIONAL_B_SPLINE_SURFACE(((1.,1.),(1.,1.),(1.,1.),(1.,1.),(1.,1.),(1.,
1.),(1.,1.),(1.,1.),(1.,1.),(1.,1.),(1.,1.),(1.,1.),(1.,1.),(1.,1.),(1.,
1.),(1.,1.),(1.,1.),(1.,1.),(1.,1.),(1.,1.),(1.,1.),(1.,1.),(1.,1.),(1.,
1.),(1.,1.),(1.,1.),(1.,1.),(1.,1.),(1.,1.),(1.,1.),(1.,1.),(1.,1.),(1.,
1.),(1.,1.),(1.,1.),(1.,1.),(1.,1.),(1.,1.),(1.,1.),(1.,1.),(1.,1.),(1.,
1.),(1.,1.),(1.,1.),(1.,1.),(1.,1.),(1.,1.),(1.,1.),(1.,1.),(1.,1.),(1.,
1.),(1.,1.),(1.,1.),(1.,1.),(1.,1.),(1.,1.),(1.,1.),(1.,1.),(1.,1.),(1.,
1.),(1.,1.),(1.,1.),(1.,1.),(1.,1.),(1.,1.),(1.,1.),(1.,1.),(1.,1.),(1.,
1.),(1.,1.)))
REPRESENTATION_ITEM('')
SURFACE()
);
#125=(
BOUNDED_SURFACE()
B_SPLINE_SURFACE(5,1,((#60988,#60989),(#60990,#60991),(#60992,#60993),(#60994,
#60995),(#60996,#60997),(#60998,#60999),(#61000,#61001),(#61002,#61003),
(#61004,#61005),(#61006,#61007),(#61008,#61009),(#61010,#61011),(#61012,
#61013),(#61014,#61015),(#61016,#61017),(#61018,#61019),(#61020,#61021),
(#61022,#61023),(#61024,#61025),(#61026,#61027),(#61028,#61029),(#61030,
#61031),(#61032,#61033),(#61034,#61035),(#61036,#61037),(#61038,#61039),
(#61040,#61041),(#61042,#61043),(#61044,#61045),(#61046,#61047),(#61048,
#61049),(#61050,#61051),(#61052,#61053),(#61054,#61055),(#61056,#61057),
(#61058,#61059),(#61060,#61061),(#61062,#61063),(#61064,#61065),(#61066,
#61067),(#61068,#61069),(#61070,#61071),(#61072,#61073),(#61074,#61075),
(#61076,#61077),(#61078,#61079),(#61080,#61081),(#61082,#61083),(#61084,
#61085),(#61086,#61087),(#61088,#61089),(#61090,#61091),(#61092,#61093),
(#61094,#61095),(#61096,#61097),(#61098,#61099),(#61100,#61101),(#61102,
#61103),(#61104,#61105),(#61106,#61107),(#61108,#61109),(#61110,#61111),
(#61112,#61113),(#61114,#61115),(#61116,#61117),(#61118,#61119),(#61120,
#61121),(#61122,#61123),(#61124,#61125),(#61126,#61127)),.UNSPECIFIED.,
 .F.,.F.,.F.)
B_SPLINE_SURFACE_WITH_KNOTS((6,1,1,1,1,1,1,1,1,1,1,1,1,1,1,1,1,1,1,1,1,
1,1,1,1,1,1,1,1,1,1,1,1,1,1,1,1,1,1,1,1,1,1,1,1,1,1,1,1,1,1,1,1,1,1,1,1,
1,1,1,1,1,1,1,1,6),(2,2),(-1.,-0.984615384615383,-0.969230769230768,-0.953846153846152,
-0.938461538461537,-0.923076923076922,-0.907692307692306,-0.892307692307691,
-0.876923076923076,-0.86153846153846,-0.846153846153845,-0.83076923076923,
-0.815384615384614,-0.799999999999999,-0.784615384615384,-0.769230769230768,
-0.753846153846153,-0.738461538461538,-0.723076923076922,-0.707692307692307,
-0.692307692307692,-0.676923076923076,-0.661538461538461,-0.646153846153846,
-0.63076923076923,-0.615384615384615,-0.6,-0.584615384615384,-0.569230769230769,
-0.553846153846154,-0.538461538461538,-0.523076923076923,-0.507692307692308,
-0.492307692307692,-0.476923076923077,-0.461538461538462,-0.446153846153846,
-0.430769230769231,-0.415384615384615,-0.4,-0.384615384615385,-0.369230769230769,
-0.353846153846154,-0.338461538461538,-0.323076923076923,-0.307692307692308,
-0.292307692307692,-0.276923076923077,-0.261538461538462,-0.246153846153846,
-0.230769230769231,-0.215384615384615,-0.2,-0.184615384615385,-0.169230769230769,
-0.153846153846154,-0.138461538461538,-0.123076923076923,-0.107692307692308,
-0.0923076923076923,-0.0769230769230769,-0.0615384615384615,-0.0461538461538462,
-0.0307692307692308,-0.0153846153846154,0.),(-1.,1.),.UNSPECIFIED.)
GEOMETRIC_REPRESENTATION_ITEM()
RATIONAL_B_SPLINE_SURFACE(((1.,1.),(1.,1.),(1.,1.),(1.,1.),(1.,1.),(1.,
1.),(1.,1.),(1.,1.),(1.,1.),(1.,1.),(1.,1.),(1.,1.),(1.,1.),(1.,1.),(1.,
1.),(1.,1.),(1.,1.),(1.,1.),(1.,1.),(1.,1.),(1.,1.),(1.,1.),(1.,1.),(1.,
1.),(1.,1.),(1.,1.),(1.,1.),(1.,1.),(1.,1.),(1.,1.),(1.,1.),(1.,1.),(1.,
1.),(1.,1.),(1.,1.),(1.,1.),(1.,1.),(1.,1.),(1.,1.),(1.,1.),(1.,1.),(1.,
1.),(1.,1.),(1.,1.),(1.,1.),(1.,1.),(1.,1.),(1.,1.),(1.,1.),(1.,1.),(1.,
1.),(1.,1.),(1.,1.),(1.,1.),(1.,1.),(1.,1.),(1.,1.),(1.,1.),(1.,1.),(1.,
1.),(1.,1.),(1.,1.),(1.,1.),(1.,1.),(1.,1.),(1.,1.),(1.,1.),(1.,1.),(1.,
1.),(1.,1.)))
REPRESENTATION_ITEM('')
SURFACE()
);
#126=(
BOUNDED_SURFACE()
B_SPLINE_SURFACE(5,1,((#61200,#61201),(#61202,#61203),(#61204,#61205),(#61206,
#61207),(#61208,#61209),(#61210,#61211),(#61212,#61213),(#61214,#61215),
(#61216,#61217),(#61218,#61219),(#61220,#61221),(#61222,#61223),(#61224,
#61225),(#61226,#61227),(#61228,#61229),(#61230,#61231),(#61232,#61233),
(#61234,#61235),(#61236,#61237),(#61238,#61239),(#61240,#61241),(#61242,
#61243),(#61244,#61245),(#61246,#61247),(#61248,#61249),(#61250,#61251),
(#61252,#61253),(#61254,#61255),(#61256,#61257),(#61258,#61259),(#61260,
#61261),(#61262,#61263),(#61264,#61265),(#61266,#61267),(#61268,#61269),
(#61270,#61271),(#61272,#61273),(#61274,#61275),(#61276,#61277),(#61278,
#61279),(#61280,#61281),(#61282,#61283),(#61284,#61285),(#61286,#61287),
(#61288,#61289),(#61290,#61291),(#61292,#61293),(#61294,#61295),(#61296,
#61297),(#61298,#61299),(#61300,#61301),(#61302,#61303),(#61304,#61305),
(#61306,#61307),(#61308,#61309),(#61310,#61311),(#61312,#61313),(#61314,
#61315),(#61316,#61317),(#61318,#61319),(#61320,#61321),(#61322,#61323),
(#61324,#61325),(#61326,#61327),(#61328,#61329),(#61330,#61331),(#61332,
#61333),(#61334,#61335),(#61336,#61337),(#61338,#61339)),.UNSPECIFIED.,
 .F.,.F.,.F.)
B_SPLINE_SURFACE_WITH_KNOTS((6,1,1,1,1,1,1,1,1,1,1,1,1,1,1,1,1,1,1,1,1,
1,1,1,1,1,1,1,1,1,1,1,1,1,1,1,1,1,1,1,1,1,1,1,1,1,1,1,1,1,1,1,1,1,1,1,1,
1,1,1,1,1,1,1,1,6),(2,2),(-1.,-0.984615384615383,-0.969230769230768,-0.953846153846152,
-0.938461538461537,-0.923076923076922,-0.907692307692306,-0.892307692307691,
-0.876923076923076,-0.86153846153846,-0.846153846153845,-0.83076923076923,
-0.815384615384614,-0.799999999999999,-0.784615384615384,-0.769230769230768,
-0.753846153846153,-0.738461538461538,-0.723076923076922,-0.707692307692307,
-0.692307692307692,-0.676923076923076,-0.661538461538461,-0.646153846153846,
-0.63076923076923,-0.615384615384615,-0.6,-0.584615384615384,-0.569230769230769,
-0.553846153846154,-0.538461538461538,-0.523076923076923,-0.507692307692308,
-0.492307692307692,-0.476923076923077,-0.461538461538462,-0.446153846153846,
-0.430769230769231,-0.415384615384615,-0.4,-0.384615384615385,-0.369230769230769,
-0.353846153846154,-0.338461538461538,-0.323076923076923,-0.307692307692308,
-0.292307692307692,-0.276923076923077,-0.261538461538462,-0.246153846153846,
-0.230769230769231,-0.215384615384615,-0.2,-0.184615384615385,-0.169230769230769,
-0.153846153846154,-0.138461538461538,-0.123076923076923,-0.107692307692308,
-0.0923076923076923,-0.0769230769230769,-0.0615384615384615,-0.0461538461538462,
-0.0307692307692308,-0.0153846153846154,0.),(-1.,1.),.UNSPECIFIED.)
GEOMETRIC_REPRESENTATION_ITEM()
RATIONAL_B_SPLINE_SURFACE(((1.,1.),(1.,1.),(1.,1.),(1.,1.),(1.,1.),(1.,
1.),(1.,1.),(1.,1.),(1.,1.),(1.,1.),(1.,1.),(1.,1.),(1.,1.),(1.,1.),(1.,
1.),(1.,1.),(1.,1.),(1.,1.),(1.,1.),(1.,1.),(1.,1.),(1.,1.),(1.,1.),(1.,
1.),(1.,1.),(1.,1.),(1.,1.),(1.,1.),(1.,1.),(1.,1.),(1.,1.),(1.,1.),(1.,
1.),(1.,1.),(1.,1.),(1.,1.),(1.,1.),(1.,1.),(1.,1.),(1.,1.),(1.,1.),(1.,
1.),(1.,1.),(1.,1.),(1.,1.),(1.,1.),(1.,1.),(1.,1.),(1.,1.),(1.,1.),(1.,
1.),(1.,1.),(1.,1.),(1.,1.),(1.,1.),(1.,1.),(1.,1.),(1.,1.),(1.,1.),(1.,
1.),(1.,1.),(1.,1.),(1.,1.),(1.,1.),(1.,1.),(1.,1.),(1.,1.),(1.,1.),(1.,
1.),(1.,1.)))
REPRESENTATION_ITEM('')
SURFACE()
);
#127=(
BOUNDED_SURFACE()
B_SPLINE_SURFACE(5,1,((#61430,#61431),(#61432,#61433),(#61434,#61435),(#61436,
#61437),(#61438,#61439),(#61440,#61441),(#61442,#61443),(#61444,#61445),
(#61446,#61447),(#61448,#61449),(#61450,#61451),(#61452,#61453),(#61454,
#61455),(#61456,#61457),(#61458,#61459),(#61460,#61461),(#61462,#61463),
(#61464,#61465),(#61466,#61467),(#61468,#61469),(#61470,#61471),(#61472,
#61473),(#61474,#61475),(#61476,#61477),(#61478,#61479),(#61480,#61481),
(#61482,#61483),(#61484,#61485),(#61486,#61487),(#61488,#61489),(#61490,
#61491),(#61492,#61493),(#61494,#61495),(#61496,#61497),(#61498,#61499),
(#61500,#61501),(#61502,#61503),(#61504,#61505),(#61506,#61507),(#61508,
#61509),(#61510,#61511),(#61512,#61513),(#61514,#61515),(#61516,#61517),
(#61518,#61519),(#61520,#61521),(#61522,#61523),(#61524,#61525),(#61526,
#61527),(#61528,#61529),(#61530,#61531),(#61532,#61533),(#61534,#61535),
(#61536,#61537),(#61538,#61539),(#61540,#61541),(#61542,#61543),(#61544,
#61545),(#61546,#61547),(#61548,#61549),(#61550,#61551),(#61552,#61553),
(#61554,#61555),(#61556,#61557),(#61558,#61559),(#61560,#61561),(#61562,
#61563),(#61564,#61565),(#61566,#61567),(#61568,#61569)),.UNSPECIFIED.,
 .F.,.F.,.F.)
B_SPLINE_SURFACE_WITH_KNOTS((6,1,1,1,1,1,1,1,1,1,1,1,1,1,1,1,1,1,1,1,1,
1,1,1,1,1,1,1,1,1,1,1,1,1,1,1,1,1,1,1,1,1,1,1,1,1,1,1,1,1,1,1,1,1,1,1,1,
1,1,1,1,1,1,1,1,6),(2,2),(-1.,-0.984615384615383,-0.969230769230768,-0.953846153846152,
-0.938461538461537,-0.923076923076922,-0.907692307692306,-0.892307692307691,
-0.876923076923076,-0.86153846153846,-0.846153846153845,-0.83076923076923,
-0.815384615384614,-0.799999999999999,-0.784615384615384,-0.769230769230768,
-0.753846153846153,-0.738461538461538,-0.723076923076922,-0.707692307692307,
-0.692307692307692,-0.676923076923076,-0.661538461538461,-0.646153846153846,
-0.63076923076923,-0.615384615384615,-0.6,-0.584615384615384,-0.569230769230769,
-0.553846153846154,-0.538461538461538,-0.523076923076923,-0.507692307692308,
-0.492307692307692,-0.476923076923077,-0.461538461538462,-0.446153846153846,
-0.430769230769231,-0.415384615384615,-0.4,-0.384615384615385,-0.369230769230769,
-0.353846153846154,-0.338461538461538,-0.323076923076923,-0.307692307692308,
-0.292307692307692,-0.276923076923077,-0.261538461538462,-0.246153846153846,
-0.230769230769231,-0.215384615384615,-0.2,-0.184615384615385,-0.169230769230769,
-0.153846153846154,-0.138461538461538,-0.123076923076923,-0.107692307692308,
-0.0923076923076923,-0.0769230769230769,-0.0615384615384615,-0.0461538461538462,
-0.0307692307692308,-0.0153846153846154,0.),(-1.,1.),.UNSPECIFIED.)
GEOMETRIC_REPRESENTATION_ITEM()
RATIONAL_B_SPLINE_SURFACE(((1.,1.),(1.,1.),(1.,1.),(1.,1.),(1.,1.),(1.,
1.),(1.,1.),(1.,1.),(1.,1.),(1.,1.),(1.,1.),(1.,1.),(1.,1.),(1.,1.),(1.,
1.),(1.,1.),(1.,1.),(1.,1.),(1.,1.),(1.,1.),(1.,1.),(1.,1.),(1.,1.),(1.,
1.),(1.,1.),(1.,1.),(1.,1.),(1.,1.),(1.,1.),(1.,1.),(1.,1.),(1.,1.),(1.,
1.),(1.,1.),(1.,1.),(1.,1.),(1.,1.),(1.,1.),(1.,1.),(1.,1.),(1.,1.),(1.,
1.),(1.,1.),(1.,1.),(1.,1.),(1.,1.),(1.,1.),(1.,1.),(1.,1.),(1.,1.),(1.,
1.),(1.,1.),(1.,1.),(1.,1.),(1.,1.),(1.,1.),(1.,1.),(1.,1.),(1.,1.),(1.,
1.),(1.,1.),(1.,1.),(1.,1.),(1.,1.),(1.,1.),(1.,1.),(1.,1.),(1.,1.),(1.,
1.),(1.,1.)))
REPRESENTATION_ITEM('')
SURFACE()
);
#128=(
BOUNDED_SURFACE()
B_SPLINE_SURFACE(5,1,((#61646,#61647),(#61648,#61649),(#61650,#61651),(#61652,
#61653),(#61654,#61655),(#61656,#61657),(#61658,#61659),(#61660,#61661),
(#61662,#61663),(#61664,#61665),(#61666,#61667),(#61668,#61669),(#61670,
#61671),(#61672,#61673),(#61674,#61675),(#61676,#61677),(#61678,#61679),
(#61680,#61681),(#61682,#61683),(#61684,#61685),(#61686,#61687),(#61688,
#61689),(#61690,#61691),(#61692,#61693),(#61694,#61695),(#61696,#61697),
(#61698,#61699),(#61700,#61701),(#61702,#61703),(#61704,#61705),(#61706,
#61707),(#61708,#61709),(#61710,#61711),(#61712,#61713),(#61714,#61715),
(#61716,#61717),(#61718,#61719),(#61720,#61721),(#61722,#61723),(#61724,
#61725),(#61726,#61727),(#61728,#61729),(#61730,#61731),(#61732,#61733),
(#61734,#61735),(#61736,#61737),(#61738,#61739),(#61740,#61741),(#61742,
#61743),(#61744,#61745),(#61746,#61747),(#61748,#61749),(#61750,#61751),
(#61752,#61753),(#61754,#61755),(#61756,#61757),(#61758,#61759),(#61760,
#61761),(#61762,#61763),(#61764,#61765),(#61766,#61767),(#61768,#61769),
(#61770,#61771),(#61772,#61773),(#61774,#61775),(#61776,#61777),(#61778,
#61779),(#61780,#61781),(#61782,#61783),(#61784,#61785)),.UNSPECIFIED.,
 .F.,.F.,.F.)
B_SPLINE_SURFACE_WITH_KNOTS((6,1,1,1,1,1,1,1,1,1,1,1,1,1,1,1,1,1,1,1,1,
1,1,1,1,1,1,1,1,1,1,1,1,1,1,1,1,1,1,1,1,1,1,1,1,1,1,1,1,1,1,1,1,1,1,1,1,
1,1,1,1,1,1,1,1,6),(2,2),(-1.,-0.984615384615383,-0.969230769230768,-0.953846153846152,
-0.938461538461537,-0.923076923076922,-0.907692307692306,-0.892307692307691,
-0.876923076923076,-0.86153846153846,-0.846153846153845,-0.83076923076923,
-0.815384615384614,-0.799999999999999,-0.784615384615384,-0.769230769230768,
-0.753846153846153,-0.738461538461538,-0.723076923076922,-0.707692307692307,
-0.692307692307692,-0.676923076923076,-0.661538461538461,-0.646153846153846,
-0.63076923076923,-0.615384615384615,-0.6,-0.584615384615384,-0.569230769230769,
-0.553846153846154,-0.538461538461538,-0.523076923076923,-0.507692307692308,
-0.492307692307692,-0.476923076923077,-0.461538461538462,-0.446153846153846,
-0.430769230769231,-0.415384615384615,-0.4,-0.384615384615385,-0.369230769230769,
-0.353846153846154,-0.338461538461538,-0.323076923076923,-0.307692307692308,
-0.292307692307692,-0.276923076923077,-0.261538461538462,-0.246153846153846,
-0.230769230769231,-0.215384615384615,-0.2,-0.184615384615385,-0.169230769230769,
-0.153846153846154,-0.138461538461538,-0.123076923076923,-0.107692307692308,
-0.0923076923076923,-0.0769230769230769,-0.0615384615384615,-0.0461538461538462,
-0.0307692307692308,-0.0153846153846154,0.),(-1.,1.),.UNSPECIFIED.)
GEOMETRIC_REPRESENTATION_ITEM()
RATIONAL_B_SPLINE_SURFACE(((1.,1.),(1.,1.),(1.,1.),(1.,1.),(1.,1.),(1.,
1.),(1.,1.),(1.,1.),(1.,1.),(1.,1.),(1.,1.),(1.,1.),(1.,1.),(1.,1.),(1.,
1.),(1.,1.),(1.,1.),(1.,1.),(1.,1.),(1.,1.),(1.,1.),(1.,1.),(1.,1.),(1.,
1.),(1.,1.),(1.,1.),(1.,1.),(1.,1.),(1.,1.),(1.,1.),(1.,1.),(1.,1.),(1.,
1.),(1.,1.),(1.,1.),(1.,1.),(1.,1.),(1.,1.),(1.,1.),(1.,1.),(1.,1.),(1.,
1.),(1.,1.),(1.,1.),(1.,1.),(1.,1.),(1.,1.),(1.,1.),(1.,1.),(1.,1.),(1.,
1.),(1.,1.),(1.,1.),(1.,1.),(1.,1.),(1.,1.),(1.,1.),(1.,1.),(1.,1.),(1.,
1.),(1.,1.),(1.,1.),(1.,1.),(1.,1.),(1.,1.),(1.,1.),(1.,1.),(1.,1.),(1.,
1.),(1.,1.)))
REPRESENTATION_ITEM('')
SURFACE()
);
#129=(
BOUNDED_SURFACE()
B_SPLINE_SURFACE(5,1,((#61872,#61873),(#61874,#61875),(#61876,#61877),(#61878,
#61879),(#61880,#61881),(#61882,#61883),(#61884,#61885),(#61886,#61887),
(#61888,#61889),(#61890,#61891),(#61892,#61893),(#61894,#61895),(#61896,
#61897),(#61898,#61899),(#61900,#61901),(#61902,#61903),(#61904,#61905),
(#61906,#61907),(#61908,#61909),(#61910,#61911),(#61912,#61913),(#61914,
#61915),(#61916,#61917),(#61918,#61919),(#61920,#61921),(#61922,#61923),
(#61924,#61925),(#61926,#61927),(#61928,#61929),(#61930,#61931),(#61932,
#61933),(#61934,#61935),(#61936,#61937),(#61938,#61939),(#61940,#61941),
(#61942,#61943),(#61944,#61945),(#61946,#61947),(#61948,#61949),(#61950,
#61951),(#61952,#61953),(#61954,#61955),(#61956,#61957),(#61958,#61959),
(#61960,#61961),(#61962,#61963),(#61964,#61965),(#61966,#61967),(#61968,
#61969),(#61970,#61971),(#61972,#61973),(#61974,#61975),(#61976,#61977),
(#61978,#61979),(#61980,#61981),(#61982,#61983),(#61984,#61985),(#61986,
#61987),(#61988,#61989),(#61990,#61991),(#61992,#61993),(#61994,#61995),
(#61996,#61997),(#61998,#61999),(#62000,#62001),(#62002,#62003),(#62004,
#62005),(#62006,#62007),(#62008,#62009),(#62010,#62011)),.UNSPECIFIED.,
 .F.,.F.,.F.)
B_SPLINE_SURFACE_WITH_KNOTS((6,1,1,1,1,1,1,1,1,1,1,1,1,1,1,1,1,1,1,1,1,
1,1,1,1,1,1,1,1,1,1,1,1,1,1,1,1,1,1,1,1,1,1,1,1,1,1,1,1,1,1,1,1,1,1,1,1,
1,1,1,1,1,1,1,1,6),(2,2),(-1.,-0.984615384615383,-0.969230769230768,-0.953846153846152,
-0.938461538461537,-0.923076923076922,-0.907692307692306,-0.892307692307691,
-0.876923076923076,-0.86153846153846,-0.846153846153845,-0.83076923076923,
-0.815384615384614,-0.799999999999999,-0.784615384615384,-0.769230769230768,
-0.753846153846153,-0.738461538461538,-0.723076923076922,-0.707692307692307,
-0.692307692307692,-0.676923076923076,-0.661538461538461,-0.646153846153846,
-0.63076923076923,-0.615384615384615,-0.6,-0.584615384615384,-0.569230769230769,
-0.553846153846154,-0.538461538461538,-0.523076923076923,-0.507692307692308,
-0.492307692307692,-0.476923076923077,-0.461538461538462,-0.446153846153846,
-0.430769230769231,-0.415384615384615,-0.4,-0.384615384615385,-0.369230769230769,
-0.353846153846154,-0.338461538461538,-0.323076923076923,-0.307692307692308,
-0.292307692307692,-0.276923076923077,-0.261538461538462,-0.246153846153846,
-0.230769230769231,-0.215384615384615,-0.2,-0.184615384615385,-0.169230769230769,
-0.153846153846154,-0.138461538461538,-0.123076923076923,-0.107692307692308,
-0.0923076923076923,-0.0769230769230769,-0.0615384615384615,-0.0461538461538462,
-0.0307692307692308,-0.0153846153846154,0.),(-1.,1.),.UNSPECIFIED.)
GEOMETRIC_REPRESENTATION_ITEM()
RATIONAL_B_SPLINE_SURFACE(((1.,1.),(1.,1.),(1.,1.),(1.,1.),(1.,1.),(1.,
1.),(1.,1.),(1.,1.),(1.,1.),(1.,1.),(1.,1.),(1.,1.),(1.,1.),(1.,1.),(1.,
1.),(1.,1.),(1.,1.),(1.,1.),(1.,1.),(1.,1.),(1.,1.),(1.,1.),(1.,1.),(1.,
1.),(1.,1.),(1.,1.),(1.,1.),(1.,1.),(1.,1.),(1.,1.),(1.,1.),(1.,1.),(1.,
1.),(1.,1.),(1.,1.),(1.,1.),(1.,1.),(1.,1.),(1.,1.),(1.,1.),(1.,1.),(1.,
1.),(1.,1.),(1.,1.),(1.,1.),(1.,1.),(1.,1.),(1.,1.),(1.,1.),(1.,1.),(1.,
1.),(1.,1.),(1.,1.),(1.,1.),(1.,1.),(1.,1.),(1.,1.),(1.,1.),(1.,1.),(1.,
1.),(1.,1.),(1.,1.),(1.,1.),(1.,1.),(1.,1.),(1.,1.),(1.,1.),(1.,1.),(1.,
1.),(1.,1.)))
REPRESENTATION_ITEM('')
SURFACE()
);
#130=(
BOUNDED_SURFACE()
B_SPLINE_SURFACE(5,1,((#62091,#62092),(#62093,#62094),(#62095,#62096),(#62097,
#62098),(#62099,#62100),(#62101,#62102),(#62103,#62104),(#62105,#62106),
(#62107,#62108),(#62109,#62110),(#62111,#62112),(#62113,#62114),(#62115,
#62116),(#62117,#62118),(#62119,#62120),(#62121,#62122),(#62123,#62124),
(#62125,#62126),(#62127,#62128),(#62129,#62130),(#62131,#62132),(#62133,
#62134),(#62135,#62136),(#62137,#62138),(#62139,#62140),(#62141,#62142),
(#62143,#62144),(#62145,#62146),(#62147,#62148),(#62149,#62150),(#62151,
#62152),(#62153,#62154),(#62155,#62156),(#62157,#62158),(#62159,#62160),
(#62161,#62162),(#62163,#62164),(#62165,#62166),(#62167,#62168),(#62169,
#62170),(#62171,#62172),(#62173,#62174),(#62175,#62176),(#62177,#62178),
(#62179,#62180),(#62181,#62182),(#62183,#62184),(#62185,#62186),(#62187,
#62188),(#62189,#62190),(#62191,#62192),(#62193,#62194),(#62195,#62196),
(#62197,#62198),(#62199,#62200),(#62201,#62202),(#62203,#62204),(#62205,
#62206),(#62207,#62208),(#62209,#62210),(#62211,#62212),(#62213,#62214),
(#62215,#62216),(#62217,#62218),(#62219,#62220),(#62221,#62222),(#62223,
#62224),(#62225,#62226),(#62227,#62228),(#62229,#62230)),.UNSPECIFIED.,
 .F.,.F.,.F.)
B_SPLINE_SURFACE_WITH_KNOTS((6,1,1,1,1,1,1,1,1,1,1,1,1,1,1,1,1,1,1,1,1,
1,1,1,1,1,1,1,1,1,1,1,1,1,1,1,1,1,1,1,1,1,1,1,1,1,1,1,1,1,1,1,1,1,1,1,1,
1,1,1,1,1,1,1,1,6),(2,2),(-1.,-0.984615384615383,-0.969230769230768,-0.953846153846152,
-0.938461538461537,-0.923076923076922,-0.907692307692306,-0.892307692307691,
-0.876923076923076,-0.86153846153846,-0.846153846153845,-0.83076923076923,
-0.815384615384614,-0.799999999999999,-0.784615384615384,-0.769230769230768,
-0.753846153846153,-0.738461538461538,-0.723076923076922,-0.707692307692307,
-0.692307692307692,-0.676923076923076,-0.661538461538461,-0.646153846153846,
-0.63076923076923,-0.615384615384615,-0.6,-0.584615384615384,-0.569230769230769,
-0.553846153846154,-0.538461538461538,-0.523076923076923,-0.507692307692308,
-0.492307692307692,-0.476923076923077,-0.461538461538462,-0.446153846153846,
-0.430769230769231,-0.415384615384615,-0.4,-0.384615384615385,-0.369230769230769,
-0.353846153846154,-0.338461538461538,-0.323076923076923,-0.307692307692308,
-0.292307692307692,-0.276923076923077,-0.261538461538462,-0.246153846153846,
-0.230769230769231,-0.215384615384615,-0.2,-0.184615384615385,-0.169230769230769,
-0.153846153846154,-0.138461538461538,-0.123076923076923,-0.107692307692308,
-0.0923076923076923,-0.0769230769230769,-0.0615384615384615,-0.0461538461538462,
-0.0307692307692308,-0.0153846153846154,0.),(-1.,1.),.UNSPECIFIED.)
GEOMETRIC_REPRESENTATION_ITEM()
RATIONAL_B_SPLINE_SURFACE(((1.,1.),(1.,1.),(1.,1.),(1.,1.),(1.,1.),(1.,
1.),(1.,1.),(1.,1.),(1.,1.),(1.,1.),(1.,1.),(1.,1.),(1.,1.),(1.,1.),(1.,
1.),(1.,1.),(1.,1.),(1.,1.),(1.,1.),(1.,1.),(1.,1.),(1.,1.),(1.,1.),(1.,
1.),(1.,1.),(1.,1.),(1.,1.),(1.,1.),(1.,1.),(1.,1.),(1.,1.),(1.,1.),(1.,
1.),(1.,1.),(1.,1.),(1.,1.),(1.,1.),(1.,1.),(1.,1.),(1.,1.),(1.,1.),(1.,
1.),(1.,1.),(1.,1.),(1.,1.),(1.,1.),(1.,1.),(1.,1.),(1.,1.),(1.,1.),(1.,
1.),(1.,1.),(1.,1.),(1.,1.),(1.,1.),(1.,1.),(1.,1.),(1.,1.),(1.,1.),(1.,
1.),(1.,1.),(1.,1.),(1.,1.),(1.,1.),(1.,1.),(1.,1.),(1.,1.),(1.,1.),(1.,
1.),(1.,1.)))
REPRESENTATION_ITEM('')
SURFACE()
);
#211=(
BOUNDED_CURVE()
B_SPLINE_CURVE(5,(#38781,#38782,#38783,#38784,#38785,#38786,#38787,#38788,
#38789,#38790,#38791,#38792,#38793,#38794,#38795,#38796,#38797,#38798,#38799,
#38800,#38801,#38802,#38803,#38804,#38805,#38806,#38807,#38808,#38809,#38810,
#38811,#38812,#38813,#38814,#38815,#38816,#38817,#38818,#38819,#38820,#38821,
#38822,#38823,#38824,#38825,#38826,#38827,#38828,#38829,#38830,#38831,#38832,
#38833,#38834,#38835,#38836,#38837,#38838,#38839,#38840,#38841,#38842,#38843,
#38844,#38845,#38846,#38847,#38848,#38849,#38850),.UNSPECIFIED.,.F.,.F.)
B_SPLINE_CURVE_WITH_KNOTS((6,1,1,1,1,1,1,1,1,1,1,1,1,1,1,1,1,1,1,1,1,1,
1,1,1,1,1,1,1,1,1,1,1,1,1,1,1,1,1,1,1,1,1,1,1,1,1,1,1,1,1,1,1,1,1,1,1,1,
1,1,1,1,1,1,1,6),(0.00577184337450058,0.0153846153846154,0.0307692307692308,
0.0461538461538462,0.0615384615384615,0.0769230769230769,0.0923076923076923,
0.107692307692308,0.123076923076923,0.138461538461538,0.153846153846154,
0.169230769230769,0.184615384615385,0.2,0.215384615384615,0.230769230769231,
0.246153846153846,0.261538461538462,0.276923076923077,0.292307692307692,
0.307692307692308,0.323076923076923,0.338461538461538,0.353846153846154,
0.369230769230769,0.384615384615385,0.4,0.415384615384615,0.430769230769231,
0.446153846153846,0.461538461538462,0.476923076923077,0.492307692307692,
0.507692307692308,0.523076923076923,0.538461538461538,0.553846153846154,
0.569230769230769,0.584615384615384,0.6,0.615384615384615,0.63076923076923,
0.646153846153846,0.661538461538461,0.676923076923076,0.692307692307692,
0.707692307692307,0.723076923076922,0.738461538461538,0.753846153846153,
0.769230769230768,0.784615384615384,0.799999999999999,0.815384615384614,
0.83076923076923,0.846153846153845,0.86153846153846,0.876923076923076,0.892307692307691,
0.907692307692306,0.923076923076922,0.938461538461537,0.953846153846152,
0.969230769230768,0.984615384615383,1.),.UNSPECIFIED.)
CURVE()
GEOMETRIC_REPRESENTATION_ITEM()
RATIONAL_B_SPLINE_CURVE((1.,1.,1.,1.,1.,1.,1.,1.,1.,1.,1.,1.,1.,1.,1.,1.,
1.,1.,1.,1.,1.,1.,1.,1.,1.,1.,1.,1.,1.,1.,1.,1.,1.,1.,1.,1.,1.,1.,1.,1.,
1.,1.,1.,1.,1.,1.,1.,1.,1.,1.,1.,1.,1.,1.,1.,1.,1.,1.,1.,1.,1.,1.,1.,1.,
1.,1.,1.,1.,1.,1.))
REPRESENTATION_ITEM('')
);
#212=(
BOUNDED_CURVE()
B_SPLINE_CURVE(5,(#38854,#38855,#38856,#38857,#38858,#38859,#38860,#38861,
#38862,#38863,#38864,#38865,#38866,#38867,#38868,#38869,#38870,#38871,#38872,
#38873,#38874,#38875,#38876,#38877,#38878,#38879,#38880,#38881,#38882,#38883,
#38884,#38885,#38886,#38887,#38888,#38889,#38890,#38891,#38892,#38893,#38894,
#38895,#38896,#38897,#38898,#38899,#38900,#38901,#38902,#38903,#38904,#38905,
#38906,#38907,#38908,#38909,#38910,#38911,#38912,#38913,#38914,#38915,#38916,
#38917,#38918,#38919,#38920,#38921,#38922,#38923),.UNSPECIFIED.,.F.,.F.)
B_SPLINE_CURVE_WITH_KNOTS((6,1,1,1,1,1,1,1,1,1,1,1,1,1,1,1,1,1,1,1,1,1,
1,1,1,1,1,1,1,1,1,1,1,1,1,1,1,1,1,1,1,1,1,1,1,1,1,1,1,1,1,1,1,1,1,1,1,1,
1,1,1,1,1,1,1,6),(0.,0.0153846153846154,0.0307692307692308,0.0461538461538462,
0.0615384615384615,0.0769230769230769,0.0923076923076923,0.107692307692308,
0.123076923076923,0.138461538461538,0.153846153846154,0.169230769230769,
0.184615384615385,0.2,0.215384615384615,0.230769230769231,0.246153846153846,
0.261538461538462,0.276923076923077,0.292307692307692,0.307692307692308,
0.323076923076923,0.338461538461538,0.353846153846154,0.369230769230769,
0.384615384615385,0.4,0.415384615384615,0.430769230769231,0.446153846153846,
0.461538461538462,0.476923076923077,0.492307692307692,0.507692307692308,
0.523076923076923,0.538461538461538,0.553846153846154,0.569230769230769,
0.584615384615384,0.6,0.615384615384615,0.63076923076923,0.646153846153846,
0.661538461538461,0.676923076923076,0.692307692307692,0.707692307692307,
0.723076923076922,0.738461538461538,0.753846153846153,0.769230769230768,
0.784615384615384,0.799999999999999,0.815384615384614,0.83076923076923,
0.846153846153845,0.86153846153846,0.876923076923076,0.892307692307691,
0.907692307692306,0.923076923076922,0.938461538461537,0.953846153846152,
0.969230769230768,0.984615384615383,0.994228156739708),.UNSPECIFIED.)
CURVE()
GEOMETRIC_REPRESENTATION_ITEM()
RATIONAL_B_SPLINE_CURVE((1.,1.,1.,1.,1.,1.,1.,1.,1.,1.,1.,1.,1.,1.,1.,1.,
1.,1.,1.,1.,1.,1.,1.,1.,1.,1.,1.,1.,1.,1.,1.,1.,1.,1.,1.,1.,1.,1.,1.,1.,
1.,1.,1.,1.,1.,1.,1.,1.,1.,1.,1.,1.,1.,1.,1.,1.,1.,1.,1.,1.,1.,1.,1.,1.,
1.,1.,1.,1.,1.,1.))
REPRESENTATION_ITEM('')
);
#213=(
BOUNDED_CURVE()
B_SPLINE_CURVE(5,(#38927,#38928,#38929,#38930,#38931,#38932,#38933,#38934,
#38935,#38936,#38937,#38938,#38939,#38940,#38941,#38942,#38943,#38944,#38945,
#38946,#38947,#38948,#38949,#38950,#38951,#38952,#38953,#38954,#38955,#38956,
#38957,#38958,#38959,#38960,#38961,#38962,#38963,#38964,#38965,#38966,#38967,
#38968,#38969,#38970,#38971,#38972,#38973,#38974,#38975,#38976,#38977,#38978,
#38979,#38980,#38981,#38982,#38983,#38984,#38985,#38986,#38987,#38988,#38989,
#38990,#38991,#38992,#38993,#38994,#38995,#38996),.UNSPECIFIED.,.F.,.F.)
B_SPLINE_CURVE_WITH_KNOTS((6,1,1,1,1,1,1,1,1,1,1,1,1,1,1,1,1,1,1,1,1,1,
1,1,1,1,1,1,1,1,1,1,1,1,1,1,1,1,1,1,1,1,1,1,1,1,1,1,1,1,1,1,1,1,1,1,1,1,
1,1,1,1,1,1,1,6),(0.0057718433745091,0.0153846153846154,0.0307692307692308,
0.0461538461538462,0.0615384615384615,0.0769230769230769,0.0923076923076923,
0.107692307692308,0.123076923076923,0.138461538461538,0.153846153846154,
0.169230769230769,0.184615384615385,0.2,0.215384615384615,0.230769230769231,
0.246153846153846,0.261538461538462,0.276923076923077,0.292307692307692,
0.307692307692308,0.323076923076923,0.338461538461538,0.353846153846154,
0.369230769230769,0.384615384615385,0.4,0.415384615384615,0.430769230769231,
0.446153846153846,0.461538461538462,0.476923076923077,0.492307692307692,
0.507692307692308,0.523076923076923,0.538461538461538,0.553846153846154,
0.569230769230769,0.584615384615384,0.6,0.615384615384615,0.63076923076923,
0.646153846153846,0.661538461538461,0.676923076923076,0.692307692307692,
0.707692307692307,0.723076923076922,0.738461538461538,0.753846153846153,
0.769230769230768,0.784615384615384,0.799999999999999,0.815384615384614,
0.83076923076923,0.846153846153845,0.86153846153846,0.876923076923076,0.892307692307691,
0.907692307692306,0.923076923076922,0.938461538461537,0.953846153846152,
0.969230769230768,0.984615384615383,1.),.UNSPECIFIED.)
CURVE()
GEOMETRIC_REPRESENTATION_ITEM()
RATIONAL_B_SPLINE_CURVE((1.,1.,1.,1.,1.,1.,1.,1.,1.,1.,1.,1.,1.,1.,1.,1.,
1.,1.,1.,1.,1.,1.,1.,1.,1.,1.,1.,1.,1.,1.,1.,1.,1.,1.,1.,1.,1.,1.,1.,1.,
1.,1.,1.,1.,1.,1.,1.,1.,1.,1.,1.,1.,1.,1.,1.,1.,1.,1.,1.,1.,1.,1.,1.,1.,
1.,1.,1.,1.,1.,1.))
REPRESENTATION_ITEM('')
);
#214=(
BOUNDED_CURVE()
B_SPLINE_CURVE(5,(#39000,#39001,#39002,#39003,#39004,#39005,#39006,#39007,
#39008,#39009,#39010,#39011,#39012,#39013,#39014,#39015,#39016,#39017,#39018,
#39019,#39020,#39021,#39022,#39023,#39024,#39025,#39026,#39027,#39028,#39029,
#39030,#39031,#39032,#39033,#39034,#39035,#39036,#39037,#39038,#39039,#39040,
#39041,#39042,#39043,#39044,#39045,#39046,#39047,#39048,#39049,#39050,#39051,
#39052,#39053,#39054,#39055,#39056,#39057,#39058,#39059,#39060,#39061,#39062,
#39063,#39064,#39065,#39066,#39067,#39068,#39069),.UNSPECIFIED.,.F.,.F.)
B_SPLINE_CURVE_WITH_KNOTS((6,1,1,1,1,1,1,1,1,1,1,1,1,1,1,1,1,1,1,1,1,1,
1,1,1,1,1,1,1,1,1,1,1,1,1,1,1,1,1,1,1,1,1,1,1,1,1,1,1,1,1,1,1,1,1,1,1,1,
1,1,1,1,1,1,1,6),(0.,0.0153846153846154,0.0307692307692308,0.0461538461538462,
0.0615384615384615,0.0769230769230769,0.0923076923076923,0.107692307692308,
0.123076923076923,0.138461538461538,0.153846153846154,0.169230769230769,
0.184615384615385,0.2,0.215384615384615,0.230769230769231,0.246153846153846,
0.261538461538462,0.276923076923077,0.292307692307692,0.307692307692308,
0.323076923076923,0.338461538461538,0.353846153846154,0.369230769230769,
0.384615384615385,0.4,0.415384615384615,0.430769230769231,0.446153846153846,
0.461538461538462,0.476923076923077,0.492307692307692,0.507692307692308,
0.523076923076923,0.538461538461538,0.553846153846154,0.569230769230769,
0.584615384615384,0.6,0.615384615384615,0.63076923076923,0.646153846153846,
0.661538461538461,0.676923076923076,0.692307692307692,0.707692307692307,
0.723076923076922,0.738461538461538,0.753846153846153,0.769230769230768,
0.784615384615384,0.799999999999999,0.815384615384614,0.83076923076923,
0.846153846153845,0.86153846153846,0.876923076923076,0.892307692307691,
0.907692307692306,0.923076923076922,0.938461538461537,0.953846153846152,
0.969230769230768,0.984615384615383,0.994228156739689),.UNSPECIFIED.)
CURVE()
GEOMETRIC_REPRESENTATION_ITEM()
RATIONAL_B_SPLINE_CURVE((1.,1.,1.,1.,1.,1.,1.,1.,1.,1.,1.,1.,1.,1.,1.,1.,
1.,1.,1.,1.,1.,1.,1.,1.,1.,1.,1.,1.,1.,1.,1.,1.,1.,1.,1.,1.,1.,1.,1.,1.,
1.,1.,1.,1.,1.,1.,1.,1.,1.,1.,1.,1.,1.,1.,1.,1.,1.,1.,1.,1.,1.,1.,1.,1.,
1.,1.,1.,1.,1.,1.))
REPRESENTATION_ITEM('')
);
#215=(
BOUNDED_CURVE()
B_SPLINE_CURVE(5,(#39073,#39074,#39075,#39076,#39077,#39078,#39079,#39080,
#39081,#39082,#39083,#39084,#39085,#39086,#39087,#39088,#39089,#39090,#39091,
#39092,#39093,#39094,#39095,#39096,#39097,#39098,#39099,#39100,#39101,#39102,
#39103,#39104,#39105,#39106,#39107,#39108,#39109,#39110,#39111,#39112,#39113,
#39114,#39115,#39116,#39117,#39118,#39119,#39120,#39121,#39122,#39123,#39124,
#39125,#39126,#39127,#39128,#39129,#39130,#39131,#39132,#39133,#39134,#39135,
#39136,#39137,#39138,#39139,#39140,#39141,#39142),.UNSPECIFIED.,.F.,.F.)
B_SPLINE_CURVE_WITH_KNOTS((6,1,1,1,1,1,1,1,1,1,1,1,1,1,1,1,1,1,1,1,1,1,
1,1,1,1,1,1,1,1,1,1,1,1,1,1,1,1,1,1,1,1,1,1,1,1,1,1,1,1,1,1,1,1,1,1,1,1,
1,1,1,1,1,1,1,6),(0.00577184337448946,0.0153846153846154,0.0307692307692308,
0.0461538461538462,0.0615384615384615,0.0769230769230769,0.0923076923076923,
0.107692307692308,0.123076923076923,0.138461538461538,0.153846153846154,
0.169230769230769,0.184615384615385,0.2,0.215384615384615,0.230769230769231,
0.246153846153846,0.261538461538462,0.276923076923077,0.292307692307692,
0.307692307692308,0.323076923076923,0.338461538461538,0.353846153846154,
0.369230769230769,0.384615384615385,0.4,0.415384615384615,0.430769230769231,
0.446153846153846,0.461538461538462,0.476923076923077,0.492307692307692,
0.507692307692308,0.523076923076923,0.538461538461538,0.553846153846154,
0.569230769230769,0.584615384615384,0.6,0.615384615384615,0.63076923076923,
0.646153846153846,0.661538461538461,0.676923076923076,0.692307692307692,
0.707692307692307,0.723076923076922,0.738461538461538,0.753846153846153,
0.769230769230768,0.784615384615384,0.799999999999999,0.815384615384614,
0.83076923076923,0.846153846153845,0.86153846153846,0.876923076923076,0.892307692307691,
0.907692307692306,0.923076923076922,0.938461538461537,0.953846153846152,
0.969230769230768,0.984615384615383,1.),.UNSPECIFIED.)
CURVE()
GEOMETRIC_REPRESENTATION_ITEM()
RATIONAL_B_SPLINE_CURVE((1.,1.,1.,1.,1.,1.,1.,1.,1.,1.,1.,1.,1.,1.,1.,1.,
1.,1.,1.,1.,1.,1.,1.,1.,1.,1.,1.,1.,1.,1.,1.,1.,1.,1.,1.,1.,1.,1.,1.,1.,
1.,1.,1.,1.,1.,1.,1.,1.,1.,1.,1.,1.,1.,1.,1.,1.,1.,1.,1.,1.,1.,1.,1.,1.,
1.,1.,1.,1.,1.,1.))
REPRESENTATION_ITEM('')
);
#216=(
BOUNDED_CURVE()
B_SPLINE_CURVE(5,(#39146,#39147,#39148,#39149,#39150,#39151,#39152,#39153,
#39154,#39155,#39156,#39157,#39158,#39159,#39160,#39161,#39162,#39163,#39164,
#39165,#39166,#39167,#39168,#39169,#39170,#39171,#39172,#39173,#39174,#39175,
#39176,#39177,#39178,#39179,#39180,#39181,#39182,#39183,#39184,#39185,#39186,
#39187,#39188,#39189,#39190,#39191,#39192,#39193,#39194,#39195,#39196,#39197,
#39198,#39199,#39200,#39201,#39202,#39203,#39204,#39205,#39206,#39207,#39208,
#39209,#39210,#39211,#39212,#39213,#39214,#39215),.UNSPECIFIED.,.F.,.F.)
B_SPLINE_CURVE_WITH_KNOTS((6,1,1,1,1,1,1,1,1,1,1,1,1,1,1,1,1,1,1,1,1,1,
1,1,1,1,1,1,1,1,1,1,1,1,1,1,1,1,1,1,1,1,1,1,1,1,1,1,1,1,1,1,1,1,1,1,1,1,
1,1,1,1,1,1,1,6),(0.,0.0153846153846154,0.0307692307692308,0.0461538461538462,
0.0615384615384615,0.0769230769230769,0.0923076923076923,0.107692307692308,
0.123076923076923,0.138461538461538,0.153846153846154,0.169230769230769,
0.184615384615385,0.2,0.215384615384615,0.230769230769231,0.246153846153846,
0.261538461538462,0.276923076923077,0.292307692307692,0.307692307692308,
0.323076923076923,0.338461538461538,0.353846153846154,0.369230769230769,
0.384615384615385,0.4,0.415384615384615,0.430769230769231,0.446153846153846,
0.461538461538462,0.476923076923077,0.492307692307692,0.507692307692308,
0.523076923076923,0.538461538461538,0.553846153846154,0.569230769230769,
0.584615384615384,0.6,0.615384615384615,0.63076923076923,0.646153846153846,
0.661538461538461,0.676923076923076,0.692307692307692,0.707692307692307,
0.723076923076922,0.738461538461538,0.753846153846153,0.769230769230768,
0.784615384615384,0.799999999999999,0.815384615384614,0.83076923076923,
0.846153846153845,0.86153846153846,0.876923076923076,0.892307692307691,
0.907692307692306,0.923076923076922,0.938461538461537,0.953846153846152,
0.969230769230768,0.984615384615383,0.994228156739718),.UNSPECIFIED.)
CURVE()
GEOMETRIC_REPRESENTATION_ITEM()
RATIONAL_B_SPLINE_CURVE((1.,1.,1.,1.,1.,1.,1.,1.,1.,1.,1.,1.,1.,1.,1.,1.,
1.,1.,1.,1.,1.,1.,1.,1.,1.,1.,1.,1.,1.,1.,1.,1.,1.,1.,1.,1.,1.,1.,1.,1.,
1.,1.,1.,1.,1.,1.,1.,1.,1.,1.,1.,1.,1.,1.,1.,1.,1.,1.,1.,1.,1.,1.,1.,1.,
1.,1.,1.,1.,1.,1.))
REPRESENTATION_ITEM('')
);
#217=(
BOUNDED_CURVE()
B_SPLINE_CURVE(5,(#39219,#39220,#39221,#39222,#39223,#39224,#39225,#39226,
#39227,#39228,#39229,#39230,#39231,#39232,#39233,#39234,#39235,#39236,#39237,
#39238,#39239,#39240,#39241,#39242,#39243,#39244,#39245,#39246,#39247,#39248,
#39249,#39250,#39251,#39252,#39253,#39254,#39255,#39256,#39257,#39258,#39259,
#39260,#39261,#39262,#39263,#39264,#39265,#39266,#39267,#39268,#39269,#39270,
#39271,#39272,#39273,#39274,#39275,#39276,#39277,#39278,#39279,#39280,#39281,
#39282,#39283,#39284,#39285,#39286,#39287,#39288),.UNSPECIFIED.,.F.,.F.)
B_SPLINE_CURVE_WITH_KNOTS((6,1,1,1,1,1,1,1,1,1,1,1,1,1,1,1,1,1,1,1,1,1,
1,1,1,1,1,1,1,1,1,1,1,1,1,1,1,1,1,1,1,1,1,1,1,1,1,1,1,1,1,1,1,1,1,1,1,1,
1,1,1,1,1,1,1,6),(0.00577184337450897,0.0153846153846154,0.0307692307692308,
0.0461538461538462,0.0615384615384615,0.0769230769230769,0.0923076923076923,
0.107692307692308,0.123076923076923,0.138461538461538,0.153846153846154,
0.169230769230769,0.184615384615385,0.2,0.215384615384615,0.230769230769231,
0.246153846153846,0.261538461538462,0.276923076923077,0.292307692307692,
0.307692307692308,0.323076923076923,0.338461538461538,0.353846153846154,
0.369230769230769,0.384615384615385,0.4,0.415384615384615,0.430769230769231,
0.446153846153846,0.461538461538462,0.476923076923077,0.492307692307692,
0.507692307692308,0.523076923076923,0.538461538461538,0.553846153846154,
0.569230769230769,0.584615384615384,0.6,0.615384615384615,0.63076923076923,
0.646153846153846,0.661538461538461,0.676923076923076,0.692307692307692,
0.707692307692307,0.723076923076922,0.738461538461538,0.753846153846153,
0.769230769230768,0.784615384615384,0.799999999999999,0.815384615384614,
0.83076923076923,0.846153846153845,0.86153846153846,0.876923076923076,0.892307692307691,
0.907692307692306,0.923076923076922,0.938461538461537,0.953846153846152,
0.969230769230768,0.984615384615383,1.),.UNSPECIFIED.)
CURVE()
GEOMETRIC_REPRESENTATION_ITEM()
RATIONAL_B_SPLINE_CURVE((1.,1.,1.,1.,1.,1.,1.,1.,1.,1.,1.,1.,1.,1.,1.,1.,
1.,1.,1.,1.,1.,1.,1.,1.,1.,1.,1.,1.,1.,1.,1.,1.,1.,1.,1.,1.,1.,1.,1.,1.,
1.,1.,1.,1.,1.,1.,1.,1.,1.,1.,1.,1.,1.,1.,1.,1.,1.,1.,1.,1.,1.,1.,1.,1.,
1.,1.,1.,1.,1.,1.))
REPRESENTATION_ITEM('')
);
#218=(
BOUNDED_CURVE()
B_SPLINE_CURVE(5,(#39292,#39293,#39294,#39295,#39296,#39297,#39298,#39299,
#39300,#39301,#39302,#39303,#39304,#39305,#39306,#39307,#39308,#39309,#39310,
#39311,#39312,#39313,#39314,#39315,#39316,#39317,#39318,#39319,#39320,#39321,
#39322,#39323,#39324,#39325,#39326,#39327,#39328,#39329,#39330,#39331,#39332,
#39333,#39334,#39335,#39336,#39337,#39338,#39339,#39340,#39341,#39342,#39343,
#39344,#39345,#39346,#39347,#39348,#39349,#39350,#39351,#39352,#39353,#39354,
#39355,#39356,#39357,#39358,#39359,#39360,#39361),.UNSPECIFIED.,.F.,.F.)
B_SPLINE_CURVE_WITH_KNOTS((6,1,1,1,1,1,1,1,1,1,1,1,1,1,1,1,1,1,1,1,1,1,
1,1,1,1,1,1,1,1,1,1,1,1,1,1,1,1,1,1,1,1,1,1,1,1,1,1,1,1,1,1,1,1,1,1,1,1,
1,1,1,1,1,1,1,6),(0.,0.0153846153846154,0.0307692307692308,0.0461538461538462,
0.0615384615384615,0.0769230769230769,0.0923076923076923,0.107692307692308,
0.123076923076923,0.138461538461538,0.153846153846154,0.169230769230769,
0.184615384615385,0.2,0.215384615384615,0.230769230769231,0.246153846153846,
0.261538461538462,0.276923076923077,0.292307692307692,0.307692307692308,
0.323076923076923,0.338461538461538,0.353846153846154,0.369230769230769,
0.384615384615385,0.4,0.415384615384615,0.430769230769231,0.446153846153846,
0.461538461538462,0.476923076923077,0.492307692307692,0.507692307692308,
0.523076923076923,0.538461538461538,0.553846153846154,0.569230769230769,
0.584615384615384,0.6,0.615384615384615,0.63076923076923,0.646153846153846,
0.661538461538461,0.676923076923076,0.692307692307692,0.707692307692307,
0.723076923076922,0.738461538461538,0.753846153846153,0.769230769230768,
0.784615384615384,0.799999999999999,0.815384615384614,0.83076923076923,
0.846153846153845,0.86153846153846,0.876923076923076,0.892307692307691,
0.907692307692306,0.923076923076922,0.938461538461537,0.953846153846152,
0.969230769230768,0.984615384615383,0.994228156739701),.UNSPECIFIED.)
CURVE()
GEOMETRIC_REPRESENTATION_ITEM()
RATIONAL_B_SPLINE_CURVE((1.,1.,1.,1.,1.,1.,1.,1.,1.,1.,1.,1.,1.,1.,1.,1.,
1.,1.,1.,1.,1.,1.,1.,1.,1.,1.,1.,1.,1.,1.,1.,1.,1.,1.,1.,1.,1.,1.,1.,1.,
1.,1.,1.,1.,1.,1.,1.,1.,1.,1.,1.,1.,1.,1.,1.,1.,1.,1.,1.,1.,1.,1.,1.,1.,
1.,1.,1.,1.,1.,1.))
REPRESENTATION_ITEM('')
);
#219=(
BOUNDED_CURVE()
B_SPLINE_CURVE(5,(#39365,#39366,#39367,#39368,#39369,#39370,#39371,#39372,
#39373,#39374,#39375,#39376,#39377,#39378,#39379,#39380,#39381,#39382,#39383,
#39384,#39385,#39386,#39387,#39388,#39389,#39390,#39391,#39392,#39393,#39394,
#39395,#39396,#39397,#39398,#39399,#39400,#39401,#39402,#39403,#39404,#39405,
#39406,#39407,#39408,#39409,#39410,#39411,#39412,#39413,#39414,#39415,#39416,
#39417,#39418,#39419,#39420,#39421,#39422,#39423,#39424,#39425,#39426,#39427,
#39428,#39429,#39430,#39431,#39432,#39433,#39434),.UNSPECIFIED.,.F.,.F.)
B_SPLINE_CURVE_WITH_KNOTS((6,1,1,1,1,1,1,1,1,1,1,1,1,1,1,1,1,1,1,1,1,1,
1,1,1,1,1,1,1,1,1,1,1,1,1,1,1,1,1,1,1,1,1,1,1,1,1,1,1,1,1,1,1,1,1,1,1,1,
1,1,1,1,1,1,1,6),(0.00577184337451001,0.0153846153846154,0.0307692307692308,
0.0461538461538462,0.0615384615384615,0.0769230769230769,0.0923076923076923,
0.107692307692308,0.123076923076923,0.138461538461538,0.153846153846154,
0.169230769230769,0.184615384615385,0.2,0.215384615384615,0.230769230769231,
0.246153846153846,0.261538461538462,0.276923076923077,0.292307692307692,
0.307692307692308,0.323076923076923,0.338461538461538,0.353846153846154,
0.369230769230769,0.384615384615385,0.4,0.415384615384615,0.430769230769231,
0.446153846153846,0.461538461538462,0.476923076923077,0.492307692307692,
0.507692307692308,0.523076923076923,0.538461538461538,0.553846153846154,
0.569230769230769,0.584615384615384,0.6,0.615384615384615,0.63076923076923,
0.646153846153846,0.661538461538461,0.676923076923076,0.692307692307692,
0.707692307692307,0.723076923076922,0.738461538461538,0.753846153846153,
0.769230769230768,0.784615384615384,0.799999999999999,0.815384615384614,
0.83076923076923,0.846153846153845,0.86153846153846,0.876923076923076,0.892307692307691,
0.907692307692306,0.923076923076922,0.938461538461537,0.953846153846152,
0.969230769230768,0.984615384615383,1.),.UNSPECIFIED.)
CURVE()
GEOMETRIC_REPRESENTATION_ITEM()
RATIONAL_B_SPLINE_CURVE((1.,1.,1.,1.,1.,1.,1.,1.,1.,1.,1.,1.,1.,1.,1.,1.,
1.,1.,1.,1.,1.,1.,1.,1.,1.,1.,1.,1.,1.,1.,1.,1.,1.,1.,1.,1.,1.,1.,1.,1.,
1.,1.,1.,1.,1.,1.,1.,1.,1.,1.,1.,1.,1.,1.,1.,1.,1.,1.,1.,1.,1.,1.,1.,1.,
1.,1.,1.,1.,1.,1.))
REPRESENTATION_ITEM('')
);
#220=(
BOUNDED_CURVE()
B_SPLINE_CURVE(5,(#39438,#39439,#39440,#39441,#39442,#39443,#39444,#39445,
#39446,#39447,#39448,#39449,#39450,#39451,#39452,#39453,#39454,#39455,#39456,
#39457,#39458,#39459,#39460,#39461,#39462,#39463,#39464,#39465,#39466,#39467,
#39468,#39469,#39470,#39471,#39472,#39473,#39474,#39475,#39476,#39477,#39478,
#39479,#39480,#39481,#39482,#39483,#39484,#39485,#39486,#39487,#39488,#39489,
#39490,#39491,#39492,#39493,#39494,#39495,#39496,#39497,#39498,#39499,#39500,
#39501,#39502,#39503,#39504,#39505,#39506,#39507),.UNSPECIFIED.,.F.,.F.)
B_SPLINE_CURVE_WITH_KNOTS((6,1,1,1,1,1,1,1,1,1,1,1,1,1,1,1,1,1,1,1,1,1,
1,1,1,1,1,1,1,1,1,1,1,1,1,1,1,1,1,1,1,1,1,1,1,1,1,1,1,1,1,1,1,1,1,1,1,1,
1,1,1,1,1,1,1,6),(0.,0.0153846153846154,0.0307692307692308,0.0461538461538462,
0.0615384615384615,0.0769230769230769,0.0923076923076923,0.107692307692308,
0.123076923076923,0.138461538461538,0.153846153846154,0.169230769230769,
0.184615384615385,0.2,0.215384615384615,0.230769230769231,0.246153846153846,
0.261538461538462,0.276923076923077,0.292307692307692,0.307692307692308,
0.323076923076923,0.338461538461538,0.353846153846154,0.369230769230769,
0.384615384615385,0.4,0.415384615384615,0.430769230769231,0.446153846153846,
0.461538461538462,0.476923076923077,0.492307692307692,0.507692307692308,
0.523076923076923,0.538461538461538,0.553846153846154,0.569230769230769,
0.584615384615384,0.6,0.615384615384615,0.63076923076923,0.646153846153846,
0.661538461538461,0.676923076923076,0.692307692307692,0.707692307692307,
0.723076923076922,0.738461538461538,0.753846153846153,0.769230769230768,
0.784615384615384,0.799999999999999,0.815384615384614,0.83076923076923,
0.846153846153845,0.86153846153846,0.876923076923076,0.892307692307691,
0.907692307692306,0.923076923076922,0.938461538461537,0.953846153846152,
0.969230769230768,0.984615384615383,0.994228156739697),.UNSPECIFIED.)
CURVE()
GEOMETRIC_REPRESENTATION_ITEM()
RATIONAL_B_SPLINE_CURVE((1.,1.,1.,1.,1.,1.,1.,1.,1.,1.,1.,1.,1.,1.,1.,1.,
1.,1.,1.,1.,1.,1.,1.,1.,1.,1.,1.,1.,1.,1.,1.,1.,1.,1.,1.,1.,1.,1.,1.,1.,
1.,1.,1.,1.,1.,1.,1.,1.,1.,1.,1.,1.,1.,1.,1.,1.,1.,1.,1.,1.,1.,1.,1.,1.,
1.,1.,1.,1.,1.,1.))
REPRESENTATION_ITEM('')
);
#221=(
BOUNDED_CURVE()
B_SPLINE_CURVE(5,(#39511,#39512,#39513,#39514,#39515,#39516,#39517,#39518,
#39519,#39520,#39521,#39522,#39523,#39524,#39525,#39526,#39527,#39528,#39529,
#39530,#39531,#39532,#39533,#39534,#39535,#39536,#39537,#39538,#39539,#39540,
#39541,#39542,#39543,#39544,#39545,#39546,#39547,#39548,#39549,#39550,#39551,
#39552,#39553,#39554,#39555,#39556,#39557,#39558,#39559,#39560,#39561,#39562,
#39563,#39564,#39565,#39566,#39567,#39568,#39569,#39570,#39571,#39572,#39573,
#39574,#39575,#39576,#39577,#39578,#39579,#39580),.UNSPECIFIED.,.F.,.F.)
B_SPLINE_CURVE_WITH_KNOTS((6,1,1,1,1,1,1,1,1,1,1,1,1,1,1,1,1,1,1,1,1,1,
1,1,1,1,1,1,1,1,1,1,1,1,1,1,1,1,1,1,1,1,1,1,1,1,1,1,1,1,1,1,1,1,1,1,1,1,
1,1,1,1,1,1,1,6),(0.00577184337452306,0.0153846153846154,0.0307692307692308,
0.0461538461538462,0.0615384615384615,0.0769230769230769,0.0923076923076923,
0.107692307692308,0.123076923076923,0.138461538461538,0.153846153846154,
0.169230769230769,0.184615384615385,0.2,0.215384615384615,0.230769230769231,
0.246153846153846,0.261538461538462,0.276923076923077,0.292307692307692,
0.307692307692308,0.323076923076923,0.338461538461538,0.353846153846154,
0.369230769230769,0.384615384615385,0.4,0.415384615384615,0.430769230769231,
0.446153846153846,0.461538461538462,0.476923076923077,0.492307692307692,
0.507692307692308,0.523076923076923,0.538461538461538,0.553846153846154,
0.569230769230769,0.584615384615384,0.6,0.615384615384615,0.63076923076923,
0.646153846153846,0.661538461538461,0.676923076923076,0.692307692307692,
0.707692307692307,0.723076923076922,0.738461538461538,0.753846153846153,
0.769230769230768,0.784615384615384,0.799999999999999,0.815384615384614,
0.83076923076923,0.846153846153845,0.86153846153846,0.876923076923076,0.892307692307691,
0.907692307692306,0.923076923076922,0.938461538461537,0.953846153846152,
0.969230769230768,0.984615384615383,1.),.UNSPECIFIED.)
CURVE()
GEOMETRIC_REPRESENTATION_ITEM()
RATIONAL_B_SPLINE_CURVE((1.,1.,1.,1.,1.,1.,1.,1.,1.,1.,1.,1.,1.,1.,1.,1.,
1.,1.,1.,1.,1.,1.,1.,1.,1.,1.,1.,1.,1.,1.,1.,1.,1.,1.,1.,1.,1.,1.,1.,1.,
1.,1.,1.,1.,1.,1.,1.,1.,1.,1.,1.,1.,1.,1.,1.,1.,1.,1.,1.,1.,1.,1.,1.,1.,
1.,1.,1.,1.,1.,1.))
REPRESENTATION_ITEM('')
);
#222=(
BOUNDED_CURVE()
B_SPLINE_CURVE(5,(#39584,#39585,#39586,#39587,#39588,#39589,#39590,#39591,
#39592,#39593,#39594,#39595,#39596,#39597,#39598,#39599,#39600,#39601,#39602,
#39603,#39604,#39605,#39606,#39607,#39608,#39609,#39610,#39611,#39612,#39613,
#39614,#39615,#39616,#39617,#39618,#39619,#39620,#39621,#39622,#39623,#39624,
#39625,#39626,#39627,#39628,#39629,#39630,#39631,#39632,#39633,#39634,#39635,
#39636,#39637,#39638,#39639,#39640,#39641,#39642,#39643,#39644,#39645,#39646,
#39647,#39648,#39649,#39650,#39651,#39652,#39653),.UNSPECIFIED.,.F.,.F.)
B_SPLINE_CURVE_WITH_KNOTS((6,1,1,1,1,1,1,1,1,1,1,1,1,1,1,1,1,1,1,1,1,1,
1,1,1,1,1,1,1,1,1,1,1,1,1,1,1,1,1,1,1,1,1,1,1,1,1,1,1,1,1,1,1,1,1,1,1,1,
1,1,1,1,1,1,1,6),(0.,0.0153846153846154,0.0307692307692308,0.0461538461538462,
0.0615384615384615,0.0769230769230769,0.0923076923076923,0.107692307692308,
0.123076923076923,0.138461538461538,0.153846153846154,0.169230769230769,
0.184615384615385,0.2,0.215384615384615,0.230769230769231,0.246153846153846,
0.261538461538462,0.276923076923077,0.292307692307692,0.307692307692308,
0.323076923076923,0.338461538461538,0.353846153846154,0.369230769230769,
0.384615384615385,0.4,0.415384615384615,0.430769230769231,0.446153846153846,
0.461538461538462,0.476923076923077,0.492307692307692,0.507692307692308,
0.523076923076923,0.538461538461538,0.553846153846154,0.569230769230769,
0.584615384615384,0.6,0.615384615384615,0.63076923076923,0.646153846153846,
0.661538461538461,0.676923076923076,0.692307692307692,0.707692307692307,
0.723076923076922,0.738461538461538,0.753846153846153,0.769230769230768,
0.784615384615384,0.799999999999999,0.815384615384614,0.83076923076923,
0.846153846153845,0.86153846153846,0.876923076923076,0.892307692307691,
0.907692307692306,0.923076923076922,0.938461538461537,0.953846153846152,
0.969230769230768,0.984615384615383,0.994228156739688),.UNSPECIFIED.)
CURVE()
GEOMETRIC_REPRESENTATION_ITEM()
RATIONAL_B_SPLINE_CURVE((1.,1.,1.,1.,1.,1.,1.,1.,1.,1.,1.,1.,1.,1.,1.,1.,
1.,1.,1.,1.,1.,1.,1.,1.,1.,1.,1.,1.,1.,1.,1.,1.,1.,1.,1.,1.,1.,1.,1.,1.,
1.,1.,1.,1.,1.,1.,1.,1.,1.,1.,1.,1.,1.,1.,1.,1.,1.,1.,1.,1.,1.,1.,1.,1.,
1.,1.,1.,1.,1.,1.))
REPRESENTATION_ITEM('')
);
#223=(
BOUNDED_CURVE()
B_SPLINE_CURVE(5,(#39657,#39658,#39659,#39660,#39661,#39662,#39663,#39664,
#39665,#39666,#39667,#39668,#39669,#39670,#39671,#39672,#39673,#39674,#39675,
#39676,#39677,#39678,#39679,#39680,#39681,#39682,#39683,#39684,#39685,#39686,
#39687,#39688,#39689,#39690,#39691,#39692,#39693,#39694,#39695,#39696,#39697,
#39698,#39699,#39700,#39701,#39702,#39703,#39704,#39705,#39706,#39707,#39708,
#39709,#39710,#39711,#39712,#39713,#39714,#39715,#39716,#39717,#39718,#39719,
#39720,#39721,#39722,#39723,#39724,#39725,#39726),.UNSPECIFIED.,.F.,.F.)
B_SPLINE_CURVE_WITH_KNOTS((6,1,1,1,1,1,1,1,1,1,1,1,1,1,1,1,1,1,1,1,1,1,
1,1,1,1,1,1,1,1,1,1,1,1,1,1,1,1,1,1,1,1,1,1,1,1,1,1,1,1,1,1,1,1,1,1,1,1,
1,1,1,1,1,1,1,6),(0.00577184337449862,0.0153846153846154,0.0307692307692308,
0.0461538461538462,0.0615384615384615,0.0769230769230769,0.0923076923076923,
0.107692307692308,0.123076923076923,0.138461538461538,0.153846153846154,
0.169230769230769,0.184615384615385,0.2,0.215384615384615,0.230769230769231,
0.246153846153846,0.261538461538462,0.276923076923077,0.292307692307692,
0.307692307692308,0.323076923076923,0.338461538461538,0.353846153846154,
0.369230769230769,0.384615384615385,0.4,0.415384615384615,0.430769230769231,
0.446153846153846,0.461538461538462,0.476923076923077,0.492307692307692,
0.507692307692308,0.523076923076923,0.538461538461538,0.553846153846154,
0.569230769230769,0.584615384615384,0.6,0.615384615384615,0.63076923076923,
0.646153846153846,0.661538461538461,0.676923076923076,0.692307692307692,
0.707692307692307,0.723076923076922,0.738461538461538,0.753846153846153,
0.769230769230768,0.784615384615384,0.799999999999999,0.815384615384614,
0.83076923076923,0.846153846153845,0.86153846153846,0.876923076923076,0.892307692307691,
0.907692307692306,0.923076923076922,0.938461538461537,0.953846153846152,
0.969230769230768,0.984615384615383,1.),.UNSPECIFIED.)
CURVE()
GEOMETRIC_REPRESENTATION_ITEM()
RATIONAL_B_SPLINE_CURVE((1.,1.,1.,1.,1.,1.,1.,1.,1.,1.,1.,1.,1.,1.,1.,1.,
1.,1.,1.,1.,1.,1.,1.,1.,1.,1.,1.,1.,1.,1.,1.,1.,1.,1.,1.,1.,1.,1.,1.,1.,
1.,1.,1.,1.,1.,1.,1.,1.,1.,1.,1.,1.,1.,1.,1.,1.,1.,1.,1.,1.,1.,1.,1.,1.,
1.,1.,1.,1.,1.,1.))
REPRESENTATION_ITEM('')
);
#224=(
BOUNDED_CURVE()
B_SPLINE_CURVE(5,(#39730,#39731,#39732,#39733,#39734,#39735,#39736,#39737,
#39738,#39739,#39740,#39741,#39742,#39743,#39744,#39745,#39746,#39747,#39748,
#39749,#39750,#39751,#39752,#39753,#39754,#39755,#39756,#39757,#39758,#39759,
#39760,#39761,#39762,#39763,#39764,#39765,#39766,#39767,#39768,#39769,#39770,
#39771,#39772,#39773,#39774,#39775,#39776,#39777,#39778,#39779,#39780,#39781,
#39782,#39783,#39784,#39785,#39786,#39787,#39788,#39789,#39790,#39791,#39792,
#39793,#39794,#39795,#39796,#39797,#39798,#39799),.UNSPECIFIED.,.F.,.F.)
B_SPLINE_CURVE_WITH_KNOTS((6,1,1,1,1,1,1,1,1,1,1,1,1,1,1,1,1,1,1,1,1,1,
1,1,1,1,1,1,1,1,1,1,1,1,1,1,1,1,1,1,1,1,1,1,1,1,1,1,1,1,1,1,1,1,1,1,1,1,
1,1,1,1,1,1,1,6),(0.,0.0153846153846154,0.0307692307692308,0.0461538461538462,
0.0615384615384615,0.0769230769230769,0.0923076923076923,0.107692307692308,
0.123076923076923,0.138461538461538,0.153846153846154,0.169230769230769,
0.184615384615385,0.2,0.215384615384615,0.230769230769231,0.246153846153846,
0.261538461538462,0.276923076923077,0.292307692307692,0.307692307692308,
0.323076923076923,0.338461538461538,0.353846153846154,0.369230769230769,
0.384615384615385,0.4,0.415384615384615,0.430769230769231,0.446153846153846,
0.461538461538462,0.476923076923077,0.492307692307692,0.507692307692308,
0.523076923076923,0.538461538461538,0.553846153846154,0.569230769230769,
0.584615384615384,0.6,0.615384615384615,0.63076923076923,0.646153846153846,
0.661538461538461,0.676923076923076,0.692307692307692,0.707692307692307,
0.723076923076922,0.738461538461538,0.753846153846153,0.769230769230768,
0.784615384615384,0.799999999999999,0.815384615384614,0.83076923076923,
0.846153846153845,0.86153846153846,0.876923076923076,0.892307692307691,
0.907692307692306,0.923076923076922,0.938461538461537,0.953846153846152,
0.969230769230768,0.984615384615383,0.994228156739696),.UNSPECIFIED.)
CURVE()
GEOMETRIC_REPRESENTATION_ITEM()
RATIONAL_B_SPLINE_CURVE((1.,1.,1.,1.,1.,1.,1.,1.,1.,1.,1.,1.,1.,1.,1.,1.,
1.,1.,1.,1.,1.,1.,1.,1.,1.,1.,1.,1.,1.,1.,1.,1.,1.,1.,1.,1.,1.,1.,1.,1.,
1.,1.,1.,1.,1.,1.,1.,1.,1.,1.,1.,1.,1.,1.,1.,1.,1.,1.,1.,1.,1.,1.,1.,1.,
1.,1.,1.,1.,1.,1.))
REPRESENTATION_ITEM('')
);
#225=(
BOUNDED_CURVE()
B_SPLINE_CURVE(5,(#39803,#39804,#39805,#39806,#39807,#39808,#39809,#39810,
#39811,#39812,#39813,#39814,#39815,#39816,#39817,#39818,#39819,#39820,#39821,
#39822,#39823,#39824,#39825,#39826,#39827,#39828,#39829,#39830,#39831,#39832,
#39833,#39834,#39835,#39836,#39837,#39838,#39839,#39840,#39841,#39842,#39843,
#39844,#39845,#39846,#39847,#39848,#39849,#39850,#39851,#39852,#39853,#39854,
#39855,#39856,#39857,#39858,#39859,#39860,#39861,#39862,#39863,#39864,#39865,
#39866,#39867,#39868,#39869,#39870,#39871,#39872),.UNSPECIFIED.,.F.,.F.)
B_SPLINE_CURVE_WITH_KNOTS((6,1,1,1,1,1,1,1,1,1,1,1,1,1,1,1,1,1,1,1,1,1,
1,1,1,1,1,1,1,1,1,1,1,1,1,1,1,1,1,1,1,1,1,1,1,1,1,1,1,1,1,1,1,1,1,1,1,1,
1,1,1,1,1,1,1,6),(0.00577184337452068,0.0153846153846154,0.0307692307692308,
0.0461538461538462,0.0615384615384615,0.0769230769230769,0.0923076923076923,
0.107692307692308,0.123076923076923,0.138461538461538,0.153846153846154,
0.169230769230769,0.184615384615385,0.2,0.215384615384615,0.230769230769231,
0.246153846153846,0.261538461538462,0.276923076923077,0.292307692307692,
0.307692307692308,0.323076923076923,0.338461538461538,0.353846153846154,
0.369230769230769,0.384615384615385,0.4,0.415384615384615,0.430769230769231,
0.446153846153846,0.461538461538462,0.476923076923077,0.492307692307692,
0.507692307692308,0.523076923076923,0.538461538461538,0.553846153846154,
0.569230769230769,0.584615384615384,0.6,0.615384615384615,0.63076923076923,
0.646153846153846,0.661538461538461,0.676923076923076,0.692307692307692,
0.707692307692307,0.723076923076922,0.738461538461538,0.753846153846153,
0.769230769230768,0.784615384615384,0.799999999999999,0.815384615384614,
0.83076923076923,0.846153846153845,0.86153846153846,0.876923076923076,0.892307692307691,
0.907692307692306,0.923076923076922,0.938461538461537,0.953846153846152,
0.969230769230768,0.984615384615383,1.),.UNSPECIFIED.)
CURVE()
GEOMETRIC_REPRESENTATION_ITEM()
RATIONAL_B_SPLINE_CURVE((1.,1.,1.,1.,1.,1.,1.,1.,1.,1.,1.,1.,1.,1.,1.,1.,
1.,1.,1.,1.,1.,1.,1.,1.,1.,1.,1.,1.,1.,1.,1.,1.,1.,1.,1.,1.,1.,1.,1.,1.,
1.,1.,1.,1.,1.,1.,1.,1.,1.,1.,1.,1.,1.,1.,1.,1.,1.,1.,1.,1.,1.,1.,1.,1.,
1.,1.,1.,1.,1.,1.))
REPRESENTATION_ITEM('')
);
#226=(
BOUNDED_CURVE()
B_SPLINE_CURVE(5,(#39876,#39877,#39878,#39879,#39880,#39881,#39882,#39883,
#39884,#39885,#39886,#39887,#39888,#39889,#39890,#39891,#39892,#39893,#39894,
#39895,#39896,#39897,#39898,#39899,#39900,#39901,#39902,#39903,#39904,#39905,
#39906,#39907,#39908,#39909,#39910,#39911,#39912,#39913,#39914,#39915,#39916,
#39917,#39918,#39919,#39920,#39921,#39922,#39923,#39924,#39925,#39926,#39927,
#39928,#39929,#39930,#39931,#39932,#39933,#39934,#39935,#39936,#39937,#39938,
#39939,#39940,#39941,#39942,#39943,#39944,#39945),.UNSPECIFIED.,.F.,.F.)
B_SPLINE_CURVE_WITH_KNOTS((6,1,1,1,1,1,1,1,1,1,1,1,1,1,1,1,1,1,1,1,1,1,
1,1,1,1,1,1,1,1,1,1,1,1,1,1,1,1,1,1,1,1,1,1,1,1,1,1,1,1,1,1,1,1,1,1,1,1,
1,1,1,1,1,1,1,6),(0.,0.0153846153846154,0.0307692307692308,0.0461538461538462,
0.0615384615384615,0.0769230769230769,0.0923076923076923,0.107692307692308,
0.123076923076923,0.138461538461538,0.153846153846154,0.169230769230769,
0.184615384615385,0.2,0.215384615384615,0.230769230769231,0.246153846153846,
0.261538461538462,0.276923076923077,0.292307692307692,0.307692307692308,
0.323076923076923,0.338461538461538,0.353846153846154,0.369230769230769,
0.384615384615385,0.4,0.415384615384615,0.430769230769231,0.446153846153846,
0.461538461538462,0.476923076923077,0.492307692307692,0.507692307692308,
0.523076923076923,0.538461538461538,0.553846153846154,0.569230769230769,
0.584615384615384,0.6,0.615384615384615,0.63076923076923,0.646153846153846,
0.661538461538461,0.676923076923076,0.692307692307692,0.707692307692307,
0.723076923076922,0.738461538461538,0.753846153846153,0.769230769230768,
0.784615384615384,0.799999999999999,0.815384615384614,0.83076923076923,
0.846153846153845,0.86153846153846,0.876923076923076,0.892307692307691,
0.907692307692306,0.923076923076922,0.938461538461537,0.953846153846152,
0.969230769230768,0.984615384615383,0.994228156739698),.UNSPECIFIED.)
CURVE()
GEOMETRIC_REPRESENTATION_ITEM()
RATIONAL_B_SPLINE_CURVE((1.,1.,1.,1.,1.,1.,1.,1.,1.,1.,1.,1.,1.,1.,1.,1.,
1.,1.,1.,1.,1.,1.,1.,1.,1.,1.,1.,1.,1.,1.,1.,1.,1.,1.,1.,1.,1.,1.,1.,1.,
1.,1.,1.,1.,1.,1.,1.,1.,1.,1.,1.,1.,1.,1.,1.,1.,1.,1.,1.,1.,1.,1.,1.,1.,
1.,1.,1.,1.,1.,1.))
REPRESENTATION_ITEM('')
);
#227=(
BOUNDED_CURVE()
B_SPLINE_CURVE(5,(#39949,#39950,#39951,#39952,#39953,#39954,#39955,#39956,
#39957,#39958,#39959,#39960,#39961,#39962,#39963,#39964,#39965,#39966,#39967,
#39968,#39969,#39970,#39971,#39972,#39973,#39974,#39975,#39976,#39977,#39978,
#39979,#39980,#39981,#39982,#39983,#39984,#39985,#39986,#39987,#39988,#39989,
#39990,#39991,#39992,#39993,#39994,#39995,#39996,#39997,#39998,#39999,#40000,
#40001,#40002,#40003,#40004,#40005,#40006,#40007,#40008,#40009,#40010,#40011,
#40012,#40013,#40014,#40015,#40016,#40017,#40018),.UNSPECIFIED.,.F.,.F.)
B_SPLINE_CURVE_WITH_KNOTS((6,1,1,1,1,1,1,1,1,1,1,1,1,1,1,1,1,1,1,1,1,1,
1,1,1,1,1,1,1,1,1,1,1,1,1,1,1,1,1,1,1,1,1,1,1,1,1,1,1,1,1,1,1,1,1,1,1,1,
1,1,1,1,1,1,1,6),(0.00577184337451607,0.0153846153846154,0.0307692307692308,
0.0461538461538462,0.0615384615384615,0.0769230769230769,0.0923076923076923,
0.107692307692308,0.123076923076923,0.138461538461538,0.153846153846154,
0.169230769230769,0.184615384615385,0.2,0.215384615384615,0.230769230769231,
0.246153846153846,0.261538461538462,0.276923076923077,0.292307692307692,
0.307692307692308,0.323076923076923,0.338461538461538,0.353846153846154,
0.369230769230769,0.384615384615385,0.4,0.415384615384615,0.430769230769231,
0.446153846153846,0.461538461538462,0.476923076923077,0.492307692307692,
0.507692307692308,0.523076923076923,0.538461538461538,0.553846153846154,
0.569230769230769,0.584615384615384,0.6,0.615384615384615,0.63076923076923,
0.646153846153846,0.661538461538461,0.676923076923076,0.692307692307692,
0.707692307692307,0.723076923076922,0.738461538461538,0.753846153846153,
0.769230769230768,0.784615384615384,0.799999999999999,0.815384615384614,
0.83076923076923,0.846153846153845,0.86153846153846,0.876923076923076,0.892307692307691,
0.907692307692306,0.923076923076922,0.938461538461537,0.953846153846152,
0.969230769230768,0.984615384615383,1.),.UNSPECIFIED.)
CURVE()
GEOMETRIC_REPRESENTATION_ITEM()
RATIONAL_B_SPLINE_CURVE((1.,1.,1.,1.,1.,1.,1.,1.,1.,1.,1.,1.,1.,1.,1.,1.,
1.,1.,1.,1.,1.,1.,1.,1.,1.,1.,1.,1.,1.,1.,1.,1.,1.,1.,1.,1.,1.,1.,1.,1.,
1.,1.,1.,1.,1.,1.,1.,1.,1.,1.,1.,1.,1.,1.,1.,1.,1.,1.,1.,1.,1.,1.,1.,1.,
1.,1.,1.,1.,1.,1.))
REPRESENTATION_ITEM('')
);
#228=(
BOUNDED_CURVE()
B_SPLINE_CURVE(5,(#40022,#40023,#40024,#40025,#40026,#40027,#40028,#40029,
#40030,#40031,#40032,#40033,#40034,#40035,#40036,#40037,#40038,#40039,#40040,
#40041,#40042,#40043,#40044,#40045,#40046,#40047,#40048,#40049,#40050,#40051,
#40052,#40053,#40054,#40055,#40056,#40057,#40058,#40059,#40060,#40061,#40062,
#40063,#40064,#40065,#40066,#40067,#40068,#40069,#40070,#40071,#40072,#40073,
#40074,#40075,#40076,#40077,#40078,#40079,#40080,#40081,#40082,#40083,#40084,
#40085,#40086,#40087,#40088,#40089,#40090,#40091),.UNSPECIFIED.,.F.,.F.)
B_SPLINE_CURVE_WITH_KNOTS((6,1,1,1,1,1,1,1,1,1,1,1,1,1,1,1,1,1,1,1,1,1,
1,1,1,1,1,1,1,1,1,1,1,1,1,1,1,1,1,1,1,1,1,1,1,1,1,1,1,1,1,1,1,1,1,1,1,1,
1,1,1,1,1,1,1,6),(0.,0.0153846153846154,0.0307692307692308,0.0461538461538462,
0.0615384615384615,0.0769230769230769,0.0923076923076923,0.107692307692308,
0.123076923076923,0.138461538461538,0.153846153846154,0.169230769230769,
0.184615384615385,0.2,0.215384615384615,0.230769230769231,0.246153846153846,
0.261538461538462,0.276923076923077,0.292307692307692,0.307692307692308,
0.323076923076923,0.338461538461538,0.353846153846154,0.369230769230769,
0.384615384615385,0.4,0.415384615384615,0.430769230769231,0.446153846153846,
0.461538461538462,0.476923076923077,0.492307692307692,0.507692307692308,
0.523076923076923,0.538461538461538,0.553846153846154,0.569230769230769,
0.584615384615384,0.6,0.615384615384615,0.63076923076923,0.646153846153846,
0.661538461538461,0.676923076923076,0.692307692307692,0.707692307692307,
0.723076923076922,0.738461538461538,0.753846153846153,0.769230769230768,
0.784615384615384,0.799999999999999,0.815384615384614,0.83076923076923,
0.846153846153845,0.86153846153846,0.876923076923076,0.892307692307691,
0.907692307692306,0.923076923076922,0.938461538461537,0.953846153846152,
0.969230769230768,0.984615384615383,0.994228156739704),.UNSPECIFIED.)
CURVE()
GEOMETRIC_REPRESENTATION_ITEM()
RATIONAL_B_SPLINE_CURVE((1.,1.,1.,1.,1.,1.,1.,1.,1.,1.,1.,1.,1.,1.,1.,1.,
1.,1.,1.,1.,1.,1.,1.,1.,1.,1.,1.,1.,1.,1.,1.,1.,1.,1.,1.,1.,1.,1.,1.,1.,
1.,1.,1.,1.,1.,1.,1.,1.,1.,1.,1.,1.,1.,1.,1.,1.,1.,1.,1.,1.,1.,1.,1.,1.,
1.,1.,1.,1.,1.,1.))
REPRESENTATION_ITEM('')
);
#229=(
BOUNDED_CURVE()
B_SPLINE_CURVE(5,(#40095,#40096,#40097,#40098,#40099,#40100,#40101,#40102,
#40103,#40104,#40105,#40106,#40107,#40108,#40109,#40110,#40111,#40112,#40113,
#40114,#40115,#40116,#40117,#40118,#40119,#40120,#40121,#40122,#40123,#40124,
#40125,#40126,#40127,#40128,#40129,#40130,#40131,#40132,#40133,#40134,#40135,
#40136,#40137,#40138,#40139,#40140,#40141,#40142,#40143,#40144,#40145,#40146,
#40147,#40148,#40149,#40150,#40151,#40152,#40153,#40154,#40155,#40156,#40157,
#40158,#40159,#40160,#40161,#40162,#40163,#40164),.UNSPECIFIED.,.F.,.F.)
B_SPLINE_CURVE_WITH_KNOTS((6,1,1,1,1,1,1,1,1,1,1,1,1,1,1,1,1,1,1,1,1,1,
1,1,1,1,1,1,1,1,1,1,1,1,1,1,1,1,1,1,1,1,1,1,1,1,1,1,1,1,1,1,1,1,1,1,1,1,
1,1,1,1,1,1,1,6),(0.00577184337449692,0.0153846153846154,0.0307692307692308,
0.0461538461538462,0.0615384615384615,0.0769230769230769,0.0923076923076923,
0.107692307692308,0.123076923076923,0.138461538461538,0.153846153846154,
0.169230769230769,0.184615384615385,0.2,0.215384615384615,0.230769230769231,
0.246153846153846,0.261538461538462,0.276923076923077,0.292307692307692,
0.307692307692308,0.323076923076923,0.338461538461538,0.353846153846154,
0.369230769230769,0.384615384615385,0.4,0.415384615384615,0.430769230769231,
0.446153846153846,0.461538461538462,0.476923076923077,0.492307692307692,
0.507692307692308,0.523076923076923,0.538461538461538,0.553846153846154,
0.569230769230769,0.584615384615384,0.6,0.615384615384615,0.63076923076923,
0.646153846153846,0.661538461538461,0.676923076923076,0.692307692307692,
0.707692307692307,0.723076923076922,0.738461538461538,0.753846153846153,
0.769230769230768,0.784615384615384,0.799999999999999,0.815384615384614,
0.83076923076923,0.846153846153845,0.86153846153846,0.876923076923076,0.892307692307691,
0.907692307692306,0.923076923076922,0.938461538461537,0.953846153846152,
0.969230769230768,0.984615384615383,1.),.UNSPECIFIED.)
CURVE()
GEOMETRIC_REPRESENTATION_ITEM()
RATIONAL_B_SPLINE_CURVE((1.,1.,1.,1.,1.,1.,1.,1.,1.,1.,1.,1.,1.,1.,1.,1.,
1.,1.,1.,1.,1.,1.,1.,1.,1.,1.,1.,1.,1.,1.,1.,1.,1.,1.,1.,1.,1.,1.,1.,1.,
1.,1.,1.,1.,1.,1.,1.,1.,1.,1.,1.,1.,1.,1.,1.,1.,1.,1.,1.,1.,1.,1.,1.,1.,
1.,1.,1.,1.,1.,1.))
REPRESENTATION_ITEM('')
);
#230=(
BOUNDED_CURVE()
B_SPLINE_CURVE(5,(#40168,#40169,#40170,#40171,#40172,#40173,#40174,#40175,
#40176,#40177,#40178,#40179,#40180,#40181,#40182,#40183,#40184,#40185,#40186,
#40187,#40188,#40189,#40190,#40191,#40192,#40193,#40194,#40195,#40196,#40197,
#40198,#40199,#40200,#40201,#40202,#40203,#40204,#40205,#40206,#40207,#40208,
#40209,#40210,#40211,#40212,#40213,#40214,#40215,#40216,#40217,#40218,#40219,
#40220,#40221,#40222,#40223,#40224,#40225,#40226,#40227,#40228,#40229,#40230,
#40231,#40232,#40233,#40234,#40235,#40236,#40237),.UNSPECIFIED.,.F.,.F.)
B_SPLINE_CURVE_WITH_KNOTS((6,1,1,1,1,1,1,1,1,1,1,1,1,1,1,1,1,1,1,1,1,1,
1,1,1,1,1,1,1,1,1,1,1,1,1,1,1,1,1,1,1,1,1,1,1,1,1,1,1,1,1,1,1,1,1,1,1,1,
1,1,1,1,1,1,1,6),(0.,0.0153846153846154,0.0307692307692308,0.0461538461538462,
0.0615384615384615,0.0769230769230769,0.0923076923076923,0.107692307692308,
0.123076923076923,0.138461538461538,0.153846153846154,0.169230769230769,
0.184615384615385,0.2,0.215384615384615,0.230769230769231,0.246153846153846,
0.261538461538462,0.276923076923077,0.292307692307692,0.307692307692308,
0.323076923076923,0.338461538461538,0.353846153846154,0.369230769230769,
0.384615384615385,0.4,0.415384615384615,0.430769230769231,0.446153846153846,
0.461538461538462,0.476923076923077,0.492307692307692,0.507692307692308,
0.523076923076923,0.538461538461538,0.553846153846154,0.569230769230769,
0.584615384615384,0.6,0.615384615384615,0.63076923076923,0.646153846153846,
0.661538461538461,0.676923076923076,0.692307692307692,0.707692307692307,
0.723076923076922,0.738461538461538,0.753846153846153,0.769230769230768,
0.784615384615384,0.799999999999999,0.815384615384614,0.83076923076923,
0.846153846153845,0.86153846153846,0.876923076923076,0.892307692307691,
0.907692307692306,0.923076923076922,0.938461538461537,0.953846153846152,
0.969230769230768,0.984615384615383,0.994228156739711),.UNSPECIFIED.)
CURVE()
GEOMETRIC_REPRESENTATION_ITEM()
RATIONAL_B_SPLINE_CURVE((1.,1.,1.,1.,1.,1.,1.,1.,1.,1.,1.,1.,1.,1.,1.,1.,
1.,1.,1.,1.,1.,1.,1.,1.,1.,1.,1.,1.,1.,1.,1.,1.,1.,1.,1.,1.,1.,1.,1.,1.,
1.,1.,1.,1.,1.,1.,1.,1.,1.,1.,1.,1.,1.,1.,1.,1.,1.,1.,1.,1.,1.,1.,1.,1.,
1.,1.,1.,1.,1.,1.))
REPRESENTATION_ITEM('')
);
#231=(
BOUNDED_CURVE()
B_SPLINE_CURVE(5,(#40241,#40242,#40243,#40244,#40245,#40246,#40247,#40248,
#40249,#40250,#40251,#40252,#40253,#40254,#40255,#40256,#40257,#40258,#40259,
#40260,#40261,#40262,#40263,#40264,#40265,#40266,#40267,#40268,#40269,#40270,
#40271,#40272,#40273,#40274,#40275,#40276,#40277,#40278,#40279,#40280,#40281,
#40282,#40283,#40284,#40285,#40286,#40287,#40288,#40289,#40290,#40291,#40292,
#40293,#40294,#40295,#40296,#40297,#40298,#40299,#40300,#40301,#40302,#40303,
#40304,#40305,#40306,#40307,#40308,#40309,#40310),.UNSPECIFIED.,.F.,.F.)
B_SPLINE_CURVE_WITH_KNOTS((6,1,1,1,1,1,1,1,1,1,1,1,1,1,1,1,1,1,1,1,1,1,
1,1,1,1,1,1,1,1,1,1,1,1,1,1,1,1,1,1,1,1,1,1,1,1,1,1,1,1,1,1,1,1,1,1,1,1,
1,1,1,1,1,1,1,6),(0.00577184337450058,0.0153846153846154,0.0307692307692308,
0.0461538461538462,0.0615384615384615,0.0769230769230769,0.0923076923076923,
0.107692307692308,0.123076923076923,0.138461538461538,0.153846153846154,
0.169230769230769,0.184615384615385,0.2,0.215384615384615,0.230769230769231,
0.246153846153846,0.261538461538462,0.276923076923077,0.292307692307692,
0.307692307692308,0.323076923076923,0.338461538461538,0.353846153846154,
0.369230769230769,0.384615384615385,0.4,0.415384615384615,0.430769230769231,
0.446153846153846,0.461538461538462,0.476923076923077,0.492307692307692,
0.507692307692308,0.523076923076923,0.538461538461538,0.553846153846154,
0.569230769230769,0.584615384615384,0.6,0.615384615384615,0.63076923076923,
0.646153846153846,0.661538461538461,0.676923076923076,0.692307692307692,
0.707692307692307,0.723076923076922,0.738461538461538,0.753846153846153,
0.769230769230768,0.784615384615384,0.799999999999999,0.815384615384614,
0.83076923076923,0.846153846153845,0.86153846153846,0.876923076923076,0.892307692307691,
0.907692307692306,0.923076923076922,0.938461538461537,0.953846153846152,
0.969230769230768,0.984615384615383,1.),.UNSPECIFIED.)
CURVE()
GEOMETRIC_REPRESENTATION_ITEM()
RATIONAL_B_SPLINE_CURVE((1.,1.,1.,1.,1.,1.,1.,1.,1.,1.,1.,1.,1.,1.,1.,1.,
1.,1.,1.,1.,1.,1.,1.,1.,1.,1.,1.,1.,1.,1.,1.,1.,1.,1.,1.,1.,1.,1.,1.,1.,
1.,1.,1.,1.,1.,1.,1.,1.,1.,1.,1.,1.,1.,1.,1.,1.,1.,1.,1.,1.,1.,1.,1.,1.,
1.,1.,1.,1.,1.,1.))
REPRESENTATION_ITEM('')
);
#232=(
BOUNDED_CURVE()
B_SPLINE_CURVE(5,(#40314,#40315,#40316,#40317,#40318,#40319,#40320,#40321,
#40322,#40323,#40324,#40325,#40326,#40327,#40328,#40329,#40330,#40331,#40332,
#40333,#40334,#40335,#40336,#40337,#40338,#40339,#40340,#40341,#40342,#40343,
#40344,#40345,#40346,#40347,#40348,#40349,#40350,#40351,#40352,#40353,#40354,
#40355,#40356,#40357,#40358,#40359,#40360,#40361,#40362,#40363,#40364,#40365,
#40366,#40367,#40368,#40369,#40370,#40371,#40372,#40373,#40374,#40375,#40376,
#40377,#40378,#40379,#40380,#40381,#40382,#40383),.UNSPECIFIED.,.F.,.F.)
B_SPLINE_CURVE_WITH_KNOTS((6,1,1,1,1,1,1,1,1,1,1,1,1,1,1,1,1,1,1,1,1,1,
1,1,1,1,1,1,1,1,1,1,1,1,1,1,1,1,1,1,1,1,1,1,1,1,1,1,1,1,1,1,1,1,1,1,1,1,
1,1,1,1,1,1,1,6),(0.,0.0153846153846154,0.0307692307692308,0.0461538461538462,
0.0615384615384615,0.0769230769230769,0.0923076923076923,0.107692307692308,
0.123076923076923,0.138461538461538,0.153846153846154,0.169230769230769,
0.184615384615385,0.2,0.215384615384615,0.230769230769231,0.246153846153846,
0.261538461538462,0.276923076923077,0.292307692307692,0.307692307692308,
0.323076923076923,0.338461538461538,0.353846153846154,0.369230769230769,
0.384615384615385,0.4,0.415384615384615,0.430769230769231,0.446153846153846,
0.461538461538462,0.476923076923077,0.492307692307692,0.507692307692308,
0.523076923076923,0.538461538461538,0.553846153846154,0.569230769230769,
0.584615384615384,0.6,0.615384615384615,0.63076923076923,0.646153846153846,
0.661538461538461,0.676923076923076,0.692307692307692,0.707692307692307,
0.723076923076922,0.738461538461538,0.753846153846153,0.769230769230768,
0.784615384615384,0.799999999999999,0.815384615384614,0.83076923076923,
0.846153846153845,0.86153846153846,0.876923076923076,0.892307692307691,
0.907692307692306,0.923076923076922,0.938461538461537,0.953846153846152,
0.969230769230768,0.984615384615383,0.994228156739701),.UNSPECIFIED.)
CURVE()
GEOMETRIC_REPRESENTATION_ITEM()
RATIONAL_B_SPLINE_CURVE((1.,1.,1.,1.,1.,1.,1.,1.,1.,1.,1.,1.,1.,1.,1.,1.,
1.,1.,1.,1.,1.,1.,1.,1.,1.,1.,1.,1.,1.,1.,1.,1.,1.,1.,1.,1.,1.,1.,1.,1.,
1.,1.,1.,1.,1.,1.,1.,1.,1.,1.,1.,1.,1.,1.,1.,1.,1.,1.,1.,1.,1.,1.,1.,1.,
1.,1.,1.,1.,1.,1.))
REPRESENTATION_ITEM('')
);
#233=(
BOUNDED_CURVE()
B_SPLINE_CURVE(5,(#40387,#40388,#40389,#40390,#40391,#40392,#40393,#40394,
#40395,#40396,#40397,#40398,#40399,#40400,#40401,#40402,#40403,#40404,#40405,
#40406,#40407,#40408,#40409,#40410,#40411,#40412,#40413,#40414,#40415,#40416,
#40417,#40418,#40419,#40420,#40421,#40422,#40423,#40424,#40425,#40426,#40427,
#40428,#40429,#40430,#40431,#40432,#40433,#40434,#40435,#40436,#40437,#40438,
#40439,#40440,#40441,#40442,#40443,#40444,#40445,#40446,#40447,#40448,#40449,
#40450,#40451,#40452,#40453,#40454,#40455,#40456),.UNSPECIFIED.,.F.,.F.)
B_SPLINE_CURVE_WITH_KNOTS((6,1,1,1,1,1,1,1,1,1,1,1,1,1,1,1,1,1,1,1,1,1,
1,1,1,1,1,1,1,1,1,1,1,1,1,1,1,1,1,1,1,1,1,1,1,1,1,1,1,1,1,1,1,1,1,1,1,1,
1,1,1,1,1,1,1,6),(0.0057718433745091,0.0153846153846154,0.0307692307692308,
0.0461538461538462,0.0615384615384615,0.0769230769230769,0.0923076923076923,
0.107692307692308,0.123076923076923,0.138461538461538,0.153846153846154,
0.169230769230769,0.184615384615385,0.2,0.215384615384615,0.230769230769231,
0.246153846153846,0.261538461538462,0.276923076923077,0.292307692307692,
0.307692307692308,0.323076923076923,0.338461538461538,0.353846153846154,
0.369230769230769,0.384615384615385,0.4,0.415384615384615,0.430769230769231,
0.446153846153846,0.461538461538462,0.476923076923077,0.492307692307692,
0.507692307692308,0.523076923076923,0.538461538461538,0.553846153846154,
0.569230769230769,0.584615384615384,0.6,0.615384615384615,0.63076923076923,
0.646153846153846,0.661538461538461,0.676923076923076,0.692307692307692,
0.707692307692307,0.723076923076922,0.738461538461538,0.753846153846153,
0.769230769230768,0.784615384615384,0.799999999999999,0.815384615384614,
0.83076923076923,0.846153846153845,0.86153846153846,0.876923076923076,0.892307692307691,
0.907692307692306,0.923076923076922,0.938461538461537,0.953846153846152,
0.969230769230768,0.984615384615383,1.),.UNSPECIFIED.)
CURVE()
GEOMETRIC_REPRESENTATION_ITEM()
RATIONAL_B_SPLINE_CURVE((1.,1.,1.,1.,1.,1.,1.,1.,1.,1.,1.,1.,1.,1.,1.,1.,
1.,1.,1.,1.,1.,1.,1.,1.,1.,1.,1.,1.,1.,1.,1.,1.,1.,1.,1.,1.,1.,1.,1.,1.,
1.,1.,1.,1.,1.,1.,1.,1.,1.,1.,1.,1.,1.,1.,1.,1.,1.,1.,1.,1.,1.,1.,1.,1.,
1.,1.,1.,1.,1.,1.))
REPRESENTATION_ITEM('')
);
#234=(
BOUNDED_CURVE()
B_SPLINE_CURVE(5,(#40460,#40461,#40462,#40463,#40464,#40465,#40466,#40467,
#40468,#40469,#40470,#40471,#40472,#40473,#40474,#40475,#40476,#40477,#40478,
#40479,#40480,#40481,#40482,#40483,#40484,#40485,#40486,#40487,#40488,#40489,
#40490,#40491,#40492,#40493,#40494,#40495,#40496,#40497,#40498,#40499,#40500,
#40501,#40502,#40503,#40504,#40505,#40506,#40507,#40508,#40509,#40510,#40511,
#40512,#40513,#40514,#40515,#40516,#40517,#40518,#40519,#40520,#40521,#40522,
#40523,#40524,#40525,#40526,#40527,#40528,#40529),.UNSPECIFIED.,.F.,.F.)
B_SPLINE_CURVE_WITH_KNOTS((6,1,1,1,1,1,1,1,1,1,1,1,1,1,1,1,1,1,1,1,1,1,
1,1,1,1,1,1,1,1,1,1,1,1,1,1,1,1,1,1,1,1,1,1,1,1,1,1,1,1,1,1,1,1,1,1,1,1,
1,1,1,1,1,1,1,6),(0.,0.0153846153846154,0.0307692307692308,0.0461538461538462,
0.0615384615384615,0.0769230769230769,0.0923076923076923,0.107692307692308,
0.123076923076923,0.138461538461538,0.153846153846154,0.169230769230769,
0.184615384615385,0.2,0.215384615384615,0.230769230769231,0.246153846153846,
0.261538461538462,0.276923076923077,0.292307692307692,0.307692307692308,
0.323076923076923,0.338461538461538,0.353846153846154,0.369230769230769,
0.384615384615385,0.4,0.415384615384615,0.430769230769231,0.446153846153846,
0.461538461538462,0.476923076923077,0.492307692307692,0.507692307692308,
0.523076923076923,0.538461538461538,0.553846153846154,0.569230769230769,
0.584615384615384,0.6,0.615384615384615,0.63076923076923,0.646153846153846,
0.661538461538461,0.676923076923076,0.692307692307692,0.707692307692307,
0.723076923076922,0.738461538461538,0.753846153846153,0.769230769230768,
0.784615384615384,0.799999999999999,0.815384615384614,0.83076923076923,
0.846153846153845,0.86153846153846,0.876923076923076,0.892307692307691,
0.907692307692306,0.923076923076922,0.938461538461537,0.953846153846152,
0.969230769230768,0.984615384615383,0.994228156739689),.UNSPECIFIED.)
CURVE()
GEOMETRIC_REPRESENTATION_ITEM()
RATIONAL_B_SPLINE_CURVE((1.,1.,1.,1.,1.,1.,1.,1.,1.,1.,1.,1.,1.,1.,1.,1.,
1.,1.,1.,1.,1.,1.,1.,1.,1.,1.,1.,1.,1.,1.,1.,1.,1.,1.,1.,1.,1.,1.,1.,1.,
1.,1.,1.,1.,1.,1.,1.,1.,1.,1.,1.,1.,1.,1.,1.,1.,1.,1.,1.,1.,1.,1.,1.,1.,
1.,1.,1.,1.,1.,1.))
REPRESENTATION_ITEM('')
);
#235=(
BOUNDED_CURVE()
B_SPLINE_CURVE(5,(#40533,#40534,#40535,#40536,#40537,#40538,#40539,#40540,
#40541,#40542,#40543,#40544,#40545,#40546,#40547,#40548,#40549,#40550,#40551,
#40552,#40553,#40554,#40555,#40556,#40557,#40558,#40559,#40560,#40561,#40562,
#40563,#40564,#40565,#40566,#40567,#40568,#40569,#40570,#40571,#40572,#40573,
#40574,#40575,#40576,#40577,#40578,#40579,#40580,#40581,#40582,#40583,#40584,
#40585,#40586,#40587,#40588,#40589,#40590,#40591,#40592,#40593,#40594,#40595,
#40596,#40597,#40598,#40599,#40600,#40601,#40602),.UNSPECIFIED.,.F.,.F.)
B_SPLINE_CURVE_WITH_KNOTS((6,1,1,1,1,1,1,1,1,1,1,1,1,1,1,1,1,1,1,1,1,1,
1,1,1,1,1,1,1,1,1,1,1,1,1,1,1,1,1,1,1,1,1,1,1,1,1,1,1,1,1,1,1,1,1,1,1,1,
1,1,1,1,1,1,1,6),(0.00577184337450777,0.0153846153846154,0.0307692307692308,
0.0461538461538462,0.0615384615384615,0.0769230769230769,0.0923076923076923,
0.107692307692308,0.123076923076923,0.138461538461538,0.153846153846154,
0.169230769230769,0.184615384615385,0.2,0.215384615384615,0.230769230769231,
0.246153846153846,0.261538461538462,0.276923076923077,0.292307692307692,
0.307692307692308,0.323076923076923,0.338461538461538,0.353846153846154,
0.369230769230769,0.384615384615385,0.4,0.415384615384615,0.430769230769231,
0.446153846153846,0.461538461538462,0.476923076923077,0.492307692307692,
0.507692307692308,0.523076923076923,0.538461538461538,0.553846153846154,
0.569230769230769,0.584615384615384,0.6,0.615384615384615,0.63076923076923,
0.646153846153846,0.661538461538461,0.676923076923076,0.692307692307692,
0.707692307692307,0.723076923076922,0.738461538461538,0.753846153846153,
0.769230769230768,0.784615384615384,0.799999999999999,0.815384615384614,
0.83076923076923,0.846153846153845,0.86153846153846,0.876923076923076,0.892307692307691,
0.907692307692306,0.923076923076922,0.938461538461537,0.953846153846152,
0.969230769230768,0.984615384615383,1.),.UNSPECIFIED.)
CURVE()
GEOMETRIC_REPRESENTATION_ITEM()
RATIONAL_B_SPLINE_CURVE((1.,1.,1.,1.,1.,1.,1.,1.,1.,1.,1.,1.,1.,1.,1.,1.,
1.,1.,1.,1.,1.,1.,1.,1.,1.,1.,1.,1.,1.,1.,1.,1.,1.,1.,1.,1.,1.,1.,1.,1.,
1.,1.,1.,1.,1.,1.,1.,1.,1.,1.,1.,1.,1.,1.,1.,1.,1.,1.,1.,1.,1.,1.,1.,1.,
1.,1.,1.,1.,1.,1.))
REPRESENTATION_ITEM('')
);
#236=(
BOUNDED_CURVE()
B_SPLINE_CURVE(5,(#40606,#40607,#40608,#40609,#40610,#40611,#40612,#40613,
#40614,#40615,#40616,#40617,#40618,#40619,#40620,#40621,#40622,#40623,#40624,
#40625,#40626,#40627,#40628,#40629,#40630,#40631,#40632,#40633,#40634,#40635,
#40636,#40637,#40638,#40639,#40640,#40641,#40642,#40643,#40644,#40645,#40646,
#40647,#40648,#40649,#40650,#40651,#40652,#40653,#40654,#40655,#40656,#40657,
#40658,#40659,#40660,#40661,#40662,#40663,#40664,#40665,#40666,#40667,#40668,
#40669,#40670,#40671,#40672,#40673,#40674,#40675),.UNSPECIFIED.,.F.,.F.)
B_SPLINE_CURVE_WITH_KNOTS((6,1,1,1,1,1,1,1,1,1,1,1,1,1,1,1,1,1,1,1,1,1,
1,1,1,1,1,1,1,1,1,1,1,1,1,1,1,1,1,1,1,1,1,1,1,1,1,1,1,1,1,1,1,1,1,1,1,1,
1,1,1,1,1,1,1,6),(0.,0.0153846153846154,0.0307692307692308,0.0461538461538462,
0.0615384615384615,0.0769230769230769,0.0923076923076923,0.107692307692308,
0.123076923076923,0.138461538461538,0.153846153846154,0.169230769230769,
0.184615384615385,0.2,0.215384615384615,0.230769230769231,0.246153846153846,
0.261538461538462,0.276923076923077,0.292307692307692,0.307692307692308,
0.323076923076923,0.338461538461538,0.353846153846154,0.369230769230769,
0.384615384615385,0.4,0.415384615384615,0.430769230769231,0.446153846153846,
0.461538461538462,0.476923076923077,0.492307692307692,0.507692307692308,
0.523076923076923,0.538461538461538,0.553846153846154,0.569230769230769,
0.584615384615384,0.6,0.615384615384615,0.63076923076923,0.646153846153846,
0.661538461538461,0.676923076923076,0.692307692307692,0.707692307692307,
0.723076923076922,0.738461538461538,0.753846153846153,0.769230769230768,
0.784615384615384,0.799999999999999,0.815384615384614,0.83076923076923,
0.846153846153845,0.86153846153846,0.876923076923076,0.892307692307691,
0.907692307692306,0.923076923076922,0.938461538461537,0.953846153846152,
0.969230769230768,0.984615384615383,0.994228156739701),.UNSPECIFIED.)
CURVE()
GEOMETRIC_REPRESENTATION_ITEM()
RATIONAL_B_SPLINE_CURVE((1.,1.,1.,1.,1.,1.,1.,1.,1.,1.,1.,1.,1.,1.,1.,1.,
1.,1.,1.,1.,1.,1.,1.,1.,1.,1.,1.,1.,1.,1.,1.,1.,1.,1.,1.,1.,1.,1.,1.,1.,
1.,1.,1.,1.,1.,1.,1.,1.,1.,1.,1.,1.,1.,1.,1.,1.,1.,1.,1.,1.,1.,1.,1.,1.,
1.,1.,1.,1.,1.,1.))
REPRESENTATION_ITEM('')
);
#237=(
BOUNDED_CURVE()
B_SPLINE_CURVE(5,(#40679,#40680,#40681,#40682,#40683,#40684,#40685,#40686,
#40687,#40688,#40689,#40690,#40691,#40692,#40693,#40694,#40695,#40696,#40697,
#40698,#40699,#40700,#40701,#40702,#40703,#40704,#40705,#40706,#40707,#40708,
#40709,#40710,#40711,#40712,#40713,#40714,#40715,#40716,#40717,#40718,#40719,
#40720,#40721,#40722,#40723,#40724,#40725,#40726,#40727,#40728,#40729,#40730,
#40731,#40732,#40733,#40734,#40735,#40736,#40737,#40738,#40739,#40740,#40741,
#40742,#40743,#40744,#40745,#40746,#40747,#40748),.UNSPECIFIED.,.F.,.F.)
B_SPLINE_CURVE_WITH_KNOTS((6,1,1,1,1,1,1,1,1,1,1,1,1,1,1,1,1,1,1,1,1,1,
1,1,1,1,1,1,1,1,1,1,1,1,1,1,1,1,1,1,1,1,1,1,1,1,1,1,1,1,1,1,1,1,1,1,1,1,
1,1,1,1,1,1,1,6),(0.00577184337450172,0.0153846153846154,0.0307692307692308,
0.0461538461538462,0.0615384615384615,0.0769230769230769,0.0923076923076923,
0.107692307692308,0.123076923076923,0.138461538461538,0.153846153846154,
0.169230769230769,0.184615384615385,0.2,0.215384615384615,0.230769230769231,
0.246153846153846,0.261538461538462,0.276923076923077,0.292307692307692,
0.307692307692308,0.323076923076923,0.338461538461538,0.353846153846154,
0.369230769230769,0.384615384615385,0.4,0.415384615384615,0.430769230769231,
0.446153846153846,0.461538461538462,0.476923076923077,0.492307692307692,
0.507692307692308,0.523076923076923,0.538461538461538,0.553846153846154,
0.569230769230769,0.584615384615384,0.6,0.615384615384615,0.63076923076923,
0.646153846153846,0.661538461538461,0.676923076923076,0.692307692307692,
0.707692307692307,0.723076923076922,0.738461538461538,0.753846153846153,
0.769230769230768,0.784615384615384,0.799999999999999,0.815384615384614,
0.83076923076923,0.846153846153845,0.86153846153846,0.876923076923076,0.892307692307691,
0.907692307692306,0.923076923076922,0.938461538461537,0.953846153846152,
0.969230769230768,0.984615384615383,1.),.UNSPECIFIED.)
CURVE()
GEOMETRIC_REPRESENTATION_ITEM()
RATIONAL_B_SPLINE_CURVE((1.,1.,1.,1.,1.,1.,1.,1.,1.,1.,1.,1.,1.,1.,1.,1.,
1.,1.,1.,1.,1.,1.,1.,1.,1.,1.,1.,1.,1.,1.,1.,1.,1.,1.,1.,1.,1.,1.,1.,1.,
1.,1.,1.,1.,1.,1.,1.,1.,1.,1.,1.,1.,1.,1.,1.,1.,1.,1.,1.,1.,1.,1.,1.,1.,
1.,1.,1.,1.,1.,1.))
REPRESENTATION_ITEM('')
);
#238=(
BOUNDED_CURVE()
B_SPLINE_CURVE(5,(#40752,#40753,#40754,#40755,#40756,#40757,#40758,#40759,
#40760,#40761,#40762,#40763,#40764,#40765,#40766,#40767,#40768,#40769,#40770,
#40771,#40772,#40773,#40774,#40775,#40776,#40777,#40778,#40779,#40780,#40781,
#40782,#40783,#40784,#40785,#40786,#40787,#40788,#40789,#40790,#40791,#40792,
#40793,#40794,#40795,#40796,#40797,#40798,#40799,#40800,#40801,#40802,#40803,
#40804,#40805,#40806,#40807,#40808,#40809,#40810,#40811,#40812,#40813,#40814,
#40815,#40816,#40817,#40818,#40819,#40820,#40821),.UNSPECIFIED.,.F.,.F.)
B_SPLINE_CURVE_WITH_KNOTS((6,1,1,1,1,1,1,1,1,1,1,1,1,1,1,1,1,1,1,1,1,1,
1,1,1,1,1,1,1,1,1,1,1,1,1,1,1,1,1,1,1,1,1,1,1,1,1,1,1,1,1,1,1,1,1,1,1,1,
1,1,1,1,1,1,1,6),(0.,0.0153846153846154,0.0307692307692308,0.0461538461538462,
0.0615384615384615,0.0769230769230769,0.0923076923076923,0.107692307692308,
0.123076923076923,0.138461538461538,0.153846153846154,0.169230769230769,
0.184615384615385,0.2,0.215384615384615,0.230769230769231,0.246153846153846,
0.261538461538462,0.276923076923077,0.292307692307692,0.307692307692308,
0.323076923076923,0.338461538461538,0.353846153846154,0.369230769230769,
0.384615384615385,0.4,0.415384615384615,0.430769230769231,0.446153846153846,
0.461538461538462,0.476923076923077,0.492307692307692,0.507692307692308,
0.523076923076923,0.538461538461538,0.553846153846154,0.569230769230769,
0.584615384615384,0.6,0.615384615384615,0.63076923076923,0.646153846153846,
0.661538461538461,0.676923076923076,0.692307692307692,0.707692307692307,
0.723076923076922,0.738461538461538,0.753846153846153,0.769230769230768,
0.784615384615384,0.799999999999999,0.815384615384614,0.83076923076923,
0.846153846153845,0.86153846153846,0.876923076923076,0.892307692307691,
0.907692307692306,0.923076923076922,0.938461538461537,0.953846153846152,
0.969230769230768,0.984615384615383,0.99422815673971),.UNSPECIFIED.)
CURVE()
GEOMETRIC_REPRESENTATION_ITEM()
RATIONAL_B_SPLINE_CURVE((1.,1.,1.,1.,1.,1.,1.,1.,1.,1.,1.,1.,1.,1.,1.,1.,
1.,1.,1.,1.,1.,1.,1.,1.,1.,1.,1.,1.,1.,1.,1.,1.,1.,1.,1.,1.,1.,1.,1.,1.,
1.,1.,1.,1.,1.,1.,1.,1.,1.,1.,1.,1.,1.,1.,1.,1.,1.,1.,1.,1.,1.,1.,1.,1.,
1.,1.,1.,1.,1.,1.))
REPRESENTATION_ITEM('')
);
#239=(
BOUNDED_CURVE()
B_SPLINE_CURVE(5,(#40825,#40826,#40827,#40828,#40829,#40830,#40831,#40832,
#40833,#40834,#40835,#40836,#40837,#40838,#40839,#40840,#40841,#40842,#40843,
#40844,#40845,#40846,#40847,#40848,#40849,#40850,#40851,#40852,#40853,#40854,
#40855,#40856,#40857,#40858,#40859,#40860,#40861,#40862,#40863,#40864,#40865,
#40866,#40867,#40868,#40869,#40870,#40871,#40872,#40873,#40874,#40875,#40876,
#40877,#40878,#40879,#40880,#40881,#40882,#40883,#40884,#40885,#40886,#40887,
#40888,#40889,#40890,#40891,#40892,#40893,#40894),.UNSPECIFIED.,.F.,.F.)
B_SPLINE_CURVE_WITH_KNOTS((6,1,1,1,1,1,1,1,1,1,1,1,1,1,1,1,1,1,1,1,1,1,
1,1,1,1,1,1,1,1,1,1,1,1,1,1,1,1,1,1,1,1,1,1,1,1,1,1,1,1,1,1,1,1,1,1,1,1,
1,1,1,1,1,1,1,6),(0.00577184337448657,0.0153846153846154,0.0307692307692308,
0.0461538461538462,0.0615384615384615,0.0769230769230769,0.0923076923076923,
0.107692307692308,0.123076923076923,0.138461538461538,0.153846153846154,
0.169230769230769,0.184615384615385,0.2,0.215384615384615,0.230769230769231,
0.246153846153846,0.261538461538462,0.276923076923077,0.292307692307692,
0.307692307692308,0.323076923076923,0.338461538461538,0.353846153846154,
0.369230769230769,0.384615384615385,0.4,0.415384615384615,0.430769230769231,
0.446153846153846,0.461538461538462,0.476923076923077,0.492307692307692,
0.507692307692308,0.523076923076923,0.538461538461538,0.553846153846154,
0.569230769230769,0.584615384615384,0.6,0.615384615384615,0.63076923076923,
0.646153846153846,0.661538461538461,0.676923076923076,0.692307692307692,
0.707692307692307,0.723076923076922,0.738461538461538,0.753846153846153,
0.769230769230768,0.784615384615384,0.799999999999999,0.815384615384614,
0.83076923076923,0.846153846153845,0.86153846153846,0.876923076923076,0.892307692307691,
0.907692307692306,0.923076923076922,0.938461538461537,0.953846153846152,
0.969230769230768,0.984615384615383,1.),.UNSPECIFIED.)
CURVE()
GEOMETRIC_REPRESENTATION_ITEM()
RATIONAL_B_SPLINE_CURVE((1.,1.,1.,1.,1.,1.,1.,1.,1.,1.,1.,1.,1.,1.,1.,1.,
1.,1.,1.,1.,1.,1.,1.,1.,1.,1.,1.,1.,1.,1.,1.,1.,1.,1.,1.,1.,1.,1.,1.,1.,
1.,1.,1.,1.,1.,1.,1.,1.,1.,1.,1.,1.,1.,1.,1.,1.,1.,1.,1.,1.,1.,1.,1.,1.,
1.,1.,1.,1.,1.,1.))
REPRESENTATION_ITEM('')
);
#240=(
BOUNDED_CURVE()
B_SPLINE_CURVE(5,(#40898,#40899,#40900,#40901,#40902,#40903,#40904,#40905,
#40906,#40907,#40908,#40909,#40910,#40911,#40912,#40913,#40914,#40915,#40916,
#40917,#40918,#40919,#40920,#40921,#40922,#40923,#40924,#40925,#40926,#40927,
#40928,#40929,#40930,#40931,#40932,#40933,#40934,#40935,#40936,#40937,#40938,
#40939,#40940,#40941,#40942,#40943,#40944,#40945,#40946,#40947,#40948,#40949,
#40950,#40951,#40952,#40953,#40954,#40955,#40956,#40957,#40958,#40959,#40960,
#40961,#40962,#40963,#40964,#40965,#40966,#40967),.UNSPECIFIED.,.F.,.F.)
B_SPLINE_CURVE_WITH_KNOTS((6,1,1,1,1,1,1,1,1,1,1,1,1,1,1,1,1,1,1,1,1,1,
1,1,1,1,1,1,1,1,1,1,1,1,1,1,1,1,1,1,1,1,1,1,1,1,1,1,1,1,1,1,1,1,1,1,1,1,
1,1,1,1,1,1,1,6),(0.,0.0153846153846154,0.0307692307692308,0.0461538461538462,
0.0615384615384615,0.0769230769230769,0.0923076923076923,0.107692307692308,
0.123076923076923,0.138461538461538,0.153846153846154,0.169230769230769,
0.184615384615385,0.2,0.215384615384615,0.230769230769231,0.246153846153846,
0.261538461538462,0.276923076923077,0.292307692307692,0.307692307692308,
0.323076923076923,0.338461538461538,0.353846153846154,0.369230769230769,
0.384615384615385,0.4,0.415384615384615,0.430769230769231,0.446153846153846,
0.461538461538462,0.476923076923077,0.492307692307692,0.507692307692308,
0.523076923076923,0.538461538461538,0.553846153846154,0.569230769230769,
0.584615384615384,0.6,0.615384615384615,0.63076923076923,0.646153846153846,
0.661538461538461,0.676923076923076,0.692307692307692,0.707692307692307,
0.723076923076922,0.738461538461538,0.753846153846153,0.769230769230768,
0.784615384615384,0.799999999999999,0.815384615384614,0.83076923076923,
0.846153846153845,0.86153846153846,0.876923076923076,0.892307692307691,
0.907692307692306,0.923076923076922,0.938461538461537,0.953846153846152,
0.969230769230768,0.984615384615383,0.994228156739709),.UNSPECIFIED.)
CURVE()
GEOMETRIC_REPRESENTATION_ITEM()
RATIONAL_B_SPLINE_CURVE((1.,1.,1.,1.,1.,1.,1.,1.,1.,1.,1.,1.,1.,1.,1.,1.,
1.,1.,1.,1.,1.,1.,1.,1.,1.,1.,1.,1.,1.,1.,1.,1.,1.,1.,1.,1.,1.,1.,1.,1.,
1.,1.,1.,1.,1.,1.,1.,1.,1.,1.,1.,1.,1.,1.,1.,1.,1.,1.,1.,1.,1.,1.,1.,1.,
1.,1.,1.,1.,1.,1.))
REPRESENTATION_ITEM('')
);
#241=(
BOUNDED_CURVE()
B_SPLINE_CURVE(5,(#40971,#40972,#40973,#40974,#40975,#40976,#40977,#40978,
#40979,#40980,#40981,#40982,#40983,#40984,#40985,#40986,#40987,#40988,#40989,
#40990,#40991,#40992,#40993,#40994,#40995,#40996,#40997,#40998,#40999,#41000,
#41001,#41002,#41003,#41004,#41005,#41006,#41007,#41008,#41009,#41010,#41011,
#41012,#41013,#41014,#41015,#41016,#41017,#41018,#41019,#41020,#41021,#41022,
#41023,#41024,#41025,#41026,#41027,#41028,#41029,#41030,#41031,#41032,#41033,
#41034,#41035,#41036,#41037,#41038,#41039,#41040),.UNSPECIFIED.,.F.,.F.)
B_SPLINE_CURVE_WITH_KNOTS((6,1,1,1,1,1,1,1,1,1,1,1,1,1,1,1,1,1,1,1,1,1,
1,1,1,1,1,1,1,1,1,1,1,1,1,1,1,1,1,1,1,1,1,1,1,1,1,1,1,1,1,1,1,1,1,1,1,1,
1,1,1,1,1,1,1,6),(0.00577184337451094,0.0153846153846154,0.0307692307692308,
0.0461538461538462,0.0615384615384615,0.0769230769230769,0.0923076923076923,
0.107692307692308,0.123076923076923,0.138461538461538,0.153846153846154,
0.169230769230769,0.184615384615385,0.2,0.215384615384615,0.230769230769231,
0.246153846153846,0.261538461538462,0.276923076923077,0.292307692307692,
0.307692307692308,0.323076923076923,0.338461538461538,0.353846153846154,
0.369230769230769,0.384615384615385,0.4,0.415384615384615,0.430769230769231,
0.446153846153846,0.461538461538462,0.476923076923077,0.492307692307692,
0.507692307692308,0.523076923076923,0.538461538461538,0.553846153846154,
0.569230769230769,0.584615384615384,0.6,0.615384615384615,0.63076923076923,
0.646153846153846,0.661538461538461,0.676923076923076,0.692307692307692,
0.707692307692307,0.723076923076922,0.738461538461538,0.753846153846153,
0.769230769230768,0.784615384615384,0.799999999999999,0.815384615384614,
0.83076923076923,0.846153846153845,0.86153846153846,0.876923076923076,0.892307692307691,
0.907692307692306,0.923076923076922,0.938461538461537,0.953846153846152,
0.969230769230768,0.984615384615383,1.),.UNSPECIFIED.)
CURVE()
GEOMETRIC_REPRESENTATION_ITEM()
RATIONAL_B_SPLINE_CURVE((1.,1.,1.,1.,1.,1.,1.,1.,1.,1.,1.,1.,1.,1.,1.,1.,
1.,1.,1.,1.,1.,1.,1.,1.,1.,1.,1.,1.,1.,1.,1.,1.,1.,1.,1.,1.,1.,1.,1.,1.,
1.,1.,1.,1.,1.,1.,1.,1.,1.,1.,1.,1.,1.,1.,1.,1.,1.,1.,1.,1.,1.,1.,1.,1.,
1.,1.,1.,1.,1.,1.))
REPRESENTATION_ITEM('')
);
#242=(
BOUNDED_CURVE()
B_SPLINE_CURVE(5,(#41044,#41045,#41046,#41047,#41048,#41049,#41050,#41051,
#41052,#41053,#41054,#41055,#41056,#41057,#41058,#41059,#41060,#41061,#41062,
#41063,#41064,#41065,#41066,#41067,#41068,#41069,#41070,#41071,#41072,#41073,
#41074,#41075,#41076,#41077,#41078,#41079,#41080,#41081,#41082,#41083,#41084,
#41085,#41086,#41087,#41088,#41089,#41090,#41091,#41092,#41093,#41094,#41095,
#41096,#41097,#41098,#41099,#41100,#41101,#41102,#41103,#41104,#41105,#41106,
#41107,#41108,#41109,#41110,#41111,#41112,#41113),.UNSPECIFIED.,.F.,.F.)
B_SPLINE_CURVE_WITH_KNOTS((6,1,1,1,1,1,1,1,1,1,1,1,1,1,1,1,1,1,1,1,1,1,
1,1,1,1,1,1,1,1,1,1,1,1,1,1,1,1,1,1,1,1,1,1,1,1,1,1,1,1,1,1,1,1,1,1,1,1,
1,1,1,1,1,1,1,6),(0.,0.0153846153846154,0.0307692307692308,0.0461538461538462,
0.0615384615384615,0.0769230769230769,0.0923076923076923,0.107692307692308,
0.123076923076923,0.138461538461538,0.153846153846154,0.169230769230769,
0.184615384615385,0.2,0.215384615384615,0.230769230769231,0.246153846153846,
0.261538461538462,0.276923076923077,0.292307692307692,0.307692307692308,
0.323076923076923,0.338461538461538,0.353846153846154,0.369230769230769,
0.384615384615385,0.4,0.415384615384615,0.430769230769231,0.446153846153846,
0.461538461538462,0.476923076923077,0.492307692307692,0.507692307692308,
0.523076923076923,0.538461538461538,0.553846153846154,0.569230769230769,
0.584615384615384,0.6,0.615384615384615,0.63076923076923,0.646153846153846,
0.661538461538461,0.676923076923076,0.692307692307692,0.707692307692307,
0.723076923076922,0.738461538461538,0.753846153846153,0.769230769230768,
0.784615384615384,0.799999999999999,0.815384615384614,0.83076923076923,
0.846153846153845,0.86153846153846,0.876923076923076,0.892307692307691,
0.907692307692306,0.923076923076922,0.938461538461537,0.953846153846152,
0.969230769230768,0.984615384615383,0.994228156739701),.UNSPECIFIED.)
CURVE()
GEOMETRIC_REPRESENTATION_ITEM()
RATIONAL_B_SPLINE_CURVE((1.,1.,1.,1.,1.,1.,1.,1.,1.,1.,1.,1.,1.,1.,1.,1.,
1.,1.,1.,1.,1.,1.,1.,1.,1.,1.,1.,1.,1.,1.,1.,1.,1.,1.,1.,1.,1.,1.,1.,1.,
1.,1.,1.,1.,1.,1.,1.,1.,1.,1.,1.,1.,1.,1.,1.,1.,1.,1.,1.,1.,1.,1.,1.,1.,
1.,1.,1.,1.,1.,1.))
REPRESENTATION_ITEM('')
);
#243=(
BOUNDED_CURVE()
B_SPLINE_CURVE(5,(#41117,#41118,#41119,#41120,#41121,#41122,#41123,#41124,
#41125,#41126,#41127,#41128,#41129,#41130,#41131,#41132,#41133,#41134,#41135,
#41136,#41137,#41138,#41139,#41140,#41141,#41142,#41143,#41144,#41145,#41146,
#41147,#41148,#41149,#41150,#41151,#41152,#41153,#41154,#41155,#41156,#41157,
#41158,#41159,#41160,#41161,#41162,#41163,#41164,#41165,#41166,#41167,#41168,
#41169,#41170,#41171,#41172,#41173,#41174,#41175,#41176,#41177,#41178,#41179,
#41180,#41181,#41182,#41183,#41184,#41185,#41186),.UNSPECIFIED.,.F.,.F.)
B_SPLINE_CURVE_WITH_KNOTS((6,1,1,1,1,1,1,1,1,1,1,1,1,1,1,1,1,1,1,1,1,1,
1,1,1,1,1,1,1,1,1,1,1,1,1,1,1,1,1,1,1,1,1,1,1,1,1,1,1,1,1,1,1,1,1,1,1,1,
1,1,1,1,1,1,1,6),(0.0057718433745102,0.0153846153846154,0.0307692307692308,
0.0461538461538462,0.0615384615384615,0.0769230769230769,0.0923076923076923,
0.107692307692308,0.123076923076923,0.138461538461538,0.153846153846154,
0.169230769230769,0.184615384615385,0.2,0.215384615384615,0.230769230769231,
0.246153846153846,0.261538461538462,0.276923076923077,0.292307692307692,
0.307692307692308,0.323076923076923,0.338461538461538,0.353846153846154,
0.369230769230769,0.384615384615385,0.4,0.415384615384615,0.430769230769231,
0.446153846153846,0.461538461538462,0.476923076923077,0.492307692307692,
0.507692307692308,0.523076923076923,0.538461538461538,0.553846153846154,
0.569230769230769,0.584615384615384,0.6,0.615384615384615,0.63076923076923,
0.646153846153846,0.661538461538461,0.676923076923076,0.692307692307692,
0.707692307692307,0.723076923076922,0.738461538461538,0.753846153846153,
0.769230769230768,0.784615384615384,0.799999999999999,0.815384615384614,
0.83076923076923,0.846153846153845,0.86153846153846,0.876923076923076,0.892307692307691,
0.907692307692306,0.923076923076922,0.938461538461537,0.953846153846152,
0.969230769230768,0.984615384615383,1.),.UNSPECIFIED.)
CURVE()
GEOMETRIC_REPRESENTATION_ITEM()
RATIONAL_B_SPLINE_CURVE((1.,1.,1.,1.,1.,1.,1.,1.,1.,1.,1.,1.,1.,1.,1.,1.,
1.,1.,1.,1.,1.,1.,1.,1.,1.,1.,1.,1.,1.,1.,1.,1.,1.,1.,1.,1.,1.,1.,1.,1.,
1.,1.,1.,1.,1.,1.,1.,1.,1.,1.,1.,1.,1.,1.,1.,1.,1.,1.,1.,1.,1.,1.,1.,1.,
1.,1.,1.,1.,1.,1.))
REPRESENTATION_ITEM('')
);
#244=(
BOUNDED_CURVE()
B_SPLINE_CURVE(5,(#41190,#41191,#41192,#41193,#41194,#41195,#41196,#41197,
#41198,#41199,#41200,#41201,#41202,#41203,#41204,#41205,#41206,#41207,#41208,
#41209,#41210,#41211,#41212,#41213,#41214,#41215,#41216,#41217,#41218,#41219,
#41220,#41221,#41222,#41223,#41224,#41225,#41226,#41227,#41228,#41229,#41230,
#41231,#41232,#41233,#41234,#41235,#41236,#41237,#41238,#41239,#41240,#41241,
#41242,#41243,#41244,#41245,#41246,#41247,#41248,#41249,#41250,#41251,#41252,
#41253,#41254,#41255,#41256,#41257,#41258,#41259),.UNSPECIFIED.,.F.,.F.)
B_SPLINE_CURVE_WITH_KNOTS((6,1,1,1,1,1,1,1,1,1,1,1,1,1,1,1,1,1,1,1,1,1,
1,1,1,1,1,1,1,1,1,1,1,1,1,1,1,1,1,1,1,1,1,1,1,1,1,1,1,1,1,1,1,1,1,1,1,1,
1,1,1,1,1,1,1,6),(0.,0.0153846153846154,0.0307692307692308,0.0461538461538462,
0.0615384615384615,0.0769230769230769,0.0923076923076923,0.107692307692308,
0.123076923076923,0.138461538461538,0.153846153846154,0.169230769230769,
0.184615384615385,0.2,0.215384615384615,0.230769230769231,0.246153846153846,
0.261538461538462,0.276923076923077,0.292307692307692,0.307692307692308,
0.323076923076923,0.338461538461538,0.353846153846154,0.369230769230769,
0.384615384615385,0.4,0.415384615384615,0.430769230769231,0.446153846153846,
0.461538461538462,0.476923076923077,0.492307692307692,0.507692307692308,
0.523076923076923,0.538461538461538,0.553846153846154,0.569230769230769,
0.584615384615384,0.6,0.615384615384615,0.63076923076923,0.646153846153846,
0.661538461538461,0.676923076923076,0.692307692307692,0.707692307692307,
0.723076923076922,0.738461538461538,0.753846153846153,0.769230769230768,
0.784615384615384,0.799999999999999,0.815384615384614,0.83076923076923,
0.846153846153845,0.86153846153846,0.876923076923076,0.892307692307691,
0.907692307692306,0.923076923076922,0.938461538461537,0.953846153846152,
0.969230769230768,0.984615384615383,0.994228156739694),.UNSPECIFIED.)
CURVE()
GEOMETRIC_REPRESENTATION_ITEM()
RATIONAL_B_SPLINE_CURVE((1.,1.,1.,1.,1.,1.,1.,1.,1.,1.,1.,1.,1.,1.,1.,1.,
1.,1.,1.,1.,1.,1.,1.,1.,1.,1.,1.,1.,1.,1.,1.,1.,1.,1.,1.,1.,1.,1.,1.,1.,
1.,1.,1.,1.,1.,1.,1.,1.,1.,1.,1.,1.,1.,1.,1.,1.,1.,1.,1.,1.,1.,1.,1.,1.,
1.,1.,1.,1.,1.,1.))
REPRESENTATION_ITEM('')
);
#245=(
BOUNDED_CURVE()
B_SPLINE_CURVE(5,(#41263,#41264,#41265,#41266,#41267,#41268,#41269,#41270,
#41271,#41272,#41273,#41274,#41275,#41276,#41277,#41278,#41279,#41280,#41281,
#41282,#41283,#41284,#41285,#41286,#41287,#41288,#41289,#41290,#41291,#41292,
#41293,#41294,#41295,#41296,#41297,#41298,#41299,#41300,#41301,#41302,#41303,
#41304,#41305,#41306,#41307,#41308,#41309,#41310,#41311,#41312,#41313,#41314,
#41315,#41316,#41317,#41318,#41319,#41320,#41321,#41322,#41323,#41324,#41325,
#41326,#41327,#41328,#41329,#41330,#41331,#41332),.UNSPECIFIED.,.F.,.F.)
B_SPLINE_CURVE_WITH_KNOTS((6,1,1,1,1,1,1,1,1,1,1,1,1,1,1,1,1,1,1,1,1,1,
1,1,1,1,1,1,1,1,1,1,1,1,1,1,1,1,1,1,1,1,1,1,1,1,1,1,1,1,1,1,1,1,1,1,1,1,
1,1,1,1,1,1,1,6),(0.00577184337452044,0.0153846153846154,0.0307692307692308,
0.0461538461538462,0.0615384615384615,0.0769230769230769,0.0923076923076923,
0.107692307692308,0.123076923076923,0.138461538461538,0.153846153846154,
0.169230769230769,0.184615384615385,0.2,0.215384615384615,0.230769230769231,
0.246153846153846,0.261538461538462,0.276923076923077,0.292307692307692,
0.307692307692308,0.323076923076923,0.338461538461538,0.353846153846154,
0.369230769230769,0.384615384615385,0.4,0.415384615384615,0.430769230769231,
0.446153846153846,0.461538461538462,0.476923076923077,0.492307692307692,
0.507692307692308,0.523076923076923,0.538461538461538,0.553846153846154,
0.569230769230769,0.584615384615384,0.6,0.615384615384615,0.63076923076923,
0.646153846153846,0.661538461538461,0.676923076923076,0.692307692307692,
0.707692307692307,0.723076923076922,0.738461538461538,0.753846153846153,
0.769230769230768,0.784615384615384,0.799999999999999,0.815384615384614,
0.83076923076923,0.846153846153845,0.86153846153846,0.876923076923076,0.892307692307691,
0.907692307692306,0.923076923076922,0.938461538461537,0.953846153846152,
0.969230769230768,0.984615384615383,1.),.UNSPECIFIED.)
CURVE()
GEOMETRIC_REPRESENTATION_ITEM()
RATIONAL_B_SPLINE_CURVE((1.,1.,1.,1.,1.,1.,1.,1.,1.,1.,1.,1.,1.,1.,1.,1.,
1.,1.,1.,1.,1.,1.,1.,1.,1.,1.,1.,1.,1.,1.,1.,1.,1.,1.,1.,1.,1.,1.,1.,1.,
1.,1.,1.,1.,1.,1.,1.,1.,1.,1.,1.,1.,1.,1.,1.,1.,1.,1.,1.,1.,1.,1.,1.,1.,
1.,1.,1.,1.,1.,1.))
REPRESENTATION_ITEM('')
);
#246=(
BOUNDED_CURVE()
B_SPLINE_CURVE(5,(#41336,#41337,#41338,#41339,#41340,#41341,#41342,#41343,
#41344,#41345,#41346,#41347,#41348,#41349,#41350,#41351,#41352,#41353,#41354,
#41355,#41356,#41357,#41358,#41359,#41360,#41361,#41362,#41363,#41364,#41365,
#41366,#41367,#41368,#41369,#41370,#41371,#41372,#41373,#41374,#41375,#41376,
#41377,#41378,#41379,#41380,#41381,#41382,#41383,#41384,#41385,#41386,#41387,
#41388,#41389,#41390,#41391,#41392,#41393,#41394,#41395,#41396,#41397,#41398,
#41399,#41400,#41401,#41402,#41403,#41404,#41405),.UNSPECIFIED.,.F.,.F.)
B_SPLINE_CURVE_WITH_KNOTS((6,1,1,1,1,1,1,1,1,1,1,1,1,1,1,1,1,1,1,1,1,1,
1,1,1,1,1,1,1,1,1,1,1,1,1,1,1,1,1,1,1,1,1,1,1,1,1,1,1,1,1,1,1,1,1,1,1,1,
1,1,1,1,1,1,1,6),(0.,0.0153846153846154,0.0307692307692308,0.0461538461538462,
0.0615384615384615,0.0769230769230769,0.0923076923076923,0.107692307692308,
0.123076923076923,0.138461538461538,0.153846153846154,0.169230769230769,
0.184615384615385,0.2,0.215384615384615,0.230769230769231,0.246153846153846,
0.261538461538462,0.276923076923077,0.292307692307692,0.307692307692308,
0.323076923076923,0.338461538461538,0.353846153846154,0.369230769230769,
0.384615384615385,0.4,0.415384615384615,0.430769230769231,0.446153846153846,
0.461538461538462,0.476923076923077,0.492307692307692,0.507692307692308,
0.523076923076923,0.538461538461538,0.553846153846154,0.569230769230769,
0.584615384615384,0.6,0.615384615384615,0.63076923076923,0.646153846153846,
0.661538461538461,0.676923076923076,0.692307692307692,0.707692307692307,
0.723076923076922,0.738461538461538,0.753846153846153,0.769230769230768,
0.784615384615384,0.799999999999999,0.815384615384614,0.83076923076923,
0.846153846153845,0.86153846153846,0.876923076923076,0.892307692307691,
0.907692307692306,0.923076923076922,0.938461538461537,0.953846153846152,
0.969230769230768,0.984615384615383,0.994228156739698),.UNSPECIFIED.)
CURVE()
GEOMETRIC_REPRESENTATION_ITEM()
RATIONAL_B_SPLINE_CURVE((1.,1.,1.,1.,1.,1.,1.,1.,1.,1.,1.,1.,1.,1.,1.,1.,
1.,1.,1.,1.,1.,1.,1.,1.,1.,1.,1.,1.,1.,1.,1.,1.,1.,1.,1.,1.,1.,1.,1.,1.,
1.,1.,1.,1.,1.,1.,1.,1.,1.,1.,1.,1.,1.,1.,1.,1.,1.,1.,1.,1.,1.,1.,1.,1.,
1.,1.,1.,1.,1.,1.))
REPRESENTATION_ITEM('')
);
#247=(
BOUNDED_CURVE()
B_SPLINE_CURVE(5,(#41409,#41410,#41411,#41412,#41413,#41414,#41415,#41416,
#41417,#41418,#41419,#41420,#41421,#41422,#41423,#41424,#41425,#41426,#41427,
#41428,#41429,#41430,#41431,#41432,#41433,#41434,#41435,#41436,#41437,#41438,
#41439,#41440,#41441,#41442,#41443,#41444,#41445,#41446,#41447,#41448,#41449,
#41450,#41451,#41452,#41453,#41454,#41455,#41456,#41457,#41458,#41459,#41460,
#41461,#41462,#41463,#41464,#41465,#41466,#41467,#41468,#41469,#41470,#41471,
#41472,#41473,#41474,#41475,#41476,#41477,#41478),.UNSPECIFIED.,.F.,.F.)
B_SPLINE_CURVE_WITH_KNOTS((6,1,1,1,1,1,1,1,1,1,1,1,1,1,1,1,1,1,1,1,1,1,
1,1,1,1,1,1,1,1,1,1,1,1,1,1,1,1,1,1,1,1,1,1,1,1,1,1,1,1,1,1,1,1,1,1,1,1,
1,1,1,1,1,1,1,6),(0.00577184337451607,0.0153846153846154,0.0307692307692308,
0.0461538461538462,0.0615384615384615,0.0769230769230769,0.0923076923076923,
0.107692307692308,0.123076923076923,0.138461538461538,0.153846153846154,
0.169230769230769,0.184615384615385,0.2,0.215384615384615,0.230769230769231,
0.246153846153846,0.261538461538462,0.276923076923077,0.292307692307692,
0.307692307692308,0.323076923076923,0.338461538461538,0.353846153846154,
0.369230769230769,0.384615384615385,0.4,0.415384615384615,0.430769230769231,
0.446153846153846,0.461538461538462,0.476923076923077,0.492307692307692,
0.507692307692308,0.523076923076923,0.538461538461538,0.553846153846154,
0.569230769230769,0.584615384615384,0.6,0.615384615384615,0.63076923076923,
0.646153846153846,0.661538461538461,0.676923076923076,0.692307692307692,
0.707692307692307,0.723076923076922,0.738461538461538,0.753846153846153,
0.769230769230768,0.784615384615384,0.799999999999999,0.815384615384614,
0.83076923076923,0.846153846153845,0.86153846153846,0.876923076923076,0.892307692307691,
0.907692307692306,0.923076923076922,0.938461538461537,0.953846153846152,
0.969230769230768,0.984615384615383,1.),.UNSPECIFIED.)
CURVE()
GEOMETRIC_REPRESENTATION_ITEM()
RATIONAL_B_SPLINE_CURVE((1.,1.,1.,1.,1.,1.,1.,1.,1.,1.,1.,1.,1.,1.,1.,1.,
1.,1.,1.,1.,1.,1.,1.,1.,1.,1.,1.,1.,1.,1.,1.,1.,1.,1.,1.,1.,1.,1.,1.,1.,
1.,1.,1.,1.,1.,1.,1.,1.,1.,1.,1.,1.,1.,1.,1.,1.,1.,1.,1.,1.,1.,1.,1.,1.,
1.,1.,1.,1.,1.,1.))
REPRESENTATION_ITEM('')
);
#248=(
BOUNDED_CURVE()
B_SPLINE_CURVE(5,(#41482,#41483,#41484,#41485,#41486,#41487,#41488,#41489,
#41490,#41491,#41492,#41493,#41494,#41495,#41496,#41497,#41498,#41499,#41500,
#41501,#41502,#41503,#41504,#41505,#41506,#41507,#41508,#41509,#41510,#41511,
#41512,#41513,#41514,#41515,#41516,#41517,#41518,#41519,#41520,#41521,#41522,
#41523,#41524,#41525,#41526,#41527,#41528,#41529,#41530,#41531,#41532,#41533,
#41534,#41535,#41536,#41537,#41538,#41539,#41540,#41541,#41542,#41543,#41544,
#41545,#41546,#41547,#41548,#41549,#41550,#41551),.UNSPECIFIED.,.F.,.F.)
B_SPLINE_CURVE_WITH_KNOTS((6,1,1,1,1,1,1,1,1,1,1,1,1,1,1,1,1,1,1,1,1,1,
1,1,1,1,1,1,1,1,1,1,1,1,1,1,1,1,1,1,1,1,1,1,1,1,1,1,1,1,1,1,1,1,1,1,1,1,
1,1,1,1,1,1,1,6),(0.,0.0153846153846154,0.0307692307692308,0.0461538461538462,
0.0615384615384615,0.0769230769230769,0.0923076923076923,0.107692307692308,
0.123076923076923,0.138461538461538,0.153846153846154,0.169230769230769,
0.184615384615385,0.2,0.215384615384615,0.230769230769231,0.246153846153846,
0.261538461538462,0.276923076923077,0.292307692307692,0.307692307692308,
0.323076923076923,0.338461538461538,0.353846153846154,0.369230769230769,
0.384615384615385,0.4,0.415384615384615,0.430769230769231,0.446153846153846,
0.461538461538462,0.476923076923077,0.492307692307692,0.507692307692308,
0.523076923076923,0.538461538461538,0.553846153846154,0.569230769230769,
0.584615384615384,0.6,0.615384615384615,0.63076923076923,0.646153846153846,
0.661538461538461,0.676923076923076,0.692307692307692,0.707692307692307,
0.723076923076922,0.738461538461538,0.753846153846153,0.769230769230768,
0.784615384615384,0.799999999999999,0.815384615384614,0.83076923076923,
0.846153846153845,0.86153846153846,0.876923076923076,0.892307692307691,
0.907692307692306,0.923076923076922,0.938461538461537,0.953846153846152,
0.969230769230768,0.984615384615383,0.994228156739704),.UNSPECIFIED.)
CURVE()
GEOMETRIC_REPRESENTATION_ITEM()
RATIONAL_B_SPLINE_CURVE((1.,1.,1.,1.,1.,1.,1.,1.,1.,1.,1.,1.,1.,1.,1.,1.,
1.,1.,1.,1.,1.,1.,1.,1.,1.,1.,1.,1.,1.,1.,1.,1.,1.,1.,1.,1.,1.,1.,1.,1.,
1.,1.,1.,1.,1.,1.,1.,1.,1.,1.,1.,1.,1.,1.,1.,1.,1.,1.,1.,1.,1.,1.,1.,1.,
1.,1.,1.,1.,1.,1.))
REPRESENTATION_ITEM('')
);
#249=(
BOUNDED_CURVE()
B_SPLINE_CURVE(5,(#41555,#41556,#41557,#41558,#41559,#41560,#41561,#41562,
#41563,#41564,#41565,#41566,#41567,#41568,#41569,#41570,#41571,#41572,#41573,
#41574,#41575,#41576,#41577,#41578,#41579,#41580,#41581,#41582,#41583,#41584,
#41585,#41586,#41587,#41588,#41589,#41590,#41591,#41592,#41593,#41594,#41595,
#41596,#41597,#41598,#41599,#41600,#41601,#41602,#41603,#41604,#41605,#41606,
#41607,#41608,#41609,#41610,#41611,#41612,#41613,#41614,#41615,#41616,#41617,
#41618,#41619,#41620,#41621,#41622,#41623,#41624),.UNSPECIFIED.,.F.,.F.)
B_SPLINE_CURVE_WITH_KNOTS((6,1,1,1,1,1,1,1,1,1,1,1,1,1,1,1,1,1,1,1,1,1,
1,1,1,1,1,1,1,1,1,1,1,1,1,1,1,1,1,1,1,1,1,1,1,1,1,1,1,1,1,1,1,1,1,1,1,1,
1,1,1,1,1,1,1,6),(0.00577184337449682,0.0153846153846154,0.0307692307692308,
0.0461538461538462,0.0615384615384615,0.0769230769230769,0.0923076923076923,
0.107692307692308,0.123076923076923,0.138461538461538,0.153846153846154,
0.169230769230769,0.184615384615385,0.2,0.215384615384615,0.230769230769231,
0.246153846153846,0.261538461538462,0.276923076923077,0.292307692307692,
0.307692307692308,0.323076923076923,0.338461538461538,0.353846153846154,
0.369230769230769,0.384615384615385,0.4,0.415384615384615,0.430769230769231,
0.446153846153846,0.461538461538462,0.476923076923077,0.492307692307692,
0.507692307692308,0.523076923076923,0.538461538461538,0.553846153846154,
0.569230769230769,0.584615384615384,0.6,0.615384615384615,0.63076923076923,
0.646153846153846,0.661538461538461,0.676923076923076,0.692307692307692,
0.707692307692307,0.723076923076922,0.738461538461538,0.753846153846153,
0.769230769230768,0.784615384615384,0.799999999999999,0.815384615384614,
0.83076923076923,0.846153846153845,0.86153846153846,0.876923076923076,0.892307692307691,
0.907692307692306,0.923076923076922,0.938461538461537,0.953846153846152,
0.969230769230768,0.984615384615383,1.),.UNSPECIFIED.)
CURVE()
GEOMETRIC_REPRESENTATION_ITEM()
RATIONAL_B_SPLINE_CURVE((1.,1.,1.,1.,1.,1.,1.,1.,1.,1.,1.,1.,1.,1.,1.,1.,
1.,1.,1.,1.,1.,1.,1.,1.,1.,1.,1.,1.,1.,1.,1.,1.,1.,1.,1.,1.,1.,1.,1.,1.,
1.,1.,1.,1.,1.,1.,1.,1.,1.,1.,1.,1.,1.,1.,1.,1.,1.,1.,1.,1.,1.,1.,1.,1.,
1.,1.,1.,1.,1.,1.))
REPRESENTATION_ITEM('')
);
#250=(
BOUNDED_CURVE()
B_SPLINE_CURVE(5,(#41628,#41629,#41630,#41631,#41632,#41633,#41634,#41635,
#41636,#41637,#41638,#41639,#41640,#41641,#41642,#41643,#41644,#41645,#41646,
#41647,#41648,#41649,#41650,#41651,#41652,#41653,#41654,#41655,#41656,#41657,
#41658,#41659,#41660,#41661,#41662,#41663,#41664,#41665,#41666,#41667,#41668,
#41669,#41670,#41671,#41672,#41673,#41674,#41675,#41676,#41677,#41678,#41679,
#41680,#41681,#41682,#41683,#41684,#41685,#41686,#41687,#41688,#41689,#41690,
#41691,#41692,#41693,#41694,#41695,#41696,#41697),.UNSPECIFIED.,.F.,.F.)
B_SPLINE_CURVE_WITH_KNOTS((6,1,1,1,1,1,1,1,1,1,1,1,1,1,1,1,1,1,1,1,1,1,
1,1,1,1,1,1,1,1,1,1,1,1,1,1,1,1,1,1,1,1,1,1,1,1,1,1,1,1,1,1,1,1,1,1,1,1,
1,1,1,1,1,1,1,6),(0.,0.0153846153846154,0.0307692307692308,0.0461538461538462,
0.0615384615384615,0.0769230769230769,0.0923076923076923,0.107692307692308,
0.123076923076923,0.138461538461538,0.153846153846154,0.169230769230769,
0.184615384615385,0.2,0.215384615384615,0.230769230769231,0.246153846153846,
0.261538461538462,0.276923076923077,0.292307692307692,0.307692307692308,
0.323076923076923,0.338461538461538,0.353846153846154,0.369230769230769,
0.384615384615385,0.4,0.415384615384615,0.430769230769231,0.446153846153846,
0.461538461538462,0.476923076923077,0.492307692307692,0.507692307692308,
0.523076923076923,0.538461538461538,0.553846153846154,0.569230769230769,
0.584615384615384,0.6,0.615384615384615,0.63076923076923,0.646153846153846,
0.661538461538461,0.676923076923076,0.692307692307692,0.707692307692307,
0.723076923076922,0.738461538461538,0.753846153846153,0.769230769230768,
0.784615384615384,0.799999999999999,0.815384615384614,0.83076923076923,
0.846153846153845,0.86153846153846,0.876923076923076,0.892307692307691,
0.907692307692306,0.923076923076922,0.938461538461537,0.953846153846152,
0.969230769230768,0.984615384615383,0.994228156739711),.UNSPECIFIED.)
CURVE()
GEOMETRIC_REPRESENTATION_ITEM()
RATIONAL_B_SPLINE_CURVE((1.,1.,1.,1.,1.,1.,1.,1.,1.,1.,1.,1.,1.,1.,1.,1.,
1.,1.,1.,1.,1.,1.,1.,1.,1.,1.,1.,1.,1.,1.,1.,1.,1.,1.,1.,1.,1.,1.,1.,1.,
1.,1.,1.,1.,1.,1.,1.,1.,1.,1.,1.,1.,1.,1.,1.,1.,1.,1.,1.,1.,1.,1.,1.,1.,
1.,1.,1.,1.,1.,1.))
REPRESENTATION_ITEM('')
);
#251=(
BOUNDED_CURVE()
B_SPLINE_CURVE(5,(#41701,#41702,#41703,#41704,#41705,#41706,#41707,#41708,
#41709,#41710,#41711,#41712,#41713,#41714,#41715,#41716,#41717,#41718,#41719,
#41720,#41721,#41722,#41723,#41724,#41725,#41726,#41727,#41728,#41729,#41730,
#41731,#41732,#41733,#41734,#41735,#41736,#41737,#41738,#41739,#41740,#41741,
#41742,#41743,#41744,#41745,#41746,#41747,#41748,#41749,#41750,#41751,#41752,
#41753,#41754,#41755,#41756,#41757,#41758,#41759,#41760,#41761,#41762,#41763,
#41764,#41765,#41766,#41767,#41768,#41769,#41770),.UNSPECIFIED.,.F.,.F.)
B_SPLINE_CURVE_WITH_KNOTS((6,1,1,1,1,1,1,1,1,1,1,1,1,1,1,1,1,1,1,1,1,1,
1,1,1,1,1,1,1,1,1,1,1,1,1,1,1,1,1,1,1,1,1,1,1,1,1,1,1,1,1,1,1,1,1,1,1,1,
1,1,1,1,1,1,1,6),(0.00577184337450313,0.0153846153846154,0.0307692307692308,
0.0461538461538462,0.0615384615384615,0.0769230769230769,0.0923076923076923,
0.107692307692308,0.123076923076923,0.138461538461538,0.153846153846154,
0.169230769230769,0.184615384615385,0.2,0.215384615384615,0.230769230769231,
0.246153846153846,0.261538461538462,0.276923076923077,0.292307692307692,
0.307692307692308,0.323076923076923,0.338461538461538,0.353846153846154,
0.369230769230769,0.384615384615385,0.4,0.415384615384615,0.430769230769231,
0.446153846153846,0.461538461538462,0.476923076923077,0.492307692307692,
0.507692307692308,0.523076923076923,0.538461538461538,0.553846153846154,
0.569230769230769,0.584615384615384,0.6,0.615384615384615,0.63076923076923,
0.646153846153846,0.661538461538461,0.676923076923076,0.692307692307692,
0.707692307692307,0.723076923076922,0.738461538461538,0.753846153846153,
0.769230769230768,0.784615384615384,0.799999999999999,0.815384615384614,
0.83076923076923,0.846153846153845,0.86153846153846,0.876923076923076,0.892307692307691,
0.907692307692306,0.923076923076922,0.938461538461537,0.953846153846152,
0.969230769230768,0.984615384615383,1.),.UNSPECIFIED.)
CURVE()
GEOMETRIC_REPRESENTATION_ITEM()
RATIONAL_B_SPLINE_CURVE((1.,1.,1.,1.,1.,1.,1.,1.,1.,1.,1.,1.,1.,1.,1.,1.,
1.,1.,1.,1.,1.,1.,1.,1.,1.,1.,1.,1.,1.,1.,1.,1.,1.,1.,1.,1.,1.,1.,1.,1.,
1.,1.,1.,1.,1.,1.,1.,1.,1.,1.,1.,1.,1.,1.,1.,1.,1.,1.,1.,1.,1.,1.,1.,1.,
1.,1.,1.,1.,1.,1.))
REPRESENTATION_ITEM('')
);
#252=(
BOUNDED_CURVE()
B_SPLINE_CURVE(5,(#41774,#41775,#41776,#41777,#41778,#41779,#41780,#41781,
#41782,#41783,#41784,#41785,#41786,#41787,#41788,#41789,#41790,#41791,#41792,
#41793,#41794,#41795,#41796,#41797,#41798,#41799,#41800,#41801,#41802,#41803,
#41804,#41805,#41806,#41807,#41808,#41809,#41810,#41811,#41812,#41813,#41814,
#41815,#41816,#41817,#41818,#41819,#41820,#41821,#41822,#41823,#41824,#41825,
#41826,#41827,#41828,#41829,#41830,#41831,#41832,#41833,#41834,#41835,#41836,
#41837,#41838,#41839,#41840,#41841,#41842,#41843),.UNSPECIFIED.,.F.,.F.)
B_SPLINE_CURVE_WITH_KNOTS((6,1,1,1,1,1,1,1,1,1,1,1,1,1,1,1,1,1,1,1,1,1,
1,1,1,1,1,1,1,1,1,1,1,1,1,1,1,1,1,1,1,1,1,1,1,1,1,1,1,1,1,1,1,1,1,1,1,1,
1,1,1,1,1,1,1,6),(0.,0.0153846153846154,0.0307692307692308,0.0461538461538462,
0.0615384615384615,0.0769230769230769,0.0923076923076923,0.107692307692308,
0.123076923076923,0.138461538461538,0.153846153846154,0.169230769230769,
0.184615384615385,0.2,0.215384615384615,0.230769230769231,0.246153846153846,
0.261538461538462,0.276923076923077,0.292307692307692,0.307692307692308,
0.323076923076923,0.338461538461538,0.353846153846154,0.369230769230769,
0.384615384615385,0.4,0.415384615384615,0.430769230769231,0.446153846153846,
0.461538461538462,0.476923076923077,0.492307692307692,0.507692307692308,
0.523076923076923,0.538461538461538,0.553846153846154,0.569230769230769,
0.584615384615384,0.6,0.615384615384615,0.63076923076923,0.646153846153846,
0.661538461538461,0.676923076923076,0.692307692307692,0.707692307692307,
0.723076923076922,0.738461538461538,0.753846153846153,0.769230769230768,
0.784615384615384,0.799999999999999,0.815384615384614,0.83076923076923,
0.846153846153845,0.86153846153846,0.876923076923076,0.892307692307691,
0.907692307692306,0.923076923076922,0.938461538461537,0.953846153846152,
0.969230769230768,0.984615384615383,0.9942281567397),.UNSPECIFIED.)
CURVE()
GEOMETRIC_REPRESENTATION_ITEM()
RATIONAL_B_SPLINE_CURVE((1.,1.,1.,1.,1.,1.,1.,1.,1.,1.,1.,1.,1.,1.,1.,1.,
1.,1.,1.,1.,1.,1.,1.,1.,1.,1.,1.,1.,1.,1.,1.,1.,1.,1.,1.,1.,1.,1.,1.,1.,
1.,1.,1.,1.,1.,1.,1.,1.,1.,1.,1.,1.,1.,1.,1.,1.,1.,1.,1.,1.,1.,1.,1.,1.,
1.,1.,1.,1.,1.,1.))
REPRESENTATION_ITEM('')
);
#253=(
BOUNDED_CURVE()
B_SPLINE_CURVE(5,(#41847,#41848,#41849,#41850,#41851,#41852,#41853,#41854,
#41855,#41856,#41857,#41858,#41859,#41860,#41861,#41862,#41863,#41864,#41865,
#41866,#41867,#41868,#41869,#41870,#41871,#41872,#41873,#41874,#41875,#41876,
#41877,#41878,#41879,#41880,#41881,#41882,#41883,#41884,#41885,#41886,#41887,
#41888,#41889,#41890,#41891,#41892,#41893,#41894,#41895,#41896,#41897,#41898,
#41899,#41900,#41901,#41902,#41903,#41904,#41905,#41906,#41907,#41908,#41909,
#41910,#41911,#41912,#41913,#41914,#41915,#41916),.UNSPECIFIED.,.F.,.F.)
B_SPLINE_CURVE_WITH_KNOTS((6,1,1,1,1,1,1,1,1,1,1,1,1,1,1,1,1,1,1,1,1,1,
1,1,1,1,1,1,1,1,1,1,1,1,1,1,1,1,1,1,1,1,1,1,1,1,1,1,1,1,1,1,1,1,1,1,1,1,
1,1,1,1,1,1,1,6),(0.00577184337452087,0.0153846153846154,0.0307692307692308,
0.0461538461538462,0.0615384615384615,0.0769230769230769,0.0923076923076923,
0.107692307692308,0.123076923076923,0.138461538461538,0.153846153846154,
0.169230769230769,0.184615384615385,0.2,0.215384615384615,0.230769230769231,
0.246153846153846,0.261538461538462,0.276923076923077,0.292307692307692,
0.307692307692308,0.323076923076923,0.338461538461538,0.353846153846154,
0.369230769230769,0.384615384615385,0.4,0.415384615384615,0.430769230769231,
0.446153846153846,0.461538461538462,0.476923076923077,0.492307692307692,
0.507692307692308,0.523076923076923,0.538461538461538,0.553846153846154,
0.569230769230769,0.584615384615384,0.6,0.615384615384615,0.63076923076923,
0.646153846153846,0.661538461538461,0.676923076923076,0.692307692307692,
0.707692307692307,0.723076923076922,0.738461538461538,0.753846153846153,
0.769230769230768,0.784615384615384,0.799999999999999,0.815384615384614,
0.83076923076923,0.846153846153845,0.86153846153846,0.876923076923076,0.892307692307691,
0.907692307692306,0.923076923076922,0.938461538461537,0.953846153846152,
0.969230769230768,0.984615384615383,1.),.UNSPECIFIED.)
CURVE()
GEOMETRIC_REPRESENTATION_ITEM()
RATIONAL_B_SPLINE_CURVE((1.,1.,1.,1.,1.,1.,1.,1.,1.,1.,1.,1.,1.,1.,1.,1.,
1.,1.,1.,1.,1.,1.,1.,1.,1.,1.,1.,1.,1.,1.,1.,1.,1.,1.,1.,1.,1.,1.,1.,1.,
1.,1.,1.,1.,1.,1.,1.,1.,1.,1.,1.,1.,1.,1.,1.,1.,1.,1.,1.,1.,1.,1.,1.,1.,
1.,1.,1.,1.,1.,1.))
REPRESENTATION_ITEM('')
);
#254=(
BOUNDED_CURVE()
B_SPLINE_CURVE(5,(#41920,#41921,#41922,#41923,#41924,#41925,#41926,#41927,
#41928,#41929,#41930,#41931,#41932,#41933,#41934,#41935,#41936,#41937,#41938,
#41939,#41940,#41941,#41942,#41943,#41944,#41945,#41946,#41947,#41948,#41949,
#41950,#41951,#41952,#41953,#41954,#41955,#41956,#41957,#41958,#41959,#41960,
#41961,#41962,#41963,#41964,#41965,#41966,#41967,#41968,#41969,#41970,#41971,
#41972,#41973,#41974,#41975,#41976,#41977,#41978,#41979,#41980,#41981,#41982,
#41983,#41984,#41985,#41986,#41987,#41988,#41989),.UNSPECIFIED.,.F.,.F.)
B_SPLINE_CURVE_WITH_KNOTS((6,1,1,1,1,1,1,1,1,1,1,1,1,1,1,1,1,1,1,1,1,1,
1,1,1,1,1,1,1,1,1,1,1,1,1,1,1,1,1,1,1,1,1,1,1,1,1,1,1,1,1,1,1,1,1,1,1,1,
1,1,1,1,1,1,1,6),(0.,0.0153846153846154,0.0307692307692308,0.0461538461538462,
0.0615384615384615,0.0769230769230769,0.0923076923076923,0.107692307692308,
0.123076923076923,0.138461538461538,0.153846153846154,0.169230769230769,
0.184615384615385,0.2,0.215384615384615,0.230769230769231,0.246153846153846,
0.261538461538462,0.276923076923077,0.292307692307692,0.307692307692308,
0.323076923076923,0.338461538461538,0.353846153846154,0.369230769230769,
0.384615384615385,0.4,0.415384615384615,0.430769230769231,0.446153846153846,
0.461538461538462,0.476923076923077,0.492307692307692,0.507692307692308,
0.523076923076923,0.538461538461538,0.553846153846154,0.569230769230769,
0.584615384615384,0.6,0.615384615384615,0.63076923076923,0.646153846153846,
0.661538461538461,0.676923076923076,0.692307692307692,0.707692307692307,
0.723076923076922,0.738461538461538,0.753846153846153,0.769230769230768,
0.784615384615384,0.799999999999999,0.815384615384614,0.83076923076923,
0.846153846153845,0.86153846153846,0.876923076923076,0.892307692307691,
0.907692307692306,0.923076923076922,0.938461538461537,0.953846153846152,
0.969230769230768,0.984615384615383,0.994228156739692),.UNSPECIFIED.)
CURVE()
GEOMETRIC_REPRESENTATION_ITEM()
RATIONAL_B_SPLINE_CURVE((1.,1.,1.,1.,1.,1.,1.,1.,1.,1.,1.,1.,1.,1.,1.,1.,
1.,1.,1.,1.,1.,1.,1.,1.,1.,1.,1.,1.,1.,1.,1.,1.,1.,1.,1.,1.,1.,1.,1.,1.,
1.,1.,1.,1.,1.,1.,1.,1.,1.,1.,1.,1.,1.,1.,1.,1.,1.,1.,1.,1.,1.,1.,1.,1.,
1.,1.,1.,1.,1.,1.))
REPRESENTATION_ITEM('')
);
#255=(
BOUNDED_CURVE()
B_SPLINE_CURVE(5,(#41993,#41994,#41995,#41996,#41997,#41998,#41999,#42000,
#42001,#42002,#42003,#42004,#42005,#42006,#42007,#42008,#42009,#42010,#42011,
#42012,#42013,#42014,#42015,#42016,#42017,#42018,#42019,#42020,#42021,#42022,
#42023,#42024,#42025,#42026,#42027,#42028,#42029,#42030,#42031,#42032,#42033,
#42034,#42035,#42036,#42037,#42038,#42039,#42040,#42041,#42042,#42043,#42044,
#42045,#42046,#42047,#42048,#42049,#42050,#42051,#42052,#42053,#42054,#42055,
#42056,#42057,#42058,#42059,#42060,#42061,#42062),.UNSPECIFIED.,.F.,.F.)
B_SPLINE_CURVE_WITH_KNOTS((6,1,1,1,1,1,1,1,1,1,1,1,1,1,1,1,1,1,1,1,1,1,
1,1,1,1,1,1,1,1,1,1,1,1,1,1,1,1,1,1,1,1,1,1,1,1,1,1,1,1,1,1,1,1,1,1,1,1,
1,1,1,1,1,1,1,6),(0.00577184337450777,0.0153846153846154,0.0307692307692308,
0.0461538461538462,0.0615384615384615,0.0769230769230769,0.0923076923076923,
0.107692307692308,0.123076923076923,0.138461538461538,0.153846153846154,
0.169230769230769,0.184615384615385,0.2,0.215384615384615,0.230769230769231,
0.246153846153846,0.261538461538462,0.276923076923077,0.292307692307692,
0.307692307692308,0.323076923076923,0.338461538461538,0.353846153846154,
0.369230769230769,0.384615384615385,0.4,0.415384615384615,0.430769230769231,
0.446153846153846,0.461538461538462,0.476923076923077,0.492307692307692,
0.507692307692308,0.523076923076923,0.538461538461538,0.553846153846154,
0.569230769230769,0.584615384615384,0.6,0.615384615384615,0.63076923076923,
0.646153846153846,0.661538461538461,0.676923076923076,0.692307692307692,
0.707692307692307,0.723076923076922,0.738461538461538,0.753846153846153,
0.769230769230768,0.784615384615384,0.799999999999999,0.815384615384614,
0.83076923076923,0.846153846153845,0.86153846153846,0.876923076923076,0.892307692307691,
0.907692307692306,0.923076923076922,0.938461538461537,0.953846153846152,
0.969230769230768,0.984615384615383,1.),.UNSPECIFIED.)
CURVE()
GEOMETRIC_REPRESENTATION_ITEM()
RATIONAL_B_SPLINE_CURVE((1.,1.,1.,1.,1.,1.,1.,1.,1.,1.,1.,1.,1.,1.,1.,1.,
1.,1.,1.,1.,1.,1.,1.,1.,1.,1.,1.,1.,1.,1.,1.,1.,1.,1.,1.,1.,1.,1.,1.,1.,
1.,1.,1.,1.,1.,1.,1.,1.,1.,1.,1.,1.,1.,1.,1.,1.,1.,1.,1.,1.,1.,1.,1.,1.,
1.,1.,1.,1.,1.,1.))
REPRESENTATION_ITEM('')
);
#256=(
BOUNDED_CURVE()
B_SPLINE_CURVE(5,(#42066,#42067,#42068,#42069,#42070,#42071,#42072,#42073,
#42074,#42075,#42076,#42077,#42078,#42079,#42080,#42081,#42082,#42083,#42084,
#42085,#42086,#42087,#42088,#42089,#42090,#42091,#42092,#42093,#42094,#42095,
#42096,#42097,#42098,#42099,#42100,#42101,#42102,#42103,#42104,#42105,#42106,
#42107,#42108,#42109,#42110,#42111,#42112,#42113,#42114,#42115,#42116,#42117,
#42118,#42119,#42120,#42121,#42122,#42123,#42124,#42125,#42126,#42127,#42128,
#42129,#42130,#42131,#42132,#42133,#42134,#42135),.UNSPECIFIED.,.F.,.F.)
B_SPLINE_CURVE_WITH_KNOTS((6,1,1,1,1,1,1,1,1,1,1,1,1,1,1,1,1,1,1,1,1,1,
1,1,1,1,1,1,1,1,1,1,1,1,1,1,1,1,1,1,1,1,1,1,1,1,1,1,1,1,1,1,1,1,1,1,1,1,
1,1,1,1,1,1,1,6),(0.,0.0153846153846154,0.0307692307692308,0.0461538461538462,
0.0615384615384615,0.0769230769230769,0.0923076923076923,0.107692307692308,
0.123076923076923,0.138461538461538,0.153846153846154,0.169230769230769,
0.184615384615385,0.2,0.215384615384615,0.230769230769231,0.246153846153846,
0.261538461538462,0.276923076923077,0.292307692307692,0.307692307692308,
0.323076923076923,0.338461538461538,0.353846153846154,0.369230769230769,
0.384615384615385,0.4,0.415384615384615,0.430769230769231,0.446153846153846,
0.461538461538462,0.476923076923077,0.492307692307692,0.507692307692308,
0.523076923076923,0.538461538461538,0.553846153846154,0.569230769230769,
0.584615384615384,0.6,0.615384615384615,0.63076923076923,0.646153846153846,
0.661538461538461,0.676923076923076,0.692307692307692,0.707692307692307,
0.723076923076922,0.738461538461538,0.753846153846153,0.769230769230768,
0.784615384615384,0.799999999999999,0.815384615384614,0.83076923076923,
0.846153846153845,0.86153846153846,0.876923076923076,0.892307692307691,
0.907692307692306,0.923076923076922,0.938461538461537,0.953846153846152,
0.969230769230768,0.984615384615383,0.994228156739701),.UNSPECIFIED.)
CURVE()
GEOMETRIC_REPRESENTATION_ITEM()
RATIONAL_B_SPLINE_CURVE((1.,1.,1.,1.,1.,1.,1.,1.,1.,1.,1.,1.,1.,1.,1.,1.,
1.,1.,1.,1.,1.,1.,1.,1.,1.,1.,1.,1.,1.,1.,1.,1.,1.,1.,1.,1.,1.,1.,1.,1.,
1.,1.,1.,1.,1.,1.,1.,1.,1.,1.,1.,1.,1.,1.,1.,1.,1.,1.,1.,1.,1.,1.,1.,1.,
1.,1.,1.,1.,1.,1.))
REPRESENTATION_ITEM('')
);
#257=(
BOUNDED_CURVE()
B_SPLINE_CURVE(5,(#42139,#42140,#42141,#42142,#42143,#42144,#42145,#42146,
#42147,#42148,#42149,#42150,#42151,#42152,#42153,#42154,#42155,#42156,#42157,
#42158,#42159,#42160,#42161,#42162,#42163,#42164,#42165,#42166,#42167,#42168,
#42169,#42170,#42171,#42172,#42173,#42174,#42175,#42176,#42177,#42178,#42179,
#42180,#42181,#42182,#42183,#42184,#42185,#42186,#42187,#42188,#42189,#42190,
#42191,#42192,#42193,#42194,#42195,#42196,#42197,#42198,#42199,#42200,#42201,
#42202,#42203,#42204,#42205,#42206,#42207,#42208),.UNSPECIFIED.,.F.,.F.)
B_SPLINE_CURVE_WITH_KNOTS((6,1,1,1,1,1,1,1,1,1,1,1,1,1,1,1,1,1,1,1,1,1,
1,1,1,1,1,1,1,1,1,1,1,1,1,1,1,1,1,1,1,1,1,1,1,1,1,1,1,1,1,1,1,1,1,1,1,1,
1,1,1,1,1,1,1,6),(0.00577184337450943,0.0153846153846154,0.0307692307692308,
0.0461538461538462,0.0615384615384615,0.0769230769230769,0.0923076923076923,
0.107692307692308,0.123076923076923,0.138461538461538,0.153846153846154,
0.169230769230769,0.184615384615385,0.2,0.215384615384615,0.230769230769231,
0.246153846153846,0.261538461538462,0.276923076923077,0.292307692307692,
0.307692307692308,0.323076923076923,0.338461538461538,0.353846153846154,
0.369230769230769,0.384615384615385,0.4,0.415384615384615,0.430769230769231,
0.446153846153846,0.461538461538462,0.476923076923077,0.492307692307692,
0.507692307692308,0.523076923076923,0.538461538461538,0.553846153846154,
0.569230769230769,0.584615384615384,0.6,0.615384615384615,0.63076923076923,
0.646153846153846,0.661538461538461,0.676923076923076,0.692307692307692,
0.707692307692307,0.723076923076922,0.738461538461538,0.753846153846153,
0.769230769230768,0.784615384615384,0.799999999999999,0.815384615384614,
0.83076923076923,0.846153846153845,0.86153846153846,0.876923076923076,0.892307692307691,
0.907692307692306,0.923076923076922,0.938461538461537,0.953846153846152,
0.969230769230768,0.984615384615383,1.),.UNSPECIFIED.)
CURVE()
GEOMETRIC_REPRESENTATION_ITEM()
RATIONAL_B_SPLINE_CURVE((1.,1.,1.,1.,1.,1.,1.,1.,1.,1.,1.,1.,1.,1.,1.,1.,
1.,1.,1.,1.,1.,1.,1.,1.,1.,1.,1.,1.,1.,1.,1.,1.,1.,1.,1.,1.,1.,1.,1.,1.,
1.,1.,1.,1.,1.,1.,1.,1.,1.,1.,1.,1.,1.,1.,1.,1.,1.,1.,1.,1.,1.,1.,1.,1.,
1.,1.,1.,1.,1.,1.))
REPRESENTATION_ITEM('')
);
#258=(
BOUNDED_CURVE()
B_SPLINE_CURVE(5,(#42212,#42213,#42214,#42215,#42216,#42217,#42218,#42219,
#42220,#42221,#42222,#42223,#42224,#42225,#42226,#42227,#42228,#42229,#42230,
#42231,#42232,#42233,#42234,#42235,#42236,#42237,#42238,#42239,#42240,#42241,
#42242,#42243,#42244,#42245,#42246,#42247,#42248,#42249,#42250,#42251,#42252,
#42253,#42254,#42255,#42256,#42257,#42258,#42259,#42260,#42261,#42262,#42263,
#42264,#42265,#42266,#42267,#42268,#42269,#42270,#42271,#42272,#42273,#42274,
#42275,#42276,#42277,#42278,#42279,#42280,#42281),.UNSPECIFIED.,.F.,.F.)
B_SPLINE_CURVE_WITH_KNOTS((6,1,1,1,1,1,1,1,1,1,1,1,1,1,1,1,1,1,1,1,1,1,
1,1,1,1,1,1,1,1,1,1,1,1,1,1,1,1,1,1,1,1,1,1,1,1,1,1,1,1,1,1,1,1,1,1,1,1,
1,1,1,1,1,1,1,6),(0.,0.0153846153846154,0.0307692307692308,0.0461538461538462,
0.0615384615384615,0.0769230769230769,0.0923076923076923,0.107692307692308,
0.123076923076923,0.138461538461538,0.153846153846154,0.169230769230769,
0.184615384615385,0.2,0.215384615384615,0.230769230769231,0.246153846153846,
0.261538461538462,0.276923076923077,0.292307692307692,0.307692307692308,
0.323076923076923,0.338461538461538,0.353846153846154,0.369230769230769,
0.384615384615385,0.4,0.415384615384615,0.430769230769231,0.446153846153846,
0.461538461538462,0.476923076923077,0.492307692307692,0.507692307692308,
0.523076923076923,0.538461538461538,0.553846153846154,0.569230769230769,
0.584615384615384,0.6,0.615384615384615,0.63076923076923,0.646153846153846,
0.661538461538461,0.676923076923076,0.692307692307692,0.707692307692307,
0.723076923076922,0.738461538461538,0.753846153846153,0.769230769230768,
0.784615384615384,0.799999999999999,0.815384615384614,0.83076923076923,
0.846153846153845,0.86153846153846,0.876923076923076,0.892307692307691,
0.907692307692306,0.923076923076922,0.938461538461537,0.953846153846152,
0.969230769230768,0.984615384615383,0.994228156739699),.UNSPECIFIED.)
CURVE()
GEOMETRIC_REPRESENTATION_ITEM()
RATIONAL_B_SPLINE_CURVE((1.,1.,1.,1.,1.,1.,1.,1.,1.,1.,1.,1.,1.,1.,1.,1.,
1.,1.,1.,1.,1.,1.,1.,1.,1.,1.,1.,1.,1.,1.,1.,1.,1.,1.,1.,1.,1.,1.,1.,1.,
1.,1.,1.,1.,1.,1.,1.,1.,1.,1.,1.,1.,1.,1.,1.,1.,1.,1.,1.,1.,1.,1.,1.,1.,
1.,1.,1.,1.,1.,1.))
REPRESENTATION_ITEM('')
);
#259=(
BOUNDED_CURVE()
B_SPLINE_CURVE(5,(#42285,#42286,#42287,#42288,#42289,#42290,#42291,#42292,
#42293,#42294,#42295,#42296,#42297,#42298,#42299,#42300,#42301,#42302,#42303,
#42304,#42305,#42306,#42307,#42308,#42309,#42310,#42311,#42312,#42313,#42314,
#42315,#42316,#42317,#42318,#42319,#42320,#42321,#42322,#42323,#42324,#42325,
#42326,#42327,#42328,#42329,#42330,#42331,#42332,#42333,#42334,#42335,#42336,
#42337,#42338,#42339,#42340,#42341,#42342,#42343,#42344,#42345,#42346,#42347,
#42348,#42349,#42350,#42351,#42352,#42353,#42354),.UNSPECIFIED.,.F.,.F.)
B_SPLINE_CURVE_WITH_KNOTS((6,1,1,1,1,1,1,1,1,1,1,1,1,1,1,1,1,1,1,1,1,1,
1,1,1,1,1,1,1,1,1,1,1,1,1,1,1,1,1,1,1,1,1,1,1,1,1,1,1,1,1,1,1,1,1,1,1,1,
1,1,1,1,1,1,1,6),(0.00577184337448657,0.0153846153846154,0.0307692307692308,
0.0461538461538462,0.0615384615384615,0.0769230769230769,0.0923076923076923,
0.107692307692308,0.123076923076923,0.138461538461538,0.153846153846154,
0.169230769230769,0.184615384615385,0.2,0.215384615384615,0.230769230769231,
0.246153846153846,0.261538461538462,0.276923076923077,0.292307692307692,
0.307692307692308,0.323076923076923,0.338461538461538,0.353846153846154,
0.369230769230769,0.384615384615385,0.4,0.415384615384615,0.430769230769231,
0.446153846153846,0.461538461538462,0.476923076923077,0.492307692307692,
0.507692307692308,0.523076923076923,0.538461538461538,0.553846153846154,
0.569230769230769,0.584615384615384,0.6,0.615384615384615,0.63076923076923,
0.646153846153846,0.661538461538461,0.676923076923076,0.692307692307692,
0.707692307692307,0.723076923076922,0.738461538461538,0.753846153846153,
0.769230769230768,0.784615384615384,0.799999999999999,0.815384615384614,
0.83076923076923,0.846153846153845,0.86153846153846,0.876923076923076,0.892307692307691,
0.907692307692306,0.923076923076922,0.938461538461537,0.953846153846152,
0.969230769230768,0.984615384615383,1.),.UNSPECIFIED.)
CURVE()
GEOMETRIC_REPRESENTATION_ITEM()
RATIONAL_B_SPLINE_CURVE((1.,1.,1.,1.,1.,1.,1.,1.,1.,1.,1.,1.,1.,1.,1.,1.,
1.,1.,1.,1.,1.,1.,1.,1.,1.,1.,1.,1.,1.,1.,1.,1.,1.,1.,1.,1.,1.,1.,1.,1.,
1.,1.,1.,1.,1.,1.,1.,1.,1.,1.,1.,1.,1.,1.,1.,1.,1.,1.,1.,1.,1.,1.,1.,1.,
1.,1.,1.,1.,1.,1.))
REPRESENTATION_ITEM('')
);
#260=(
BOUNDED_CURVE()
B_SPLINE_CURVE(5,(#42358,#42359,#42360,#42361,#42362,#42363,#42364,#42365,
#42366,#42367,#42368,#42369,#42370,#42371,#42372,#42373,#42374,#42375,#42376,
#42377,#42378,#42379,#42380,#42381,#42382,#42383,#42384,#42385,#42386,#42387,
#42388,#42389,#42390,#42391,#42392,#42393,#42394,#42395,#42396,#42397,#42398,
#42399,#42400,#42401,#42402,#42403,#42404,#42405,#42406,#42407,#42408,#42409,
#42410,#42411,#42412,#42413,#42414,#42415,#42416,#42417,#42418,#42419,#42420,
#42421,#42422,#42423,#42424,#42425,#42426,#42427),.UNSPECIFIED.,.F.,.F.)
B_SPLINE_CURVE_WITH_KNOTS((6,1,1,1,1,1,1,1,1,1,1,1,1,1,1,1,1,1,1,1,1,1,
1,1,1,1,1,1,1,1,1,1,1,1,1,1,1,1,1,1,1,1,1,1,1,1,1,1,1,1,1,1,1,1,1,1,1,1,
1,1,1,1,1,1,1,6),(0.,0.0153846153846154,0.0307692307692308,0.0461538461538462,
0.0615384615384615,0.0769230769230769,0.0923076923076923,0.107692307692308,
0.123076923076923,0.138461538461538,0.153846153846154,0.169230769230769,
0.184615384615385,0.2,0.215384615384615,0.230769230769231,0.246153846153846,
0.261538461538462,0.276923076923077,0.292307692307692,0.307692307692308,
0.323076923076923,0.338461538461538,0.353846153846154,0.369230769230769,
0.384615384615385,0.4,0.415384615384615,0.430769230769231,0.446153846153846,
0.461538461538462,0.476923076923077,0.492307692307692,0.507692307692308,
0.523076923076923,0.538461538461538,0.553846153846154,0.569230769230769,
0.584615384615384,0.6,0.615384615384615,0.63076923076923,0.646153846153846,
0.661538461538461,0.676923076923076,0.692307692307692,0.707692307692307,
0.723076923076922,0.738461538461538,0.753846153846153,0.769230769230768,
0.784615384615384,0.799999999999999,0.815384615384614,0.83076923076923,
0.846153846153845,0.86153846153846,0.876923076923076,0.892307692307691,
0.907692307692306,0.923076923076922,0.938461538461537,0.953846153846152,
0.969230769230768,0.984615384615383,0.994228156739709),.UNSPECIFIED.)
CURVE()
GEOMETRIC_REPRESENTATION_ITEM()
RATIONAL_B_SPLINE_CURVE((1.,1.,1.,1.,1.,1.,1.,1.,1.,1.,1.,1.,1.,1.,1.,1.,
1.,1.,1.,1.,1.,1.,1.,1.,1.,1.,1.,1.,1.,1.,1.,1.,1.,1.,1.,1.,1.,1.,1.,1.,
1.,1.,1.,1.,1.,1.,1.,1.,1.,1.,1.,1.,1.,1.,1.,1.,1.,1.,1.,1.,1.,1.,1.,1.,
1.,1.,1.,1.,1.,1.))
REPRESENTATION_ITEM('')
);
#261=(
BOUNDED_CURVE()
B_SPLINE_CURVE(5,(#42431,#42432,#42433,#42434,#42435,#42436,#42437,#42438,
#42439,#42440,#42441,#42442,#42443,#42444,#42445,#42446,#42447,#42448,#42449,
#42450,#42451,#42452,#42453,#42454,#42455,#42456,#42457,#42458,#42459,#42460,
#42461,#42462,#42463,#42464,#42465,#42466,#42467,#42468,#42469,#42470,#42471,
#42472,#42473,#42474,#42475,#42476,#42477,#42478,#42479,#42480,#42481,#42482,
#42483,#42484,#42485,#42486,#42487,#42488,#42489,#42490,#42491,#42492,#42493,
#42494,#42495,#42496,#42497,#42498,#42499,#42500),.UNSPECIFIED.,.F.,.F.)
B_SPLINE_CURVE_WITH_KNOTS((6,1,1,1,1,1,1,1,1,1,1,1,1,1,1,1,1,1,1,1,1,1,
1,1,1,1,1,1,1,1,1,1,1,1,1,1,1,1,1,1,1,1,1,1,1,1,1,1,1,1,1,1,1,1,1,1,1,1,
1,1,1,1,1,1,1,6),(0.00577184337451132,0.0153846153846154,0.0307692307692308,
0.0461538461538462,0.0615384615384615,0.0769230769230769,0.0923076923076923,
0.107692307692308,0.123076923076923,0.138461538461538,0.153846153846154,
0.169230769230769,0.184615384615385,0.2,0.215384615384615,0.230769230769231,
0.246153846153846,0.261538461538462,0.276923076923077,0.292307692307692,
0.307692307692308,0.323076923076923,0.338461538461538,0.353846153846154,
0.369230769230769,0.384615384615385,0.4,0.415384615384615,0.430769230769231,
0.446153846153846,0.461538461538462,0.476923076923077,0.492307692307692,
0.507692307692308,0.523076923076923,0.538461538461538,0.553846153846154,
0.569230769230769,0.584615384615384,0.6,0.615384615384615,0.63076923076923,
0.646153846153846,0.661538461538461,0.676923076923076,0.692307692307692,
0.707692307692307,0.723076923076922,0.738461538461538,0.753846153846153,
0.769230769230768,0.784615384615384,0.799999999999999,0.815384615384614,
0.83076923076923,0.846153846153845,0.86153846153846,0.876923076923076,0.892307692307691,
0.907692307692306,0.923076923076922,0.938461538461537,0.953846153846152,
0.969230769230768,0.984615384615383,1.),.UNSPECIFIED.)
CURVE()
GEOMETRIC_REPRESENTATION_ITEM()
RATIONAL_B_SPLINE_CURVE((1.,1.,1.,1.,1.,1.,1.,1.,1.,1.,1.,1.,1.,1.,1.,1.,
1.,1.,1.,1.,1.,1.,1.,1.,1.,1.,1.,1.,1.,1.,1.,1.,1.,1.,1.,1.,1.,1.,1.,1.,
1.,1.,1.,1.,1.,1.,1.,1.,1.,1.,1.,1.,1.,1.,1.,1.,1.,1.,1.,1.,1.,1.,1.,1.,
1.,1.,1.,1.,1.,1.))
REPRESENTATION_ITEM('')
);
#262=(
BOUNDED_CURVE()
B_SPLINE_CURVE(5,(#42504,#42505,#42506,#42507,#42508,#42509,#42510,#42511,
#42512,#42513,#42514,#42515,#42516,#42517,#42518,#42519,#42520,#42521,#42522,
#42523,#42524,#42525,#42526,#42527,#42528,#42529,#42530,#42531,#42532,#42533,
#42534,#42535,#42536,#42537,#42538,#42539,#42540,#42541,#42542,#42543,#42544,
#42545,#42546,#42547,#42548,#42549,#42550,#42551,#42552,#42553,#42554,#42555,
#42556,#42557,#42558,#42559,#42560,#42561,#42562,#42563,#42564,#42565,#42566,
#42567,#42568,#42569,#42570,#42571,#42572,#42573),.UNSPECIFIED.,.F.,.F.)
B_SPLINE_CURVE_WITH_KNOTS((6,1,1,1,1,1,1,1,1,1,1,1,1,1,1,1,1,1,1,1,1,1,
1,1,1,1,1,1,1,1,1,1,1,1,1,1,1,1,1,1,1,1,1,1,1,1,1,1,1,1,1,1,1,1,1,1,1,1,
1,1,1,1,1,1,1,6),(0.,0.0153846153846154,0.0307692307692308,0.0461538461538462,
0.0615384615384615,0.0769230769230769,0.0923076923076923,0.107692307692308,
0.123076923076923,0.138461538461538,0.153846153846154,0.169230769230769,
0.184615384615385,0.2,0.215384615384615,0.230769230769231,0.246153846153846,
0.261538461538462,0.276923076923077,0.292307692307692,0.307692307692308,
0.323076923076923,0.338461538461538,0.353846153846154,0.369230769230769,
0.384615384615385,0.4,0.415384615384615,0.430769230769231,0.446153846153846,
0.461538461538462,0.476923076923077,0.492307692307692,0.507692307692308,
0.523076923076923,0.538461538461538,0.553846153846154,0.569230769230769,
0.584615384615384,0.6,0.615384615384615,0.63076923076923,0.646153846153846,
0.661538461538461,0.676923076923076,0.692307692307692,0.707692307692307,
0.723076923076922,0.738461538461538,0.753846153846153,0.769230769230768,
0.784615384615384,0.799999999999999,0.815384615384614,0.83076923076923,
0.846153846153845,0.86153846153846,0.876923076923076,0.892307692307691,
0.907692307692306,0.923076923076922,0.938461538461537,0.953846153846152,
0.969230769230768,0.984615384615383,0.994228156739705),.UNSPECIFIED.)
CURVE()
GEOMETRIC_REPRESENTATION_ITEM()
RATIONAL_B_SPLINE_CURVE((1.,1.,1.,1.,1.,1.,1.,1.,1.,1.,1.,1.,1.,1.,1.,1.,
1.,1.,1.,1.,1.,1.,1.,1.,1.,1.,1.,1.,1.,1.,1.,1.,1.,1.,1.,1.,1.,1.,1.,1.,
1.,1.,1.,1.,1.,1.,1.,1.,1.,1.,1.,1.,1.,1.,1.,1.,1.,1.,1.,1.,1.,1.,1.,1.,
1.,1.,1.,1.,1.,1.))
REPRESENTATION_ITEM('')
);
#263=(
BOUNDED_CURVE()
B_SPLINE_CURVE(5,(#42577,#42578,#42579,#42580,#42581,#42582,#42583,#42584,
#42585,#42586,#42587,#42588,#42589,#42590,#42591,#42592,#42593,#42594,#42595,
#42596,#42597,#42598,#42599,#42600,#42601,#42602,#42603,#42604,#42605,#42606,
#42607,#42608,#42609,#42610,#42611,#42612,#42613,#42614,#42615,#42616,#42617,
#42618,#42619,#42620,#42621,#42622,#42623,#42624,#42625,#42626,#42627,#42628,
#42629,#42630,#42631,#42632,#42633,#42634,#42635,#42636,#42637,#42638,#42639,
#42640,#42641,#42642,#42643,#42644,#42645,#42646),.UNSPECIFIED.,.F.,.F.)
B_SPLINE_CURVE_WITH_KNOTS((6,1,1,1,1,1,1,1,1,1,1,1,1,1,1,1,1,1,1,1,1,1,
1,1,1,1,1,1,1,1,1,1,1,1,1,1,1,1,1,1,1,1,1,1,1,1,1,1,1,1,1,1,1,1,1,1,1,1,
1,1,1,1,1,1,1,6),(0.00577184337450072,0.0153846153846154,0.0307692307692308,
0.0461538461538462,0.0615384615384615,0.0769230769230769,0.0923076923076923,
0.107692307692308,0.123076923076923,0.138461538461538,0.153846153846154,
0.169230769230769,0.184615384615385,0.2,0.215384615384615,0.230769230769231,
0.246153846153846,0.261538461538462,0.276923076923077,0.292307692307692,
0.307692307692308,0.323076923076923,0.338461538461538,0.353846153846154,
0.369230769230769,0.384615384615385,0.4,0.415384615384615,0.430769230769231,
0.446153846153846,0.461538461538462,0.476923076923077,0.492307692307692,
0.507692307692308,0.523076923076923,0.538461538461538,0.553846153846154,
0.569230769230769,0.584615384615384,0.6,0.615384615384615,0.63076923076923,
0.646153846153846,0.661538461538461,0.676923076923076,0.692307692307692,
0.707692307692307,0.723076923076922,0.738461538461538,0.753846153846153,
0.769230769230768,0.784615384615384,0.799999999999999,0.815384615384614,
0.83076923076923,0.846153846153845,0.86153846153846,0.876923076923076,0.892307692307691,
0.907692307692306,0.923076923076922,0.938461538461537,0.953846153846152,
0.969230769230768,0.984615384615383,1.),.UNSPECIFIED.)
CURVE()
GEOMETRIC_REPRESENTATION_ITEM()
RATIONAL_B_SPLINE_CURVE((1.,1.,1.,1.,1.,1.,1.,1.,1.,1.,1.,1.,1.,1.,1.,1.,
1.,1.,1.,1.,1.,1.,1.,1.,1.,1.,1.,1.,1.,1.,1.,1.,1.,1.,1.,1.,1.,1.,1.,1.,
1.,1.,1.,1.,1.,1.,1.,1.,1.,1.,1.,1.,1.,1.,1.,1.,1.,1.,1.,1.,1.,1.,1.,1.,
1.,1.,1.,1.,1.,1.))
REPRESENTATION_ITEM('')
);
#264=(
BOUNDED_CURVE()
B_SPLINE_CURVE(5,(#42650,#42651,#42652,#42653,#42654,#42655,#42656,#42657,
#42658,#42659,#42660,#42661,#42662,#42663,#42664,#42665,#42666,#42667,#42668,
#42669,#42670,#42671,#42672,#42673,#42674,#42675,#42676,#42677,#42678,#42679,
#42680,#42681,#42682,#42683,#42684,#42685,#42686,#42687,#42688,#42689,#42690,
#42691,#42692,#42693,#42694,#42695,#42696,#42697,#42698,#42699,#42700,#42701,
#42702,#42703,#42704,#42705,#42706,#42707,#42708,#42709,#42710,#42711,#42712,
#42713,#42714,#42715,#42716,#42717,#42718,#42719),.UNSPECIFIED.,.F.,.F.)
B_SPLINE_CURVE_WITH_KNOTS((6,1,1,1,1,1,1,1,1,1,1,1,1,1,1,1,1,1,1,1,1,1,
1,1,1,1,1,1,1,1,1,1,1,1,1,1,1,1,1,1,1,1,1,1,1,1,1,1,1,1,1,1,1,1,1,1,1,1,
1,1,1,1,1,1,1,6),(0.,0.0153846153846154,0.0307692307692308,0.0461538461538462,
0.0615384615384615,0.0769230769230769,0.0923076923076923,0.107692307692308,
0.123076923076923,0.138461538461538,0.153846153846154,0.169230769230769,
0.184615384615385,0.2,0.215384615384615,0.230769230769231,0.246153846153846,
0.261538461538462,0.276923076923077,0.292307692307692,0.307692307692308,
0.323076923076923,0.338461538461538,0.353846153846154,0.369230769230769,
0.384615384615385,0.4,0.415384615384615,0.430769230769231,0.446153846153846,
0.461538461538462,0.476923076923077,0.492307692307692,0.507692307692308,
0.523076923076923,0.538461538461538,0.553846153846154,0.569230769230769,
0.584615384615384,0.6,0.615384615384615,0.63076923076923,0.646153846153846,
0.661538461538461,0.676923076923076,0.692307692307692,0.707692307692307,
0.723076923076922,0.738461538461538,0.753846153846153,0.769230769230768,
0.784615384615384,0.799999999999999,0.815384615384614,0.83076923076923,
0.846153846153845,0.86153846153846,0.876923076923076,0.892307692307691,
0.907692307692306,0.923076923076922,0.938461538461537,0.953846153846152,
0.969230769230768,0.984615384615383,0.994228156739706),.UNSPECIFIED.)
CURVE()
GEOMETRIC_REPRESENTATION_ITEM()
RATIONAL_B_SPLINE_CURVE((1.,1.,1.,1.,1.,1.,1.,1.,1.,1.,1.,1.,1.,1.,1.,1.,
1.,1.,1.,1.,1.,1.,1.,1.,1.,1.,1.,1.,1.,1.,1.,1.,1.,1.,1.,1.,1.,1.,1.,1.,
1.,1.,1.,1.,1.,1.,1.,1.,1.,1.,1.,1.,1.,1.,1.,1.,1.,1.,1.,1.,1.,1.,1.,1.,
1.,1.,1.,1.,1.,1.))
REPRESENTATION_ITEM('')
);
#265=(
BOUNDED_CURVE()
B_SPLINE_CURVE(5,(#42723,#42724,#42725,#42726,#42727,#42728,#42729,#42730,
#42731,#42732,#42733,#42734,#42735,#42736,#42737,#42738,#42739,#42740,#42741,
#42742,#42743,#42744,#42745,#42746,#42747,#42748,#42749,#42750,#42751,#42752,
#42753,#42754,#42755,#42756,#42757,#42758,#42759,#42760,#42761,#42762,#42763,
#42764,#42765,#42766,#42767,#42768,#42769,#42770,#42771,#42772,#42773,#42774,
#42775,#42776,#42777,#42778,#42779,#42780,#42781,#42782,#42783,#42784,#42785,
#42786,#42787,#42788,#42789,#42790,#42791,#42792),.UNSPECIFIED.,.F.,.F.)
B_SPLINE_CURVE_WITH_KNOTS((6,1,1,1,1,1,1,1,1,1,1,1,1,1,1,1,1,1,1,1,1,1,
1,1,1,1,1,1,1,1,1,1,1,1,1,1,1,1,1,1,1,1,1,1,1,1,1,1,1,1,1,1,1,1,1,1,1,1,
1,1,1,1,1,1,1,6),(0.00577184337450902,0.0153846153846154,0.0307692307692308,
0.0461538461538462,0.0615384615384615,0.0769230769230769,0.0923076923076923,
0.107692307692308,0.123076923076923,0.138461538461538,0.153846153846154,
0.169230769230769,0.184615384615385,0.2,0.215384615384615,0.230769230769231,
0.246153846153846,0.261538461538462,0.276923076923077,0.292307692307692,
0.307692307692308,0.323076923076923,0.338461538461538,0.353846153846154,
0.369230769230769,0.384615384615385,0.4,0.415384615384615,0.430769230769231,
0.446153846153846,0.461538461538462,0.476923076923077,0.492307692307692,
0.507692307692308,0.523076923076923,0.538461538461538,0.553846153846154,
0.569230769230769,0.584615384615384,0.6,0.615384615384615,0.63076923076923,
0.646153846153846,0.661538461538461,0.676923076923076,0.692307692307692,
0.707692307692307,0.723076923076922,0.738461538461538,0.753846153846153,
0.769230769230768,0.784615384615384,0.799999999999999,0.815384615384614,
0.83076923076923,0.846153846153845,0.86153846153846,0.876923076923076,0.892307692307691,
0.907692307692306,0.923076923076922,0.938461538461537,0.953846153846152,
0.969230769230768,0.984615384615383,1.),.UNSPECIFIED.)
CURVE()
GEOMETRIC_REPRESENTATION_ITEM()
RATIONAL_B_SPLINE_CURVE((1.,1.,1.,1.,1.,1.,1.,1.,1.,1.,1.,1.,1.,1.,1.,1.,
1.,1.,1.,1.,1.,1.,1.,1.,1.,1.,1.,1.,1.,1.,1.,1.,1.,1.,1.,1.,1.,1.,1.,1.,
1.,1.,1.,1.,1.,1.,1.,1.,1.,1.,1.,1.,1.,1.,1.,1.,1.,1.,1.,1.,1.,1.,1.,1.,
1.,1.,1.,1.,1.,1.))
REPRESENTATION_ITEM('')
);
#266=(
BOUNDED_CURVE()
B_SPLINE_CURVE(5,(#42796,#42797,#42798,#42799,#42800,#42801,#42802,#42803,
#42804,#42805,#42806,#42807,#42808,#42809,#42810,#42811,#42812,#42813,#42814,
#42815,#42816,#42817,#42818,#42819,#42820,#42821,#42822,#42823,#42824,#42825,
#42826,#42827,#42828,#42829,#42830,#42831,#42832,#42833,#42834,#42835,#42836,
#42837,#42838,#42839,#42840,#42841,#42842,#42843,#42844,#42845,#42846,#42847,
#42848,#42849,#42850,#42851,#42852,#42853,#42854,#42855,#42856,#42857,#42858,
#42859,#42860,#42861,#42862,#42863,#42864,#42865),.UNSPECIFIED.,.F.,.F.)
B_SPLINE_CURVE_WITH_KNOTS((6,1,1,1,1,1,1,1,1,1,1,1,1,1,1,1,1,1,1,1,1,1,
1,1,1,1,1,1,1,1,1,1,1,1,1,1,1,1,1,1,1,1,1,1,1,1,1,1,1,1,1,1,1,1,1,1,1,1,
1,1,1,1,1,1,1,6),(0.,0.0153846153846154,0.0307692307692308,0.0461538461538462,
0.0615384615384615,0.0769230769230769,0.0923076923076923,0.107692307692308,
0.123076923076923,0.138461538461538,0.153846153846154,0.169230769230769,
0.184615384615385,0.2,0.215384615384615,0.230769230769231,0.246153846153846,
0.261538461538462,0.276923076923077,0.292307692307692,0.307692307692308,
0.323076923076923,0.338461538461538,0.353846153846154,0.369230769230769,
0.384615384615385,0.4,0.415384615384615,0.430769230769231,0.446153846153846,
0.461538461538462,0.476923076923077,0.492307692307692,0.507692307692308,
0.523076923076923,0.538461538461538,0.553846153846154,0.569230769230769,
0.584615384615384,0.6,0.615384615384615,0.63076923076923,0.646153846153846,
0.661538461538461,0.676923076923076,0.692307692307692,0.707692307692307,
0.723076923076922,0.738461538461538,0.753846153846153,0.769230769230768,
0.784615384615384,0.799999999999999,0.815384615384614,0.83076923076923,
0.846153846153845,0.86153846153846,0.876923076923076,0.892307692307691,
0.907692307692306,0.923076923076922,0.938461538461537,0.953846153846152,
0.969230769230768,0.984615384615383,0.994228156739698),.UNSPECIFIED.)
CURVE()
GEOMETRIC_REPRESENTATION_ITEM()
RATIONAL_B_SPLINE_CURVE((1.,1.,1.,1.,1.,1.,1.,1.,1.,1.,1.,1.,1.,1.,1.,1.,
1.,1.,1.,1.,1.,1.,1.,1.,1.,1.,1.,1.,1.,1.,1.,1.,1.,1.,1.,1.,1.,1.,1.,1.,
1.,1.,1.,1.,1.,1.,1.,1.,1.,1.,1.,1.,1.,1.,1.,1.,1.,1.,1.,1.,1.,1.,1.,1.,
1.,1.,1.,1.,1.,1.))
REPRESENTATION_ITEM('')
);
#267=(
BOUNDED_CURVE()
B_SPLINE_CURVE(5,(#42869,#42870,#42871,#42872,#42873,#42874,#42875,#42876,
#42877,#42878,#42879,#42880,#42881,#42882,#42883,#42884,#42885,#42886,#42887,
#42888,#42889,#42890,#42891,#42892,#42893,#42894,#42895,#42896,#42897,#42898,
#42899,#42900,#42901,#42902,#42903,#42904,#42905,#42906,#42907,#42908,#42909,
#42910,#42911,#42912,#42913,#42914,#42915,#42916,#42917,#42918,#42919,#42920,
#42921,#42922,#42923,#42924,#42925,#42926,#42927,#42928,#42929,#42930,#42931,
#42932,#42933,#42934,#42935,#42936,#42937,#42938),.UNSPECIFIED.,.F.,.F.)
B_SPLINE_CURVE_WITH_KNOTS((6,1,1,1,1,1,1,1,1,1,1,1,1,1,1,1,1,1,1,1,1,1,
1,1,1,1,1,1,1,1,1,1,1,1,1,1,1,1,1,1,1,1,1,1,1,1,1,1,1,1,1,1,1,1,1,1,1,1,
1,1,1,1,1,1,1,6),(0.00577184337451611,0.0153846153846154,0.0307692307692308,
0.0461538461538462,0.0615384615384615,0.0769230769230769,0.0923076923076923,
0.107692307692308,0.123076923076923,0.138461538461538,0.153846153846154,
0.169230769230769,0.184615384615385,0.2,0.215384615384615,0.230769230769231,
0.246153846153846,0.261538461538462,0.276923076923077,0.292307692307692,
0.307692307692308,0.323076923076923,0.338461538461538,0.353846153846154,
0.369230769230769,0.384615384615385,0.4,0.415384615384615,0.430769230769231,
0.446153846153846,0.461538461538462,0.476923076923077,0.492307692307692,
0.507692307692308,0.523076923076923,0.538461538461538,0.553846153846154,
0.569230769230769,0.584615384615384,0.6,0.615384615384615,0.63076923076923,
0.646153846153846,0.661538461538461,0.676923076923076,0.692307692307692,
0.707692307692307,0.723076923076922,0.738461538461538,0.753846153846153,
0.769230769230768,0.784615384615384,0.799999999999999,0.815384615384614,
0.83076923076923,0.846153846153845,0.86153846153846,0.876923076923076,0.892307692307691,
0.907692307692306,0.923076923076922,0.938461538461537,0.953846153846152,
0.969230769230768,0.984615384615383,1.),.UNSPECIFIED.)
CURVE()
GEOMETRIC_REPRESENTATION_ITEM()
RATIONAL_B_SPLINE_CURVE((1.,1.,1.,1.,1.,1.,1.,1.,1.,1.,1.,1.,1.,1.,1.,1.,
1.,1.,1.,1.,1.,1.,1.,1.,1.,1.,1.,1.,1.,1.,1.,1.,1.,1.,1.,1.,1.,1.,1.,1.,
1.,1.,1.,1.,1.,1.,1.,1.,1.,1.,1.,1.,1.,1.,1.,1.,1.,1.,1.,1.,1.,1.,1.,1.,
1.,1.,1.,1.,1.,1.))
REPRESENTATION_ITEM('')
);
#268=(
BOUNDED_CURVE()
B_SPLINE_CURVE(5,(#42942,#42943,#42944,#42945,#42946,#42947,#42948,#42949,
#42950,#42951,#42952,#42953,#42954,#42955,#42956,#42957,#42958,#42959,#42960,
#42961,#42962,#42963,#42964,#42965,#42966,#42967,#42968,#42969,#42970,#42971,
#42972,#42973,#42974,#42975,#42976,#42977,#42978,#42979,#42980,#42981,#42982,
#42983,#42984,#42985,#42986,#42987,#42988,#42989,#42990,#42991,#42992,#42993,
#42994,#42995,#42996,#42997,#42998,#42999,#43000,#43001,#43002,#43003,#43004,
#43005,#43006,#43007,#43008,#43009,#43010,#43011),.UNSPECIFIED.,.F.,.F.)
B_SPLINE_CURVE_WITH_KNOTS((6,1,1,1,1,1,1,1,1,1,1,1,1,1,1,1,1,1,1,1,1,1,
1,1,1,1,1,1,1,1,1,1,1,1,1,1,1,1,1,1,1,1,1,1,1,1,1,1,1,1,1,1,1,1,1,1,1,1,
1,1,1,1,1,1,1,6),(0.,0.0153846153846154,0.0307692307692308,0.0461538461538462,
0.0615384615384615,0.0769230769230769,0.0923076923076923,0.107692307692308,
0.123076923076923,0.138461538461538,0.153846153846154,0.169230769230769,
0.184615384615385,0.2,0.215384615384615,0.230769230769231,0.246153846153846,
0.261538461538462,0.276923076923077,0.292307692307692,0.307692307692308,
0.323076923076923,0.338461538461538,0.353846153846154,0.369230769230769,
0.384615384615385,0.4,0.415384615384615,0.430769230769231,0.446153846153846,
0.461538461538462,0.476923076923077,0.492307692307692,0.507692307692308,
0.523076923076923,0.538461538461538,0.553846153846154,0.569230769230769,
0.584615384615384,0.6,0.615384615384615,0.63076923076923,0.646153846153846,
0.661538461538461,0.676923076923076,0.692307692307692,0.707692307692307,
0.723076923076922,0.738461538461538,0.753846153846153,0.769230769230768,
0.784615384615384,0.799999999999999,0.815384615384614,0.83076923076923,
0.846153846153845,0.86153846153846,0.876923076923076,0.892307692307691,
0.907692307692306,0.923076923076922,0.938461538461537,0.953846153846152,
0.969230769230768,0.984615384615383,0.994228156739704),.UNSPECIFIED.)
CURVE()
GEOMETRIC_REPRESENTATION_ITEM()
RATIONAL_B_SPLINE_CURVE((1.,1.,1.,1.,1.,1.,1.,1.,1.,1.,1.,1.,1.,1.,1.,1.,
1.,1.,1.,1.,1.,1.,1.,1.,1.,1.,1.,1.,1.,1.,1.,1.,1.,1.,1.,1.,1.,1.,1.,1.,
1.,1.,1.,1.,1.,1.,1.,1.,1.,1.,1.,1.,1.,1.,1.,1.,1.,1.,1.,1.,1.,1.,1.,1.,
1.,1.,1.,1.,1.,1.))
REPRESENTATION_ITEM('')
);
#269=(
BOUNDED_CURVE()
B_SPLINE_CURVE(5,(#43015,#43016,#43017,#43018,#43019,#43020,#43021,#43022,
#43023,#43024,#43025,#43026,#43027,#43028,#43029,#43030,#43031,#43032,#43033,
#43034,#43035,#43036,#43037,#43038,#43039,#43040,#43041,#43042,#43043,#43044,
#43045,#43046,#43047,#43048,#43049,#43050,#43051,#43052,#43053,#43054,#43055,
#43056,#43057,#43058,#43059,#43060,#43061,#43062,#43063,#43064,#43065,#43066,
#43067,#43068,#43069,#43070,#43071,#43072,#43073,#43074,#43075,#43076,#43077,
#43078,#43079,#43080,#43081,#43082,#43083,#43084),.UNSPECIFIED.,.F.,.F.)
B_SPLINE_CURVE_WITH_KNOTS((6,1,1,1,1,1,1,1,1,1,1,1,1,1,1,1,1,1,1,1,1,1,
1,1,1,1,1,1,1,1,1,1,1,1,1,1,1,1,1,1,1,1,1,1,1,1,1,1,1,1,1,1,1,1,1,1,1,1,
1,1,1,1,1,1,1,6),(0.00577184337449682,0.0153846153846154,0.0307692307692308,
0.0461538461538462,0.0615384615384615,0.0769230769230769,0.0923076923076923,
0.107692307692308,0.123076923076923,0.138461538461538,0.153846153846154,
0.169230769230769,0.184615384615385,0.2,0.215384615384615,0.230769230769231,
0.246153846153846,0.261538461538462,0.276923076923077,0.292307692307692,
0.307692307692308,0.323076923076923,0.338461538461538,0.353846153846154,
0.369230769230769,0.384615384615385,0.4,0.415384615384615,0.430769230769231,
0.446153846153846,0.461538461538462,0.476923076923077,0.492307692307692,
0.507692307692308,0.523076923076923,0.538461538461538,0.553846153846154,
0.569230769230769,0.584615384615384,0.6,0.615384615384615,0.63076923076923,
0.646153846153846,0.661538461538461,0.676923076923076,0.692307692307692,
0.707692307692307,0.723076923076922,0.738461538461538,0.753846153846153,
0.769230769230768,0.784615384615384,0.799999999999999,0.815384615384614,
0.83076923076923,0.846153846153845,0.86153846153846,0.876923076923076,0.892307692307691,
0.907692307692306,0.923076923076922,0.938461538461537,0.953846153846152,
0.969230769230768,0.984615384615383,1.),.UNSPECIFIED.)
CURVE()
GEOMETRIC_REPRESENTATION_ITEM()
RATIONAL_B_SPLINE_CURVE((1.,1.,1.,1.,1.,1.,1.,1.,1.,1.,1.,1.,1.,1.,1.,1.,
1.,1.,1.,1.,1.,1.,1.,1.,1.,1.,1.,1.,1.,1.,1.,1.,1.,1.,1.,1.,1.,1.,1.,1.,
1.,1.,1.,1.,1.,1.,1.,1.,1.,1.,1.,1.,1.,1.,1.,1.,1.,1.,1.,1.,1.,1.,1.,1.,
1.,1.,1.,1.,1.,1.))
REPRESENTATION_ITEM('')
);
#270=(
BOUNDED_CURVE()
B_SPLINE_CURVE(5,(#43088,#43089,#43090,#43091,#43092,#43093,#43094,#43095,
#43096,#43097,#43098,#43099,#43100,#43101,#43102,#43103,#43104,#43105,#43106,
#43107,#43108,#43109,#43110,#43111,#43112,#43113,#43114,#43115,#43116,#43117,
#43118,#43119,#43120,#43121,#43122,#43123,#43124,#43125,#43126,#43127,#43128,
#43129,#43130,#43131,#43132,#43133,#43134,#43135,#43136,#43137,#43138,#43139,
#43140,#43141,#43142,#43143,#43144,#43145,#43146,#43147,#43148,#43149,#43150,
#43151,#43152,#43153,#43154,#43155,#43156,#43157),.UNSPECIFIED.,.F.,.F.)
B_SPLINE_CURVE_WITH_KNOTS((6,1,1,1,1,1,1,1,1,1,1,1,1,1,1,1,1,1,1,1,1,1,
1,1,1,1,1,1,1,1,1,1,1,1,1,1,1,1,1,1,1,1,1,1,1,1,1,1,1,1,1,1,1,1,1,1,1,1,
1,1,1,1,1,1,1,6),(0.,0.0153846153846154,0.0307692307692308,0.0461538461538462,
0.0615384615384615,0.0769230769230769,0.0923076923076923,0.107692307692308,
0.123076923076923,0.138461538461538,0.153846153846154,0.169230769230769,
0.184615384615385,0.2,0.215384615384615,0.230769230769231,0.246153846153846,
0.261538461538462,0.276923076923077,0.292307692307692,0.307692307692308,
0.323076923076923,0.338461538461538,0.353846153846154,0.369230769230769,
0.384615384615385,0.4,0.415384615384615,0.430769230769231,0.446153846153846,
0.461538461538462,0.476923076923077,0.492307692307692,0.507692307692308,
0.523076923076923,0.538461538461538,0.553846153846154,0.569230769230769,
0.584615384615384,0.6,0.615384615384615,0.63076923076923,0.646153846153846,
0.661538461538461,0.676923076923076,0.692307692307692,0.707692307692307,
0.723076923076922,0.738461538461538,0.753846153846153,0.769230769230768,
0.784615384615384,0.799999999999999,0.815384615384614,0.83076923076923,
0.846153846153845,0.86153846153846,0.876923076923076,0.892307692307691,
0.907692307692306,0.923076923076922,0.938461538461537,0.953846153846152,
0.969230769230768,0.984615384615383,0.994228156739711),.UNSPECIFIED.)
CURVE()
GEOMETRIC_REPRESENTATION_ITEM()
RATIONAL_B_SPLINE_CURVE((1.,1.,1.,1.,1.,1.,1.,1.,1.,1.,1.,1.,1.,1.,1.,1.,
1.,1.,1.,1.,1.,1.,1.,1.,1.,1.,1.,1.,1.,1.,1.,1.,1.,1.,1.,1.,1.,1.,1.,1.,
1.,1.,1.,1.,1.,1.,1.,1.,1.,1.,1.,1.,1.,1.,1.,1.,1.,1.,1.,1.,1.,1.,1.,1.,
1.,1.,1.,1.,1.,1.))
REPRESENTATION_ITEM('')
);
#271=(
BOUNDED_CURVE()
B_SPLINE_CURVE(5,(#43161,#43162,#43163,#43164,#43165,#43166,#43167,#43168,
#43169,#43170,#43171,#43172,#43173,#43174,#43175,#43176,#43177,#43178,#43179,
#43180,#43181,#43182,#43183,#43184,#43185,#43186,#43187,#43188,#43189,#43190,
#43191,#43192,#43193,#43194,#43195,#43196,#43197,#43198,#43199,#43200,#43201,
#43202,#43203,#43204,#43205,#43206,#43207,#43208,#43209,#43210,#43211,#43212,
#43213,#43214,#43215,#43216,#43217,#43218,#43219,#43220,#43221,#43222,#43223,
#43224,#43225,#43226,#43227,#43228,#43229,#43230),.UNSPECIFIED.,.F.,.F.)
B_SPLINE_CURVE_WITH_KNOTS((6,1,1,1,1,1,1,1,1,1,1,1,1,1,1,1,1,1,1,1,1,1,
1,1,1,1,1,1,1,1,1,1,1,1,1,1,1,1,1,1,1,1,1,1,1,1,1,1,1,1,1,1,1,1,1,1,1,1,
1,1,1,1,1,1,1,6),(0.00577184337449159,0.0153846153846154,0.0307692307692308,
0.0461538461538462,0.0615384615384615,0.0769230769230769,0.0923076923076923,
0.107692307692308,0.123076923076923,0.138461538461538,0.153846153846154,
0.169230769230769,0.184615384615385,0.2,0.215384615384615,0.230769230769231,
0.246153846153846,0.261538461538462,0.276923076923077,0.292307692307692,
0.307692307692308,0.323076923076923,0.338461538461538,0.353846153846154,
0.369230769230769,0.384615384615385,0.4,0.415384615384615,0.430769230769231,
0.446153846153846,0.461538461538462,0.476923076923077,0.492307692307692,
0.507692307692308,0.523076923076923,0.538461538461538,0.553846153846154,
0.569230769230769,0.584615384615384,0.6,0.615384615384615,0.63076923076923,
0.646153846153846,0.661538461538461,0.676923076923076,0.692307692307692,
0.707692307692307,0.723076923076922,0.738461538461538,0.753846153846153,
0.769230769230768,0.784615384615384,0.799999999999999,0.815384615384614,
0.83076923076923,0.846153846153845,0.86153846153846,0.876923076923076,0.892307692307691,
0.907692307692306,0.923076923076922,0.938461538461537,0.953846153846152,
0.969230769230768,0.984615384615383,1.),.UNSPECIFIED.)
CURVE()
GEOMETRIC_REPRESENTATION_ITEM()
RATIONAL_B_SPLINE_CURVE((1.,1.,1.,1.,1.,1.,1.,1.,1.,1.,1.,1.,1.,1.,1.,1.,
1.,1.,1.,1.,1.,1.,1.,1.,1.,1.,1.,1.,1.,1.,1.,1.,1.,1.,1.,1.,1.,1.,1.,1.,
1.,1.,1.,1.,1.,1.,1.,1.,1.,1.,1.,1.,1.,1.,1.,1.,1.,1.,1.,1.,1.,1.,1.,1.,
1.,1.,1.,1.,1.,1.))
REPRESENTATION_ITEM('')
);
#272=(
BOUNDED_CURVE()
B_SPLINE_CURVE(5,(#43234,#43235,#43236,#43237,#43238,#43239,#43240,#43241,
#43242,#43243,#43244,#43245,#43246,#43247,#43248,#43249,#43250,#43251,#43252,
#43253,#43254,#43255,#43256,#43257,#43258,#43259,#43260,#43261,#43262,#43263,
#43264,#43265,#43266,#43267,#43268,#43269,#43270,#43271,#43272,#43273,#43274,
#43275,#43276,#43277,#43278,#43279,#43280,#43281,#43282,#43283,#43284,#43285,
#43286,#43287,#43288,#43289,#43290,#43291,#43292,#43293,#43294,#43295,#43296,
#43297,#43298,#43299,#43300,#43301,#43302,#43303),.UNSPECIFIED.,.F.,.F.)
B_SPLINE_CURVE_WITH_KNOTS((6,1,1,1,1,1,1,1,1,1,1,1,1,1,1,1,1,1,1,1,1,1,
1,1,1,1,1,1,1,1,1,1,1,1,1,1,1,1,1,1,1,1,1,1,1,1,1,1,1,1,1,1,1,1,1,1,1,1,
1,1,1,1,1,1,1,6),(0.,0.0153846153846154,0.0307692307692308,0.0461538461538462,
0.0615384615384615,0.0769230769230769,0.0923076923076923,0.107692307692308,
0.123076923076923,0.138461538461538,0.153846153846154,0.169230769230769,
0.184615384615385,0.2,0.215384615384615,0.230769230769231,0.246153846153846,
0.261538461538462,0.276923076923077,0.292307692307692,0.307692307692308,
0.323076923076923,0.338461538461538,0.353846153846154,0.369230769230769,
0.384615384615385,0.4,0.415384615384615,0.430769230769231,0.446153846153846,
0.461538461538462,0.476923076923077,0.492307692307692,0.507692307692308,
0.523076923076923,0.538461538461538,0.553846153846154,0.569230769230769,
0.584615384615384,0.6,0.615384615384615,0.63076923076923,0.646153846153846,
0.661538461538461,0.676923076923076,0.692307692307692,0.707692307692307,
0.723076923076922,0.738461538461538,0.753846153846153,0.769230769230768,
0.784615384615384,0.799999999999999,0.815384615384614,0.83076923076923,
0.846153846153845,0.86153846153846,0.876923076923076,0.892307692307691,
0.907692307692306,0.923076923076922,0.938461538461537,0.953846153846152,
0.969230769230768,0.984615384615383,0.994228156739723),.UNSPECIFIED.)
CURVE()
GEOMETRIC_REPRESENTATION_ITEM()
RATIONAL_B_SPLINE_CURVE((1.,1.,1.,1.,1.,1.,1.,1.,1.,1.,1.,1.,1.,1.,1.,1.,
1.,1.,1.,1.,1.,1.,1.,1.,1.,1.,1.,1.,1.,1.,1.,1.,1.,1.,1.,1.,1.,1.,1.,1.,
1.,1.,1.,1.,1.,1.,1.,1.,1.,1.,1.,1.,1.,1.,1.,1.,1.,1.,1.,1.,1.,1.,1.,1.,
1.,1.,1.,1.,1.,1.))
REPRESENTATION_ITEM('')
);
#273=(
BOUNDED_CURVE()
B_SPLINE_CURVE(5,(#43307,#43308,#43309,#43310,#43311,#43312,#43313,#43314,
#43315,#43316,#43317,#43318,#43319,#43320,#43321,#43322,#43323,#43324,#43325,
#43326,#43327,#43328,#43329,#43330,#43331,#43332,#43333,#43334,#43335,#43336,
#43337,#43338,#43339,#43340,#43341,#43342,#43343,#43344,#43345,#43346,#43347,
#43348,#43349,#43350,#43351,#43352,#43353,#43354,#43355,#43356,#43357,#43358,
#43359,#43360,#43361,#43362,#43363,#43364,#43365,#43366,#43367,#43368,#43369,
#43370,#43371,#43372,#43373,#43374,#43375,#43376),.UNSPECIFIED.,.F.,.F.)
B_SPLINE_CURVE_WITH_KNOTS((6,1,1,1,1,1,1,1,1,1,1,1,1,1,1,1,1,1,1,1,1,1,
1,1,1,1,1,1,1,1,1,1,1,1,1,1,1,1,1,1,1,1,1,1,1,1,1,1,1,1,1,1,1,1,1,1,1,1,
1,1,1,1,1,1,1,6),(0.00577184337450718,0.0153846153846154,0.0307692307692308,
0.0461538461538462,0.0615384615384615,0.0769230769230769,0.0923076923076923,
0.107692307692308,0.123076923076923,0.138461538461538,0.153846153846154,
0.169230769230769,0.184615384615385,0.2,0.215384615384615,0.230769230769231,
0.246153846153846,0.261538461538462,0.276923076923077,0.292307692307692,
0.307692307692308,0.323076923076923,0.338461538461538,0.353846153846154,
0.369230769230769,0.384615384615385,0.4,0.415384615384615,0.430769230769231,
0.446153846153846,0.461538461538462,0.476923076923077,0.492307692307692,
0.507692307692308,0.523076923076923,0.538461538461538,0.553846153846154,
0.569230769230769,0.584615384615384,0.6,0.615384615384615,0.63076923076923,
0.646153846153846,0.661538461538461,0.676923076923076,0.692307692307692,
0.707692307692307,0.723076923076922,0.738461538461538,0.753846153846153,
0.769230769230768,0.784615384615384,0.799999999999999,0.815384615384614,
0.83076923076923,0.846153846153845,0.86153846153846,0.876923076923076,0.892307692307691,
0.907692307692306,0.923076923076922,0.938461538461537,0.953846153846152,
0.969230769230768,0.984615384615383,1.),.UNSPECIFIED.)
CURVE()
GEOMETRIC_REPRESENTATION_ITEM()
RATIONAL_B_SPLINE_CURVE((1.,1.,1.,1.,1.,1.,1.,1.,1.,1.,1.,1.,1.,1.,1.,1.,
1.,1.,1.,1.,1.,1.,1.,1.,1.,1.,1.,1.,1.,1.,1.,1.,1.,1.,1.,1.,1.,1.,1.,1.,
1.,1.,1.,1.,1.,1.,1.,1.,1.,1.,1.,1.,1.,1.,1.,1.,1.,1.,1.,1.,1.,1.,1.,1.,
1.,1.,1.,1.,1.,1.))
REPRESENTATION_ITEM('')
);
#274=(
BOUNDED_CURVE()
B_SPLINE_CURVE(5,(#43380,#43381,#43382,#43383,#43384,#43385,#43386,#43387,
#43388,#43389,#43390,#43391,#43392,#43393,#43394,#43395,#43396,#43397,#43398,
#43399,#43400,#43401,#43402,#43403,#43404,#43405,#43406,#43407,#43408,#43409,
#43410,#43411,#43412,#43413,#43414,#43415,#43416,#43417,#43418,#43419,#43420,
#43421,#43422,#43423,#43424,#43425,#43426,#43427,#43428,#43429,#43430,#43431,
#43432,#43433,#43434,#43435,#43436,#43437,#43438,#43439,#43440,#43441,#43442,
#43443,#43444,#43445,#43446,#43447,#43448,#43449),.UNSPECIFIED.,.F.,.F.)
B_SPLINE_CURVE_WITH_KNOTS((6,1,1,1,1,1,1,1,1,1,1,1,1,1,1,1,1,1,1,1,1,1,
1,1,1,1,1,1,1,1,1,1,1,1,1,1,1,1,1,1,1,1,1,1,1,1,1,1,1,1,1,1,1,1,1,1,1,1,
1,1,1,1,1,1,1,6),(0.,0.0153846153846154,0.0307692307692308,0.0461538461538462,
0.0615384615384615,0.0769230769230769,0.0923076923076923,0.107692307692308,
0.123076923076923,0.138461538461538,0.153846153846154,0.169230769230769,
0.184615384615385,0.2,0.215384615384615,0.230769230769231,0.246153846153846,
0.261538461538462,0.276923076923077,0.292307692307692,0.307692307692308,
0.323076923076923,0.338461538461538,0.353846153846154,0.369230769230769,
0.384615384615385,0.4,0.415384615384615,0.430769230769231,0.446153846153846,
0.461538461538462,0.476923076923077,0.492307692307692,0.507692307692308,
0.523076923076923,0.538461538461538,0.553846153846154,0.569230769230769,
0.584615384615384,0.6,0.615384615384615,0.63076923076923,0.646153846153846,
0.661538461538461,0.676923076923076,0.692307692307692,0.707692307692307,
0.723076923076922,0.738461538461538,0.753846153846153,0.769230769230768,
0.784615384615384,0.799999999999999,0.815384615384614,0.83076923076923,
0.846153846153845,0.86153846153846,0.876923076923076,0.892307692307691,
0.907692307692306,0.923076923076922,0.938461538461537,0.953846153846152,
0.969230769230768,0.984615384615383,0.994228156739716),.UNSPECIFIED.)
CURVE()
GEOMETRIC_REPRESENTATION_ITEM()
RATIONAL_B_SPLINE_CURVE((1.,1.,1.,1.,1.,1.,1.,1.,1.,1.,1.,1.,1.,1.,1.,1.,
1.,1.,1.,1.,1.,1.,1.,1.,1.,1.,1.,1.,1.,1.,1.,1.,1.,1.,1.,1.,1.,1.,1.,1.,
1.,1.,1.,1.,1.,1.,1.,1.,1.,1.,1.,1.,1.,1.,1.,1.,1.,1.,1.,1.,1.,1.,1.,1.,
1.,1.,1.,1.,1.,1.))
REPRESENTATION_ITEM('')
);
#275=(
BOUNDED_CURVE()
B_SPLINE_CURVE(5,(#43453,#43454,#43455,#43456,#43457,#43458,#43459,#43460,
#43461,#43462,#43463,#43464,#43465,#43466,#43467,#43468,#43469,#43470,#43471,
#43472,#43473,#43474,#43475,#43476,#43477,#43478,#43479,#43480,#43481,#43482,
#43483,#43484,#43485,#43486,#43487,#43488,#43489,#43490,#43491,#43492,#43493,
#43494,#43495,#43496,#43497,#43498,#43499,#43500,#43501,#43502,#43503,#43504,
#43505,#43506,#43507,#43508,#43509,#43510,#43511,#43512,#43513,#43514,#43515,
#43516,#43517,#43518,#43519,#43520,#43521,#43522),.UNSPECIFIED.,.F.,.F.)
B_SPLINE_CURVE_WITH_KNOTS((6,1,1,1,1,1,1,1,1,1,1,1,1,1,1,1,1,1,1,1,1,1,
1,1,1,1,1,1,1,1,1,1,1,1,1,1,1,1,1,1,1,1,1,1,1,1,1,1,1,1,1,1,1,1,1,1,1,1,
1,1,1,1,1,1,1,6),(0.00577184337450174,0.0153846153846154,0.0307692307692308,
0.0461538461538462,0.0615384615384615,0.0769230769230769,0.0923076923076923,
0.107692307692308,0.123076923076923,0.138461538461538,0.153846153846154,
0.169230769230769,0.184615384615385,0.2,0.215384615384615,0.230769230769231,
0.246153846153846,0.261538461538462,0.276923076923077,0.292307692307692,
0.307692307692308,0.323076923076923,0.338461538461538,0.353846153846154,
0.369230769230769,0.384615384615385,0.4,0.415384615384615,0.430769230769231,
0.446153846153846,0.461538461538462,0.476923076923077,0.492307692307692,
0.507692307692308,0.523076923076923,0.538461538461538,0.553846153846154,
0.569230769230769,0.584615384615384,0.6,0.615384615384615,0.63076923076923,
0.646153846153846,0.661538461538461,0.676923076923076,0.692307692307692,
0.707692307692307,0.723076923076922,0.738461538461538,0.753846153846153,
0.769230769230768,0.784615384615384,0.799999999999999,0.815384615384614,
0.83076923076923,0.846153846153845,0.86153846153846,0.876923076923076,0.892307692307691,
0.907692307692306,0.923076923076922,0.938461538461537,0.953846153846152,
0.969230769230768,0.984615384615383,1.),.UNSPECIFIED.)
CURVE()
GEOMETRIC_REPRESENTATION_ITEM()
RATIONAL_B_SPLINE_CURVE((1.,1.,1.,1.,1.,1.,1.,1.,1.,1.,1.,1.,1.,1.,1.,1.,
1.,1.,1.,1.,1.,1.,1.,1.,1.,1.,1.,1.,1.,1.,1.,1.,1.,1.,1.,1.,1.,1.,1.,1.,
1.,1.,1.,1.,1.,1.,1.,1.,1.,1.,1.,1.,1.,1.,1.,1.,1.,1.,1.,1.,1.,1.,1.,1.,
1.,1.,1.,1.,1.,1.))
REPRESENTATION_ITEM('')
);
#276=(
BOUNDED_CURVE()
B_SPLINE_CURVE(5,(#43526,#43527,#43528,#43529,#43530,#43531,#43532,#43533,
#43534,#43535,#43536,#43537,#43538,#43539,#43540,#43541,#43542,#43543,#43544,
#43545,#43546,#43547,#43548,#43549,#43550,#43551,#43552,#43553,#43554,#43555,
#43556,#43557,#43558,#43559,#43560,#43561,#43562,#43563,#43564,#43565,#43566,
#43567,#43568,#43569,#43570,#43571,#43572,#43573,#43574,#43575,#43576,#43577,
#43578,#43579,#43580,#43581,#43582,#43583,#43584,#43585,#43586,#43587,#43588,
#43589,#43590,#43591,#43592,#43593,#43594,#43595),.UNSPECIFIED.,.F.,.F.)
B_SPLINE_CURVE_WITH_KNOTS((6,1,1,1,1,1,1,1,1,1,1,1,1,1,1,1,1,1,1,1,1,1,
1,1,1,1,1,1,1,1,1,1,1,1,1,1,1,1,1,1,1,1,1,1,1,1,1,1,1,1,1,1,1,1,1,1,1,1,
1,1,1,1,1,1,1,6),(0.,0.0153846153846154,0.0307692307692308,0.0461538461538462,
0.0615384615384615,0.0769230769230769,0.0923076923076923,0.107692307692308,
0.123076923076923,0.138461538461538,0.153846153846154,0.169230769230769,
0.184615384615385,0.2,0.215384615384615,0.230769230769231,0.246153846153846,
0.261538461538462,0.276923076923077,0.292307692307692,0.307692307692308,
0.323076923076923,0.338461538461538,0.353846153846154,0.369230769230769,
0.384615384615385,0.4,0.415384615384615,0.430769230769231,0.446153846153846,
0.461538461538462,0.476923076923077,0.492307692307692,0.507692307692308,
0.523076923076923,0.538461538461538,0.553846153846154,0.569230769230769,
0.584615384615384,0.6,0.615384615384615,0.63076923076923,0.646153846153846,
0.661538461538461,0.676923076923076,0.692307692307692,0.707692307692307,
0.723076923076922,0.738461538461538,0.753846153846153,0.769230769230768,
0.784615384615384,0.799999999999999,0.815384615384614,0.83076923076923,
0.846153846153845,0.86153846153846,0.876923076923076,0.892307692307691,
0.907692307692306,0.923076923076922,0.938461538461537,0.953846153846152,
0.969230769230768,0.984615384615383,0.994228156739722),.UNSPECIFIED.)
CURVE()
GEOMETRIC_REPRESENTATION_ITEM()
RATIONAL_B_SPLINE_CURVE((1.,1.,1.,1.,1.,1.,1.,1.,1.,1.,1.,1.,1.,1.,1.,1.,
1.,1.,1.,1.,1.,1.,1.,1.,1.,1.,1.,1.,1.,1.,1.,1.,1.,1.,1.,1.,1.,1.,1.,1.,
1.,1.,1.,1.,1.,1.,1.,1.,1.,1.,1.,1.,1.,1.,1.,1.,1.,1.,1.,1.,1.,1.,1.,1.,
1.,1.,1.,1.,1.,1.))
REPRESENTATION_ITEM('')
);
#277=(
BOUNDED_CURVE()
B_SPLINE_CURVE(5,(#43599,#43600,#43601,#43602,#43603,#43604,#43605,#43606,
#43607,#43608,#43609,#43610,#43611,#43612,#43613,#43614,#43615,#43616,#43617,
#43618,#43619,#43620,#43621,#43622,#43623,#43624,#43625,#43626,#43627,#43628,
#43629,#43630,#43631,#43632,#43633,#43634,#43635,#43636,#43637,#43638,#43639,
#43640,#43641,#43642,#43643,#43644,#43645,#43646,#43647,#43648,#43649,#43650,
#43651,#43652,#43653,#43654,#43655,#43656,#43657,#43658,#43659,#43660,#43661,
#43662,#43663,#43664,#43665,#43666,#43667,#43668),.UNSPECIFIED.,.F.,.F.)
B_SPLINE_CURVE_WITH_KNOTS((6,1,1,1,1,1,1,1,1,1,1,1,1,1,1,1,1,1,1,1,1,1,
1,1,1,1,1,1,1,1,1,1,1,1,1,1,1,1,1,1,1,1,1,1,1,1,1,1,1,1,1,1,1,1,1,1,1,1,
1,1,1,1,1,1,1,6),(0.00577184337450943,0.0153846153846154,0.0307692307692308,
0.0461538461538462,0.0615384615384615,0.0769230769230769,0.0923076923076923,
0.107692307692308,0.123076923076923,0.138461538461538,0.153846153846154,
0.169230769230769,0.184615384615385,0.2,0.215384615384615,0.230769230769231,
0.246153846153846,0.261538461538462,0.276923076923077,0.292307692307692,
0.307692307692308,0.323076923076923,0.338461538461538,0.353846153846154,
0.369230769230769,0.384615384615385,0.4,0.415384615384615,0.430769230769231,
0.446153846153846,0.461538461538462,0.476923076923077,0.492307692307692,
0.507692307692308,0.523076923076923,0.538461538461538,0.553846153846154,
0.569230769230769,0.584615384615384,0.6,0.615384615384615,0.63076923076923,
0.646153846153846,0.661538461538461,0.676923076923076,0.692307692307692,
0.707692307692307,0.723076923076922,0.738461538461538,0.753846153846153,
0.769230769230768,0.784615384615384,0.799999999999999,0.815384615384614,
0.83076923076923,0.846153846153845,0.86153846153846,0.876923076923076,0.892307692307691,
0.907692307692306,0.923076923076922,0.938461538461537,0.953846153846152,
0.969230769230768,0.984615384615383,1.),.UNSPECIFIED.)
CURVE()
GEOMETRIC_REPRESENTATION_ITEM()
RATIONAL_B_SPLINE_CURVE((1.,1.,1.,1.,1.,1.,1.,1.,1.,1.,1.,1.,1.,1.,1.,1.,
1.,1.,1.,1.,1.,1.,1.,1.,1.,1.,1.,1.,1.,1.,1.,1.,1.,1.,1.,1.,1.,1.,1.,1.,
1.,1.,1.,1.,1.,1.,1.,1.,1.,1.,1.,1.,1.,1.,1.,1.,1.,1.,1.,1.,1.,1.,1.,1.,
1.,1.,1.,1.,1.,1.))
REPRESENTATION_ITEM('')
);
#278=(
BOUNDED_CURVE()
B_SPLINE_CURVE(5,(#43672,#43673,#43674,#43675,#43676,#43677,#43678,#43679,
#43680,#43681,#43682,#43683,#43684,#43685,#43686,#43687,#43688,#43689,#43690,
#43691,#43692,#43693,#43694,#43695,#43696,#43697,#43698,#43699,#43700,#43701,
#43702,#43703,#43704,#43705,#43706,#43707,#43708,#43709,#43710,#43711,#43712,
#43713,#43714,#43715,#43716,#43717,#43718,#43719,#43720,#43721,#43722,#43723,
#43724,#43725,#43726,#43727,#43728,#43729,#43730,#43731,#43732,#43733,#43734,
#43735,#43736,#43737,#43738,#43739,#43740,#43741),.UNSPECIFIED.,.F.,.F.)
B_SPLINE_CURVE_WITH_KNOTS((6,1,1,1,1,1,1,1,1,1,1,1,1,1,1,1,1,1,1,1,1,1,
1,1,1,1,1,1,1,1,1,1,1,1,1,1,1,1,1,1,1,1,1,1,1,1,1,1,1,1,1,1,1,1,1,1,1,1,
1,1,1,1,1,1,1,6),(0.,0.0153846153846154,0.0307692307692308,0.0461538461538462,
0.0615384615384615,0.0769230769230769,0.0923076923076923,0.107692307692308,
0.123076923076923,0.138461538461538,0.153846153846154,0.169230769230769,
0.184615384615385,0.2,0.215384615384615,0.230769230769231,0.246153846153846,
0.261538461538462,0.276923076923077,0.292307692307692,0.307692307692308,
0.323076923076923,0.338461538461538,0.353846153846154,0.369230769230769,
0.384615384615385,0.4,0.415384615384615,0.430769230769231,0.446153846153846,
0.461538461538462,0.476923076923077,0.492307692307692,0.507692307692308,
0.523076923076923,0.538461538461538,0.553846153846154,0.569230769230769,
0.584615384615384,0.6,0.615384615384615,0.63076923076923,0.646153846153846,
0.661538461538461,0.676923076923076,0.692307692307692,0.707692307692307,
0.723076923076922,0.738461538461538,0.753846153846153,0.769230769230768,
0.784615384615384,0.799999999999999,0.815384615384614,0.83076923076923,
0.846153846153845,0.86153846153846,0.876923076923076,0.892307692307691,
0.907692307692306,0.923076923076922,0.938461538461537,0.953846153846152,
0.969230769230768,0.984615384615383,0.994228156739699),.UNSPECIFIED.)
CURVE()
GEOMETRIC_REPRESENTATION_ITEM()
RATIONAL_B_SPLINE_CURVE((1.,1.,1.,1.,1.,1.,1.,1.,1.,1.,1.,1.,1.,1.,1.,1.,
1.,1.,1.,1.,1.,1.,1.,1.,1.,1.,1.,1.,1.,1.,1.,1.,1.,1.,1.,1.,1.,1.,1.,1.,
1.,1.,1.,1.,1.,1.,1.,1.,1.,1.,1.,1.,1.,1.,1.,1.,1.,1.,1.,1.,1.,1.,1.,1.,
1.,1.,1.,1.,1.,1.))
REPRESENTATION_ITEM('')
);
#279=(
BOUNDED_CURVE()
B_SPLINE_CURVE(5,(#43745,#43746,#43747,#43748,#43749,#43750,#43751,#43752,
#43753,#43754,#43755,#43756,#43757,#43758,#43759,#43760,#43761,#43762,#43763,
#43764,#43765,#43766,#43767,#43768,#43769,#43770,#43771,#43772,#43773,#43774,
#43775,#43776,#43777,#43778,#43779,#43780,#43781,#43782,#43783,#43784,#43785,
#43786,#43787,#43788,#43789,#43790,#43791,#43792,#43793,#43794,#43795,#43796,
#43797,#43798,#43799,#43800,#43801,#43802,#43803,#43804,#43805,#43806,#43807,
#43808,#43809,#43810,#43811,#43812,#43813,#43814),.UNSPECIFIED.,.F.,.F.)
B_SPLINE_CURVE_WITH_KNOTS((6,1,1,1,1,1,1,1,1,1,1,1,1,1,1,1,1,1,1,1,1,1,
1,1,1,1,1,1,1,1,1,1,1,1,1,1,1,1,1,1,1,1,1,1,1,1,1,1,1,1,1,1,1,1,1,1,1,1,
1,1,1,1,1,1,1,6),(0.00577184337450665,0.0153846153846154,0.0307692307692308,
0.0461538461538462,0.0615384615384615,0.0769230769230769,0.0923076923076923,
0.107692307692308,0.123076923076923,0.138461538461538,0.153846153846154,
0.169230769230769,0.184615384615385,0.2,0.215384615384615,0.230769230769231,
0.246153846153846,0.261538461538462,0.276923076923077,0.292307692307692,
0.307692307692308,0.323076923076923,0.338461538461538,0.353846153846154,
0.369230769230769,0.384615384615385,0.4,0.415384615384615,0.430769230769231,
0.446153846153846,0.461538461538462,0.476923076923077,0.492307692307692,
0.507692307692308,0.523076923076923,0.538461538461538,0.553846153846154,
0.569230769230769,0.584615384615384,0.6,0.615384615384615,0.63076923076923,
0.646153846153846,0.661538461538461,0.676923076923076,0.692307692307692,
0.707692307692307,0.723076923076922,0.738461538461538,0.753846153846153,
0.769230769230768,0.784615384615384,0.799999999999999,0.815384615384614,
0.83076923076923,0.846153846153845,0.86153846153846,0.876923076923076,0.892307692307691,
0.907692307692306,0.923076923076922,0.938461538461537,0.953846153846152,
0.969230769230768,0.984615384615383,1.),.UNSPECIFIED.)
CURVE()
GEOMETRIC_REPRESENTATION_ITEM()
RATIONAL_B_SPLINE_CURVE((1.,1.,1.,1.,1.,1.,1.,1.,1.,1.,1.,1.,1.,1.,1.,1.,
1.,1.,1.,1.,1.,1.,1.,1.,1.,1.,1.,1.,1.,1.,1.,1.,1.,1.,1.,1.,1.,1.,1.,1.,
1.,1.,1.,1.,1.,1.,1.,1.,1.,1.,1.,1.,1.,1.,1.,1.,1.,1.,1.,1.,1.,1.,1.,1.,
1.,1.,1.,1.,1.,1.))
REPRESENTATION_ITEM('')
);
#280=(
BOUNDED_CURVE()
B_SPLINE_CURVE(5,(#43818,#43819,#43820,#43821,#43822,#43823,#43824,#43825,
#43826,#43827,#43828,#43829,#43830,#43831,#43832,#43833,#43834,#43835,#43836,
#43837,#43838,#43839,#43840,#43841,#43842,#43843,#43844,#43845,#43846,#43847,
#43848,#43849,#43850,#43851,#43852,#43853,#43854,#43855,#43856,#43857,#43858,
#43859,#43860,#43861,#43862,#43863,#43864,#43865,#43866,#43867,#43868,#43869,
#43870,#43871,#43872,#43873,#43874,#43875,#43876,#43877,#43878,#43879,#43880,
#43881,#43882,#43883,#43884,#43885,#43886,#43887),.UNSPECIFIED.,.F.,.F.)
B_SPLINE_CURVE_WITH_KNOTS((6,1,1,1,1,1,1,1,1,1,1,1,1,1,1,1,1,1,1,1,1,1,
1,1,1,1,1,1,1,1,1,1,1,1,1,1,1,1,1,1,1,1,1,1,1,1,1,1,1,1,1,1,1,1,1,1,1,1,
1,1,1,1,1,1,1,6),(0.,0.0153846153846154,0.0307692307692308,0.0461538461538462,
0.0615384615384615,0.0769230769230769,0.0923076923076923,0.107692307692308,
0.123076923076923,0.138461538461538,0.153846153846154,0.169230769230769,
0.184615384615385,0.2,0.215384615384615,0.230769230769231,0.246153846153846,
0.261538461538462,0.276923076923077,0.292307692307692,0.307692307692308,
0.323076923076923,0.338461538461538,0.353846153846154,0.369230769230769,
0.384615384615385,0.4,0.415384615384615,0.430769230769231,0.446153846153846,
0.461538461538462,0.476923076923077,0.492307692307692,0.507692307692308,
0.523076923076923,0.538461538461538,0.553846153846154,0.569230769230769,
0.584615384615384,0.6,0.615384615384615,0.63076923076923,0.646153846153846,
0.661538461538461,0.676923076923076,0.692307692307692,0.707692307692307,
0.723076923076922,0.738461538461538,0.753846153846153,0.769230769230768,
0.784615384615384,0.799999999999999,0.815384615384614,0.83076923076923,
0.846153846153845,0.86153846153846,0.876923076923076,0.892307692307691,
0.907692307692306,0.923076923076922,0.938461538461537,0.953846153846152,
0.969230769230768,0.984615384615383,0.994228156739691),.UNSPECIFIED.)
CURVE()
GEOMETRIC_REPRESENTATION_ITEM()
RATIONAL_B_SPLINE_CURVE((1.,1.,1.,1.,1.,1.,1.,1.,1.,1.,1.,1.,1.,1.,1.,1.,
1.,1.,1.,1.,1.,1.,1.,1.,1.,1.,1.,1.,1.,1.,1.,1.,1.,1.,1.,1.,1.,1.,1.,1.,
1.,1.,1.,1.,1.,1.,1.,1.,1.,1.,1.,1.,1.,1.,1.,1.,1.,1.,1.,1.,1.,1.,1.,1.,
1.,1.,1.,1.,1.,1.))
REPRESENTATION_ITEM('')
);
#281=(
BOUNDED_CURVE()
B_SPLINE_CURVE(5,(#43891,#43892,#43893,#43894,#43895,#43896,#43897,#43898,
#43899,#43900,#43901,#43902,#43903,#43904,#43905,#43906,#43907,#43908,#43909,
#43910,#43911,#43912,#43913,#43914,#43915,#43916,#43917,#43918,#43919,#43920,
#43921,#43922,#43923,#43924,#43925,#43926,#43927,#43928,#43929,#43930,#43931,
#43932,#43933,#43934,#43935,#43936,#43937,#43938,#43939,#43940,#43941,#43942,
#43943,#43944,#43945,#43946,#43947,#43948,#43949,#43950,#43951,#43952,#43953,
#43954,#43955,#43956,#43957,#43958,#43959,#43960),.UNSPECIFIED.,.F.,.F.)
B_SPLINE_CURVE_WITH_KNOTS((6,1,1,1,1,1,1,1,1,1,1,1,1,1,1,1,1,1,1,1,1,1,
1,1,1,1,1,1,1,1,1,1,1,1,1,1,1,1,1,1,1,1,1,1,1,1,1,1,1,1,1,1,1,1,1,1,1,1,
1,1,1,1,1,1,1,6),(0.00577184337450785,0.0153846153846154,0.0307692307692308,
0.0461538461538462,0.0615384615384615,0.0769230769230769,0.0923076923076923,
0.107692307692308,0.123076923076923,0.138461538461538,0.153846153846154,
0.169230769230769,0.184615384615385,0.2,0.215384615384615,0.230769230769231,
0.246153846153846,0.261538461538462,0.276923076923077,0.292307692307692,
0.307692307692308,0.323076923076923,0.338461538461538,0.353846153846154,
0.369230769230769,0.384615384615385,0.4,0.415384615384615,0.430769230769231,
0.446153846153846,0.461538461538462,0.476923076923077,0.492307692307692,
0.507692307692308,0.523076923076923,0.538461538461538,0.553846153846154,
0.569230769230769,0.584615384615384,0.6,0.615384615384615,0.63076923076923,
0.646153846153846,0.661538461538461,0.676923076923076,0.692307692307692,
0.707692307692307,0.723076923076922,0.738461538461538,0.753846153846153,
0.769230769230768,0.784615384615384,0.799999999999999,0.815384615384614,
0.83076923076923,0.846153846153845,0.86153846153846,0.876923076923076,0.892307692307691,
0.907692307692306,0.923076923076922,0.938461538461537,0.953846153846152,
0.969230769230768,0.984615384615383,1.),.UNSPECIFIED.)
CURVE()
GEOMETRIC_REPRESENTATION_ITEM()
RATIONAL_B_SPLINE_CURVE((1.,1.,1.,1.,1.,1.,1.,1.,1.,1.,1.,1.,1.,1.,1.,1.,
1.,1.,1.,1.,1.,1.,1.,1.,1.,1.,1.,1.,1.,1.,1.,1.,1.,1.,1.,1.,1.,1.,1.,1.,
1.,1.,1.,1.,1.,1.,1.,1.,1.,1.,1.,1.,1.,1.,1.,1.,1.,1.,1.,1.,1.,1.,1.,1.,
1.,1.,1.,1.,1.,1.))
REPRESENTATION_ITEM('')
);
#282=(
BOUNDED_CURVE()
B_SPLINE_CURVE(5,(#43964,#43965,#43966,#43967,#43968,#43969,#43970,#43971,
#43972,#43973,#43974,#43975,#43976,#43977,#43978,#43979,#43980,#43981,#43982,
#43983,#43984,#43985,#43986,#43987,#43988,#43989,#43990,#43991,#43992,#43993,
#43994,#43995,#43996,#43997,#43998,#43999,#44000,#44001,#44002,#44003,#44004,
#44005,#44006,#44007,#44008,#44009,#44010,#44011,#44012,#44013,#44014,#44015,
#44016,#44017,#44018,#44019,#44020,#44021,#44022,#44023,#44024,#44025,#44026,
#44027,#44028,#44029,#44030,#44031,#44032,#44033),.UNSPECIFIED.,.F.,.F.)
B_SPLINE_CURVE_WITH_KNOTS((6,1,1,1,1,1,1,1,1,1,1,1,1,1,1,1,1,1,1,1,1,1,
1,1,1,1,1,1,1,1,1,1,1,1,1,1,1,1,1,1,1,1,1,1,1,1,1,1,1,1,1,1,1,1,1,1,1,1,
1,1,1,1,1,1,1,6),(0.,0.0153846153846154,0.0307692307692308,0.0461538461538462,
0.0615384615384615,0.0769230769230769,0.0923076923076923,0.107692307692308,
0.123076923076923,0.138461538461538,0.153846153846154,0.169230769230769,
0.184615384615385,0.2,0.215384615384615,0.230769230769231,0.246153846153846,
0.261538461538462,0.276923076923077,0.292307692307692,0.307692307692308,
0.323076923076923,0.338461538461538,0.353846153846154,0.369230769230769,
0.384615384615385,0.4,0.415384615384615,0.430769230769231,0.446153846153846,
0.461538461538462,0.476923076923077,0.492307692307692,0.507692307692308,
0.523076923076923,0.538461538461538,0.553846153846154,0.569230769230769,
0.584615384615384,0.6,0.615384615384615,0.63076923076923,0.646153846153846,
0.661538461538461,0.676923076923076,0.692307692307692,0.707692307692307,
0.723076923076922,0.738461538461538,0.753846153846153,0.769230769230768,
0.784615384615384,0.799999999999999,0.815384615384614,0.83076923076923,
0.846153846153845,0.86153846153846,0.876923076923076,0.892307692307691,
0.907692307692306,0.923076923076922,0.938461538461537,0.953846153846152,
0.969230769230768,0.984615384615383,0.994228156739708),.UNSPECIFIED.)
CURVE()
GEOMETRIC_REPRESENTATION_ITEM()
RATIONAL_B_SPLINE_CURVE((1.,1.,1.,1.,1.,1.,1.,1.,1.,1.,1.,1.,1.,1.,1.,1.,
1.,1.,1.,1.,1.,1.,1.,1.,1.,1.,1.,1.,1.,1.,1.,1.,1.,1.,1.,1.,1.,1.,1.,1.,
1.,1.,1.,1.,1.,1.,1.,1.,1.,1.,1.,1.,1.,1.,1.,1.,1.,1.,1.,1.,1.,1.,1.,1.,
1.,1.,1.,1.,1.,1.))
REPRESENTATION_ITEM('')
);
#283=(
BOUNDED_CURVE()
B_SPLINE_CURVE(5,(#44037,#44038,#44039,#44040,#44041,#44042,#44043,#44044,
#44045,#44046,#44047,#44048,#44049,#44050,#44051,#44052,#44053,#44054,#44055,
#44056,#44057,#44058,#44059,#44060,#44061,#44062,#44063,#44064,#44065,#44066,
#44067,#44068,#44069,#44070,#44071,#44072,#44073,#44074,#44075,#44076,#44077,
#44078,#44079,#44080,#44081,#44082,#44083,#44084,#44085,#44086,#44087,#44088,
#44089,#44090,#44091,#44092,#44093,#44094,#44095,#44096,#44097,#44098,#44099,
#44100,#44101,#44102,#44103,#44104,#44105,#44106),.UNSPECIFIED.,.F.,.F.)
B_SPLINE_CURVE_WITH_KNOTS((6,1,1,1,1,1,1,1,1,1,1,1,1,1,1,1,1,1,1,1,1,1,
1,1,1,1,1,1,1,1,1,1,1,1,1,1,1,1,1,1,1,1,1,1,1,1,1,1,1,1,1,1,1,1,1,1,1,1,
1,1,1,1,1,1,1,6),(0.00577184337450072,0.0153846153846154,0.0307692307692308,
0.0461538461538462,0.0615384615384615,0.0769230769230769,0.0923076923076923,
0.107692307692308,0.123076923076923,0.138461538461538,0.153846153846154,
0.169230769230769,0.184615384615385,0.2,0.215384615384615,0.230769230769231,
0.246153846153846,0.261538461538462,0.276923076923077,0.292307692307692,
0.307692307692308,0.323076923076923,0.338461538461538,0.353846153846154,
0.369230769230769,0.384615384615385,0.4,0.415384615384615,0.430769230769231,
0.446153846153846,0.461538461538462,0.476923076923077,0.492307692307692,
0.507692307692308,0.523076923076923,0.538461538461538,0.553846153846154,
0.569230769230769,0.584615384615384,0.6,0.615384615384615,0.63076923076923,
0.646153846153846,0.661538461538461,0.676923076923076,0.692307692307692,
0.707692307692307,0.723076923076922,0.738461538461538,0.753846153846153,
0.769230769230768,0.784615384615384,0.799999999999999,0.815384615384614,
0.83076923076923,0.846153846153845,0.86153846153846,0.876923076923076,0.892307692307691,
0.907692307692306,0.923076923076922,0.938461538461537,0.953846153846152,
0.969230769230768,0.984615384615383,1.),.UNSPECIFIED.)
CURVE()
GEOMETRIC_REPRESENTATION_ITEM()
RATIONAL_B_SPLINE_CURVE((1.,1.,1.,1.,1.,1.,1.,1.,1.,1.,1.,1.,1.,1.,1.,1.,
1.,1.,1.,1.,1.,1.,1.,1.,1.,1.,1.,1.,1.,1.,1.,1.,1.,1.,1.,1.,1.,1.,1.,1.,
1.,1.,1.,1.,1.,1.,1.,1.,1.,1.,1.,1.,1.,1.,1.,1.,1.,1.,1.,1.,1.,1.,1.,1.,
1.,1.,1.,1.,1.,1.))
REPRESENTATION_ITEM('')
);
#284=(
BOUNDED_CURVE()
B_SPLINE_CURVE(5,(#44110,#44111,#44112,#44113,#44114,#44115,#44116,#44117,
#44118,#44119,#44120,#44121,#44122,#44123,#44124,#44125,#44126,#44127,#44128,
#44129,#44130,#44131,#44132,#44133,#44134,#44135,#44136,#44137,#44138,#44139,
#44140,#44141,#44142,#44143,#44144,#44145,#44146,#44147,#44148,#44149,#44150,
#44151,#44152,#44153,#44154,#44155,#44156,#44157,#44158,#44159,#44160,#44161,
#44162,#44163,#44164,#44165,#44166,#44167,#44168,#44169,#44170,#44171,#44172,
#44173,#44174,#44175,#44176,#44177,#44178,#44179),.UNSPECIFIED.,.F.,.F.)
B_SPLINE_CURVE_WITH_KNOTS((6,1,1,1,1,1,1,1,1,1,1,1,1,1,1,1,1,1,1,1,1,1,
1,1,1,1,1,1,1,1,1,1,1,1,1,1,1,1,1,1,1,1,1,1,1,1,1,1,1,1,1,1,1,1,1,1,1,1,
1,1,1,1,1,1,1,6),(0.,0.0153846153846154,0.0307692307692308,0.0461538461538462,
0.0615384615384615,0.0769230769230769,0.0923076923076923,0.107692307692308,
0.123076923076923,0.138461538461538,0.153846153846154,0.169230769230769,
0.184615384615385,0.2,0.215384615384615,0.230769230769231,0.246153846153846,
0.261538461538462,0.276923076923077,0.292307692307692,0.307692307692308,
0.323076923076923,0.338461538461538,0.353846153846154,0.369230769230769,
0.384615384615385,0.4,0.415384615384615,0.430769230769231,0.446153846153846,
0.461538461538462,0.476923076923077,0.492307692307692,0.507692307692308,
0.523076923076923,0.538461538461538,0.553846153846154,0.569230769230769,
0.584615384615384,0.6,0.615384615384615,0.63076923076923,0.646153846153846,
0.661538461538461,0.676923076923076,0.692307692307692,0.707692307692307,
0.723076923076922,0.738461538461538,0.753846153846153,0.769230769230768,
0.784615384615384,0.799999999999999,0.815384615384614,0.83076923076923,
0.846153846153845,0.86153846153846,0.876923076923076,0.892307692307691,
0.907692307692306,0.923076923076922,0.938461538461537,0.953846153846152,
0.969230769230768,0.984615384615383,0.994228156739706),.UNSPECIFIED.)
CURVE()
GEOMETRIC_REPRESENTATION_ITEM()
RATIONAL_B_SPLINE_CURVE((1.,1.,1.,1.,1.,1.,1.,1.,1.,1.,1.,1.,1.,1.,1.,1.,
1.,1.,1.,1.,1.,1.,1.,1.,1.,1.,1.,1.,1.,1.,1.,1.,1.,1.,1.,1.,1.,1.,1.,1.,
1.,1.,1.,1.,1.,1.,1.,1.,1.,1.,1.,1.,1.,1.,1.,1.,1.,1.,1.,1.,1.,1.,1.,1.,
1.,1.,1.,1.,1.,1.))
REPRESENTATION_ITEM('')
);
#285=(
BOUNDED_CURVE()
B_SPLINE_CURVE(5,(#44183,#44184,#44185,#44186,#44187,#44188,#44189,#44190,
#44191,#44192,#44193,#44194,#44195,#44196,#44197,#44198,#44199,#44200,#44201,
#44202,#44203,#44204,#44205,#44206,#44207,#44208,#44209,#44210,#44211,#44212,
#44213,#44214,#44215,#44216,#44217,#44218,#44219,#44220,#44221,#44222,#44223,
#44224,#44225,#44226,#44227,#44228,#44229,#44230,#44231,#44232,#44233,#44234,
#44235,#44236,#44237,#44238,#44239,#44240,#44241,#44242,#44243,#44244,#44245,
#44246,#44247,#44248,#44249,#44250,#44251,#44252),.UNSPECIFIED.,.F.,.F.)
B_SPLINE_CURVE_WITH_KNOTS((6,1,1,1,1,1,1,1,1,1,1,1,1,1,1,1,1,1,1,1,1,1,
1,1,1,1,1,1,1,1,1,1,1,1,1,1,1,1,1,1,1,1,1,1,1,1,1,1,1,1,1,1,1,1,1,1,1,1,
1,1,1,1,1,1,1,6),(0.00577184337450902,0.0153846153846154,0.0307692307692308,
0.0461538461538462,0.0615384615384615,0.0769230769230769,0.0923076923076923,
0.107692307692308,0.123076923076923,0.138461538461538,0.153846153846154,
0.169230769230769,0.184615384615385,0.2,0.215384615384615,0.230769230769231,
0.246153846153846,0.261538461538462,0.276923076923077,0.292307692307692,
0.307692307692308,0.323076923076923,0.338461538461538,0.353846153846154,
0.369230769230769,0.384615384615385,0.4,0.415384615384615,0.430769230769231,
0.446153846153846,0.461538461538462,0.476923076923077,0.492307692307692,
0.507692307692308,0.523076923076923,0.538461538461538,0.553846153846154,
0.569230769230769,0.584615384615384,0.6,0.615384615384615,0.63076923076923,
0.646153846153846,0.661538461538461,0.676923076923076,0.692307692307692,
0.707692307692307,0.723076923076922,0.738461538461538,0.753846153846153,
0.769230769230768,0.784615384615384,0.799999999999999,0.815384615384614,
0.83076923076923,0.846153846153845,0.86153846153846,0.876923076923076,0.892307692307691,
0.907692307692306,0.923076923076922,0.938461538461537,0.953846153846152,
0.969230769230768,0.984615384615383,1.),.UNSPECIFIED.)
CURVE()
GEOMETRIC_REPRESENTATION_ITEM()
RATIONAL_B_SPLINE_CURVE((1.,1.,1.,1.,1.,1.,1.,1.,1.,1.,1.,1.,1.,1.,1.,1.,
1.,1.,1.,1.,1.,1.,1.,1.,1.,1.,1.,1.,1.,1.,1.,1.,1.,1.,1.,1.,1.,1.,1.,1.,
1.,1.,1.,1.,1.,1.,1.,1.,1.,1.,1.,1.,1.,1.,1.,1.,1.,1.,1.,1.,1.,1.,1.,1.,
1.,1.,1.,1.,1.,1.))
REPRESENTATION_ITEM('')
);
#286=(
BOUNDED_CURVE()
B_SPLINE_CURVE(5,(#44256,#44257,#44258,#44259,#44260,#44261,#44262,#44263,
#44264,#44265,#44266,#44267,#44268,#44269,#44270,#44271,#44272,#44273,#44274,
#44275,#44276,#44277,#44278,#44279,#44280,#44281,#44282,#44283,#44284,#44285,
#44286,#44287,#44288,#44289,#44290,#44291,#44292,#44293,#44294,#44295,#44296,
#44297,#44298,#44299,#44300,#44301,#44302,#44303,#44304,#44305,#44306,#44307,
#44308,#44309,#44310,#44311,#44312,#44313,#44314,#44315,#44316,#44317,#44318,
#44319,#44320,#44321,#44322,#44323,#44324,#44325),.UNSPECIFIED.,.F.,.F.)
B_SPLINE_CURVE_WITH_KNOTS((6,1,1,1,1,1,1,1,1,1,1,1,1,1,1,1,1,1,1,1,1,1,
1,1,1,1,1,1,1,1,1,1,1,1,1,1,1,1,1,1,1,1,1,1,1,1,1,1,1,1,1,1,1,1,1,1,1,1,
1,1,1,1,1,1,1,6),(0.,0.0153846153846154,0.0307692307692308,0.0461538461538462,
0.0615384615384615,0.0769230769230769,0.0923076923076923,0.107692307692308,
0.123076923076923,0.138461538461538,0.153846153846154,0.169230769230769,
0.184615384615385,0.2,0.215384615384615,0.230769230769231,0.246153846153846,
0.261538461538462,0.276923076923077,0.292307692307692,0.307692307692308,
0.323076923076923,0.338461538461538,0.353846153846154,0.369230769230769,
0.384615384615385,0.4,0.415384615384615,0.430769230769231,0.446153846153846,
0.461538461538462,0.476923076923077,0.492307692307692,0.507692307692308,
0.523076923076923,0.538461538461538,0.553846153846154,0.569230769230769,
0.584615384615384,0.6,0.615384615384615,0.63076923076923,0.646153846153846,
0.661538461538461,0.676923076923076,0.692307692307692,0.707692307692307,
0.723076923076922,0.738461538461538,0.753846153846153,0.769230769230768,
0.784615384615384,0.799999999999999,0.815384615384614,0.83076923076923,
0.846153846153845,0.86153846153846,0.876923076923076,0.892307692307691,
0.907692307692306,0.923076923076922,0.938461538461537,0.953846153846152,
0.969230769230768,0.984615384615383,0.994228156739698),.UNSPECIFIED.)
CURVE()
GEOMETRIC_REPRESENTATION_ITEM()
RATIONAL_B_SPLINE_CURVE((1.,1.,1.,1.,1.,1.,1.,1.,1.,1.,1.,1.,1.,1.,1.,1.,
1.,1.,1.,1.,1.,1.,1.,1.,1.,1.,1.,1.,1.,1.,1.,1.,1.,1.,1.,1.,1.,1.,1.,1.,
1.,1.,1.,1.,1.,1.,1.,1.,1.,1.,1.,1.,1.,1.,1.,1.,1.,1.,1.,1.,1.,1.,1.,1.,
1.,1.,1.,1.,1.,1.))
REPRESENTATION_ITEM('')
);
#287=(
BOUNDED_CURVE()
B_SPLINE_CURVE(5,(#44329,#44330,#44331,#44332,#44333,#44334,#44335,#44336,
#44337,#44338,#44339,#44340,#44341,#44342,#44343,#44344,#44345,#44346,#44347,
#44348,#44349,#44350,#44351,#44352,#44353,#44354,#44355,#44356,#44357,#44358,
#44359,#44360,#44361,#44362,#44363,#44364,#44365,#44366,#44367,#44368,#44369,
#44370,#44371,#44372,#44373,#44374,#44375,#44376,#44377,#44378,#44379,#44380,
#44381,#44382,#44383,#44384,#44385,#44386,#44387,#44388,#44389,#44390,#44391,
#44392,#44393,#44394,#44395,#44396,#44397,#44398),.UNSPECIFIED.,.F.,.F.)
B_SPLINE_CURVE_WITH_KNOTS((6,1,1,1,1,1,1,1,1,1,1,1,1,1,1,1,1,1,1,1,1,1,
1,1,1,1,1,1,1,1,1,1,1,1,1,1,1,1,1,1,1,1,1,1,1,1,1,1,1,1,1,1,1,1,1,1,1,1,
1,1,1,1,1,1,1,6),(0.00577184337451611,0.0153846153846154,0.0307692307692308,
0.0461538461538462,0.0615384615384615,0.0769230769230769,0.0923076923076923,
0.107692307692308,0.123076923076923,0.138461538461538,0.153846153846154,
0.169230769230769,0.184615384615385,0.2,0.215384615384615,0.230769230769231,
0.246153846153846,0.261538461538462,0.276923076923077,0.292307692307692,
0.307692307692308,0.323076923076923,0.338461538461538,0.353846153846154,
0.369230769230769,0.384615384615385,0.4,0.415384615384615,0.430769230769231,
0.446153846153846,0.461538461538462,0.476923076923077,0.492307692307692,
0.507692307692308,0.523076923076923,0.538461538461538,0.553846153846154,
0.569230769230769,0.584615384615384,0.6,0.615384615384615,0.63076923076923,
0.646153846153846,0.661538461538461,0.676923076923076,0.692307692307692,
0.707692307692307,0.723076923076922,0.738461538461538,0.753846153846153,
0.769230769230768,0.784615384615384,0.799999999999999,0.815384615384614,
0.83076923076923,0.846153846153845,0.86153846153846,0.876923076923076,0.892307692307691,
0.907692307692306,0.923076923076922,0.938461538461537,0.953846153846152,
0.969230769230768,0.984615384615383,1.),.UNSPECIFIED.)
CURVE()
GEOMETRIC_REPRESENTATION_ITEM()
RATIONAL_B_SPLINE_CURVE((1.,1.,1.,1.,1.,1.,1.,1.,1.,1.,1.,1.,1.,1.,1.,1.,
1.,1.,1.,1.,1.,1.,1.,1.,1.,1.,1.,1.,1.,1.,1.,1.,1.,1.,1.,1.,1.,1.,1.,1.,
1.,1.,1.,1.,1.,1.,1.,1.,1.,1.,1.,1.,1.,1.,1.,1.,1.,1.,1.,1.,1.,1.,1.,1.,
1.,1.,1.,1.,1.,1.))
REPRESENTATION_ITEM('')
);
#288=(
BOUNDED_CURVE()
B_SPLINE_CURVE(5,(#44402,#44403,#44404,#44405,#44406,#44407,#44408,#44409,
#44410,#44411,#44412,#44413,#44414,#44415,#44416,#44417,#44418,#44419,#44420,
#44421,#44422,#44423,#44424,#44425,#44426,#44427,#44428,#44429,#44430,#44431,
#44432,#44433,#44434,#44435,#44436,#44437,#44438,#44439,#44440,#44441,#44442,
#44443,#44444,#44445,#44446,#44447,#44448,#44449,#44450,#44451,#44452,#44453,
#44454,#44455,#44456,#44457,#44458,#44459,#44460,#44461,#44462,#44463,#44464,
#44465,#44466,#44467,#44468,#44469,#44470,#44471),.UNSPECIFIED.,.F.,.F.)
B_SPLINE_CURVE_WITH_KNOTS((6,1,1,1,1,1,1,1,1,1,1,1,1,1,1,1,1,1,1,1,1,1,
1,1,1,1,1,1,1,1,1,1,1,1,1,1,1,1,1,1,1,1,1,1,1,1,1,1,1,1,1,1,1,1,1,1,1,1,
1,1,1,1,1,1,1,6),(0.,0.0153846153846154,0.0307692307692308,0.0461538461538462,
0.0615384615384615,0.0769230769230769,0.0923076923076923,0.107692307692308,
0.123076923076923,0.138461538461538,0.153846153846154,0.169230769230769,
0.184615384615385,0.2,0.215384615384615,0.230769230769231,0.246153846153846,
0.261538461538462,0.276923076923077,0.292307692307692,0.307692307692308,
0.323076923076923,0.338461538461538,0.353846153846154,0.369230769230769,
0.384615384615385,0.4,0.415384615384615,0.430769230769231,0.446153846153846,
0.461538461538462,0.476923076923077,0.492307692307692,0.507692307692308,
0.523076923076923,0.538461538461538,0.553846153846154,0.569230769230769,
0.584615384615384,0.6,0.615384615384615,0.63076923076923,0.646153846153846,
0.661538461538461,0.676923076923076,0.692307692307692,0.707692307692307,
0.723076923076922,0.738461538461538,0.753846153846153,0.769230769230768,
0.784615384615384,0.799999999999999,0.815384615384614,0.83076923076923,
0.846153846153845,0.86153846153846,0.876923076923076,0.892307692307691,
0.907692307692306,0.923076923076922,0.938461538461537,0.953846153846152,
0.969230769230768,0.984615384615383,0.994228156739704),.UNSPECIFIED.)
CURVE()
GEOMETRIC_REPRESENTATION_ITEM()
RATIONAL_B_SPLINE_CURVE((1.,1.,1.,1.,1.,1.,1.,1.,1.,1.,1.,1.,1.,1.,1.,1.,
1.,1.,1.,1.,1.,1.,1.,1.,1.,1.,1.,1.,1.,1.,1.,1.,1.,1.,1.,1.,1.,1.,1.,1.,
1.,1.,1.,1.,1.,1.,1.,1.,1.,1.,1.,1.,1.,1.,1.,1.,1.,1.,1.,1.,1.,1.,1.,1.,
1.,1.,1.,1.,1.,1.))
REPRESENTATION_ITEM('')
);
#289=(
BOUNDED_CURVE()
B_SPLINE_CURVE(5,(#44475,#44476,#44477,#44478,#44479,#44480,#44481,#44482,
#44483,#44484,#44485,#44486,#44487,#44488,#44489,#44490,#44491,#44492,#44493,
#44494,#44495,#44496,#44497,#44498,#44499,#44500,#44501,#44502,#44503,#44504,
#44505,#44506,#44507,#44508,#44509,#44510,#44511,#44512,#44513,#44514,#44515,
#44516,#44517,#44518,#44519,#44520,#44521,#44522,#44523,#44524,#44525,#44526,
#44527,#44528,#44529,#44530,#44531,#44532,#44533,#44534,#44535,#44536,#44537,
#44538,#44539,#44540,#44541,#44542,#44543,#44544),.UNSPECIFIED.,.F.,.F.)
B_SPLINE_CURVE_WITH_KNOTS((6,1,1,1,1,1,1,1,1,1,1,1,1,1,1,1,1,1,1,1,1,1,
1,1,1,1,1,1,1,1,1,1,1,1,1,1,1,1,1,1,1,1,1,1,1,1,1,1,1,1,1,1,1,1,1,1,1,1,
1,1,1,1,1,1,1,6),(0.00577184337449692,0.0153846153846154,0.0307692307692308,
0.0461538461538462,0.0615384615384615,0.0769230769230769,0.0923076923076923,
0.107692307692308,0.123076923076923,0.138461538461538,0.153846153846154,
0.169230769230769,0.184615384615385,0.2,0.215384615384615,0.230769230769231,
0.246153846153846,0.261538461538462,0.276923076923077,0.292307692307692,
0.307692307692308,0.323076923076923,0.338461538461538,0.353846153846154,
0.369230769230769,0.384615384615385,0.4,0.415384615384615,0.430769230769231,
0.446153846153846,0.461538461538462,0.476923076923077,0.492307692307692,
0.507692307692308,0.523076923076923,0.538461538461538,0.553846153846154,
0.569230769230769,0.584615384615384,0.6,0.615384615384615,0.63076923076923,
0.646153846153846,0.661538461538461,0.676923076923076,0.692307692307692,
0.707692307692307,0.723076923076922,0.738461538461538,0.753846153846153,
0.769230769230768,0.784615384615384,0.799999999999999,0.815384615384614,
0.83076923076923,0.846153846153845,0.86153846153846,0.876923076923076,0.892307692307691,
0.907692307692306,0.923076923076922,0.938461538461537,0.953846153846152,
0.969230769230768,0.984615384615383,1.),.UNSPECIFIED.)
CURVE()
GEOMETRIC_REPRESENTATION_ITEM()
RATIONAL_B_SPLINE_CURVE((1.,1.,1.,1.,1.,1.,1.,1.,1.,1.,1.,1.,1.,1.,1.,1.,
1.,1.,1.,1.,1.,1.,1.,1.,1.,1.,1.,1.,1.,1.,1.,1.,1.,1.,1.,1.,1.,1.,1.,1.,
1.,1.,1.,1.,1.,1.,1.,1.,1.,1.,1.,1.,1.,1.,1.,1.,1.,1.,1.,1.,1.,1.,1.,1.,
1.,1.,1.,1.,1.,1.))
REPRESENTATION_ITEM('')
);
#290=(
BOUNDED_CURVE()
B_SPLINE_CURVE(5,(#44547,#44548,#44549,#44550,#44551,#44552,#44553,#44554,
#44555,#44556,#44557,#44558,#44559,#44560,#44561,#44562,#44563,#44564,#44565,
#44566,#44567,#44568,#44569,#44570,#44571,#44572,#44573,#44574,#44575,#44576,
#44577,#44578,#44579,#44580,#44581,#44582,#44583,#44584,#44585,#44586,#44587,
#44588,#44589,#44590,#44591,#44592,#44593,#44594,#44595,#44596,#44597,#44598,
#44599,#44600,#44601,#44602,#44603,#44604,#44605,#44606,#44607,#44608,#44609,
#44610,#44611,#44612,#44613,#44614,#44615,#44616),.UNSPECIFIED.,.F.,.F.)
B_SPLINE_CURVE_WITH_KNOTS((6,1,1,1,1,1,1,1,1,1,1,1,1,1,1,1,1,1,1,1,1,1,
1,1,1,1,1,1,1,1,1,1,1,1,1,1,1,1,1,1,1,1,1,1,1,1,1,1,1,1,1,1,1,1,1,1,1,1,
1,1,1,1,1,1,1,6),(0.,0.0153846153846154,0.0307692307692308,0.0461538461538462,
0.0615384615384615,0.0769230769230769,0.0923076923076923,0.107692307692308,
0.123076923076923,0.138461538461538,0.153846153846154,0.169230769230769,
0.184615384615385,0.2,0.215384615384615,0.230769230769231,0.246153846153846,
0.261538461538462,0.276923076923077,0.292307692307692,0.307692307692308,
0.323076923076923,0.338461538461538,0.353846153846154,0.369230769230769,
0.384615384615385,0.4,0.415384615384615,0.430769230769231,0.446153846153846,
0.461538461538462,0.476923076923077,0.492307692307692,0.507692307692308,
0.523076923076923,0.538461538461538,0.553846153846154,0.569230769230769,
0.584615384615384,0.6,0.615384615384615,0.63076923076923,0.646153846153846,
0.661538461538461,0.676923076923076,0.692307692307692,0.707692307692307,
0.723076923076922,0.738461538461538,0.753846153846153,0.769230769230768,
0.784615384615384,0.799999999999999,0.815384615384614,0.83076923076923,
0.846153846153845,0.86153846153846,0.876923076923076,0.892307692307691,
0.907692307692306,0.923076923076922,0.938461538461537,0.953846153846152,
0.969230769230768,0.984615384615383,0.994228156739723),.UNSPECIFIED.)
CURVE()
GEOMETRIC_REPRESENTATION_ITEM()
RATIONAL_B_SPLINE_CURVE((1.,1.,1.,1.,1.,1.,1.,1.,1.,1.,1.,1.,1.,1.,1.,1.,
1.,1.,1.,1.,1.,1.,1.,1.,1.,1.,1.,1.,1.,1.,1.,1.,1.,1.,1.,1.,1.,1.,1.,1.,
1.,1.,1.,1.,1.,1.,1.,1.,1.,1.,1.,1.,1.,1.,1.,1.,1.,1.,1.,1.,1.,1.,1.,1.,
1.,1.,1.,1.,1.,1.))
REPRESENTATION_ITEM('')
);
#291=(
BOUNDED_CURVE()
B_SPLINE_CURVE(5,(#44775,#44776,#44777,#44778,#44779,#44780,#44781,#44782,
#44783,#44784,#44785,#44786,#44787,#44788,#44789,#44790,#44791,#44792,#44793,
#44794,#44795,#44796,#44797,#44798,#44799,#44800,#44801,#44802,#44803,#44804,
#44805,#44806,#44807,#44808,#44809,#44810,#44811,#44812,#44813,#44814,#44815,
#44816,#44817,#44818,#44819,#44820,#44821,#44822,#44823,#44824,#44825,#44826,
#44827,#44828,#44829,#44830,#44831,#44832,#44833,#44834,#44835,#44836,#44837,
#44838,#44839,#44840,#44841,#44842,#44843,#44844),.UNSPECIFIED.,.F.,.F.)
B_SPLINE_CURVE_WITH_KNOTS((6,1,1,1,1,1,1,1,1,1,1,1,1,1,1,1,1,1,1,1,1,1,
1,1,1,1,1,1,1,1,1,1,1,1,1,1,1,1,1,1,1,1,1,1,1,1,1,1,1,1,1,1,1,1,1,1,1,1,
1,1,1,1,1,1,1,6),(-1.,-0.984615384615383,-0.969230769230768,-0.953846153846152,
-0.938461538461537,-0.923076923076922,-0.907692307692306,-0.892307692307691,
-0.876923076923076,-0.86153846153846,-0.846153846153845,-0.83076923076923,
-0.815384615384614,-0.799999999999999,-0.784615384615384,-0.769230769230768,
-0.753846153846153,-0.738461538461538,-0.723076923076922,-0.707692307692307,
-0.692307692307692,-0.676923076923076,-0.661538461538461,-0.646153846153846,
-0.63076923076923,-0.615384615384615,-0.6,-0.584615384615384,-0.569230769230769,
-0.553846153846154,-0.538461538461538,-0.523076923076923,-0.507692307692308,
-0.492307692307692,-0.476923076923077,-0.461538461538462,-0.446153846153846,
-0.430769230769231,-0.415384615384615,-0.4,-0.384615384615385,-0.369230769230769,
-0.353846153846154,-0.338461538461538,-0.323076923076923,-0.307692307692308,
-0.292307692307692,-0.276923076923077,-0.261538461538462,-0.246153846153846,
-0.230769230769231,-0.215384615384615,-0.2,-0.184615384615385,-0.169230769230769,
-0.153846153846154,-0.138461538461538,-0.123076923076923,-0.107692307692308,
-0.0923076923076923,-0.0769230769230769,-0.0615384615384615,-0.0461538461538462,
-0.0307692307692308,-0.0153846153846154,-0.00577184337448906),
 .UNSPECIFIED.)
CURVE()
GEOMETRIC_REPRESENTATION_ITEM()
RATIONAL_B_SPLINE_CURVE((1.,1.,1.,1.,1.,1.,1.,1.,1.,1.,1.,1.,1.,1.,1.,1.,
1.,1.,1.,1.,1.,1.,1.,1.,1.,1.,1.,1.,1.,1.,1.,1.,1.,1.,1.,1.,1.,1.,1.,1.,
1.,1.,1.,1.,1.,1.,1.,1.,1.,1.,1.,1.,1.,1.,1.,1.,1.,1.,1.,1.,1.,1.,1.,1.,
1.,1.,1.,1.,1.,1.))
REPRESENTATION_ITEM('')
);
#292=(
BOUNDED_CURVE()
B_SPLINE_CURVE(5,(#44995,#44996,#44997,#44998,#44999,#45000,#45001,#45002,
#45003,#45004,#45005,#45006,#45007,#45008,#45009,#45010,#45011,#45012,#45013,
#45014,#45015,#45016,#45017,#45018,#45019,#45020,#45021,#45022,#45023,#45024,
#45025,#45026,#45027,#45028,#45029,#45030,#45031,#45032,#45033,#45034,#45035,
#45036,#45037,#45038,#45039,#45040,#45041,#45042,#45043,#45044,#45045,#45046,
#45047,#45048,#45049,#45050,#45051,#45052,#45053,#45054,#45055,#45056,#45057,
#45058,#45059,#45060,#45061,#45062,#45063,#45064),.UNSPECIFIED.,.F.,.F.)
B_SPLINE_CURVE_WITH_KNOTS((6,1,1,1,1,1,1,1,1,1,1,1,1,1,1,1,1,1,1,1,1,1,
1,1,1,1,1,1,1,1,1,1,1,1,1,1,1,1,1,1,1,1,1,1,1,1,1,1,1,1,1,1,1,1,1,1,1,1,
1,1,1,1,1,1,1,6),(-0.994228156739728,-0.984615384615383,-0.969230769230768,
-0.953846153846152,-0.938461538461537,-0.923076923076922,-0.907692307692306,
-0.892307692307691,-0.876923076923076,-0.86153846153846,-0.846153846153845,
-0.83076923076923,-0.815384615384614,-0.799999999999999,-0.784615384615384,
-0.769230769230768,-0.753846153846153,-0.738461538461538,-0.723076923076922,
-0.707692307692307,-0.692307692307692,-0.676923076923076,-0.661538461538461,
-0.646153846153846,-0.63076923076923,-0.615384615384615,-0.6,-0.584615384615384,
-0.569230769230769,-0.553846153846154,-0.538461538461538,-0.523076923076923,
-0.507692307692308,-0.492307692307692,-0.476923076923077,-0.461538461538462,
-0.446153846153846,-0.430769230769231,-0.415384615384615,-0.4,-0.384615384615385,
-0.369230769230769,-0.353846153846154,-0.338461538461538,-0.323076923076923,
-0.307692307692308,-0.292307692307692,-0.276923076923077,-0.261538461538462,
-0.246153846153846,-0.230769230769231,-0.215384615384615,-0.2,-0.184615384615385,
-0.169230769230769,-0.153846153846154,-0.138461538461538,-0.123076923076923,
-0.107692307692308,-0.0923076923076923,-0.0769230769230769,-0.0615384615384615,
-0.0461538461538462,-0.0307692307692308,-0.0153846153846154,0.),
 .UNSPECIFIED.)
CURVE()
GEOMETRIC_REPRESENTATION_ITEM()
RATIONAL_B_SPLINE_CURVE((1.,1.,1.,1.,1.,1.,1.,1.,1.,1.,1.,1.,1.,1.,1.,1.,
1.,1.,1.,1.,1.,1.,1.,1.,1.,1.,1.,1.,1.,1.,1.,1.,1.,1.,1.,1.,1.,1.,1.,1.,
1.,1.,1.,1.,1.,1.,1.,1.,1.,1.,1.,1.,1.,1.,1.,1.,1.,1.,1.,1.,1.,1.,1.,1.,
1.,1.,1.,1.,1.,1.))
REPRESENTATION_ITEM('')
);
#293=(
BOUNDED_CURVE()
B_SPLINE_CURVE(5,(#45217,#45218,#45219,#45220,#45221,#45222,#45223,#45224,
#45225,#45226,#45227,#45228,#45229,#45230,#45231,#45232,#45233,#45234,#45235,
#45236,#45237,#45238,#45239,#45240,#45241,#45242,#45243,#45244,#45245,#45246,
#45247,#45248,#45249,#45250,#45251,#45252,#45253,#45254,#45255,#45256,#45257,
#45258,#45259,#45260,#45261,#45262,#45263,#45264,#45265,#45266,#45267,#45268,
#45269,#45270,#45271,#45272,#45273,#45274,#45275,#45276,#45277,#45278,#45279,
#45280,#45281,#45282,#45283,#45284,#45285,#45286),.UNSPECIFIED.,.F.,.F.)
B_SPLINE_CURVE_WITH_KNOTS((6,1,1,1,1,1,1,1,1,1,1,1,1,1,1,1,1,1,1,1,1,1,
1,1,1,1,1,1,1,1,1,1,1,1,1,1,1,1,1,1,1,1,1,1,1,1,1,1,1,1,1,1,1,1,1,1,1,1,
1,1,1,1,1,1,1,6),(-1.,-0.984615384615383,-0.969230769230768,-0.953846153846152,
-0.938461538461537,-0.923076923076922,-0.907692307692306,-0.892307692307691,
-0.876923076923076,-0.86153846153846,-0.846153846153845,-0.83076923076923,
-0.815384615384614,-0.799999999999999,-0.784615384615384,-0.769230769230768,
-0.753846153846153,-0.738461538461538,-0.723076923076922,-0.707692307692307,
-0.692307692307692,-0.676923076923076,-0.661538461538461,-0.646153846153846,
-0.63076923076923,-0.615384615384615,-0.6,-0.584615384615384,-0.569230769230769,
-0.553846153846154,-0.538461538461538,-0.523076923076923,-0.507692307692308,
-0.492307692307692,-0.476923076923077,-0.461538461538462,-0.446153846153846,
-0.430769230769231,-0.415384615384615,-0.4,-0.384615384615385,-0.369230769230769,
-0.353846153846154,-0.338461538461538,-0.323076923076923,-0.307692307692308,
-0.292307692307692,-0.276923076923077,-0.261538461538462,-0.246153846153846,
-0.230769230769231,-0.215384615384615,-0.2,-0.184615384615385,-0.169230769230769,
-0.153846153846154,-0.138461538461538,-0.123076923076923,-0.107692307692308,
-0.0923076923076923,-0.0769230769230769,-0.0615384615384615,-0.0461538461538462,
-0.0307692307692308,-0.0153846153846154,-0.0057718433744926),
 .UNSPECIFIED.)
CURVE()
GEOMETRIC_REPRESENTATION_ITEM()
RATIONAL_B_SPLINE_CURVE((1.,1.,1.,1.,1.,1.,1.,1.,1.,1.,1.,1.,1.,1.,1.,1.,
1.,1.,1.,1.,1.,1.,1.,1.,1.,1.,1.,1.,1.,1.,1.,1.,1.,1.,1.,1.,1.,1.,1.,1.,
1.,1.,1.,1.,1.,1.,1.,1.,1.,1.,1.,1.,1.,1.,1.,1.,1.,1.,1.,1.,1.,1.,1.,1.,
1.,1.,1.,1.,1.,1.))
REPRESENTATION_ITEM('')
);
#294=(
BOUNDED_CURVE()
B_SPLINE_CURVE(5,(#45437,#45438,#45439,#45440,#45441,#45442,#45443,#45444,
#45445,#45446,#45447,#45448,#45449,#45450,#45451,#45452,#45453,#45454,#45455,
#45456,#45457,#45458,#45459,#45460,#45461,#45462,#45463,#45464,#45465,#45466,
#45467,#45468,#45469,#45470,#45471,#45472,#45473,#45474,#45475,#45476,#45477,
#45478,#45479,#45480,#45481,#45482,#45483,#45484,#45485,#45486,#45487,#45488,
#45489,#45490,#45491,#45492,#45493,#45494,#45495,#45496,#45497,#45498,#45499,
#45500,#45501,#45502,#45503,#45504,#45505,#45506),.UNSPECIFIED.,.F.,.F.)
B_SPLINE_CURVE_WITH_KNOTS((6,1,1,1,1,1,1,1,1,1,1,1,1,1,1,1,1,1,1,1,1,1,
1,1,1,1,1,1,1,1,1,1,1,1,1,1,1,1,1,1,1,1,1,1,1,1,1,1,1,1,1,1,1,1,1,1,1,1,
1,1,1,1,1,1,1,6),(-0.994228156739718,-0.984615384615383,-0.969230769230768,
-0.953846153846152,-0.938461538461537,-0.923076923076922,-0.907692307692306,
-0.892307692307691,-0.876923076923076,-0.86153846153846,-0.846153846153845,
-0.83076923076923,-0.815384615384614,-0.799999999999999,-0.784615384615384,
-0.769230769230768,-0.753846153846153,-0.738461538461538,-0.723076923076922,
-0.707692307692307,-0.692307692307692,-0.676923076923076,-0.661538461538461,
-0.646153846153846,-0.63076923076923,-0.615384615384615,-0.6,-0.584615384615384,
-0.569230769230769,-0.553846153846154,-0.538461538461538,-0.523076923076923,
-0.507692307692308,-0.492307692307692,-0.476923076923077,-0.461538461538462,
-0.446153846153846,-0.430769230769231,-0.415384615384615,-0.4,-0.384615384615385,
-0.369230769230769,-0.353846153846154,-0.338461538461538,-0.323076923076923,
-0.307692307692308,-0.292307692307692,-0.276923076923077,-0.261538461538462,
-0.246153846153846,-0.230769230769231,-0.215384615384615,-0.2,-0.184615384615385,
-0.169230769230769,-0.153846153846154,-0.138461538461538,-0.123076923076923,
-0.107692307692308,-0.0923076923076923,-0.0769230769230769,-0.0615384615384615,
-0.0461538461538462,-0.0307692307692308,-0.0153846153846154,0.),
 .UNSPECIFIED.)
CURVE()
GEOMETRIC_REPRESENTATION_ITEM()
RATIONAL_B_SPLINE_CURVE((1.,1.,1.,1.,1.,1.,1.,1.,1.,1.,1.,1.,1.,1.,1.,1.,
1.,1.,1.,1.,1.,1.,1.,1.,1.,1.,1.,1.,1.,1.,1.,1.,1.,1.,1.,1.,1.,1.,1.,1.,
1.,1.,1.,1.,1.,1.,1.,1.,1.,1.,1.,1.,1.,1.,1.,1.,1.,1.,1.,1.,1.,1.,1.,1.,
1.,1.,1.,1.,1.,1.))
REPRESENTATION_ITEM('')
);
#295=(
BOUNDED_CURVE()
B_SPLINE_CURVE(5,(#45659,#45660,#45661,#45662,#45663,#45664,#45665,#45666,
#45667,#45668,#45669,#45670,#45671,#45672,#45673,#45674,#45675,#45676,#45677,
#45678,#45679,#45680,#45681,#45682,#45683,#45684,#45685,#45686,#45687,#45688,
#45689,#45690,#45691,#45692,#45693,#45694,#45695,#45696,#45697,#45698,#45699,
#45700,#45701,#45702,#45703,#45704,#45705,#45706,#45707,#45708,#45709,#45710,
#45711,#45712,#45713,#45714,#45715,#45716,#45717,#45718,#45719,#45720,#45721,
#45722,#45723,#45724,#45725,#45726,#45727,#45728),.UNSPECIFIED.,.F.,.F.)
B_SPLINE_CURVE_WITH_KNOTS((6,1,1,1,1,1,1,1,1,1,1,1,1,1,1,1,1,1,1,1,1,1,
1,1,1,1,1,1,1,1,1,1,1,1,1,1,1,1,1,1,1,1,1,1,1,1,1,1,1,1,1,1,1,1,1,1,1,1,
1,1,1,1,1,1,1,6),(-1.,-0.984615384615383,-0.969230769230768,-0.953846153846152,
-0.938461538461537,-0.923076923076922,-0.907692307692306,-0.892307692307691,
-0.876923076923076,-0.86153846153846,-0.846153846153845,-0.83076923076923,
-0.815384615384614,-0.799999999999999,-0.784615384615384,-0.769230769230768,
-0.753846153846153,-0.738461538461538,-0.723076923076922,-0.707692307692307,
-0.692307692307692,-0.676923076923076,-0.661538461538461,-0.646153846153846,
-0.63076923076923,-0.615384615384615,-0.6,-0.584615384615384,-0.569230769230769,
-0.553846153846154,-0.538461538461538,-0.523076923076923,-0.507692307692308,
-0.492307692307692,-0.476923076923077,-0.461538461538462,-0.446153846153846,
-0.430769230769231,-0.415384615384615,-0.4,-0.384615384615385,-0.369230769230769,
-0.353846153846154,-0.338461538461538,-0.323076923076923,-0.307692307692308,
-0.292307692307692,-0.276923076923077,-0.261538461538462,-0.246153846153846,
-0.230769230769231,-0.215384615384615,-0.2,-0.184615384615385,-0.169230769230769,
-0.153846153846154,-0.138461538461538,-0.123076923076923,-0.107692307692308,
-0.0923076923076923,-0.0769230769230769,-0.0615384615384615,-0.0461538461538462,
-0.0307692307692308,-0.0153846153846154,-0.00577184337449396),
 .UNSPECIFIED.)
CURVE()
GEOMETRIC_REPRESENTATION_ITEM()
RATIONAL_B_SPLINE_CURVE((1.,1.,1.,1.,1.,1.,1.,1.,1.,1.,1.,1.,1.,1.,1.,1.,
1.,1.,1.,1.,1.,1.,1.,1.,1.,1.,1.,1.,1.,1.,1.,1.,1.,1.,1.,1.,1.,1.,1.,1.,
1.,1.,1.,1.,1.,1.,1.,1.,1.,1.,1.,1.,1.,1.,1.,1.,1.,1.,1.,1.,1.,1.,1.,1.,
1.,1.,1.,1.,1.,1.))
REPRESENTATION_ITEM('')
);
#296=(
BOUNDED_CURVE()
B_SPLINE_CURVE(5,(#45879,#45880,#45881,#45882,#45883,#45884,#45885,#45886,
#45887,#45888,#45889,#45890,#45891,#45892,#45893,#45894,#45895,#45896,#45897,
#45898,#45899,#45900,#45901,#45902,#45903,#45904,#45905,#45906,#45907,#45908,
#45909,#45910,#45911,#45912,#45913,#45914,#45915,#45916,#45917,#45918,#45919,
#45920,#45921,#45922,#45923,#45924,#45925,#45926,#45927,#45928,#45929,#45930,
#45931,#45932,#45933,#45934,#45935,#45936,#45937,#45938,#45939,#45940,#45941,
#45942,#45943,#45944,#45945,#45946,#45947,#45948),.UNSPECIFIED.,.F.,.F.)
B_SPLINE_CURVE_WITH_KNOTS((6,1,1,1,1,1,1,1,1,1,1,1,1,1,1,1,1,1,1,1,1,1,
1,1,1,1,1,1,1,1,1,1,1,1,1,1,1,1,1,1,1,1,1,1,1,1,1,1,1,1,1,1,1,1,1,1,1,1,
1,1,1,1,1,1,1,6),(-0.994228156739702,-0.984615384615383,-0.969230769230768,
-0.953846153846152,-0.938461538461537,-0.923076923076922,-0.907692307692306,
-0.892307692307691,-0.876923076923076,-0.86153846153846,-0.846153846153845,
-0.83076923076923,-0.815384615384614,-0.799999999999999,-0.784615384615384,
-0.769230769230768,-0.753846153846153,-0.738461538461538,-0.723076923076922,
-0.707692307692307,-0.692307692307692,-0.676923076923076,-0.661538461538461,
-0.646153846153846,-0.63076923076923,-0.615384615384615,-0.6,-0.584615384615384,
-0.569230769230769,-0.553846153846154,-0.538461538461538,-0.523076923076923,
-0.507692307692308,-0.492307692307692,-0.476923076923077,-0.461538461538462,
-0.446153846153846,-0.430769230769231,-0.415384615384615,-0.4,-0.384615384615385,
-0.369230769230769,-0.353846153846154,-0.338461538461538,-0.323076923076923,
-0.307692307692308,-0.292307692307692,-0.276923076923077,-0.261538461538462,
-0.246153846153846,-0.230769230769231,-0.215384615384615,-0.2,-0.184615384615385,
-0.169230769230769,-0.153846153846154,-0.138461538461538,-0.123076923076923,
-0.107692307692308,-0.0923076923076923,-0.0769230769230769,-0.0615384615384615,
-0.0461538461538462,-0.0307692307692308,-0.0153846153846154,0.),
 .UNSPECIFIED.)
CURVE()
GEOMETRIC_REPRESENTATION_ITEM()
RATIONAL_B_SPLINE_CURVE((1.,1.,1.,1.,1.,1.,1.,1.,1.,1.,1.,1.,1.,1.,1.,1.,
1.,1.,1.,1.,1.,1.,1.,1.,1.,1.,1.,1.,1.,1.,1.,1.,1.,1.,1.,1.,1.,1.,1.,1.,
1.,1.,1.,1.,1.,1.,1.,1.,1.,1.,1.,1.,1.,1.,1.,1.,1.,1.,1.,1.,1.,1.,1.,1.,
1.,1.,1.,1.,1.,1.))
REPRESENTATION_ITEM('')
);
#297=(
BOUNDED_CURVE()
B_SPLINE_CURVE(5,(#46101,#46102,#46103,#46104,#46105,#46106,#46107,#46108,
#46109,#46110,#46111,#46112,#46113,#46114,#46115,#46116,#46117,#46118,#46119,
#46120,#46121,#46122,#46123,#46124,#46125,#46126,#46127,#46128,#46129,#46130,
#46131,#46132,#46133,#46134,#46135,#46136,#46137,#46138,#46139,#46140,#46141,
#46142,#46143,#46144,#46145,#46146,#46147,#46148,#46149,#46150,#46151,#46152,
#46153,#46154,#46155,#46156,#46157,#46158,#46159,#46160,#46161,#46162,#46163,
#46164,#46165,#46166,#46167,#46168,#46169,#46170),.UNSPECIFIED.,.F.,.F.)
B_SPLINE_CURVE_WITH_KNOTS((6,1,1,1,1,1,1,1,1,1,1,1,1,1,1,1,1,1,1,1,1,1,
1,1,1,1,1,1,1,1,1,1,1,1,1,1,1,1,1,1,1,1,1,1,1,1,1,1,1,1,1,1,1,1,1,1,1,1,
1,1,1,1,1,1,1,6),(-1.,-0.984615384615383,-0.969230769230768,-0.953846153846152,
-0.938461538461537,-0.923076923076922,-0.907692307692306,-0.892307692307691,
-0.876923076923076,-0.86153846153846,-0.846153846153845,-0.83076923076923,
-0.815384615384614,-0.799999999999999,-0.784615384615384,-0.769230769230768,
-0.753846153846153,-0.738461538461538,-0.723076923076922,-0.707692307692307,
-0.692307692307692,-0.676923076923076,-0.661538461538461,-0.646153846153846,
-0.63076923076923,-0.615384615384615,-0.6,-0.584615384615384,-0.569230769230769,
-0.553846153846154,-0.538461538461538,-0.523076923076923,-0.507692307692308,
-0.492307692307692,-0.476923076923077,-0.461538461538462,-0.446153846153846,
-0.430769230769231,-0.415384615384615,-0.4,-0.384615384615385,-0.369230769230769,
-0.353846153846154,-0.338461538461538,-0.323076923076923,-0.307692307692308,
-0.292307692307692,-0.276923076923077,-0.261538461538462,-0.246153846153846,
-0.230769230769231,-0.215384615384615,-0.2,-0.184615384615385,-0.169230769230769,
-0.153846153846154,-0.138461538461538,-0.123076923076923,-0.107692307692308,
-0.0923076923076923,-0.0769230769230769,-0.0615384615384615,-0.0461538461538462,
-0.0307692307692308,-0.0153846153846154,-0.00577184337450989),
 .UNSPECIFIED.)
CURVE()
GEOMETRIC_REPRESENTATION_ITEM()
RATIONAL_B_SPLINE_CURVE((1.,1.,1.,1.,1.,1.,1.,1.,1.,1.,1.,1.,1.,1.,1.,1.,
1.,1.,1.,1.,1.,1.,1.,1.,1.,1.,1.,1.,1.,1.,1.,1.,1.,1.,1.,1.,1.,1.,1.,1.,
1.,1.,1.,1.,1.,1.,1.,1.,1.,1.,1.,1.,1.,1.,1.,1.,1.,1.,1.,1.,1.,1.,1.,1.,
1.,1.,1.,1.,1.,1.))
REPRESENTATION_ITEM('')
);
#298=(
BOUNDED_CURVE()
B_SPLINE_CURVE(5,(#46321,#46322,#46323,#46324,#46325,#46326,#46327,#46328,
#46329,#46330,#46331,#46332,#46333,#46334,#46335,#46336,#46337,#46338,#46339,
#46340,#46341,#46342,#46343,#46344,#46345,#46346,#46347,#46348,#46349,#46350,
#46351,#46352,#46353,#46354,#46355,#46356,#46357,#46358,#46359,#46360,#46361,
#46362,#46363,#46364,#46365,#46366,#46367,#46368,#46369,#46370,#46371,#46372,
#46373,#46374,#46375,#46376,#46377,#46378,#46379,#46380,#46381,#46382,#46383,
#46384,#46385,#46386,#46387,#46388,#46389,#46390),.UNSPECIFIED.,.F.,.F.)
B_SPLINE_CURVE_WITH_KNOTS((6,1,1,1,1,1,1,1,1,1,1,1,1,1,1,1,1,1,1,1,1,1,
1,1,1,1,1,1,1,1,1,1,1,1,1,1,1,1,1,1,1,1,1,1,1,1,1,1,1,1,1,1,1,1,1,1,1,1,
1,1,1,1,1,1,1,6),(-0.994228156739736,-0.984615384615383,-0.969230769230768,
-0.953846153846152,-0.938461538461537,-0.923076923076922,-0.907692307692306,
-0.892307692307691,-0.876923076923076,-0.86153846153846,-0.846153846153845,
-0.83076923076923,-0.815384615384614,-0.799999999999999,-0.784615384615384,
-0.769230769230768,-0.753846153846153,-0.738461538461538,-0.723076923076922,
-0.707692307692307,-0.692307692307692,-0.676923076923076,-0.661538461538461,
-0.646153846153846,-0.63076923076923,-0.615384615384615,-0.6,-0.584615384615384,
-0.569230769230769,-0.553846153846154,-0.538461538461538,-0.523076923076923,
-0.507692307692308,-0.492307692307692,-0.476923076923077,-0.461538461538462,
-0.446153846153846,-0.430769230769231,-0.415384615384615,-0.4,-0.384615384615385,
-0.369230769230769,-0.353846153846154,-0.338461538461538,-0.323076923076923,
-0.307692307692308,-0.292307692307692,-0.276923076923077,-0.261538461538462,
-0.246153846153846,-0.230769230769231,-0.215384615384615,-0.2,-0.184615384615385,
-0.169230769230769,-0.153846153846154,-0.138461538461538,-0.123076923076923,
-0.107692307692308,-0.0923076923076923,-0.0769230769230769,-0.0615384615384615,
-0.0461538461538462,-0.0307692307692308,-0.0153846153846154,0.),
 .UNSPECIFIED.)
CURVE()
GEOMETRIC_REPRESENTATION_ITEM()
RATIONAL_B_SPLINE_CURVE((1.,1.,1.,1.,1.,1.,1.,1.,1.,1.,1.,1.,1.,1.,1.,1.,
1.,1.,1.,1.,1.,1.,1.,1.,1.,1.,1.,1.,1.,1.,1.,1.,1.,1.,1.,1.,1.,1.,1.,1.,
1.,1.,1.,1.,1.,1.,1.,1.,1.,1.,1.,1.,1.,1.,1.,1.,1.,1.,1.,1.,1.,1.,1.,1.,
1.,1.,1.,1.,1.,1.))
REPRESENTATION_ITEM('')
);
#299=(
BOUNDED_CURVE()
B_SPLINE_CURVE(5,(#46543,#46544,#46545,#46546,#46547,#46548,#46549,#46550,
#46551,#46552,#46553,#46554,#46555,#46556,#46557,#46558,#46559,#46560,#46561,
#46562,#46563,#46564,#46565,#46566,#46567,#46568,#46569,#46570,#46571,#46572,
#46573,#46574,#46575,#46576,#46577,#46578,#46579,#46580,#46581,#46582,#46583,
#46584,#46585,#46586,#46587,#46588,#46589,#46590,#46591,#46592,#46593,#46594,
#46595,#46596,#46597,#46598,#46599,#46600,#46601,#46602,#46603,#46604,#46605,
#46606,#46607,#46608,#46609,#46610,#46611,#46612),.UNSPECIFIED.,.F.,.F.)
B_SPLINE_CURVE_WITH_KNOTS((6,1,1,1,1,1,1,1,1,1,1,1,1,1,1,1,1,1,1,1,1,1,
1,1,1,1,1,1,1,1,1,1,1,1,1,1,1,1,1,1,1,1,1,1,1,1,1,1,1,1,1,1,1,1,1,1,1,1,
1,1,1,1,1,1,1,6),(-1.,-0.984615384615383,-0.969230769230768,-0.953846153846152,
-0.938461538461537,-0.923076923076922,-0.907692307692306,-0.892307692307691,
-0.876923076923076,-0.86153846153846,-0.846153846153845,-0.83076923076923,
-0.815384615384614,-0.799999999999999,-0.784615384615384,-0.769230769230768,
-0.753846153846153,-0.738461538461538,-0.723076923076922,-0.707692307692307,
-0.692307692307692,-0.676923076923076,-0.661538461538461,-0.646153846153846,
-0.63076923076923,-0.615384615384615,-0.6,-0.584615384615384,-0.569230769230769,
-0.553846153846154,-0.538461538461538,-0.523076923076923,-0.507692307692308,
-0.492307692307692,-0.476923076923077,-0.461538461538462,-0.446153846153846,
-0.430769230769231,-0.415384615384615,-0.4,-0.384615384615385,-0.369230769230769,
-0.353846153846154,-0.338461538461538,-0.323076923076923,-0.307692307692308,
-0.292307692307692,-0.276923076923077,-0.261538461538462,-0.246153846153846,
-0.230769230769231,-0.215384615384615,-0.2,-0.184615384615385,-0.169230769230769,
-0.153846153846154,-0.138461538461538,-0.123076923076923,-0.107692307692308,
-0.0923076923076923,-0.0769230769230769,-0.0615384615384615,-0.0461538461538462,
-0.0307692307692308,-0.0153846153846154,-0.00577184337452469),
 .UNSPECIFIED.)
CURVE()
GEOMETRIC_REPRESENTATION_ITEM()
RATIONAL_B_SPLINE_CURVE((1.,1.,1.,1.,1.,1.,1.,1.,1.,1.,1.,1.,1.,1.,1.,1.,
1.,1.,1.,1.,1.,1.,1.,1.,1.,1.,1.,1.,1.,1.,1.,1.,1.,1.,1.,1.,1.,1.,1.,1.,
1.,1.,1.,1.,1.,1.,1.,1.,1.,1.,1.,1.,1.,1.,1.,1.,1.,1.,1.,1.,1.,1.,1.,1.,
1.,1.,1.,1.,1.,1.))
REPRESENTATION_ITEM('')
);
#300=(
BOUNDED_CURVE()
B_SPLINE_CURVE(5,(#46763,#46764,#46765,#46766,#46767,#46768,#46769,#46770,
#46771,#46772,#46773,#46774,#46775,#46776,#46777,#46778,#46779,#46780,#46781,
#46782,#46783,#46784,#46785,#46786,#46787,#46788,#46789,#46790,#46791,#46792,
#46793,#46794,#46795,#46796,#46797,#46798,#46799,#46800,#46801,#46802,#46803,
#46804,#46805,#46806,#46807,#46808,#46809,#46810,#46811,#46812,#46813,#46814,
#46815,#46816,#46817,#46818,#46819,#46820,#46821,#46822,#46823,#46824,#46825,
#46826,#46827,#46828,#46829,#46830,#46831,#46832),.UNSPECIFIED.,.F.,.F.)
B_SPLINE_CURVE_WITH_KNOTS((6,1,1,1,1,1,1,1,1,1,1,1,1,1,1,1,1,1,1,1,1,1,
1,1,1,1,1,1,1,1,1,1,1,1,1,1,1,1,1,1,1,1,1,1,1,1,1,1,1,1,1,1,1,1,1,1,1,1,
1,1,1,1,1,1,1,6),(-0.994228156739717,-0.984615384615383,-0.969230769230768,
-0.953846153846152,-0.938461538461537,-0.923076923076922,-0.907692307692306,
-0.892307692307691,-0.876923076923076,-0.86153846153846,-0.846153846153845,
-0.83076923076923,-0.815384615384614,-0.799999999999999,-0.784615384615384,
-0.769230769230768,-0.753846153846153,-0.738461538461538,-0.723076923076922,
-0.707692307692307,-0.692307692307692,-0.676923076923076,-0.661538461538461,
-0.646153846153846,-0.63076923076923,-0.615384615384615,-0.6,-0.584615384615384,
-0.569230769230769,-0.553846153846154,-0.538461538461538,-0.523076923076923,
-0.507692307692308,-0.492307692307692,-0.476923076923077,-0.461538461538462,
-0.446153846153846,-0.430769230769231,-0.415384615384615,-0.4,-0.384615384615385,
-0.369230769230769,-0.353846153846154,-0.338461538461538,-0.323076923076923,
-0.307692307692308,-0.292307692307692,-0.276923076923077,-0.261538461538462,
-0.246153846153846,-0.230769230769231,-0.215384615384615,-0.2,-0.184615384615385,
-0.169230769230769,-0.153846153846154,-0.138461538461538,-0.123076923076923,
-0.107692307692308,-0.0923076923076923,-0.0769230769230769,-0.0615384615384615,
-0.0461538461538462,-0.0307692307692308,-0.0153846153846154,0.),
 .UNSPECIFIED.)
CURVE()
GEOMETRIC_REPRESENTATION_ITEM()
RATIONAL_B_SPLINE_CURVE((1.,1.,1.,1.,1.,1.,1.,1.,1.,1.,1.,1.,1.,1.,1.,1.,
1.,1.,1.,1.,1.,1.,1.,1.,1.,1.,1.,1.,1.,1.,1.,1.,1.,1.,1.,1.,1.,1.,1.,1.,
1.,1.,1.,1.,1.,1.,1.,1.,1.,1.,1.,1.,1.,1.,1.,1.,1.,1.,1.,1.,1.,1.,1.,1.,
1.,1.,1.,1.,1.,1.))
REPRESENTATION_ITEM('')
);
#301=(
BOUNDED_CURVE()
B_SPLINE_CURVE(5,(#46985,#46986,#46987,#46988,#46989,#46990,#46991,#46992,
#46993,#46994,#46995,#46996,#46997,#46998,#46999,#47000,#47001,#47002,#47003,
#47004,#47005,#47006,#47007,#47008,#47009,#47010,#47011,#47012,#47013,#47014,
#47015,#47016,#47017,#47018,#47019,#47020,#47021,#47022,#47023,#47024,#47025,
#47026,#47027,#47028,#47029,#47030,#47031,#47032,#47033,#47034,#47035,#47036,
#47037,#47038,#47039,#47040,#47041,#47042,#47043,#47044,#47045,#47046,#47047,
#47048,#47049,#47050,#47051,#47052,#47053,#47054),.UNSPECIFIED.,.F.,.F.)
B_SPLINE_CURVE_WITH_KNOTS((6,1,1,1,1,1,1,1,1,1,1,1,1,1,1,1,1,1,1,1,1,1,
1,1,1,1,1,1,1,1,1,1,1,1,1,1,1,1,1,1,1,1,1,1,1,1,1,1,1,1,1,1,1,1,1,1,1,1,
1,1,1,1,1,1,1,6),(-1.,-0.984615384615383,-0.969230769230768,-0.953846153846152,
-0.938461538461537,-0.923076923076922,-0.907692307692306,-0.892307692307691,
-0.876923076923076,-0.86153846153846,-0.846153846153845,-0.83076923076923,
-0.815384615384614,-0.799999999999999,-0.784615384615384,-0.769230769230768,
-0.753846153846153,-0.738461538461538,-0.723076923076922,-0.707692307692307,
-0.692307692307692,-0.676923076923076,-0.661538461538461,-0.646153846153846,
-0.63076923076923,-0.615384615384615,-0.6,-0.584615384615384,-0.569230769230769,
-0.553846153846154,-0.538461538461538,-0.523076923076923,-0.507692307692308,
-0.492307692307692,-0.476923076923077,-0.461538461538462,-0.446153846153846,
-0.430769230769231,-0.415384615384615,-0.4,-0.384615384615385,-0.369230769230769,
-0.353846153846154,-0.338461538461538,-0.323076923076923,-0.307692307692308,
-0.292307692307692,-0.276923076923077,-0.261538461538462,-0.246153846153846,
-0.230769230769231,-0.215384615384615,-0.2,-0.184615384615385,-0.169230769230769,
-0.153846153846154,-0.138461538461538,-0.123076923076923,-0.107692307692308,
-0.0923076923076923,-0.0769230769230769,-0.0615384615384615,-0.0461538461538462,
-0.0307692307692308,-0.0153846153846154,-0.00577184337453472),
 .UNSPECIFIED.)
CURVE()
GEOMETRIC_REPRESENTATION_ITEM()
RATIONAL_B_SPLINE_CURVE((1.,1.,1.,1.,1.,1.,1.,1.,1.,1.,1.,1.,1.,1.,1.,1.,
1.,1.,1.,1.,1.,1.,1.,1.,1.,1.,1.,1.,1.,1.,1.,1.,1.,1.,1.,1.,1.,1.,1.,1.,
1.,1.,1.,1.,1.,1.,1.,1.,1.,1.,1.,1.,1.,1.,1.,1.,1.,1.,1.,1.,1.,1.,1.,1.,
1.,1.,1.,1.,1.,1.))
REPRESENTATION_ITEM('')
);
#302=(
BOUNDED_CURVE()
B_SPLINE_CURVE(5,(#47205,#47206,#47207,#47208,#47209,#47210,#47211,#47212,
#47213,#47214,#47215,#47216,#47217,#47218,#47219,#47220,#47221,#47222,#47223,
#47224,#47225,#47226,#47227,#47228,#47229,#47230,#47231,#47232,#47233,#47234,
#47235,#47236,#47237,#47238,#47239,#47240,#47241,#47242,#47243,#47244,#47245,
#47246,#47247,#47248,#47249,#47250,#47251,#47252,#47253,#47254,#47255,#47256,
#47257,#47258,#47259,#47260,#47261,#47262,#47263,#47264,#47265,#47266,#47267,
#47268,#47269,#47270,#47271,#47272,#47273,#47274),.UNSPECIFIED.,.F.,.F.)
B_SPLINE_CURVE_WITH_KNOTS((6,1,1,1,1,1,1,1,1,1,1,1,1,1,1,1,1,1,1,1,1,1,
1,1,1,1,1,1,1,1,1,1,1,1,1,1,1,1,1,1,1,1,1,1,1,1,1,1,1,1,1,1,1,1,1,1,1,1,
1,1,1,1,1,1,1,6),(-0.994228156739652,-0.984615384615383,-0.969230769230768,
-0.953846153846152,-0.938461538461537,-0.923076923076922,-0.907692307692306,
-0.892307692307691,-0.876923076923076,-0.86153846153846,-0.846153846153845,
-0.83076923076923,-0.815384615384614,-0.799999999999999,-0.784615384615384,
-0.769230769230768,-0.753846153846153,-0.738461538461538,-0.723076923076922,
-0.707692307692307,-0.692307692307692,-0.676923076923076,-0.661538461538461,
-0.646153846153846,-0.63076923076923,-0.615384615384615,-0.6,-0.584615384615384,
-0.569230769230769,-0.553846153846154,-0.538461538461538,-0.523076923076923,
-0.507692307692308,-0.492307692307692,-0.476923076923077,-0.461538461538462,
-0.446153846153846,-0.430769230769231,-0.415384615384615,-0.4,-0.384615384615385,
-0.369230769230769,-0.353846153846154,-0.338461538461538,-0.323076923076923,
-0.307692307692308,-0.292307692307692,-0.276923076923077,-0.261538461538462,
-0.246153846153846,-0.230769230769231,-0.215384615384615,-0.2,-0.184615384615385,
-0.169230769230769,-0.153846153846154,-0.138461538461538,-0.123076923076923,
-0.107692307692308,-0.0923076923076923,-0.0769230769230769,-0.0615384615384615,
-0.0461538461538462,-0.0307692307692308,-0.0153846153846154,0.),
 .UNSPECIFIED.)
CURVE()
GEOMETRIC_REPRESENTATION_ITEM()
RATIONAL_B_SPLINE_CURVE((1.,1.,1.,1.,1.,1.,1.,1.,1.,1.,1.,1.,1.,1.,1.,1.,
1.,1.,1.,1.,1.,1.,1.,1.,1.,1.,1.,1.,1.,1.,1.,1.,1.,1.,1.,1.,1.,1.,1.,1.,
1.,1.,1.,1.,1.,1.,1.,1.,1.,1.,1.,1.,1.,1.,1.,1.,1.,1.,1.,1.,1.,1.,1.,1.,
1.,1.,1.,1.,1.,1.))
REPRESENTATION_ITEM('')
);
#303=(
BOUNDED_CURVE()
B_SPLINE_CURVE(5,(#47427,#47428,#47429,#47430,#47431,#47432,#47433,#47434,
#47435,#47436,#47437,#47438,#47439,#47440,#47441,#47442,#47443,#47444,#47445,
#47446,#47447,#47448,#47449,#47450,#47451,#47452,#47453,#47454,#47455,#47456,
#47457,#47458,#47459,#47460,#47461,#47462,#47463,#47464,#47465,#47466,#47467,
#47468,#47469,#47470,#47471,#47472,#47473,#47474,#47475,#47476,#47477,#47478,
#47479,#47480,#47481,#47482,#47483,#47484,#47485,#47486,#47487,#47488,#47489,
#47490,#47491,#47492,#47493,#47494,#47495,#47496),.UNSPECIFIED.,.F.,.F.)
B_SPLINE_CURVE_WITH_KNOTS((6,1,1,1,1,1,1,1,1,1,1,1,1,1,1,1,1,1,1,1,1,1,
1,1,1,1,1,1,1,1,1,1,1,1,1,1,1,1,1,1,1,1,1,1,1,1,1,1,1,1,1,1,1,1,1,1,1,1,
1,1,1,1,1,1,1,6),(-1.,-0.984615384615383,-0.969230769230768,-0.953846153846152,
-0.938461538461537,-0.923076923076922,-0.907692307692306,-0.892307692307691,
-0.876923076923076,-0.86153846153846,-0.846153846153845,-0.83076923076923,
-0.815384615384614,-0.799999999999999,-0.784615384615384,-0.769230769230768,
-0.753846153846153,-0.738461538461538,-0.723076923076922,-0.707692307692307,
-0.692307692307692,-0.676923076923076,-0.661538461538461,-0.646153846153846,
-0.63076923076923,-0.615384615384615,-0.6,-0.584615384615384,-0.569230769230769,
-0.553846153846154,-0.538461538461538,-0.523076923076923,-0.507692307692308,
-0.492307692307692,-0.476923076923077,-0.461538461538462,-0.446153846153846,
-0.430769230769231,-0.415384615384615,-0.4,-0.384615384615385,-0.369230769230769,
-0.353846153846154,-0.338461538461538,-0.323076923076923,-0.307692307692308,
-0.292307692307692,-0.276923076923077,-0.261538461538462,-0.246153846153846,
-0.230769230769231,-0.215384615384615,-0.2,-0.184615384615385,-0.169230769230769,
-0.153846153846154,-0.138461538461538,-0.123076923076923,-0.107692307692308,
-0.0923076923076923,-0.0769230769230769,-0.0615384615384615,-0.0461538461538462,
-0.0307692307692308,-0.0153846153846154,-0.00577184337450876),
 .UNSPECIFIED.)
CURVE()
GEOMETRIC_REPRESENTATION_ITEM()
RATIONAL_B_SPLINE_CURVE((1.,1.,1.,1.,1.,1.,1.,1.,1.,1.,1.,1.,1.,1.,1.,1.,
1.,1.,1.,1.,1.,1.,1.,1.,1.,1.,1.,1.,1.,1.,1.,1.,1.,1.,1.,1.,1.,1.,1.,1.,
1.,1.,1.,1.,1.,1.,1.,1.,1.,1.,1.,1.,1.,1.,1.,1.,1.,1.,1.,1.,1.,1.,1.,1.,
1.,1.,1.,1.,1.,1.))
REPRESENTATION_ITEM('')
);
#304=(
BOUNDED_CURVE()
B_SPLINE_CURVE(5,(#47647,#47648,#47649,#47650,#47651,#47652,#47653,#47654,
#47655,#47656,#47657,#47658,#47659,#47660,#47661,#47662,#47663,#47664,#47665,
#47666,#47667,#47668,#47669,#47670,#47671,#47672,#47673,#47674,#47675,#47676,
#47677,#47678,#47679,#47680,#47681,#47682,#47683,#47684,#47685,#47686,#47687,
#47688,#47689,#47690,#47691,#47692,#47693,#47694,#47695,#47696,#47697,#47698,
#47699,#47700,#47701,#47702,#47703,#47704,#47705,#47706,#47707,#47708,#47709,
#47710,#47711,#47712,#47713,#47714,#47715,#47716),.UNSPECIFIED.,.F.,.F.)
B_SPLINE_CURVE_WITH_KNOTS((6,1,1,1,1,1,1,1,1,1,1,1,1,1,1,1,1,1,1,1,1,1,
1,1,1,1,1,1,1,1,1,1,1,1,1,1,1,1,1,1,1,1,1,1,1,1,1,1,1,1,1,1,1,1,1,1,1,1,
1,1,1,1,1,1,1,6),(-0.994228156739683,-0.984615384615383,-0.969230769230768,
-0.953846153846152,-0.938461538461537,-0.923076923076922,-0.907692307692306,
-0.892307692307691,-0.876923076923076,-0.86153846153846,-0.846153846153845,
-0.83076923076923,-0.815384615384614,-0.799999999999999,-0.784615384615384,
-0.769230769230768,-0.753846153846153,-0.738461538461538,-0.723076923076922,
-0.707692307692307,-0.692307692307692,-0.676923076923076,-0.661538461538461,
-0.646153846153846,-0.63076923076923,-0.615384615384615,-0.6,-0.584615384615384,
-0.569230769230769,-0.553846153846154,-0.538461538461538,-0.523076923076923,
-0.507692307692308,-0.492307692307692,-0.476923076923077,-0.461538461538462,
-0.446153846153846,-0.430769230769231,-0.415384615384615,-0.4,-0.384615384615385,
-0.369230769230769,-0.353846153846154,-0.338461538461538,-0.323076923076923,
-0.307692307692308,-0.292307692307692,-0.276923076923077,-0.261538461538462,
-0.246153846153846,-0.230769230769231,-0.215384615384615,-0.2,-0.184615384615385,
-0.169230769230769,-0.153846153846154,-0.138461538461538,-0.123076923076923,
-0.107692307692308,-0.0923076923076923,-0.0769230769230769,-0.0615384615384615,
-0.0461538461538462,-0.0307692307692308,-0.0153846153846154,0.),
 .UNSPECIFIED.)
CURVE()
GEOMETRIC_REPRESENTATION_ITEM()
RATIONAL_B_SPLINE_CURVE((1.,1.,1.,1.,1.,1.,1.,1.,1.,1.,1.,1.,1.,1.,1.,1.,
1.,1.,1.,1.,1.,1.,1.,1.,1.,1.,1.,1.,1.,1.,1.,1.,1.,1.,1.,1.,1.,1.,1.,1.,
1.,1.,1.,1.,1.,1.,1.,1.,1.,1.,1.,1.,1.,1.,1.,1.,1.,1.,1.,1.,1.,1.,1.,1.,
1.,1.,1.,1.,1.,1.))
REPRESENTATION_ITEM('')
);
#305=(
BOUNDED_CURVE()
B_SPLINE_CURVE(5,(#47869,#47870,#47871,#47872,#47873,#47874,#47875,#47876,
#47877,#47878,#47879,#47880,#47881,#47882,#47883,#47884,#47885,#47886,#47887,
#47888,#47889,#47890,#47891,#47892,#47893,#47894,#47895,#47896,#47897,#47898,
#47899,#47900,#47901,#47902,#47903,#47904,#47905,#47906,#47907,#47908,#47909,
#47910,#47911,#47912,#47913,#47914,#47915,#47916,#47917,#47918,#47919,#47920,
#47921,#47922,#47923,#47924,#47925,#47926,#47927,#47928,#47929,#47930,#47931,
#47932,#47933,#47934,#47935,#47936,#47937,#47938),.UNSPECIFIED.,.F.,.F.)
B_SPLINE_CURVE_WITH_KNOTS((6,1,1,1,1,1,1,1,1,1,1,1,1,1,1,1,1,1,1,1,1,1,
1,1,1,1,1,1,1,1,1,1,1,1,1,1,1,1,1,1,1,1,1,1,1,1,1,1,1,1,1,1,1,1,1,1,1,1,
1,1,1,1,1,1,1,6),(-1.,-0.984615384615383,-0.969230769230768,-0.953846153846152,
-0.938461538461537,-0.923076923076922,-0.907692307692306,-0.892307692307691,
-0.876923076923076,-0.86153846153846,-0.846153846153845,-0.83076923076923,
-0.815384615384614,-0.799999999999999,-0.784615384615384,-0.769230769230768,
-0.753846153846153,-0.738461538461538,-0.723076923076922,-0.707692307692307,
-0.692307692307692,-0.676923076923076,-0.661538461538461,-0.646153846153846,
-0.63076923076923,-0.615384615384615,-0.6,-0.584615384615384,-0.569230769230769,
-0.553846153846154,-0.538461538461538,-0.523076923076923,-0.507692307692308,
-0.492307692307692,-0.476923076923077,-0.461538461538462,-0.446153846153846,
-0.430769230769231,-0.415384615384615,-0.4,-0.384615384615385,-0.369230769230769,
-0.353846153846154,-0.338461538461538,-0.323076923076923,-0.307692307692308,
-0.292307692307692,-0.276923076923077,-0.261538461538462,-0.246153846153846,
-0.230769230769231,-0.215384615384615,-0.2,-0.184615384615385,-0.169230769230769,
-0.153846153846154,-0.138461538461538,-0.123076923076923,-0.107692307692308,
-0.0923076923076923,-0.0769230769230769,-0.0615384615384615,-0.0461538461538462,
-0.0307692307692308,-0.0153846153846154,-0.00577184337450277),
 .UNSPECIFIED.)
CURVE()
GEOMETRIC_REPRESENTATION_ITEM()
RATIONAL_B_SPLINE_CURVE((1.,1.,1.,1.,1.,1.,1.,1.,1.,1.,1.,1.,1.,1.,1.,1.,
1.,1.,1.,1.,1.,1.,1.,1.,1.,1.,1.,1.,1.,1.,1.,1.,1.,1.,1.,1.,1.,1.,1.,1.,
1.,1.,1.,1.,1.,1.,1.,1.,1.,1.,1.,1.,1.,1.,1.,1.,1.,1.,1.,1.,1.,1.,1.,1.,
1.,1.,1.,1.,1.,1.))
REPRESENTATION_ITEM('')
);
#306=(
BOUNDED_CURVE()
B_SPLINE_CURVE(5,(#48089,#48090,#48091,#48092,#48093,#48094,#48095,#48096,
#48097,#48098,#48099,#48100,#48101,#48102,#48103,#48104,#48105,#48106,#48107,
#48108,#48109,#48110,#48111,#48112,#48113,#48114,#48115,#48116,#48117,#48118,
#48119,#48120,#48121,#48122,#48123,#48124,#48125,#48126,#48127,#48128,#48129,
#48130,#48131,#48132,#48133,#48134,#48135,#48136,#48137,#48138,#48139,#48140,
#48141,#48142,#48143,#48144,#48145,#48146,#48147,#48148,#48149,#48150,#48151,
#48152,#48153,#48154,#48155,#48156,#48157,#48158),.UNSPECIFIED.,.F.,.F.)
B_SPLINE_CURVE_WITH_KNOTS((6,1,1,1,1,1,1,1,1,1,1,1,1,1,1,1,1,1,1,1,1,1,
1,1,1,1,1,1,1,1,1,1,1,1,1,1,1,1,1,1,1,1,1,1,1,1,1,1,1,1,1,1,1,1,1,1,1,1,
1,1,1,1,1,1,1,6),(-0.994228156739689,-0.984615384615383,-0.969230769230768,
-0.953846153846152,-0.938461538461537,-0.923076923076922,-0.907692307692306,
-0.892307692307691,-0.876923076923076,-0.86153846153846,-0.846153846153845,
-0.83076923076923,-0.815384615384614,-0.799999999999999,-0.784615384615384,
-0.769230769230768,-0.753846153846153,-0.738461538461538,-0.723076923076922,
-0.707692307692307,-0.692307692307692,-0.676923076923076,-0.661538461538461,
-0.646153846153846,-0.63076923076923,-0.615384615384615,-0.6,-0.584615384615384,
-0.569230769230769,-0.553846153846154,-0.538461538461538,-0.523076923076923,
-0.507692307692308,-0.492307692307692,-0.476923076923077,-0.461538461538462,
-0.446153846153846,-0.430769230769231,-0.415384615384615,-0.4,-0.384615384615385,
-0.369230769230769,-0.353846153846154,-0.338461538461538,-0.323076923076923,
-0.307692307692308,-0.292307692307692,-0.276923076923077,-0.261538461538462,
-0.246153846153846,-0.230769230769231,-0.215384615384615,-0.2,-0.184615384615385,
-0.169230769230769,-0.153846153846154,-0.138461538461538,-0.123076923076923,
-0.107692307692308,-0.0923076923076923,-0.0769230769230769,-0.0615384615384615,
-0.0461538461538462,-0.0307692307692308,-0.0153846153846154,0.),
 .UNSPECIFIED.)
CURVE()
GEOMETRIC_REPRESENTATION_ITEM()
RATIONAL_B_SPLINE_CURVE((1.,1.,1.,1.,1.,1.,1.,1.,1.,1.,1.,1.,1.,1.,1.,1.,
1.,1.,1.,1.,1.,1.,1.,1.,1.,1.,1.,1.,1.,1.,1.,1.,1.,1.,1.,1.,1.,1.,1.,1.,
1.,1.,1.,1.,1.,1.,1.,1.,1.,1.,1.,1.,1.,1.,1.,1.,1.,1.,1.,1.,1.,1.,1.,1.,
1.,1.,1.,1.,1.,1.))
REPRESENTATION_ITEM('')
);
#307=(
BOUNDED_CURVE()
B_SPLINE_CURVE(5,(#48311,#48312,#48313,#48314,#48315,#48316,#48317,#48318,
#48319,#48320,#48321,#48322,#48323,#48324,#48325,#48326,#48327,#48328,#48329,
#48330,#48331,#48332,#48333,#48334,#48335,#48336,#48337,#48338,#48339,#48340,
#48341,#48342,#48343,#48344,#48345,#48346,#48347,#48348,#48349,#48350,#48351,
#48352,#48353,#48354,#48355,#48356,#48357,#48358,#48359,#48360,#48361,#48362,
#48363,#48364,#48365,#48366,#48367,#48368,#48369,#48370,#48371,#48372,#48373,
#48374,#48375,#48376,#48377,#48378,#48379,#48380),.UNSPECIFIED.,.F.,.F.)
B_SPLINE_CURVE_WITH_KNOTS((6,1,1,1,1,1,1,1,1,1,1,1,1,1,1,1,1,1,1,1,1,1,
1,1,1,1,1,1,1,1,1,1,1,1,1,1,1,1,1,1,1,1,1,1,1,1,1,1,1,1,1,1,1,1,1,1,1,1,
1,1,1,1,1,1,1,6),(-1.,-0.984615384615383,-0.969230769230768,-0.953846153846152,
-0.938461538461537,-0.923076923076922,-0.907692307692306,-0.892307692307691,
-0.876923076923076,-0.86153846153846,-0.846153846153845,-0.83076923076923,
-0.815384615384614,-0.799999999999999,-0.784615384615384,-0.769230769230768,
-0.753846153846153,-0.738461538461538,-0.723076923076922,-0.707692307692307,
-0.692307692307692,-0.676923076923076,-0.661538461538461,-0.646153846153846,
-0.63076923076923,-0.615384615384615,-0.6,-0.584615384615384,-0.569230769230769,
-0.553846153846154,-0.538461538461538,-0.523076923076923,-0.507692307692308,
-0.492307692307692,-0.476923076923077,-0.461538461538462,-0.446153846153846,
-0.430769230769231,-0.415384615384615,-0.4,-0.384615384615385,-0.369230769230769,
-0.353846153846154,-0.338461538461538,-0.323076923076923,-0.307692307692308,
-0.292307692307692,-0.276923076923077,-0.261538461538462,-0.246153846153846,
-0.230769230769231,-0.215384615384615,-0.2,-0.184615384615385,-0.169230769230769,
-0.153846153846154,-0.138461538461538,-0.123076923076923,-0.107692307692308,
-0.0923076923076923,-0.0769230769230769,-0.0615384615384615,-0.0461538461538462,
-0.0307692307692308,-0.0153846153846154,-0.00577184337451766),
 .UNSPECIFIED.)
CURVE()
GEOMETRIC_REPRESENTATION_ITEM()
RATIONAL_B_SPLINE_CURVE((1.,1.,1.,1.,1.,1.,1.,1.,1.,1.,1.,1.,1.,1.,1.,1.,
1.,1.,1.,1.,1.,1.,1.,1.,1.,1.,1.,1.,1.,1.,1.,1.,1.,1.,1.,1.,1.,1.,1.,1.,
1.,1.,1.,1.,1.,1.,1.,1.,1.,1.,1.,1.,1.,1.,1.,1.,1.,1.,1.,1.,1.,1.,1.,1.,
1.,1.,1.,1.,1.,1.))
REPRESENTATION_ITEM('')
);
#308=(
BOUNDED_CURVE()
B_SPLINE_CURVE(5,(#48531,#48532,#48533,#48534,#48535,#48536,#48537,#48538,
#48539,#48540,#48541,#48542,#48543,#48544,#48545,#48546,#48547,#48548,#48549,
#48550,#48551,#48552,#48553,#48554,#48555,#48556,#48557,#48558,#48559,#48560,
#48561,#48562,#48563,#48564,#48565,#48566,#48567,#48568,#48569,#48570,#48571,
#48572,#48573,#48574,#48575,#48576,#48577,#48578,#48579,#48580,#48581,#48582,
#48583,#48584,#48585,#48586,#48587,#48588,#48589,#48590,#48591,#48592,#48593,
#48594,#48595,#48596,#48597,#48598,#48599,#48600),.UNSPECIFIED.,.F.,.F.)
B_SPLINE_CURVE_WITH_KNOTS((6,1,1,1,1,1,1,1,1,1,1,1,1,1,1,1,1,1,1,1,1,1,
1,1,1,1,1,1,1,1,1,1,1,1,1,1,1,1,1,1,1,1,1,1,1,1,1,1,1,1,1,1,1,1,1,1,1,1,
1,1,1,1,1,1,1,6),(-0.994228156739687,-0.984615384615383,-0.969230769230768,
-0.953846153846152,-0.938461538461537,-0.923076923076922,-0.907692307692306,
-0.892307692307691,-0.876923076923076,-0.86153846153846,-0.846153846153845,
-0.83076923076923,-0.815384615384614,-0.799999999999999,-0.784615384615384,
-0.769230769230768,-0.753846153846153,-0.738461538461538,-0.723076923076922,
-0.707692307692307,-0.692307692307692,-0.676923076923076,-0.661538461538461,
-0.646153846153846,-0.63076923076923,-0.615384615384615,-0.6,-0.584615384615384,
-0.569230769230769,-0.553846153846154,-0.538461538461538,-0.523076923076923,
-0.507692307692308,-0.492307692307692,-0.476923076923077,-0.461538461538462,
-0.446153846153846,-0.430769230769231,-0.415384615384615,-0.4,-0.384615384615385,
-0.369230769230769,-0.353846153846154,-0.338461538461538,-0.323076923076923,
-0.307692307692308,-0.292307692307692,-0.276923076923077,-0.261538461538462,
-0.246153846153846,-0.230769230769231,-0.215384615384615,-0.2,-0.184615384615385,
-0.169230769230769,-0.153846153846154,-0.138461538461538,-0.123076923076923,
-0.107692307692308,-0.0923076923076923,-0.0769230769230769,-0.0615384615384615,
-0.0461538461538462,-0.0307692307692308,-0.0153846153846154,0.),
 .UNSPECIFIED.)
CURVE()
GEOMETRIC_REPRESENTATION_ITEM()
RATIONAL_B_SPLINE_CURVE((1.,1.,1.,1.,1.,1.,1.,1.,1.,1.,1.,1.,1.,1.,1.,1.,
1.,1.,1.,1.,1.,1.,1.,1.,1.,1.,1.,1.,1.,1.,1.,1.,1.,1.,1.,1.,1.,1.,1.,1.,
1.,1.,1.,1.,1.,1.,1.,1.,1.,1.,1.,1.,1.,1.,1.,1.,1.,1.,1.,1.,1.,1.,1.,1.,
1.,1.,1.,1.,1.,1.))
REPRESENTATION_ITEM('')
);
#309=(
BOUNDED_CURVE()
B_SPLINE_CURVE(5,(#48753,#48754,#48755,#48756,#48757,#48758,#48759,#48760,
#48761,#48762,#48763,#48764,#48765,#48766,#48767,#48768,#48769,#48770,#48771,
#48772,#48773,#48774,#48775,#48776,#48777,#48778,#48779,#48780,#48781,#48782,
#48783,#48784,#48785,#48786,#48787,#48788,#48789,#48790,#48791,#48792,#48793,
#48794,#48795,#48796,#48797,#48798,#48799,#48800,#48801,#48802,#48803,#48804,
#48805,#48806,#48807,#48808,#48809,#48810,#48811,#48812,#48813,#48814,#48815,
#48816,#48817,#48818,#48819,#48820,#48821,#48822),.UNSPECIFIED.,.F.,.F.)
B_SPLINE_CURVE_WITH_KNOTS((6,1,1,1,1,1,1,1,1,1,1,1,1,1,1,1,1,1,1,1,1,1,
1,1,1,1,1,1,1,1,1,1,1,1,1,1,1,1,1,1,1,1,1,1,1,1,1,1,1,1,1,1,1,1,1,1,1,1,
1,1,1,1,1,1,1,6),(-1.,-0.984615384615383,-0.969230769230768,-0.953846153846152,
-0.938461538461537,-0.923076923076922,-0.907692307692306,-0.892307692307691,
-0.876923076923076,-0.86153846153846,-0.846153846153845,-0.83076923076923,
-0.815384615384614,-0.799999999999999,-0.784615384615384,-0.769230769230768,
-0.753846153846153,-0.738461538461538,-0.723076923076922,-0.707692307692307,
-0.692307692307692,-0.676923076923076,-0.661538461538461,-0.646153846153846,
-0.63076923076923,-0.615384615384615,-0.6,-0.584615384615384,-0.569230769230769,
-0.553846153846154,-0.538461538461538,-0.523076923076923,-0.507692307692308,
-0.492307692307692,-0.476923076923077,-0.461538461538462,-0.446153846153846,
-0.430769230769231,-0.415384615384615,-0.4,-0.384615384615385,-0.369230769230769,
-0.353846153846154,-0.338461538461538,-0.323076923076923,-0.307692307692308,
-0.292307692307692,-0.276923076923077,-0.261538461538462,-0.246153846153846,
-0.230769230769231,-0.215384615384615,-0.2,-0.184615384615385,-0.169230769230769,
-0.153846153846154,-0.138461538461538,-0.123076923076923,-0.107692307692308,
-0.0923076923076923,-0.0769230769230769,-0.0615384615384615,-0.0461538461538462,
-0.0307692307692308,-0.0153846153846154,-0.00577184337452512),
 .UNSPECIFIED.)
CURVE()
GEOMETRIC_REPRESENTATION_ITEM()
RATIONAL_B_SPLINE_CURVE((1.,1.,1.,1.,1.,1.,1.,1.,1.,1.,1.,1.,1.,1.,1.,1.,
1.,1.,1.,1.,1.,1.,1.,1.,1.,1.,1.,1.,1.,1.,1.,1.,1.,1.,1.,1.,1.,1.,1.,1.,
1.,1.,1.,1.,1.,1.,1.,1.,1.,1.,1.,1.,1.,1.,1.,1.,1.,1.,1.,1.,1.,1.,1.,1.,
1.,1.,1.,1.,1.,1.))
REPRESENTATION_ITEM('')
);
#310=(
BOUNDED_CURVE()
B_SPLINE_CURVE(5,(#48973,#48974,#48975,#48976,#48977,#48978,#48979,#48980,
#48981,#48982,#48983,#48984,#48985,#48986,#48987,#48988,#48989,#48990,#48991,
#48992,#48993,#48994,#48995,#48996,#48997,#48998,#48999,#49000,#49001,#49002,
#49003,#49004,#49005,#49006,#49007,#49008,#49009,#49010,#49011,#49012,#49013,
#49014,#49015,#49016,#49017,#49018,#49019,#49020,#49021,#49022,#49023,#49024,
#49025,#49026,#49027,#49028,#49029,#49030,#49031,#49032,#49033,#49034,#49035,
#49036,#49037,#49038,#49039,#49040,#49041,#49042),.UNSPECIFIED.,.F.,.F.)
B_SPLINE_CURVE_WITH_KNOTS((6,1,1,1,1,1,1,1,1,1,1,1,1,1,1,1,1,1,1,1,1,1,
1,1,1,1,1,1,1,1,1,1,1,1,1,1,1,1,1,1,1,1,1,1,1,1,1,1,1,1,1,1,1,1,1,1,1,1,
1,1,1,1,1,1,1,6),(-0.994228156739691,-0.984615384615383,-0.969230769230768,
-0.953846153846152,-0.938461538461537,-0.923076923076922,-0.907692307692306,
-0.892307692307691,-0.876923076923076,-0.86153846153846,-0.846153846153845,
-0.83076923076923,-0.815384615384614,-0.799999999999999,-0.784615384615384,
-0.769230769230768,-0.753846153846153,-0.738461538461538,-0.723076923076922,
-0.707692307692307,-0.692307692307692,-0.676923076923076,-0.661538461538461,
-0.646153846153846,-0.63076923076923,-0.615384615384615,-0.6,-0.584615384615384,
-0.569230769230769,-0.553846153846154,-0.538461538461538,-0.523076923076923,
-0.507692307692308,-0.492307692307692,-0.476923076923077,-0.461538461538462,
-0.446153846153846,-0.430769230769231,-0.415384615384615,-0.4,-0.384615384615385,
-0.369230769230769,-0.353846153846154,-0.338461538461538,-0.323076923076923,
-0.307692307692308,-0.292307692307692,-0.276923076923077,-0.261538461538462,
-0.246153846153846,-0.230769230769231,-0.215384615384615,-0.2,-0.184615384615385,
-0.169230769230769,-0.153846153846154,-0.138461538461538,-0.123076923076923,
-0.107692307692308,-0.0923076923076923,-0.0769230769230769,-0.0615384615384615,
-0.0461538461538462,-0.0307692307692308,-0.0153846153846154,0.),
 .UNSPECIFIED.)
CURVE()
GEOMETRIC_REPRESENTATION_ITEM()
RATIONAL_B_SPLINE_CURVE((1.,1.,1.,1.,1.,1.,1.,1.,1.,1.,1.,1.,1.,1.,1.,1.,
1.,1.,1.,1.,1.,1.,1.,1.,1.,1.,1.,1.,1.,1.,1.,1.,1.,1.,1.,1.,1.,1.,1.,1.,
1.,1.,1.,1.,1.,1.,1.,1.,1.,1.,1.,1.,1.,1.,1.,1.,1.,1.,1.,1.,1.,1.,1.,1.,
1.,1.,1.,1.,1.,1.))
REPRESENTATION_ITEM('')
);
#311=(
BOUNDED_CURVE()
B_SPLINE_CURVE(5,(#49195,#49196,#49197,#49198,#49199,#49200,#49201,#49202,
#49203,#49204,#49205,#49206,#49207,#49208,#49209,#49210,#49211,#49212,#49213,
#49214,#49215,#49216,#49217,#49218,#49219,#49220,#49221,#49222,#49223,#49224,
#49225,#49226,#49227,#49228,#49229,#49230,#49231,#49232,#49233,#49234,#49235,
#49236,#49237,#49238,#49239,#49240,#49241,#49242,#49243,#49244,#49245,#49246,
#49247,#49248,#49249,#49250,#49251,#49252,#49253,#49254,#49255,#49256,#49257,
#49258,#49259,#49260,#49261,#49262,#49263,#49264),.UNSPECIFIED.,.F.,.F.)
B_SPLINE_CURVE_WITH_KNOTS((6,1,1,1,1,1,1,1,1,1,1,1,1,1,1,1,1,1,1,1,1,1,
1,1,1,1,1,1,1,1,1,1,1,1,1,1,1,1,1,1,1,1,1,1,1,1,1,1,1,1,1,1,1,1,1,1,1,1,
1,1,1,1,1,1,1,6),(-1.,-0.984615384615383,-0.969230769230768,-0.953846153846152,
-0.938461538461537,-0.923076923076922,-0.907692307692306,-0.892307692307691,
-0.876923076923076,-0.86153846153846,-0.846153846153845,-0.83076923076923,
-0.815384615384614,-0.799999999999999,-0.784615384615384,-0.769230769230768,
-0.753846153846153,-0.738461538461538,-0.723076923076922,-0.707692307692307,
-0.692307692307692,-0.676923076923076,-0.661538461538461,-0.646153846153846,
-0.63076923076923,-0.615384615384615,-0.6,-0.584615384615384,-0.569230769230769,
-0.553846153846154,-0.538461538461538,-0.523076923076923,-0.507692307692308,
-0.492307692307692,-0.476923076923077,-0.461538461538462,-0.446153846153846,
-0.430769230769231,-0.415384615384615,-0.4,-0.384615384615385,-0.369230769230769,
-0.353846153846154,-0.338461538461538,-0.323076923076923,-0.307692307692308,
-0.292307692307692,-0.276923076923077,-0.261538461538462,-0.246153846153846,
-0.230769230769231,-0.215384615384615,-0.2,-0.184615384615385,-0.169230769230769,
-0.153846153846154,-0.138461538461538,-0.123076923076923,-0.107692307692308,
-0.0923076923076923,-0.0769230769230769,-0.0615384615384615,-0.0461538461538462,
-0.0307692307692308,-0.0153846153846154,-0.00577184337448448),
 .UNSPECIFIED.)
CURVE()
GEOMETRIC_REPRESENTATION_ITEM()
RATIONAL_B_SPLINE_CURVE((1.,1.,1.,1.,1.,1.,1.,1.,1.,1.,1.,1.,1.,1.,1.,1.,
1.,1.,1.,1.,1.,1.,1.,1.,1.,1.,1.,1.,1.,1.,1.,1.,1.,1.,1.,1.,1.,1.,1.,1.,
1.,1.,1.,1.,1.,1.,1.,1.,1.,1.,1.,1.,1.,1.,1.,1.,1.,1.,1.,1.,1.,1.,1.,1.,
1.,1.,1.,1.,1.,1.))
REPRESENTATION_ITEM('')
);
#312=(
BOUNDED_CURVE()
B_SPLINE_CURVE(5,(#49415,#49416,#49417,#49418,#49419,#49420,#49421,#49422,
#49423,#49424,#49425,#49426,#49427,#49428,#49429,#49430,#49431,#49432,#49433,
#49434,#49435,#49436,#49437,#49438,#49439,#49440,#49441,#49442,#49443,#49444,
#49445,#49446,#49447,#49448,#49449,#49450,#49451,#49452,#49453,#49454,#49455,
#49456,#49457,#49458,#49459,#49460,#49461,#49462,#49463,#49464,#49465,#49466,
#49467,#49468,#49469,#49470,#49471,#49472,#49473,#49474,#49475,#49476,#49477,
#49478,#49479,#49480,#49481,#49482,#49483,#49484),.UNSPECIFIED.,.F.,.F.)
B_SPLINE_CURVE_WITH_KNOTS((6,1,1,1,1,1,1,1,1,1,1,1,1,1,1,1,1,1,1,1,1,1,
1,1,1,1,1,1,1,1,1,1,1,1,1,1,1,1,1,1,1,1,1,1,1,1,1,1,1,1,1,1,1,1,1,1,1,1,
1,1,1,1,1,1,1,6),(-0.99422815673972,-0.984615384615383,-0.969230769230768,
-0.953846153846152,-0.938461538461537,-0.923076923076922,-0.907692307692306,
-0.892307692307691,-0.876923076923076,-0.86153846153846,-0.846153846153845,
-0.83076923076923,-0.815384615384614,-0.799999999999999,-0.784615384615384,
-0.769230769230768,-0.753846153846153,-0.738461538461538,-0.723076923076922,
-0.707692307692307,-0.692307692307692,-0.676923076923076,-0.661538461538461,
-0.646153846153846,-0.63076923076923,-0.615384615384615,-0.6,-0.584615384615384,
-0.569230769230769,-0.553846153846154,-0.538461538461538,-0.523076923076923,
-0.507692307692308,-0.492307692307692,-0.476923076923077,-0.461538461538462,
-0.446153846153846,-0.430769230769231,-0.415384615384615,-0.4,-0.384615384615385,
-0.369230769230769,-0.353846153846154,-0.338461538461538,-0.323076923076923,
-0.307692307692308,-0.292307692307692,-0.276923076923077,-0.261538461538462,
-0.246153846153846,-0.230769230769231,-0.215384615384615,-0.2,-0.184615384615385,
-0.169230769230769,-0.153846153846154,-0.138461538461538,-0.123076923076923,
-0.107692307692308,-0.0923076923076923,-0.0769230769230769,-0.0615384615384615,
-0.0461538461538462,-0.0307692307692308,-0.0153846153846154,0.),
 .UNSPECIFIED.)
CURVE()
GEOMETRIC_REPRESENTATION_ITEM()
RATIONAL_B_SPLINE_CURVE((1.,1.,1.,1.,1.,1.,1.,1.,1.,1.,1.,1.,1.,1.,1.,1.,
1.,1.,1.,1.,1.,1.,1.,1.,1.,1.,1.,1.,1.,1.,1.,1.,1.,1.,1.,1.,1.,1.,1.,1.,
1.,1.,1.,1.,1.,1.,1.,1.,1.,1.,1.,1.,1.,1.,1.,1.,1.,1.,1.,1.,1.,1.,1.,1.,
1.,1.,1.,1.,1.,1.))
REPRESENTATION_ITEM('')
);
#313=(
BOUNDED_CURVE()
B_SPLINE_CURVE(5,(#49637,#49638,#49639,#49640,#49641,#49642,#49643,#49644,
#49645,#49646,#49647,#49648,#49649,#49650,#49651,#49652,#49653,#49654,#49655,
#49656,#49657,#49658,#49659,#49660,#49661,#49662,#49663,#49664,#49665,#49666,
#49667,#49668,#49669,#49670,#49671,#49672,#49673,#49674,#49675,#49676,#49677,
#49678,#49679,#49680,#49681,#49682,#49683,#49684,#49685,#49686,#49687,#49688,
#49689,#49690,#49691,#49692,#49693,#49694,#49695,#49696,#49697,#49698,#49699,
#49700,#49701,#49702,#49703,#49704,#49705,#49706),.UNSPECIFIED.,.F.,.F.)
B_SPLINE_CURVE_WITH_KNOTS((6,1,1,1,1,1,1,1,1,1,1,1,1,1,1,1,1,1,1,1,1,1,
1,1,1,1,1,1,1,1,1,1,1,1,1,1,1,1,1,1,1,1,1,1,1,1,1,1,1,1,1,1,1,1,1,1,1,1,
1,1,1,1,1,1,1,6),(-1.,-0.984615384615383,-0.969230769230768,-0.953846153846152,
-0.938461538461537,-0.923076923076922,-0.907692307692306,-0.892307692307691,
-0.876923076923076,-0.86153846153846,-0.846153846153845,-0.83076923076923,
-0.815384615384614,-0.799999999999999,-0.784615384615384,-0.769230769230768,
-0.753846153846153,-0.738461538461538,-0.723076923076922,-0.707692307692307,
-0.692307692307692,-0.676923076923076,-0.661538461538461,-0.646153846153846,
-0.63076923076923,-0.615384615384615,-0.6,-0.584615384615384,-0.569230769230769,
-0.553846153846154,-0.538461538461538,-0.523076923076923,-0.507692307692308,
-0.492307692307692,-0.476923076923077,-0.461538461538462,-0.446153846153846,
-0.430769230769231,-0.415384615384615,-0.4,-0.384615384615385,-0.369230769230769,
-0.353846153846154,-0.338461538461538,-0.323076923076923,-0.307692307692308,
-0.292307692307692,-0.276923076923077,-0.261538461538462,-0.246153846153846,
-0.230769230769231,-0.215384615384615,-0.2,-0.184615384615385,-0.169230769230769,
-0.153846153846154,-0.138461538461538,-0.123076923076923,-0.107692307692308,
-0.0923076923076923,-0.0769230769230769,-0.0615384615384615,-0.0461538461538462,
-0.0307692307692308,-0.0153846153846154,-0.00577184337448251),
 .UNSPECIFIED.)
CURVE()
GEOMETRIC_REPRESENTATION_ITEM()
RATIONAL_B_SPLINE_CURVE((1.,1.,1.,1.,1.,1.,1.,1.,1.,1.,1.,1.,1.,1.,1.,1.,
1.,1.,1.,1.,1.,1.,1.,1.,1.,1.,1.,1.,1.,1.,1.,1.,1.,1.,1.,1.,1.,1.,1.,1.,
1.,1.,1.,1.,1.,1.,1.,1.,1.,1.,1.,1.,1.,1.,1.,1.,1.,1.,1.,1.,1.,1.,1.,1.,
1.,1.,1.,1.,1.,1.))
REPRESENTATION_ITEM('')
);
#314=(
BOUNDED_CURVE()
B_SPLINE_CURVE(5,(#49857,#49858,#49859,#49860,#49861,#49862,#49863,#49864,
#49865,#49866,#49867,#49868,#49869,#49870,#49871,#49872,#49873,#49874,#49875,
#49876,#49877,#49878,#49879,#49880,#49881,#49882,#49883,#49884,#49885,#49886,
#49887,#49888,#49889,#49890,#49891,#49892,#49893,#49894,#49895,#49896,#49897,
#49898,#49899,#49900,#49901,#49902,#49903,#49904,#49905,#49906,#49907,#49908,
#49909,#49910,#49911,#49912,#49913,#49914,#49915,#49916,#49917,#49918,#49919,
#49920,#49921,#49922,#49923,#49924,#49925,#49926),.UNSPECIFIED.,.F.,.F.)
B_SPLINE_CURVE_WITH_KNOTS((6,1,1,1,1,1,1,1,1,1,1,1,1,1,1,1,1,1,1,1,1,1,
1,1,1,1,1,1,1,1,1,1,1,1,1,1,1,1,1,1,1,1,1,1,1,1,1,1,1,1,1,1,1,1,1,1,1,1,
1,1,1,1,1,1,1,6),(-0.994228156739703,-0.984615384615383,-0.969230769230768,
-0.953846153846152,-0.938461538461537,-0.923076923076922,-0.907692307692306,
-0.892307692307691,-0.876923076923076,-0.86153846153846,-0.846153846153845,
-0.83076923076923,-0.815384615384614,-0.799999999999999,-0.784615384615384,
-0.769230769230768,-0.753846153846153,-0.738461538461538,-0.723076923076922,
-0.707692307692307,-0.692307692307692,-0.676923076923076,-0.661538461538461,
-0.646153846153846,-0.63076923076923,-0.615384615384615,-0.6,-0.584615384615384,
-0.569230769230769,-0.553846153846154,-0.538461538461538,-0.523076923076923,
-0.507692307692308,-0.492307692307692,-0.476923076923077,-0.461538461538462,
-0.446153846153846,-0.430769230769231,-0.415384615384615,-0.4,-0.384615384615385,
-0.369230769230769,-0.353846153846154,-0.338461538461538,-0.323076923076923,
-0.307692307692308,-0.292307692307692,-0.276923076923077,-0.261538461538462,
-0.246153846153846,-0.230769230769231,-0.215384615384615,-0.2,-0.184615384615385,
-0.169230769230769,-0.153846153846154,-0.138461538461538,-0.123076923076923,
-0.107692307692308,-0.0923076923076923,-0.0769230769230769,-0.0615384615384615,
-0.0461538461538462,-0.0307692307692308,-0.0153846153846154,0.),
 .UNSPECIFIED.)
CURVE()
GEOMETRIC_REPRESENTATION_ITEM()
RATIONAL_B_SPLINE_CURVE((1.,1.,1.,1.,1.,1.,1.,1.,1.,1.,1.,1.,1.,1.,1.,1.,
1.,1.,1.,1.,1.,1.,1.,1.,1.,1.,1.,1.,1.,1.,1.,1.,1.,1.,1.,1.,1.,1.,1.,1.,
1.,1.,1.,1.,1.,1.,1.,1.,1.,1.,1.,1.,1.,1.,1.,1.,1.,1.,1.,1.,1.,1.,1.,1.,
1.,1.,1.,1.,1.,1.))
REPRESENTATION_ITEM('')
);
#315=(
BOUNDED_CURVE()
B_SPLINE_CURVE(5,(#50079,#50080,#50081,#50082,#50083,#50084,#50085,#50086,
#50087,#50088,#50089,#50090,#50091,#50092,#50093,#50094,#50095,#50096,#50097,
#50098,#50099,#50100,#50101,#50102,#50103,#50104,#50105,#50106,#50107,#50108,
#50109,#50110,#50111,#50112,#50113,#50114,#50115,#50116,#50117,#50118,#50119,
#50120,#50121,#50122,#50123,#50124,#50125,#50126,#50127,#50128,#50129,#50130,
#50131,#50132,#50133,#50134,#50135,#50136,#50137,#50138,#50139,#50140,#50141,
#50142,#50143,#50144,#50145,#50146,#50147,#50148),.UNSPECIFIED.,.F.,.F.)
B_SPLINE_CURVE_WITH_KNOTS((6,1,1,1,1,1,1,1,1,1,1,1,1,1,1,1,1,1,1,1,1,1,
1,1,1,1,1,1,1,1,1,1,1,1,1,1,1,1,1,1,1,1,1,1,1,1,1,1,1,1,1,1,1,1,1,1,1,1,
1,1,1,1,1,1,1,6),(-1.,-0.984615384615383,-0.969230769230768,-0.953846153846152,
-0.938461538461537,-0.923076923076922,-0.907692307692306,-0.892307692307691,
-0.876923076923076,-0.86153846153846,-0.846153846153845,-0.83076923076923,
-0.815384615384614,-0.799999999999999,-0.784615384615384,-0.769230769230768,
-0.753846153846153,-0.738461538461538,-0.723076923076922,-0.707692307692307,
-0.692307692307692,-0.676923076923076,-0.661538461538461,-0.646153846153846,
-0.63076923076923,-0.615384615384615,-0.6,-0.584615384615384,-0.569230769230769,
-0.553846153846154,-0.538461538461538,-0.523076923076923,-0.507692307692308,
-0.492307692307692,-0.476923076923077,-0.461538461538462,-0.446153846153846,
-0.430769230769231,-0.415384615384615,-0.4,-0.384615384615385,-0.369230769230769,
-0.353846153846154,-0.338461538461538,-0.323076923076923,-0.307692307692308,
-0.292307692307692,-0.276923076923077,-0.261538461538462,-0.246153846153846,
-0.230769230769231,-0.215384615384615,-0.2,-0.184615384615385,-0.169230769230769,
-0.153846153846154,-0.138461538461538,-0.123076923076923,-0.107692307692308,
-0.0923076923076923,-0.0769230769230769,-0.0615384615384615,-0.0461538461538462,
-0.0307692307692308,-0.0153846153846154,-0.00577184337449602),
 .UNSPECIFIED.)
CURVE()
GEOMETRIC_REPRESENTATION_ITEM()
RATIONAL_B_SPLINE_CURVE((1.,1.,1.,1.,1.,1.,1.,1.,1.,1.,1.,1.,1.,1.,1.,1.,
1.,1.,1.,1.,1.,1.,1.,1.,1.,1.,1.,1.,1.,1.,1.,1.,1.,1.,1.,1.,1.,1.,1.,1.,
1.,1.,1.,1.,1.,1.,1.,1.,1.,1.,1.,1.,1.,1.,1.,1.,1.,1.,1.,1.,1.,1.,1.,1.,
1.,1.,1.,1.,1.,1.))
REPRESENTATION_ITEM('')
);
#316=(
BOUNDED_CURVE()
B_SPLINE_CURVE(5,(#50299,#50300,#50301,#50302,#50303,#50304,#50305,#50306,
#50307,#50308,#50309,#50310,#50311,#50312,#50313,#50314,#50315,#50316,#50317,
#50318,#50319,#50320,#50321,#50322,#50323,#50324,#50325,#50326,#50327,#50328,
#50329,#50330,#50331,#50332,#50333,#50334,#50335,#50336,#50337,#50338,#50339,
#50340,#50341,#50342,#50343,#50344,#50345,#50346,#50347,#50348,#50349,#50350,
#50351,#50352,#50353,#50354,#50355,#50356,#50357,#50358,#50359,#50360,#50361,
#50362,#50363,#50364,#50365,#50366,#50367,#50368),.UNSPECIFIED.,.F.,.F.)
B_SPLINE_CURVE_WITH_KNOTS((6,1,1,1,1,1,1,1,1,1,1,1,1,1,1,1,1,1,1,1,1,1,
1,1,1,1,1,1,1,1,1,1,1,1,1,1,1,1,1,1,1,1,1,1,1,1,1,1,1,1,1,1,1,1,1,1,1,1,
1,1,1,1,1,1,1,6),(-0.994228156739695,-0.984615384615383,-0.969230769230768,
-0.953846153846152,-0.938461538461537,-0.923076923076922,-0.907692307692306,
-0.892307692307691,-0.876923076923076,-0.86153846153846,-0.846153846153845,
-0.83076923076923,-0.815384615384614,-0.799999999999999,-0.784615384615384,
-0.769230769230768,-0.753846153846153,-0.738461538461538,-0.723076923076922,
-0.707692307692307,-0.692307692307692,-0.676923076923076,-0.661538461538461,
-0.646153846153846,-0.63076923076923,-0.615384615384615,-0.6,-0.584615384615384,
-0.569230769230769,-0.553846153846154,-0.538461538461538,-0.523076923076923,
-0.507692307692308,-0.492307692307692,-0.476923076923077,-0.461538461538462,
-0.446153846153846,-0.430769230769231,-0.415384615384615,-0.4,-0.384615384615385,
-0.369230769230769,-0.353846153846154,-0.338461538461538,-0.323076923076923,
-0.307692307692308,-0.292307692307692,-0.276923076923077,-0.261538461538462,
-0.246153846153846,-0.230769230769231,-0.215384615384615,-0.2,-0.184615384615385,
-0.169230769230769,-0.153846153846154,-0.138461538461538,-0.123076923076923,
-0.107692307692308,-0.0923076923076923,-0.0769230769230769,-0.0615384615384615,
-0.0461538461538462,-0.0307692307692308,-0.0153846153846154,0.),
 .UNSPECIFIED.)
CURVE()
GEOMETRIC_REPRESENTATION_ITEM()
RATIONAL_B_SPLINE_CURVE((1.,1.,1.,1.,1.,1.,1.,1.,1.,1.,1.,1.,1.,1.,1.,1.,
1.,1.,1.,1.,1.,1.,1.,1.,1.,1.,1.,1.,1.,1.,1.,1.,1.,1.,1.,1.,1.,1.,1.,1.,
1.,1.,1.,1.,1.,1.,1.,1.,1.,1.,1.,1.,1.,1.,1.,1.,1.,1.,1.,1.,1.,1.,1.,1.,
1.,1.,1.,1.,1.,1.))
REPRESENTATION_ITEM('')
);
#317=(
BOUNDED_CURVE()
B_SPLINE_CURVE(5,(#50521,#50522,#50523,#50524,#50525,#50526,#50527,#50528,
#50529,#50530,#50531,#50532,#50533,#50534,#50535,#50536,#50537,#50538,#50539,
#50540,#50541,#50542,#50543,#50544,#50545,#50546,#50547,#50548,#50549,#50550,
#50551,#50552,#50553,#50554,#50555,#50556,#50557,#50558,#50559,#50560,#50561,
#50562,#50563,#50564,#50565,#50566,#50567,#50568,#50569,#50570,#50571,#50572,
#50573,#50574,#50575,#50576,#50577,#50578,#50579,#50580,#50581,#50582,#50583,
#50584,#50585,#50586,#50587,#50588,#50589,#50590),.UNSPECIFIED.,.F.,.F.)
B_SPLINE_CURVE_WITH_KNOTS((6,1,1,1,1,1,1,1,1,1,1,1,1,1,1,1,1,1,1,1,1,1,
1,1,1,1,1,1,1,1,1,1,1,1,1,1,1,1,1,1,1,1,1,1,1,1,1,1,1,1,1,1,1,1,1,1,1,1,
1,1,1,1,1,1,1,6),(-1.,-0.984615384615383,-0.969230769230768,-0.953846153846152,
-0.938461538461537,-0.923076923076922,-0.907692307692306,-0.892307692307691,
-0.876923076923076,-0.86153846153846,-0.846153846153845,-0.83076923076923,
-0.815384615384614,-0.799999999999999,-0.784615384615384,-0.769230769230768,
-0.753846153846153,-0.738461538461538,-0.723076923076922,-0.707692307692307,
-0.692307692307692,-0.676923076923076,-0.661538461538461,-0.646153846153846,
-0.63076923076923,-0.615384615384615,-0.6,-0.584615384615384,-0.569230769230769,
-0.553846153846154,-0.538461538461538,-0.523076923076923,-0.507692307692308,
-0.492307692307692,-0.476923076923077,-0.461538461538462,-0.446153846153846,
-0.430769230769231,-0.415384615384615,-0.4,-0.384615384615385,-0.369230769230769,
-0.353846153846154,-0.338461538461538,-0.323076923076923,-0.307692307692308,
-0.292307692307692,-0.276923076923077,-0.261538461538462,-0.246153846153846,
-0.230769230769231,-0.215384615384615,-0.2,-0.184615384615385,-0.169230769230769,
-0.153846153846154,-0.138461538461538,-0.123076923076923,-0.107692307692308,
-0.0923076923076923,-0.0769230769230769,-0.0615384615384615,-0.0461538461538462,
-0.0307692307692308,-0.0153846153846154,-0.00577184337450911),
 .UNSPECIFIED.)
CURVE()
GEOMETRIC_REPRESENTATION_ITEM()
RATIONAL_B_SPLINE_CURVE((1.,1.,1.,1.,1.,1.,1.,1.,1.,1.,1.,1.,1.,1.,1.,1.,
1.,1.,1.,1.,1.,1.,1.,1.,1.,1.,1.,1.,1.,1.,1.,1.,1.,1.,1.,1.,1.,1.,1.,1.,
1.,1.,1.,1.,1.,1.,1.,1.,1.,1.,1.,1.,1.,1.,1.,1.,1.,1.,1.,1.,1.,1.,1.,1.,
1.,1.,1.,1.,1.,1.))
REPRESENTATION_ITEM('')
);
#318=(
BOUNDED_CURVE()
B_SPLINE_CURVE(5,(#50741,#50742,#50743,#50744,#50745,#50746,#50747,#50748,
#50749,#50750,#50751,#50752,#50753,#50754,#50755,#50756,#50757,#50758,#50759,
#50760,#50761,#50762,#50763,#50764,#50765,#50766,#50767,#50768,#50769,#50770,
#50771,#50772,#50773,#50774,#50775,#50776,#50777,#50778,#50779,#50780,#50781,
#50782,#50783,#50784,#50785,#50786,#50787,#50788,#50789,#50790,#50791,#50792,
#50793,#50794,#50795,#50796,#50797,#50798,#50799,#50800,#50801,#50802,#50803,
#50804,#50805,#50806,#50807,#50808,#50809,#50810),.UNSPECIFIED.,.F.,.F.)
B_SPLINE_CURVE_WITH_KNOTS((6,1,1,1,1,1,1,1,1,1,1,1,1,1,1,1,1,1,1,1,1,1,
1,1,1,1,1,1,1,1,1,1,1,1,1,1,1,1,1,1,1,1,1,1,1,1,1,1,1,1,1,1,1,1,1,1,1,1,
1,1,1,1,1,1,1,6),(-0.994228156739712,-0.984615384615383,-0.969230769230768,
-0.953846153846152,-0.938461538461537,-0.923076923076922,-0.907692307692306,
-0.892307692307691,-0.876923076923076,-0.86153846153846,-0.846153846153845,
-0.83076923076923,-0.815384615384614,-0.799999999999999,-0.784615384615384,
-0.769230769230768,-0.753846153846153,-0.738461538461538,-0.723076923076922,
-0.707692307692307,-0.692307692307692,-0.676923076923076,-0.661538461538461,
-0.646153846153846,-0.63076923076923,-0.615384615384615,-0.6,-0.584615384615384,
-0.569230769230769,-0.553846153846154,-0.538461538461538,-0.523076923076923,
-0.507692307692308,-0.492307692307692,-0.476923076923077,-0.461538461538462,
-0.446153846153846,-0.430769230769231,-0.415384615384615,-0.4,-0.384615384615385,
-0.369230769230769,-0.353846153846154,-0.338461538461538,-0.323076923076923,
-0.307692307692308,-0.292307692307692,-0.276923076923077,-0.261538461538462,
-0.246153846153846,-0.230769230769231,-0.215384615384615,-0.2,-0.184615384615385,
-0.169230769230769,-0.153846153846154,-0.138461538461538,-0.123076923076923,
-0.107692307692308,-0.0923076923076923,-0.0769230769230769,-0.0615384615384615,
-0.0461538461538462,-0.0307692307692308,-0.0153846153846154,0.),
 .UNSPECIFIED.)
CURVE()
GEOMETRIC_REPRESENTATION_ITEM()
RATIONAL_B_SPLINE_CURVE((1.,1.,1.,1.,1.,1.,1.,1.,1.,1.,1.,1.,1.,1.,1.,1.,
1.,1.,1.,1.,1.,1.,1.,1.,1.,1.,1.,1.,1.,1.,1.,1.,1.,1.,1.,1.,1.,1.,1.,1.,
1.,1.,1.,1.,1.,1.,1.,1.,1.,1.,1.,1.,1.,1.,1.,1.,1.,1.,1.,1.,1.,1.,1.,1.,
1.,1.,1.,1.,1.,1.))
REPRESENTATION_ITEM('')
);
#319=(
BOUNDED_CURVE()
B_SPLINE_CURVE(5,(#50963,#50964,#50965,#50966,#50967,#50968,#50969,#50970,
#50971,#50972,#50973,#50974,#50975,#50976,#50977,#50978,#50979,#50980,#50981,
#50982,#50983,#50984,#50985,#50986,#50987,#50988,#50989,#50990,#50991,#50992,
#50993,#50994,#50995,#50996,#50997,#50998,#50999,#51000,#51001,#51002,#51003,
#51004,#51005,#51006,#51007,#51008,#51009,#51010,#51011,#51012,#51013,#51014,
#51015,#51016,#51017,#51018,#51019,#51020,#51021,#51022,#51023,#51024,#51025,
#51026,#51027,#51028,#51029,#51030,#51031,#51032),.UNSPECIFIED.,.F.,.F.)
B_SPLINE_CURVE_WITH_KNOTS((6,1,1,1,1,1,1,1,1,1,1,1,1,1,1,1,1,1,1,1,1,1,
1,1,1,1,1,1,1,1,1,1,1,1,1,1,1,1,1,1,1,1,1,1,1,1,1,1,1,1,1,1,1,1,1,1,1,1,
1,1,1,1,1,1,1,6),(-1.,-0.984615384615383,-0.969230769230768,-0.953846153846152,
-0.938461538461537,-0.923076923076922,-0.907692307692306,-0.892307692307691,
-0.876923076923076,-0.86153846153846,-0.846153846153845,-0.83076923076923,
-0.815384615384614,-0.799999999999999,-0.784615384615384,-0.769230769230768,
-0.753846153846153,-0.738461538461538,-0.723076923076922,-0.707692307692307,
-0.692307692307692,-0.676923076923076,-0.661538461538461,-0.646153846153846,
-0.63076923076923,-0.615384615384615,-0.6,-0.584615384615384,-0.569230769230769,
-0.553846153846154,-0.538461538461538,-0.523076923076923,-0.507692307692308,
-0.492307692307692,-0.476923076923077,-0.461538461538462,-0.446153846153846,
-0.430769230769231,-0.415384615384615,-0.4,-0.384615384615385,-0.369230769230769,
-0.353846153846154,-0.338461538461538,-0.323076923076923,-0.307692307692308,
-0.292307692307692,-0.276923076923077,-0.261538461538462,-0.246153846153846,
-0.230769230769231,-0.215384615384615,-0.2,-0.184615384615385,-0.169230769230769,
-0.153846153846154,-0.138461538461538,-0.123076923076923,-0.107692307692308,
-0.0923076923076923,-0.0769230769230769,-0.0615384615384615,-0.0461538461538462,
-0.0307692307692308,-0.0153846153846154,-0.00577184337451206),
 .UNSPECIFIED.)
CURVE()
GEOMETRIC_REPRESENTATION_ITEM()
RATIONAL_B_SPLINE_CURVE((1.,1.,1.,1.,1.,1.,1.,1.,1.,1.,1.,1.,1.,1.,1.,1.,
1.,1.,1.,1.,1.,1.,1.,1.,1.,1.,1.,1.,1.,1.,1.,1.,1.,1.,1.,1.,1.,1.,1.,1.,
1.,1.,1.,1.,1.,1.,1.,1.,1.,1.,1.,1.,1.,1.,1.,1.,1.,1.,1.,1.,1.,1.,1.,1.,
1.,1.,1.,1.,1.,1.))
REPRESENTATION_ITEM('')
);
#320=(
BOUNDED_CURVE()
B_SPLINE_CURVE(5,(#51183,#51184,#51185,#51186,#51187,#51188,#51189,#51190,
#51191,#51192,#51193,#51194,#51195,#51196,#51197,#51198,#51199,#51200,#51201,
#51202,#51203,#51204,#51205,#51206,#51207,#51208,#51209,#51210,#51211,#51212,
#51213,#51214,#51215,#51216,#51217,#51218,#51219,#51220,#51221,#51222,#51223,
#51224,#51225,#51226,#51227,#51228,#51229,#51230,#51231,#51232,#51233,#51234,
#51235,#51236,#51237,#51238,#51239,#51240,#51241,#51242,#51243,#51244,#51245,
#51246,#51247,#51248,#51249,#51250,#51251,#51252),.UNSPECIFIED.,.F.,.F.)
B_SPLINE_CURVE_WITH_KNOTS((6,1,1,1,1,1,1,1,1,1,1,1,1,1,1,1,1,1,1,1,1,1,
1,1,1,1,1,1,1,1,1,1,1,1,1,1,1,1,1,1,1,1,1,1,1,1,1,1,1,1,1,1,1,1,1,1,1,1,
1,1,1,1,1,1,1,6),(-0.994228156739717,-0.984615384615383,-0.969230769230768,
-0.953846153846152,-0.938461538461537,-0.923076923076922,-0.907692307692306,
-0.892307692307691,-0.876923076923076,-0.86153846153846,-0.846153846153845,
-0.83076923076923,-0.815384615384614,-0.799999999999999,-0.784615384615384,
-0.769230769230768,-0.753846153846153,-0.738461538461538,-0.723076923076922,
-0.707692307692307,-0.692307692307692,-0.676923076923076,-0.661538461538461,
-0.646153846153846,-0.63076923076923,-0.615384615384615,-0.6,-0.584615384615384,
-0.569230769230769,-0.553846153846154,-0.538461538461538,-0.523076923076923,
-0.507692307692308,-0.492307692307692,-0.476923076923077,-0.461538461538462,
-0.446153846153846,-0.430769230769231,-0.415384615384615,-0.4,-0.384615384615385,
-0.369230769230769,-0.353846153846154,-0.338461538461538,-0.323076923076923,
-0.307692307692308,-0.292307692307692,-0.276923076923077,-0.261538461538462,
-0.246153846153846,-0.230769230769231,-0.215384615384615,-0.2,-0.184615384615385,
-0.169230769230769,-0.153846153846154,-0.138461538461538,-0.123076923076923,
-0.107692307692308,-0.0923076923076923,-0.0769230769230769,-0.0615384615384615,
-0.0461538461538462,-0.0307692307692308,-0.0153846153846154,0.),
 .UNSPECIFIED.)
CURVE()
GEOMETRIC_REPRESENTATION_ITEM()
RATIONAL_B_SPLINE_CURVE((1.,1.,1.,1.,1.,1.,1.,1.,1.,1.,1.,1.,1.,1.,1.,1.,
1.,1.,1.,1.,1.,1.,1.,1.,1.,1.,1.,1.,1.,1.,1.,1.,1.,1.,1.,1.,1.,1.,1.,1.,
1.,1.,1.,1.,1.,1.,1.,1.,1.,1.,1.,1.,1.,1.,1.,1.,1.,1.,1.,1.,1.,1.,1.,1.,
1.,1.,1.,1.,1.,1.))
REPRESENTATION_ITEM('')
);
#321=(
BOUNDED_CURVE()
B_SPLINE_CURVE(5,(#51405,#51406,#51407,#51408,#51409,#51410,#51411,#51412,
#51413,#51414,#51415,#51416,#51417,#51418,#51419,#51420,#51421,#51422,#51423,
#51424,#51425,#51426,#51427,#51428,#51429,#51430,#51431,#51432,#51433,#51434,
#51435,#51436,#51437,#51438,#51439,#51440,#51441,#51442,#51443,#51444,#51445,
#51446,#51447,#51448,#51449,#51450,#51451,#51452,#51453,#51454,#51455,#51456,
#51457,#51458,#51459,#51460,#51461,#51462,#51463,#51464,#51465,#51466,#51467,
#51468,#51469,#51470,#51471,#51472,#51473,#51474),.UNSPECIFIED.,.F.,.F.)
B_SPLINE_CURVE_WITH_KNOTS((6,1,1,1,1,1,1,1,1,1,1,1,1,1,1,1,1,1,1,1,1,1,
1,1,1,1,1,1,1,1,1,1,1,1,1,1,1,1,1,1,1,1,1,1,1,1,1,1,1,1,1,1,1,1,1,1,1,1,
1,1,1,1,1,1,1,6),(-1.,-0.984615384615383,-0.969230769230768,-0.953846153846152,
-0.938461538461537,-0.923076923076922,-0.907692307692306,-0.892307692307691,
-0.876923076923076,-0.86153846153846,-0.846153846153845,-0.83076923076923,
-0.815384615384614,-0.799999999999999,-0.784615384615384,-0.769230769230768,
-0.753846153846153,-0.738461538461538,-0.723076923076922,-0.707692307692307,
-0.692307692307692,-0.676923076923076,-0.661538461538461,-0.646153846153846,
-0.63076923076923,-0.615384615384615,-0.6,-0.584615384615384,-0.569230769230769,
-0.553846153846154,-0.538461538461538,-0.523076923076923,-0.507692307692308,
-0.492307692307692,-0.476923076923077,-0.461538461538462,-0.446153846153846,
-0.430769230769231,-0.415384615384615,-0.4,-0.384615384615385,-0.369230769230769,
-0.353846153846154,-0.338461538461538,-0.323076923076923,-0.307692307692308,
-0.292307692307692,-0.276923076923077,-0.261538461538462,-0.246153846153846,
-0.230769230769231,-0.215384615384615,-0.2,-0.184615384615385,-0.169230769230769,
-0.153846153846154,-0.138461538461538,-0.123076923076923,-0.107692307692308,
-0.0923076923076923,-0.0769230769230769,-0.0615384615384615,-0.0461538461538462,
-0.0307692307692308,-0.0153846153846154,-0.00577184337448646),
 .UNSPECIFIED.)
CURVE()
GEOMETRIC_REPRESENTATION_ITEM()
RATIONAL_B_SPLINE_CURVE((1.,1.,1.,1.,1.,1.,1.,1.,1.,1.,1.,1.,1.,1.,1.,1.,
1.,1.,1.,1.,1.,1.,1.,1.,1.,1.,1.,1.,1.,1.,1.,1.,1.,1.,1.,1.,1.,1.,1.,1.,
1.,1.,1.,1.,1.,1.,1.,1.,1.,1.,1.,1.,1.,1.,1.,1.,1.,1.,1.,1.,1.,1.,1.,1.,
1.,1.,1.,1.,1.,1.))
REPRESENTATION_ITEM('')
);
#322=(
BOUNDED_CURVE()
B_SPLINE_CURVE(5,(#51625,#51626,#51627,#51628,#51629,#51630,#51631,#51632,
#51633,#51634,#51635,#51636,#51637,#51638,#51639,#51640,#51641,#51642,#51643,
#51644,#51645,#51646,#51647,#51648,#51649,#51650,#51651,#51652,#51653,#51654,
#51655,#51656,#51657,#51658,#51659,#51660,#51661,#51662,#51663,#51664,#51665,
#51666,#51667,#51668,#51669,#51670,#51671,#51672,#51673,#51674,#51675,#51676,
#51677,#51678,#51679,#51680,#51681,#51682,#51683,#51684,#51685,#51686,#51687,
#51688,#51689,#51690,#51691,#51692,#51693,#51694),.UNSPECIFIED.,.F.,.F.)
B_SPLINE_CURVE_WITH_KNOTS((6,1,1,1,1,1,1,1,1,1,1,1,1,1,1,1,1,1,1,1,1,1,
1,1,1,1,1,1,1,1,1,1,1,1,1,1,1,1,1,1,1,1,1,1,1,1,1,1,1,1,1,1,1,1,1,1,1,1,
1,1,1,1,1,1,1,6),(-0.994228156739708,-0.984615384615383,-0.969230769230768,
-0.953846153846152,-0.938461538461537,-0.923076923076922,-0.907692307692306,
-0.892307692307691,-0.876923076923076,-0.86153846153846,-0.846153846153845,
-0.83076923076923,-0.815384615384614,-0.799999999999999,-0.784615384615384,
-0.769230769230768,-0.753846153846153,-0.738461538461538,-0.723076923076922,
-0.707692307692307,-0.692307692307692,-0.676923076923076,-0.661538461538461,
-0.646153846153846,-0.63076923076923,-0.615384615384615,-0.6,-0.584615384615384,
-0.569230769230769,-0.553846153846154,-0.538461538461538,-0.523076923076923,
-0.507692307692308,-0.492307692307692,-0.476923076923077,-0.461538461538462,
-0.446153846153846,-0.430769230769231,-0.415384615384615,-0.4,-0.384615384615385,
-0.369230769230769,-0.353846153846154,-0.338461538461538,-0.323076923076923,
-0.307692307692308,-0.292307692307692,-0.276923076923077,-0.261538461538462,
-0.246153846153846,-0.230769230769231,-0.215384615384615,-0.2,-0.184615384615385,
-0.169230769230769,-0.153846153846154,-0.138461538461538,-0.123076923076923,
-0.107692307692308,-0.0923076923076923,-0.0769230769230769,-0.0615384615384615,
-0.0461538461538462,-0.0307692307692308,-0.0153846153846154,0.),
 .UNSPECIFIED.)
CURVE()
GEOMETRIC_REPRESENTATION_ITEM()
RATIONAL_B_SPLINE_CURVE((1.,1.,1.,1.,1.,1.,1.,1.,1.,1.,1.,1.,1.,1.,1.,1.,
1.,1.,1.,1.,1.,1.,1.,1.,1.,1.,1.,1.,1.,1.,1.,1.,1.,1.,1.,1.,1.,1.,1.,1.,
1.,1.,1.,1.,1.,1.,1.,1.,1.,1.,1.,1.,1.,1.,1.,1.,1.,1.,1.,1.,1.,1.,1.,1.,
1.,1.,1.,1.,1.,1.))
REPRESENTATION_ITEM('')
);
#323=(
BOUNDED_CURVE()
B_SPLINE_CURVE(5,(#51847,#51848,#51849,#51850,#51851,#51852,#51853,#51854,
#51855,#51856,#51857,#51858,#51859,#51860,#51861,#51862,#51863,#51864,#51865,
#51866,#51867,#51868,#51869,#51870,#51871,#51872,#51873,#51874,#51875,#51876,
#51877,#51878,#51879,#51880,#51881,#51882,#51883,#51884,#51885,#51886,#51887,
#51888,#51889,#51890,#51891,#51892,#51893,#51894,#51895,#51896,#51897,#51898,
#51899,#51900,#51901,#51902,#51903,#51904,#51905,#51906,#51907,#51908,#51909,
#51910,#51911,#51912,#51913,#51914,#51915,#51916),.UNSPECIFIED.,.F.,.F.)
B_SPLINE_CURVE_WITH_KNOTS((6,1,1,1,1,1,1,1,1,1,1,1,1,1,1,1,1,1,1,1,1,1,
1,1,1,1,1,1,1,1,1,1,1,1,1,1,1,1,1,1,1,1,1,1,1,1,1,1,1,1,1,1,1,1,1,1,1,1,
1,1,1,1,1,1,1,6),(-1.,-0.984615384615383,-0.969230769230768,-0.953846153846152,
-0.938461538461537,-0.923076923076922,-0.907692307692306,-0.892307692307691,
-0.876923076923076,-0.86153846153846,-0.846153846153845,-0.83076923076923,
-0.815384615384614,-0.799999999999999,-0.784615384615384,-0.769230769230768,
-0.753846153846153,-0.738461538461538,-0.723076923076922,-0.707692307692307,
-0.692307692307692,-0.676923076923076,-0.661538461538461,-0.646153846153846,
-0.63076923076923,-0.615384615384615,-0.6,-0.584615384615384,-0.569230769230769,
-0.553846153846154,-0.538461538461538,-0.523076923076923,-0.507692307692308,
-0.492307692307692,-0.476923076923077,-0.461538461538462,-0.446153846153846,
-0.430769230769231,-0.415384615384615,-0.4,-0.384615384615385,-0.369230769230769,
-0.353846153846154,-0.338461538461538,-0.323076923076923,-0.307692307692308,
-0.292307692307692,-0.276923076923077,-0.261538461538462,-0.246153846153846,
-0.230769230769231,-0.215384615384615,-0.2,-0.184615384615385,-0.169230769230769,
-0.153846153846154,-0.138461538461538,-0.123076923076923,-0.107692307692308,
-0.0923076923076923,-0.0769230769230769,-0.0615384615384615,-0.0461538461538462,
-0.0307692307692308,-0.0153846153846154,-0.00577184337451626),
 .UNSPECIFIED.)
CURVE()
GEOMETRIC_REPRESENTATION_ITEM()
RATIONAL_B_SPLINE_CURVE((1.,1.,1.,1.,1.,1.,1.,1.,1.,1.,1.,1.,1.,1.,1.,1.,
1.,1.,1.,1.,1.,1.,1.,1.,1.,1.,1.,1.,1.,1.,1.,1.,1.,1.,1.,1.,1.,1.,1.,1.,
1.,1.,1.,1.,1.,1.,1.,1.,1.,1.,1.,1.,1.,1.,1.,1.,1.,1.,1.,1.,1.,1.,1.,1.,
1.,1.,1.,1.,1.,1.))
REPRESENTATION_ITEM('')
);
#324=(
BOUNDED_CURVE()
B_SPLINE_CURVE(5,(#52067,#52068,#52069,#52070,#52071,#52072,#52073,#52074,
#52075,#52076,#52077,#52078,#52079,#52080,#52081,#52082,#52083,#52084,#52085,
#52086,#52087,#52088,#52089,#52090,#52091,#52092,#52093,#52094,#52095,#52096,
#52097,#52098,#52099,#52100,#52101,#52102,#52103,#52104,#52105,#52106,#52107,
#52108,#52109,#52110,#52111,#52112,#52113,#52114,#52115,#52116,#52117,#52118,
#52119,#52120,#52121,#52122,#52123,#52124,#52125,#52126,#52127,#52128,#52129,
#52130,#52131,#52132,#52133,#52134,#52135,#52136),.UNSPECIFIED.,.F.,.F.)
B_SPLINE_CURVE_WITH_KNOTS((6,1,1,1,1,1,1,1,1,1,1,1,1,1,1,1,1,1,1,1,1,1,
1,1,1,1,1,1,1,1,1,1,1,1,1,1,1,1,1,1,1,1,1,1,1,1,1,1,1,1,1,1,1,1,1,1,1,1,
1,1,1,1,1,1,1,6),(-0.994228156739708,-0.984615384615383,-0.969230769230768,
-0.953846153846152,-0.938461538461537,-0.923076923076922,-0.907692307692306,
-0.892307692307691,-0.876923076923076,-0.86153846153846,-0.846153846153845,
-0.83076923076923,-0.815384615384614,-0.799999999999999,-0.784615384615384,
-0.769230769230768,-0.753846153846153,-0.738461538461538,-0.723076923076922,
-0.707692307692307,-0.692307692307692,-0.676923076923076,-0.661538461538461,
-0.646153846153846,-0.63076923076923,-0.615384615384615,-0.6,-0.584615384615384,
-0.569230769230769,-0.553846153846154,-0.538461538461538,-0.523076923076923,
-0.507692307692308,-0.492307692307692,-0.476923076923077,-0.461538461538462,
-0.446153846153846,-0.430769230769231,-0.415384615384615,-0.4,-0.384615384615385,
-0.369230769230769,-0.353846153846154,-0.338461538461538,-0.323076923076923,
-0.307692307692308,-0.292307692307692,-0.276923076923077,-0.261538461538462,
-0.246153846153846,-0.230769230769231,-0.215384615384615,-0.2,-0.184615384615385,
-0.169230769230769,-0.153846153846154,-0.138461538461538,-0.123076923076923,
-0.107692307692308,-0.0923076923076923,-0.0769230769230769,-0.0615384615384615,
-0.0461538461538462,-0.0307692307692308,-0.0153846153846154,0.),
 .UNSPECIFIED.)
CURVE()
GEOMETRIC_REPRESENTATION_ITEM()
RATIONAL_B_SPLINE_CURVE((1.,1.,1.,1.,1.,1.,1.,1.,1.,1.,1.,1.,1.,1.,1.,1.,
1.,1.,1.,1.,1.,1.,1.,1.,1.,1.,1.,1.,1.,1.,1.,1.,1.,1.,1.,1.,1.,1.,1.,1.,
1.,1.,1.,1.,1.,1.,1.,1.,1.,1.,1.,1.,1.,1.,1.,1.,1.,1.,1.,1.,1.,1.,1.,1.,
1.,1.,1.,1.,1.,1.))
REPRESENTATION_ITEM('')
);
#325=(
BOUNDED_CURVE()
B_SPLINE_CURVE(5,(#52289,#52290,#52291,#52292,#52293,#52294,#52295,#52296,
#52297,#52298,#52299,#52300,#52301,#52302,#52303,#52304,#52305,#52306,#52307,
#52308,#52309,#52310,#52311,#52312,#52313,#52314,#52315,#52316,#52317,#52318,
#52319,#52320,#52321,#52322,#52323,#52324,#52325,#52326,#52327,#52328,#52329,
#52330,#52331,#52332,#52333,#52334,#52335,#52336,#52337,#52338,#52339,#52340,
#52341,#52342,#52343,#52344,#52345,#52346,#52347,#52348,#52349,#52350,#52351,
#52352,#52353,#52354,#52355,#52356,#52357,#52358),.UNSPECIFIED.,.F.,.F.)
B_SPLINE_CURVE_WITH_KNOTS((6,1,1,1,1,1,1,1,1,1,1,1,1,1,1,1,1,1,1,1,1,1,
1,1,1,1,1,1,1,1,1,1,1,1,1,1,1,1,1,1,1,1,1,1,1,1,1,1,1,1,1,1,1,1,1,1,1,1,
1,1,1,1,1,1,1,6),(-1.,-0.984615384615383,-0.969230769230768,-0.953846153846152,
-0.938461538461537,-0.923076923076922,-0.907692307692306,-0.892307692307691,
-0.876923076923076,-0.86153846153846,-0.846153846153845,-0.83076923076923,
-0.815384615384614,-0.799999999999999,-0.784615384615384,-0.769230769230768,
-0.753846153846153,-0.738461538461538,-0.723076923076922,-0.707692307692307,
-0.692307692307692,-0.676923076923076,-0.661538461538461,-0.646153846153846,
-0.63076923076923,-0.615384615384615,-0.6,-0.584615384615384,-0.569230769230769,
-0.553846153846154,-0.538461538461538,-0.523076923076923,-0.507692307692308,
-0.492307692307692,-0.476923076923077,-0.461538461538462,-0.446153846153846,
-0.430769230769231,-0.415384615384615,-0.4,-0.384615384615385,-0.369230769230769,
-0.353846153846154,-0.338461538461538,-0.323076923076923,-0.307692307692308,
-0.292307692307692,-0.276923076923077,-0.261538461538462,-0.246153846153846,
-0.230769230769231,-0.215384615384615,-0.2,-0.184615384615385,-0.169230769230769,
-0.153846153846154,-0.138461538461538,-0.123076923076923,-0.107692307692308,
-0.0923076923076923,-0.0769230769230769,-0.0615384615384615,-0.0461538461538462,
-0.0307692307692308,-0.0153846153846154,-0.00577184337451372),
 .UNSPECIFIED.)
CURVE()
GEOMETRIC_REPRESENTATION_ITEM()
RATIONAL_B_SPLINE_CURVE((1.,1.,1.,1.,1.,1.,1.,1.,1.,1.,1.,1.,1.,1.,1.,1.,
1.,1.,1.,1.,1.,1.,1.,1.,1.,1.,1.,1.,1.,1.,1.,1.,1.,1.,1.,1.,1.,1.,1.,1.,
1.,1.,1.,1.,1.,1.,1.,1.,1.,1.,1.,1.,1.,1.,1.,1.,1.,1.,1.,1.,1.,1.,1.,1.,
1.,1.,1.,1.,1.,1.))
REPRESENTATION_ITEM('')
);
#326=(
BOUNDED_CURVE()
B_SPLINE_CURVE(5,(#52509,#52510,#52511,#52512,#52513,#52514,#52515,#52516,
#52517,#52518,#52519,#52520,#52521,#52522,#52523,#52524,#52525,#52526,#52527,
#52528,#52529,#52530,#52531,#52532,#52533,#52534,#52535,#52536,#52537,#52538,
#52539,#52540,#52541,#52542,#52543,#52544,#52545,#52546,#52547,#52548,#52549,
#52550,#52551,#52552,#52553,#52554,#52555,#52556,#52557,#52558,#52559,#52560,
#52561,#52562,#52563,#52564,#52565,#52566,#52567,#52568,#52569,#52570,#52571,
#52572,#52573,#52574,#52575,#52576,#52577,#52578),.UNSPECIFIED.,.F.,.F.)
B_SPLINE_CURVE_WITH_KNOTS((6,1,1,1,1,1,1,1,1,1,1,1,1,1,1,1,1,1,1,1,1,1,
1,1,1,1,1,1,1,1,1,1,1,1,1,1,1,1,1,1,1,1,1,1,1,1,1,1,1,1,1,1,1,1,1,1,1,1,
1,1,1,1,1,1,1,6),(-0.994228156739703,-0.984615384615383,-0.969230769230768,
-0.953846153846152,-0.938461538461537,-0.923076923076922,-0.907692307692306,
-0.892307692307691,-0.876923076923076,-0.86153846153846,-0.846153846153845,
-0.83076923076923,-0.815384615384614,-0.799999999999999,-0.784615384615384,
-0.769230769230768,-0.753846153846153,-0.738461538461538,-0.723076923076922,
-0.707692307692307,-0.692307692307692,-0.676923076923076,-0.661538461538461,
-0.646153846153846,-0.63076923076923,-0.615384615384615,-0.6,-0.584615384615384,
-0.569230769230769,-0.553846153846154,-0.538461538461538,-0.523076923076923,
-0.507692307692308,-0.492307692307692,-0.476923076923077,-0.461538461538462,
-0.446153846153846,-0.430769230769231,-0.415384615384615,-0.4,-0.384615384615385,
-0.369230769230769,-0.353846153846154,-0.338461538461538,-0.323076923076923,
-0.307692307692308,-0.292307692307692,-0.276923076923077,-0.261538461538462,
-0.246153846153846,-0.230769230769231,-0.215384615384615,-0.2,-0.184615384615385,
-0.169230769230769,-0.153846153846154,-0.138461538461538,-0.123076923076923,
-0.107692307692308,-0.0923076923076923,-0.0769230769230769,-0.0615384615384615,
-0.0461538461538462,-0.0307692307692308,-0.0153846153846154,0.),
 .UNSPECIFIED.)
CURVE()
GEOMETRIC_REPRESENTATION_ITEM()
RATIONAL_B_SPLINE_CURVE((1.,1.,1.,1.,1.,1.,1.,1.,1.,1.,1.,1.,1.,1.,1.,1.,
1.,1.,1.,1.,1.,1.,1.,1.,1.,1.,1.,1.,1.,1.,1.,1.,1.,1.,1.,1.,1.,1.,1.,1.,
1.,1.,1.,1.,1.,1.,1.,1.,1.,1.,1.,1.,1.,1.,1.,1.,1.,1.,1.,1.,1.,1.,1.,1.,
1.,1.,1.,1.,1.,1.))
REPRESENTATION_ITEM('')
);
#327=(
BOUNDED_CURVE()
B_SPLINE_CURVE(5,(#52731,#52732,#52733,#52734,#52735,#52736,#52737,#52738,
#52739,#52740,#52741,#52742,#52743,#52744,#52745,#52746,#52747,#52748,#52749,
#52750,#52751,#52752,#52753,#52754,#52755,#52756,#52757,#52758,#52759,#52760,
#52761,#52762,#52763,#52764,#52765,#52766,#52767,#52768,#52769,#52770,#52771,
#52772,#52773,#52774,#52775,#52776,#52777,#52778,#52779,#52780,#52781,#52782,
#52783,#52784,#52785,#52786,#52787,#52788,#52789,#52790,#52791,#52792,#52793,
#52794,#52795,#52796,#52797,#52798,#52799,#52800),.UNSPECIFIED.,.F.,.F.)
B_SPLINE_CURVE_WITH_KNOTS((6,1,1,1,1,1,1,1,1,1,1,1,1,1,1,1,1,1,1,1,1,1,
1,1,1,1,1,1,1,1,1,1,1,1,1,1,1,1,1,1,1,1,1,1,1,1,1,1,1,1,1,1,1,1,1,1,1,1,
1,1,1,1,1,1,1,6),(-1.,-0.984615384615383,-0.969230769230768,-0.953846153846152,
-0.938461538461537,-0.923076923076922,-0.907692307692306,-0.892307692307691,
-0.876923076923076,-0.86153846153846,-0.846153846153845,-0.83076923076923,
-0.815384615384614,-0.799999999999999,-0.784615384615384,-0.769230769230768,
-0.753846153846153,-0.738461538461538,-0.723076923076922,-0.707692307692307,
-0.692307692307692,-0.676923076923076,-0.661538461538461,-0.646153846153846,
-0.63076923076923,-0.615384615384615,-0.6,-0.584615384615384,-0.569230769230769,
-0.553846153846154,-0.538461538461538,-0.523076923076923,-0.507692307692308,
-0.492307692307692,-0.476923076923077,-0.461538461538462,-0.446153846153846,
-0.430769230769231,-0.415384615384615,-0.4,-0.384615384615385,-0.369230769230769,
-0.353846153846154,-0.338461538461538,-0.323076923076923,-0.307692307692308,
-0.292307692307692,-0.276923076923077,-0.261538461538462,-0.246153846153846,
-0.230769230769231,-0.215384615384615,-0.2,-0.184615384615385,-0.169230769230769,
-0.153846153846154,-0.138461538461538,-0.123076923076923,-0.107692307692308,
-0.0923076923076923,-0.0769230769230769,-0.0615384615384615,-0.0461538461538462,
-0.0307692307692308,-0.0153846153846154,-0.00577184337451698),
 .UNSPECIFIED.)
CURVE()
GEOMETRIC_REPRESENTATION_ITEM()
RATIONAL_B_SPLINE_CURVE((1.,1.,1.,1.,1.,1.,1.,1.,1.,1.,1.,1.,1.,1.,1.,1.,
1.,1.,1.,1.,1.,1.,1.,1.,1.,1.,1.,1.,1.,1.,1.,1.,1.,1.,1.,1.,1.,1.,1.,1.,
1.,1.,1.,1.,1.,1.,1.,1.,1.,1.,1.,1.,1.,1.,1.,1.,1.,1.,1.,1.,1.,1.,1.,1.,
1.,1.,1.,1.,1.,1.))
REPRESENTATION_ITEM('')
);
#328=(
BOUNDED_CURVE()
B_SPLINE_CURVE(5,(#52951,#52952,#52953,#52954,#52955,#52956,#52957,#52958,
#52959,#52960,#52961,#52962,#52963,#52964,#52965,#52966,#52967,#52968,#52969,
#52970,#52971,#52972,#52973,#52974,#52975,#52976,#52977,#52978,#52979,#52980,
#52981,#52982,#52983,#52984,#52985,#52986,#52987,#52988,#52989,#52990,#52991,
#52992,#52993,#52994,#52995,#52996,#52997,#52998,#52999,#53000,#53001,#53002,
#53003,#53004,#53005,#53006,#53007,#53008,#53009,#53010,#53011,#53012,#53013,
#53014,#53015,#53016,#53017,#53018,#53019,#53020),.UNSPECIFIED.,.F.,.F.)
B_SPLINE_CURVE_WITH_KNOTS((6,1,1,1,1,1,1,1,1,1,1,1,1,1,1,1,1,1,1,1,1,1,
1,1,1,1,1,1,1,1,1,1,1,1,1,1,1,1,1,1,1,1,1,1,1,1,1,1,1,1,1,1,1,1,1,1,1,1,
1,1,1,1,1,1,1,6),(-0.994228156739706,-0.984615384615383,-0.969230769230768,
-0.953846153846152,-0.938461538461537,-0.923076923076922,-0.907692307692306,
-0.892307692307691,-0.876923076923076,-0.86153846153846,-0.846153846153845,
-0.83076923076923,-0.815384615384614,-0.799999999999999,-0.784615384615384,
-0.769230769230768,-0.753846153846153,-0.738461538461538,-0.723076923076922,
-0.707692307692307,-0.692307692307692,-0.676923076923076,-0.661538461538461,
-0.646153846153846,-0.63076923076923,-0.615384615384615,-0.6,-0.584615384615384,
-0.569230769230769,-0.553846153846154,-0.538461538461538,-0.523076923076923,
-0.507692307692308,-0.492307692307692,-0.476923076923077,-0.461538461538462,
-0.446153846153846,-0.430769230769231,-0.415384615384615,-0.4,-0.384615384615385,
-0.369230769230769,-0.353846153846154,-0.338461538461538,-0.323076923076923,
-0.307692307692308,-0.292307692307692,-0.276923076923077,-0.261538461538462,
-0.246153846153846,-0.230769230769231,-0.215384615384615,-0.2,-0.184615384615385,
-0.169230769230769,-0.153846153846154,-0.138461538461538,-0.123076923076923,
-0.107692307692308,-0.0923076923076923,-0.0769230769230769,-0.0615384615384615,
-0.0461538461538462,-0.0307692307692308,-0.0153846153846154,0.),
 .UNSPECIFIED.)
CURVE()
GEOMETRIC_REPRESENTATION_ITEM()
RATIONAL_B_SPLINE_CURVE((1.,1.,1.,1.,1.,1.,1.,1.,1.,1.,1.,1.,1.,1.,1.,1.,
1.,1.,1.,1.,1.,1.,1.,1.,1.,1.,1.,1.,1.,1.,1.,1.,1.,1.,1.,1.,1.,1.,1.,1.,
1.,1.,1.,1.,1.,1.,1.,1.,1.,1.,1.,1.,1.,1.,1.,1.,1.,1.,1.,1.,1.,1.,1.,1.,
1.,1.,1.,1.,1.,1.))
REPRESENTATION_ITEM('')
);
#329=(
BOUNDED_CURVE()
B_SPLINE_CURVE(5,(#53173,#53174,#53175,#53176,#53177,#53178,#53179,#53180,
#53181,#53182,#53183,#53184,#53185,#53186,#53187,#53188,#53189,#53190,#53191,
#53192,#53193,#53194,#53195,#53196,#53197,#53198,#53199,#53200,#53201,#53202,
#53203,#53204,#53205,#53206,#53207,#53208,#53209,#53210,#53211,#53212,#53213,
#53214,#53215,#53216,#53217,#53218,#53219,#53220,#53221,#53222,#53223,#53224,
#53225,#53226,#53227,#53228,#53229,#53230,#53231,#53232,#53233,#53234,#53235,
#53236,#53237,#53238,#53239,#53240,#53241,#53242),.UNSPECIFIED.,.F.,.F.)
B_SPLINE_CURVE_WITH_KNOTS((6,1,1,1,1,1,1,1,1,1,1,1,1,1,1,1,1,1,1,1,1,1,
1,1,1,1,1,1,1,1,1,1,1,1,1,1,1,1,1,1,1,1,1,1,1,1,1,1,1,1,1,1,1,1,1,1,1,1,
1,1,1,1,1,1,1,6),(-1.,-0.984615384615383,-0.969230769230768,-0.953846153846152,
-0.938461538461537,-0.923076923076922,-0.907692307692306,-0.892307692307691,
-0.876923076923076,-0.86153846153846,-0.846153846153845,-0.83076923076923,
-0.815384615384614,-0.799999999999999,-0.784615384615384,-0.769230769230768,
-0.753846153846153,-0.738461538461538,-0.723076923076922,-0.707692307692307,
-0.692307692307692,-0.676923076923076,-0.661538461538461,-0.646153846153846,
-0.63076923076923,-0.615384615384615,-0.6,-0.584615384615384,-0.569230769230769,
-0.553846153846154,-0.538461538461538,-0.523076923076923,-0.507692307692308,
-0.492307692307692,-0.476923076923077,-0.461538461538462,-0.446153846153846,
-0.430769230769231,-0.415384615384615,-0.4,-0.384615384615385,-0.369230769230769,
-0.353846153846154,-0.338461538461538,-0.323076923076923,-0.307692307692308,
-0.292307692307692,-0.276923076923077,-0.261538461538462,-0.246153846153846,
-0.230769230769231,-0.215384615384615,-0.2,-0.184615384615385,-0.169230769230769,
-0.153846153846154,-0.138461538461538,-0.123076923076923,-0.107692307692308,
-0.0923076923076923,-0.0769230769230769,-0.0615384615384615,-0.0461538461538462,
-0.0307692307692308,-0.0153846153846154,-0.00577184337452512),
 .UNSPECIFIED.)
CURVE()
GEOMETRIC_REPRESENTATION_ITEM()
RATIONAL_B_SPLINE_CURVE((1.,1.,1.,1.,1.,1.,1.,1.,1.,1.,1.,1.,1.,1.,1.,1.,
1.,1.,1.,1.,1.,1.,1.,1.,1.,1.,1.,1.,1.,1.,1.,1.,1.,1.,1.,1.,1.,1.,1.,1.,
1.,1.,1.,1.,1.,1.,1.,1.,1.,1.,1.,1.,1.,1.,1.,1.,1.,1.,1.,1.,1.,1.,1.,1.,
1.,1.,1.,1.,1.,1.))
REPRESENTATION_ITEM('')
);
#330=(
BOUNDED_CURVE()
B_SPLINE_CURVE(5,(#53393,#53394,#53395,#53396,#53397,#53398,#53399,#53400,
#53401,#53402,#53403,#53404,#53405,#53406,#53407,#53408,#53409,#53410,#53411,
#53412,#53413,#53414,#53415,#53416,#53417,#53418,#53419,#53420,#53421,#53422,
#53423,#53424,#53425,#53426,#53427,#53428,#53429,#53430,#53431,#53432,#53433,
#53434,#53435,#53436,#53437,#53438,#53439,#53440,#53441,#53442,#53443,#53444,
#53445,#53446,#53447,#53448,#53449,#53450,#53451,#53452,#53453,#53454,#53455,
#53456,#53457,#53458,#53459,#53460,#53461,#53462),.UNSPECIFIED.,.F.,.F.)
B_SPLINE_CURVE_WITH_KNOTS((6,1,1,1,1,1,1,1,1,1,1,1,1,1,1,1,1,1,1,1,1,1,
1,1,1,1,1,1,1,1,1,1,1,1,1,1,1,1,1,1,1,1,1,1,1,1,1,1,1,1,1,1,1,1,1,1,1,1,
1,1,1,1,1,1,1,6),(-0.994228156739713,-0.984615384615383,-0.969230769230768,
-0.953846153846152,-0.938461538461537,-0.923076923076922,-0.907692307692306,
-0.892307692307691,-0.876923076923076,-0.86153846153846,-0.846153846153845,
-0.83076923076923,-0.815384615384614,-0.799999999999999,-0.784615384615384,
-0.769230769230768,-0.753846153846153,-0.738461538461538,-0.723076923076922,
-0.707692307692307,-0.692307692307692,-0.676923076923076,-0.661538461538461,
-0.646153846153846,-0.63076923076923,-0.615384615384615,-0.6,-0.584615384615384,
-0.569230769230769,-0.553846153846154,-0.538461538461538,-0.523076923076923,
-0.507692307692308,-0.492307692307692,-0.476923076923077,-0.461538461538462,
-0.446153846153846,-0.430769230769231,-0.415384615384615,-0.4,-0.384615384615385,
-0.369230769230769,-0.353846153846154,-0.338461538461538,-0.323076923076923,
-0.307692307692308,-0.292307692307692,-0.276923076923077,-0.261538461538462,
-0.246153846153846,-0.230769230769231,-0.215384615384615,-0.2,-0.184615384615385,
-0.169230769230769,-0.153846153846154,-0.138461538461538,-0.123076923076923,
-0.107692307692308,-0.0923076923076923,-0.0769230769230769,-0.0615384615384615,
-0.0461538461538462,-0.0307692307692308,-0.0153846153846154,0.),
 .UNSPECIFIED.)
CURVE()
GEOMETRIC_REPRESENTATION_ITEM()
RATIONAL_B_SPLINE_CURVE((1.,1.,1.,1.,1.,1.,1.,1.,1.,1.,1.,1.,1.,1.,1.,1.,
1.,1.,1.,1.,1.,1.,1.,1.,1.,1.,1.,1.,1.,1.,1.,1.,1.,1.,1.,1.,1.,1.,1.,1.,
1.,1.,1.,1.,1.,1.,1.,1.,1.,1.,1.,1.,1.,1.,1.,1.,1.,1.,1.,1.,1.,1.,1.,1.,
1.,1.,1.,1.,1.,1.))
REPRESENTATION_ITEM('')
);
#331=(
BOUNDED_CURVE()
B_SPLINE_CURVE(5,(#53615,#53616,#53617,#53618,#53619,#53620,#53621,#53622,
#53623,#53624,#53625,#53626,#53627,#53628,#53629,#53630,#53631,#53632,#53633,
#53634,#53635,#53636,#53637,#53638,#53639,#53640,#53641,#53642,#53643,#53644,
#53645,#53646,#53647,#53648,#53649,#53650,#53651,#53652,#53653,#53654,#53655,
#53656,#53657,#53658,#53659,#53660,#53661,#53662,#53663,#53664,#53665,#53666,
#53667,#53668,#53669,#53670,#53671,#53672,#53673,#53674,#53675,#53676,#53677,
#53678,#53679,#53680,#53681,#53682,#53683,#53684),.UNSPECIFIED.,.F.,.F.)
B_SPLINE_CURVE_WITH_KNOTS((6,1,1,1,1,1,1,1,1,1,1,1,1,1,1,1,1,1,1,1,1,1,
1,1,1,1,1,1,1,1,1,1,1,1,1,1,1,1,1,1,1,1,1,1,1,1,1,1,1,1,1,1,1,1,1,1,1,1,
1,1,1,1,1,1,1,6),(-1.,-0.984615384615383,-0.969230769230768,-0.953846153846152,
-0.938461538461537,-0.923076923076922,-0.907692307692306,-0.892307692307691,
-0.876923076923076,-0.86153846153846,-0.846153846153845,-0.83076923076923,
-0.815384615384614,-0.799999999999999,-0.784615384615384,-0.769230769230768,
-0.753846153846153,-0.738461538461538,-0.723076923076922,-0.707692307692307,
-0.692307692307692,-0.676923076923076,-0.661538461538461,-0.646153846153846,
-0.63076923076923,-0.615384615384615,-0.6,-0.584615384615384,-0.569230769230769,
-0.553846153846154,-0.538461538461538,-0.523076923076923,-0.507692307692308,
-0.492307692307692,-0.476923076923077,-0.461538461538462,-0.446153846153846,
-0.430769230769231,-0.415384615384615,-0.4,-0.384615384615385,-0.369230769230769,
-0.353846153846154,-0.338461538461538,-0.323076923076923,-0.307692307692308,
-0.292307692307692,-0.276923076923077,-0.261538461538462,-0.246153846153846,
-0.230769230769231,-0.215384615384615,-0.2,-0.184615384615385,-0.169230769230769,
-0.153846153846154,-0.138461538461538,-0.123076923076923,-0.107692307692308,
-0.0923076923076923,-0.0769230769230769,-0.0615384615384615,-0.0461538461538462,
-0.0307692307692308,-0.0153846153846154,-0.00577184337450204),
 .UNSPECIFIED.)
CURVE()
GEOMETRIC_REPRESENTATION_ITEM()
RATIONAL_B_SPLINE_CURVE((1.,1.,1.,1.,1.,1.,1.,1.,1.,1.,1.,1.,1.,1.,1.,1.,
1.,1.,1.,1.,1.,1.,1.,1.,1.,1.,1.,1.,1.,1.,1.,1.,1.,1.,1.,1.,1.,1.,1.,1.,
1.,1.,1.,1.,1.,1.,1.,1.,1.,1.,1.,1.,1.,1.,1.,1.,1.,1.,1.,1.,1.,1.,1.,1.,
1.,1.,1.,1.,1.,1.))
REPRESENTATION_ITEM('')
);
#332=(
BOUNDED_CURVE()
B_SPLINE_CURVE(5,(#53835,#53836,#53837,#53838,#53839,#53840,#53841,#53842,
#53843,#53844,#53845,#53846,#53847,#53848,#53849,#53850,#53851,#53852,#53853,
#53854,#53855,#53856,#53857,#53858,#53859,#53860,#53861,#53862,#53863,#53864,
#53865,#53866,#53867,#53868,#53869,#53870,#53871,#53872,#53873,#53874,#53875,
#53876,#53877,#53878,#53879,#53880,#53881,#53882,#53883,#53884,#53885,#53886,
#53887,#53888,#53889,#53890,#53891,#53892,#53893,#53894,#53895,#53896,#53897,
#53898,#53899,#53900,#53901,#53902,#53903,#53904),.UNSPECIFIED.,.F.,.F.)
B_SPLINE_CURVE_WITH_KNOTS((6,1,1,1,1,1,1,1,1,1,1,1,1,1,1,1,1,1,1,1,1,1,
1,1,1,1,1,1,1,1,1,1,1,1,1,1,1,1,1,1,1,1,1,1,1,1,1,1,1,1,1,1,1,1,1,1,1,1,
1,1,1,1,1,1,1,6),(-0.99422815673972,-0.984615384615383,-0.969230769230768,
-0.953846153846152,-0.938461538461537,-0.923076923076922,-0.907692307692306,
-0.892307692307691,-0.876923076923076,-0.86153846153846,-0.846153846153845,
-0.83076923076923,-0.815384615384614,-0.799999999999999,-0.784615384615384,
-0.769230769230768,-0.753846153846153,-0.738461538461538,-0.723076923076922,
-0.707692307692307,-0.692307692307692,-0.676923076923076,-0.661538461538461,
-0.646153846153846,-0.63076923076923,-0.615384615384615,-0.6,-0.584615384615384,
-0.569230769230769,-0.553846153846154,-0.538461538461538,-0.523076923076923,
-0.507692307692308,-0.492307692307692,-0.476923076923077,-0.461538461538462,
-0.446153846153846,-0.430769230769231,-0.415384615384615,-0.4,-0.384615384615385,
-0.369230769230769,-0.353846153846154,-0.338461538461538,-0.323076923076923,
-0.307692307692308,-0.292307692307692,-0.276923076923077,-0.261538461538462,
-0.246153846153846,-0.230769230769231,-0.215384615384615,-0.2,-0.184615384615385,
-0.169230769230769,-0.153846153846154,-0.138461538461538,-0.123076923076923,
-0.107692307692308,-0.0923076923076923,-0.0769230769230769,-0.0615384615384615,
-0.0461538461538462,-0.0307692307692308,-0.0153846153846154,0.),
 .UNSPECIFIED.)
CURVE()
GEOMETRIC_REPRESENTATION_ITEM()
RATIONAL_B_SPLINE_CURVE((1.,1.,1.,1.,1.,1.,1.,1.,1.,1.,1.,1.,1.,1.,1.,1.,
1.,1.,1.,1.,1.,1.,1.,1.,1.,1.,1.,1.,1.,1.,1.,1.,1.,1.,1.,1.,1.,1.,1.,1.,
1.,1.,1.,1.,1.,1.,1.,1.,1.,1.,1.,1.,1.,1.,1.,1.,1.,1.,1.,1.,1.,1.,1.,1.,
1.,1.,1.,1.,1.,1.))
REPRESENTATION_ITEM('')
);
#333=(
BOUNDED_CURVE()
B_SPLINE_CURVE(5,(#54057,#54058,#54059,#54060,#54061,#54062,#54063,#54064,
#54065,#54066,#54067,#54068,#54069,#54070,#54071,#54072,#54073,#54074,#54075,
#54076,#54077,#54078,#54079,#54080,#54081,#54082,#54083,#54084,#54085,#54086,
#54087,#54088,#54089,#54090,#54091,#54092,#54093,#54094,#54095,#54096,#54097,
#54098,#54099,#54100,#54101,#54102,#54103,#54104,#54105,#54106,#54107,#54108,
#54109,#54110,#54111,#54112,#54113,#54114,#54115,#54116,#54117,#54118,#54119,
#54120,#54121,#54122,#54123,#54124,#54125,#54126),.UNSPECIFIED.,.F.,.F.)
B_SPLINE_CURVE_WITH_KNOTS((6,1,1,1,1,1,1,1,1,1,1,1,1,1,1,1,1,1,1,1,1,1,
1,1,1,1,1,1,1,1,1,1,1,1,1,1,1,1,1,1,1,1,1,1,1,1,1,1,1,1,1,1,1,1,1,1,1,1,
1,1,1,1,1,1,1,6),(-1.,-0.984615384615383,-0.969230769230768,-0.953846153846152,
-0.938461538461537,-0.923076923076922,-0.907692307692306,-0.892307692307691,
-0.876923076923076,-0.86153846153846,-0.846153846153845,-0.83076923076923,
-0.815384615384614,-0.799999999999999,-0.784615384615384,-0.769230769230768,
-0.753846153846153,-0.738461538461538,-0.723076923076922,-0.707692307692307,
-0.692307692307692,-0.676923076923076,-0.661538461538461,-0.646153846153846,
-0.63076923076923,-0.615384615384615,-0.6,-0.584615384615384,-0.569230769230769,
-0.553846153846154,-0.538461538461538,-0.523076923076923,-0.507692307692308,
-0.492307692307692,-0.476923076923077,-0.461538461538462,-0.446153846153846,
-0.430769230769231,-0.415384615384615,-0.4,-0.384615384615385,-0.369230769230769,
-0.353846153846154,-0.338461538461538,-0.323076923076923,-0.307692307692308,
-0.292307692307692,-0.276923076923077,-0.261538461538462,-0.246153846153846,
-0.230769230769231,-0.215384615384615,-0.2,-0.184615384615385,-0.169230769230769,
-0.153846153846154,-0.138461538461538,-0.123076923076923,-0.107692307692308,
-0.0923076923076923,-0.0769230769230769,-0.0615384615384615,-0.0461538461538462,
-0.0307692307692308,-0.0153846153846154,-0.0057718433745107),
 .UNSPECIFIED.)
CURVE()
GEOMETRIC_REPRESENTATION_ITEM()
RATIONAL_B_SPLINE_CURVE((1.,1.,1.,1.,1.,1.,1.,1.,1.,1.,1.,1.,1.,1.,1.,1.,
1.,1.,1.,1.,1.,1.,1.,1.,1.,1.,1.,1.,1.,1.,1.,1.,1.,1.,1.,1.,1.,1.,1.,1.,
1.,1.,1.,1.,1.,1.,1.,1.,1.,1.,1.,1.,1.,1.,1.,1.,1.,1.,1.,1.,1.,1.,1.,1.,
1.,1.,1.,1.,1.,1.))
REPRESENTATION_ITEM('')
);
#334=(
BOUNDED_CURVE()
B_SPLINE_CURVE(5,(#54277,#54278,#54279,#54280,#54281,#54282,#54283,#54284,
#54285,#54286,#54287,#54288,#54289,#54290,#54291,#54292,#54293,#54294,#54295,
#54296,#54297,#54298,#54299,#54300,#54301,#54302,#54303,#54304,#54305,#54306,
#54307,#54308,#54309,#54310,#54311,#54312,#54313,#54314,#54315,#54316,#54317,
#54318,#54319,#54320,#54321,#54322,#54323,#54324,#54325,#54326,#54327,#54328,
#54329,#54330,#54331,#54332,#54333,#54334,#54335,#54336,#54337,#54338,#54339,
#54340,#54341,#54342,#54343,#54344,#54345,#54346),.UNSPECIFIED.,.F.,.F.)
B_SPLINE_CURVE_WITH_KNOTS((6,1,1,1,1,1,1,1,1,1,1,1,1,1,1,1,1,1,1,1,1,1,
1,1,1,1,1,1,1,1,1,1,1,1,1,1,1,1,1,1,1,1,1,1,1,1,1,1,1,1,1,1,1,1,1,1,1,1,
1,1,1,1,1,1,1,6),(-0.994228156739708,-0.984615384615383,-0.969230769230768,
-0.953846153846152,-0.938461538461537,-0.923076923076922,-0.907692307692306,
-0.892307692307691,-0.876923076923076,-0.86153846153846,-0.846153846153845,
-0.83076923076923,-0.815384615384614,-0.799999999999999,-0.784615384615384,
-0.769230769230768,-0.753846153846153,-0.738461538461538,-0.723076923076922,
-0.707692307692307,-0.692307692307692,-0.676923076923076,-0.661538461538461,
-0.646153846153846,-0.63076923076923,-0.615384615384615,-0.6,-0.584615384615384,
-0.569230769230769,-0.553846153846154,-0.538461538461538,-0.523076923076923,
-0.507692307692308,-0.492307692307692,-0.476923076923077,-0.461538461538462,
-0.446153846153846,-0.430769230769231,-0.415384615384615,-0.4,-0.384615384615385,
-0.369230769230769,-0.353846153846154,-0.338461538461538,-0.323076923076923,
-0.307692307692308,-0.292307692307692,-0.276923076923077,-0.261538461538462,
-0.246153846153846,-0.230769230769231,-0.215384615384615,-0.2,-0.184615384615385,
-0.169230769230769,-0.153846153846154,-0.138461538461538,-0.123076923076923,
-0.107692307692308,-0.0923076923076923,-0.0769230769230769,-0.0615384615384615,
-0.0461538461538462,-0.0307692307692308,-0.0153846153846154,0.),
 .UNSPECIFIED.)
CURVE()
GEOMETRIC_REPRESENTATION_ITEM()
RATIONAL_B_SPLINE_CURVE((1.,1.,1.,1.,1.,1.,1.,1.,1.,1.,1.,1.,1.,1.,1.,1.,
1.,1.,1.,1.,1.,1.,1.,1.,1.,1.,1.,1.,1.,1.,1.,1.,1.,1.,1.,1.,1.,1.,1.,1.,
1.,1.,1.,1.,1.,1.,1.,1.,1.,1.,1.,1.,1.,1.,1.,1.,1.,1.,1.,1.,1.,1.,1.,1.,
1.,1.,1.,1.,1.,1.))
REPRESENTATION_ITEM('')
);
#335=(
BOUNDED_CURVE()
B_SPLINE_CURVE(5,(#54499,#54500,#54501,#54502,#54503,#54504,#54505,#54506,
#54507,#54508,#54509,#54510,#54511,#54512,#54513,#54514,#54515,#54516,#54517,
#54518,#54519,#54520,#54521,#54522,#54523,#54524,#54525,#54526,#54527,#54528,
#54529,#54530,#54531,#54532,#54533,#54534,#54535,#54536,#54537,#54538,#54539,
#54540,#54541,#54542,#54543,#54544,#54545,#54546,#54547,#54548,#54549,#54550,
#54551,#54552,#54553,#54554,#54555,#54556,#54557,#54558,#54559,#54560,#54561,
#54562,#54563,#54564,#54565,#54566,#54567,#54568),.UNSPECIFIED.,.F.,.F.)
B_SPLINE_CURVE_WITH_KNOTS((6,1,1,1,1,1,1,1,1,1,1,1,1,1,1,1,1,1,1,1,1,1,
1,1,1,1,1,1,1,1,1,1,1,1,1,1,1,1,1,1,1,1,1,1,1,1,1,1,1,1,1,1,1,1,1,1,1,1,
1,1,1,1,1,1,1,6),(-1.,-0.984615384615383,-0.969230769230768,-0.953846153846152,
-0.938461538461537,-0.923076923076922,-0.907692307692306,-0.892307692307691,
-0.876923076923076,-0.86153846153846,-0.846153846153845,-0.83076923076923,
-0.815384615384614,-0.799999999999999,-0.784615384615384,-0.769230769230768,
-0.753846153846153,-0.738461538461538,-0.723076923076922,-0.707692307692307,
-0.692307692307692,-0.676923076923076,-0.661538461538461,-0.646153846153846,
-0.63076923076923,-0.615384615384615,-0.6,-0.584615384615384,-0.569230769230769,
-0.553846153846154,-0.538461538461538,-0.523076923076923,-0.507692307692308,
-0.492307692307692,-0.476923076923077,-0.461538461538462,-0.446153846153846,
-0.430769230769231,-0.415384615384615,-0.4,-0.384615384615385,-0.369230769230769,
-0.353846153846154,-0.338461538461538,-0.323076923076923,-0.307692307692308,
-0.292307692307692,-0.276923076923077,-0.261538461538462,-0.246153846153846,
-0.230769230769231,-0.215384615384615,-0.2,-0.184615384615385,-0.169230769230769,
-0.153846153846154,-0.138461538461538,-0.123076923076923,-0.107692307692308,
-0.0923076923076923,-0.0769230769230769,-0.0615384615384615,-0.0461538461538462,
-0.0307692307692308,-0.0153846153846154,-0.00577184337451708),
 .UNSPECIFIED.)
CURVE()
GEOMETRIC_REPRESENTATION_ITEM()
RATIONAL_B_SPLINE_CURVE((1.,1.,1.,1.,1.,1.,1.,1.,1.,1.,1.,1.,1.,1.,1.,1.,
1.,1.,1.,1.,1.,1.,1.,1.,1.,1.,1.,1.,1.,1.,1.,1.,1.,1.,1.,1.,1.,1.,1.,1.,
1.,1.,1.,1.,1.,1.,1.,1.,1.,1.,1.,1.,1.,1.,1.,1.,1.,1.,1.,1.,1.,1.,1.,1.,
1.,1.,1.,1.,1.,1.))
REPRESENTATION_ITEM('')
);
#336=(
BOUNDED_CURVE()
B_SPLINE_CURVE(5,(#54719,#54720,#54721,#54722,#54723,#54724,#54725,#54726,
#54727,#54728,#54729,#54730,#54731,#54732,#54733,#54734,#54735,#54736,#54737,
#54738,#54739,#54740,#54741,#54742,#54743,#54744,#54745,#54746,#54747,#54748,
#54749,#54750,#54751,#54752,#54753,#54754,#54755,#54756,#54757,#54758,#54759,
#54760,#54761,#54762,#54763,#54764,#54765,#54766,#54767,#54768,#54769,#54770,
#54771,#54772,#54773,#54774,#54775,#54776,#54777,#54778,#54779,#54780,#54781,
#54782,#54783,#54784,#54785,#54786,#54787,#54788),.UNSPECIFIED.,.F.,.F.)
B_SPLINE_CURVE_WITH_KNOTS((6,1,1,1,1,1,1,1,1,1,1,1,1,1,1,1,1,1,1,1,1,1,
1,1,1,1,1,1,1,1,1,1,1,1,1,1,1,1,1,1,1,1,1,1,1,1,1,1,1,1,1,1,1,1,1,1,1,1,
1,1,1,1,1,1,1,6),(-0.994228156739669,-0.984615384615383,-0.969230769230768,
-0.953846153846152,-0.938461538461537,-0.923076923076922,-0.907692307692306,
-0.892307692307691,-0.876923076923076,-0.86153846153846,-0.846153846153845,
-0.83076923076923,-0.815384615384614,-0.799999999999999,-0.784615384615384,
-0.769230769230768,-0.753846153846153,-0.738461538461538,-0.723076923076922,
-0.707692307692307,-0.692307692307692,-0.676923076923076,-0.661538461538461,
-0.646153846153846,-0.63076923076923,-0.615384615384615,-0.6,-0.584615384615384,
-0.569230769230769,-0.553846153846154,-0.538461538461538,-0.523076923076923,
-0.507692307692308,-0.492307692307692,-0.476923076923077,-0.461538461538462,
-0.446153846153846,-0.430769230769231,-0.415384615384615,-0.4,-0.384615384615385,
-0.369230769230769,-0.353846153846154,-0.338461538461538,-0.323076923076923,
-0.307692307692308,-0.292307692307692,-0.276923076923077,-0.261538461538462,
-0.246153846153846,-0.230769230769231,-0.215384615384615,-0.2,-0.184615384615385,
-0.169230769230769,-0.153846153846154,-0.138461538461538,-0.123076923076923,
-0.107692307692308,-0.0923076923076923,-0.0769230769230769,-0.0615384615384615,
-0.0461538461538462,-0.0307692307692308,-0.0153846153846154,0.),
 .UNSPECIFIED.)
CURVE()
GEOMETRIC_REPRESENTATION_ITEM()
RATIONAL_B_SPLINE_CURVE((1.,1.,1.,1.,1.,1.,1.,1.,1.,1.,1.,1.,1.,1.,1.,1.,
1.,1.,1.,1.,1.,1.,1.,1.,1.,1.,1.,1.,1.,1.,1.,1.,1.,1.,1.,1.,1.,1.,1.,1.,
1.,1.,1.,1.,1.,1.,1.,1.,1.,1.,1.,1.,1.,1.,1.,1.,1.,1.,1.,1.,1.,1.,1.,1.,
1.,1.,1.,1.,1.,1.))
REPRESENTATION_ITEM('')
);
#337=(
BOUNDED_CURVE()
B_SPLINE_CURVE(5,(#54941,#54942,#54943,#54944,#54945,#54946,#54947,#54948,
#54949,#54950,#54951,#54952,#54953,#54954,#54955,#54956,#54957,#54958,#54959,
#54960,#54961,#54962,#54963,#54964,#54965,#54966,#54967,#54968,#54969,#54970,
#54971,#54972,#54973,#54974,#54975,#54976,#54977,#54978,#54979,#54980,#54981,
#54982,#54983,#54984,#54985,#54986,#54987,#54988,#54989,#54990,#54991,#54992,
#54993,#54994,#54995,#54996,#54997,#54998,#54999,#55000,#55001,#55002,#55003,
#55004,#55005,#55006,#55007,#55008,#55009,#55010),.UNSPECIFIED.,.F.,.F.)
B_SPLINE_CURVE_WITH_KNOTS((6,1,1,1,1,1,1,1,1,1,1,1,1,1,1,1,1,1,1,1,1,1,
1,1,1,1,1,1,1,1,1,1,1,1,1,1,1,1,1,1,1,1,1,1,1,1,1,1,1,1,1,1,1,1,1,1,1,1,
1,1,1,1,1,1,1,6),(-1.,-0.984615384615383,-0.969230769230768,-0.953846153846152,
-0.938461538461537,-0.923076923076922,-0.907692307692306,-0.892307692307691,
-0.876923076923076,-0.86153846153846,-0.846153846153845,-0.83076923076923,
-0.815384615384614,-0.799999999999999,-0.784615384615384,-0.769230769230768,
-0.753846153846153,-0.738461538461538,-0.723076923076922,-0.707692307692307,
-0.692307692307692,-0.676923076923076,-0.661538461538461,-0.646153846153846,
-0.63076923076923,-0.615384615384615,-0.6,-0.584615384615384,-0.569230769230769,
-0.553846153846154,-0.538461538461538,-0.523076923076923,-0.507692307692308,
-0.492307692307692,-0.476923076923077,-0.461538461538462,-0.446153846153846,
-0.430769230769231,-0.415384615384615,-0.4,-0.384615384615385,-0.369230769230769,
-0.353846153846154,-0.338461538461538,-0.323076923076923,-0.307692307692308,
-0.292307692307692,-0.276923076923077,-0.261538461538462,-0.246153846153846,
-0.230769230769231,-0.215384615384615,-0.2,-0.184615384615385,-0.169230769230769,
-0.153846153846154,-0.138461538461538,-0.123076923076923,-0.107692307692308,
-0.0923076923076923,-0.0769230769230769,-0.0615384615384615,-0.0461538461538462,
-0.0307692307692308,-0.0153846153846154,-0.0057718433744903),
 .UNSPECIFIED.)
CURVE()
GEOMETRIC_REPRESENTATION_ITEM()
RATIONAL_B_SPLINE_CURVE((1.,1.,1.,1.,1.,1.,1.,1.,1.,1.,1.,1.,1.,1.,1.,1.,
1.,1.,1.,1.,1.,1.,1.,1.,1.,1.,1.,1.,1.,1.,1.,1.,1.,1.,1.,1.,1.,1.,1.,1.,
1.,1.,1.,1.,1.,1.,1.,1.,1.,1.,1.,1.,1.,1.,1.,1.,1.,1.,1.,1.,1.,1.,1.,1.,
1.,1.,1.,1.,1.,1.))
REPRESENTATION_ITEM('')
);
#338=(
BOUNDED_CURVE()
B_SPLINE_CURVE(5,(#55161,#55162,#55163,#55164,#55165,#55166,#55167,#55168,
#55169,#55170,#55171,#55172,#55173,#55174,#55175,#55176,#55177,#55178,#55179,
#55180,#55181,#55182,#55183,#55184,#55185,#55186,#55187,#55188,#55189,#55190,
#55191,#55192,#55193,#55194,#55195,#55196,#55197,#55198,#55199,#55200,#55201,
#55202,#55203,#55204,#55205,#55206,#55207,#55208,#55209,#55210,#55211,#55212,
#55213,#55214,#55215,#55216,#55217,#55218,#55219,#55220,#55221,#55222,#55223,
#55224,#55225,#55226,#55227,#55228,#55229,#55230),.UNSPECIFIED.,.F.,.F.)
B_SPLINE_CURVE_WITH_KNOTS((6,1,1,1,1,1,1,1,1,1,1,1,1,1,1,1,1,1,1,1,1,1,
1,1,1,1,1,1,1,1,1,1,1,1,1,1,1,1,1,1,1,1,1,1,1,1,1,1,1,1,1,1,1,1,1,1,1,1,
1,1,1,1,1,1,1,6),(-0.994228156739712,-0.984615384615383,-0.969230769230768,
-0.953846153846152,-0.938461538461537,-0.923076923076922,-0.907692307692306,
-0.892307692307691,-0.876923076923076,-0.86153846153846,-0.846153846153845,
-0.83076923076923,-0.815384615384614,-0.799999999999999,-0.784615384615384,
-0.769230769230768,-0.753846153846153,-0.738461538461538,-0.723076923076922,
-0.707692307692307,-0.692307692307692,-0.676923076923076,-0.661538461538461,
-0.646153846153846,-0.63076923076923,-0.615384615384615,-0.6,-0.584615384615384,
-0.569230769230769,-0.553846153846154,-0.538461538461538,-0.523076923076923,
-0.507692307692308,-0.492307692307692,-0.476923076923077,-0.461538461538462,
-0.446153846153846,-0.430769230769231,-0.415384615384615,-0.4,-0.384615384615385,
-0.369230769230769,-0.353846153846154,-0.338461538461538,-0.323076923076923,
-0.307692307692308,-0.292307692307692,-0.276923076923077,-0.261538461538462,
-0.246153846153846,-0.230769230769231,-0.215384615384615,-0.2,-0.184615384615385,
-0.169230769230769,-0.153846153846154,-0.138461538461538,-0.123076923076923,
-0.107692307692308,-0.0923076923076923,-0.0769230769230769,-0.0615384615384615,
-0.0461538461538462,-0.0307692307692308,-0.0153846153846154,0.),
 .UNSPECIFIED.)
CURVE()
GEOMETRIC_REPRESENTATION_ITEM()
RATIONAL_B_SPLINE_CURVE((1.,1.,1.,1.,1.,1.,1.,1.,1.,1.,1.,1.,1.,1.,1.,1.,
1.,1.,1.,1.,1.,1.,1.,1.,1.,1.,1.,1.,1.,1.,1.,1.,1.,1.,1.,1.,1.,1.,1.,1.,
1.,1.,1.,1.,1.,1.,1.,1.,1.,1.,1.,1.,1.,1.,1.,1.,1.,1.,1.,1.,1.,1.,1.,1.,
1.,1.,1.,1.,1.,1.))
REPRESENTATION_ITEM('')
);
#339=(
BOUNDED_CURVE()
B_SPLINE_CURVE(5,(#55383,#55384,#55385,#55386,#55387,#55388,#55389,#55390,
#55391,#55392,#55393,#55394,#55395,#55396,#55397,#55398,#55399,#55400,#55401,
#55402,#55403,#55404,#55405,#55406,#55407,#55408,#55409,#55410,#55411,#55412,
#55413,#55414,#55415,#55416,#55417,#55418,#55419,#55420,#55421,#55422,#55423,
#55424,#55425,#55426,#55427,#55428,#55429,#55430,#55431,#55432,#55433,#55434,
#55435,#55436,#55437,#55438,#55439,#55440,#55441,#55442,#55443,#55444,#55445,
#55446,#55447,#55448,#55449,#55450,#55451,#55452),.UNSPECIFIED.,.F.,.F.)
B_SPLINE_CURVE_WITH_KNOTS((6,1,1,1,1,1,1,1,1,1,1,1,1,1,1,1,1,1,1,1,1,1,
1,1,1,1,1,1,1,1,1,1,1,1,1,1,1,1,1,1,1,1,1,1,1,1,1,1,1,1,1,1,1,1,1,1,1,1,
1,1,1,1,1,1,1,6),(-1.,-0.984615384615383,-0.969230769230768,-0.953846153846152,
-0.938461538461537,-0.923076923076922,-0.907692307692306,-0.892307692307691,
-0.876923076923076,-0.86153846153846,-0.846153846153845,-0.83076923076923,
-0.815384615384614,-0.799999999999999,-0.784615384615384,-0.769230769230768,
-0.753846153846153,-0.738461538461538,-0.723076923076922,-0.707692307692307,
-0.692307692307692,-0.676923076923076,-0.661538461538461,-0.646153846153846,
-0.63076923076923,-0.615384615384615,-0.6,-0.584615384615384,-0.569230769230769,
-0.553846153846154,-0.538461538461538,-0.523076923076923,-0.507692307692308,
-0.492307692307692,-0.476923076923077,-0.461538461538462,-0.446153846153846,
-0.430769230769231,-0.415384615384615,-0.4,-0.384615384615385,-0.369230769230769,
-0.353846153846154,-0.338461538461538,-0.323076923076923,-0.307692307692308,
-0.292307692307692,-0.276923076923077,-0.261538461538462,-0.246153846153846,
-0.230769230769231,-0.215384615384615,-0.2,-0.184615384615385,-0.169230769230769,
-0.153846153846154,-0.138461538461538,-0.123076923076923,-0.107692307692308,
-0.0923076923076923,-0.0769230769230769,-0.0615384615384615,-0.0461538461538462,
-0.0307692307692308,-0.0153846153846154,-0.0057718433745291),
 .UNSPECIFIED.)
CURVE()
GEOMETRIC_REPRESENTATION_ITEM()
RATIONAL_B_SPLINE_CURVE((1.,1.,1.,1.,1.,1.,1.,1.,1.,1.,1.,1.,1.,1.,1.,1.,
1.,1.,1.,1.,1.,1.,1.,1.,1.,1.,1.,1.,1.,1.,1.,1.,1.,1.,1.,1.,1.,1.,1.,1.,
1.,1.,1.,1.,1.,1.,1.,1.,1.,1.,1.,1.,1.,1.,1.,1.,1.,1.,1.,1.,1.,1.,1.,1.,
1.,1.,1.,1.,1.,1.))
REPRESENTATION_ITEM('')
);
#340=(
BOUNDED_CURVE()
B_SPLINE_CURVE(5,(#55603,#55604,#55605,#55606,#55607,#55608,#55609,#55610,
#55611,#55612,#55613,#55614,#55615,#55616,#55617,#55618,#55619,#55620,#55621,
#55622,#55623,#55624,#55625,#55626,#55627,#55628,#55629,#55630,#55631,#55632,
#55633,#55634,#55635,#55636,#55637,#55638,#55639,#55640,#55641,#55642,#55643,
#55644,#55645,#55646,#55647,#55648,#55649,#55650,#55651,#55652,#55653,#55654,
#55655,#55656,#55657,#55658,#55659,#55660,#55661,#55662,#55663,#55664,#55665,
#55666,#55667,#55668,#55669,#55670,#55671,#55672),.UNSPECIFIED.,.F.,.F.)
B_SPLINE_CURVE_WITH_KNOTS((6,1,1,1,1,1,1,1,1,1,1,1,1,1,1,1,1,1,1,1,1,1,
1,1,1,1,1,1,1,1,1,1,1,1,1,1,1,1,1,1,1,1,1,1,1,1,1,1,1,1,1,1,1,1,1,1,1,1,
1,1,1,1,1,1,1,6),(-0.994228156739695,-0.984615384615383,-0.969230769230768,
-0.953846153846152,-0.938461538461537,-0.923076923076922,-0.907692307692306,
-0.892307692307691,-0.876923076923076,-0.86153846153846,-0.846153846153845,
-0.83076923076923,-0.815384615384614,-0.799999999999999,-0.784615384615384,
-0.769230769230768,-0.753846153846153,-0.738461538461538,-0.723076923076922,
-0.707692307692307,-0.692307692307692,-0.676923076923076,-0.661538461538461,
-0.646153846153846,-0.63076923076923,-0.615384615384615,-0.6,-0.584615384615384,
-0.569230769230769,-0.553846153846154,-0.538461538461538,-0.523076923076923,
-0.507692307692308,-0.492307692307692,-0.476923076923077,-0.461538461538462,
-0.446153846153846,-0.430769230769231,-0.415384615384615,-0.4,-0.384615384615385,
-0.369230769230769,-0.353846153846154,-0.338461538461538,-0.323076923076923,
-0.307692307692308,-0.292307692307692,-0.276923076923077,-0.261538461538462,
-0.246153846153846,-0.230769230769231,-0.215384615384615,-0.2,-0.184615384615385,
-0.169230769230769,-0.153846153846154,-0.138461538461538,-0.123076923076923,
-0.107692307692308,-0.0923076923076923,-0.0769230769230769,-0.0615384615384615,
-0.0461538461538462,-0.0307692307692308,-0.0153846153846154,0.),
 .UNSPECIFIED.)
CURVE()
GEOMETRIC_REPRESENTATION_ITEM()
RATIONAL_B_SPLINE_CURVE((1.,1.,1.,1.,1.,1.,1.,1.,1.,1.,1.,1.,1.,1.,1.,1.,
1.,1.,1.,1.,1.,1.,1.,1.,1.,1.,1.,1.,1.,1.,1.,1.,1.,1.,1.,1.,1.,1.,1.,1.,
1.,1.,1.,1.,1.,1.,1.,1.,1.,1.,1.,1.,1.,1.,1.,1.,1.,1.,1.,1.,1.,1.,1.,1.,
1.,1.,1.,1.,1.,1.))
REPRESENTATION_ITEM('')
);
#341=(
BOUNDED_CURVE()
B_SPLINE_CURVE(5,(#55825,#55826,#55827,#55828,#55829,#55830,#55831,#55832,
#55833,#55834,#55835,#55836,#55837,#55838,#55839,#55840,#55841,#55842,#55843,
#55844,#55845,#55846,#55847,#55848,#55849,#55850,#55851,#55852,#55853,#55854,
#55855,#55856,#55857,#55858,#55859,#55860,#55861,#55862,#55863,#55864,#55865,
#55866,#55867,#55868,#55869,#55870,#55871,#55872,#55873,#55874,#55875,#55876,
#55877,#55878,#55879,#55880,#55881,#55882,#55883,#55884,#55885,#55886,#55887,
#55888,#55889,#55890,#55891,#55892,#55893,#55894),.UNSPECIFIED.,.F.,.F.)
B_SPLINE_CURVE_WITH_KNOTS((6,1,1,1,1,1,1,1,1,1,1,1,1,1,1,1,1,1,1,1,1,1,
1,1,1,1,1,1,1,1,1,1,1,1,1,1,1,1,1,1,1,1,1,1,1,1,1,1,1,1,1,1,1,1,1,1,1,1,
1,1,1,1,1,1,1,6),(-1.,-0.984615384615383,-0.969230769230768,-0.953846153846152,
-0.938461538461537,-0.923076923076922,-0.907692307692306,-0.892307692307691,
-0.876923076923076,-0.86153846153846,-0.846153846153845,-0.83076923076923,
-0.815384615384614,-0.799999999999999,-0.784615384615384,-0.769230769230768,
-0.753846153846153,-0.738461538461538,-0.723076923076922,-0.707692307692307,
-0.692307692307692,-0.676923076923076,-0.661538461538461,-0.646153846153846,
-0.63076923076923,-0.615384615384615,-0.6,-0.584615384615384,-0.569230769230769,
-0.553846153846154,-0.538461538461538,-0.523076923076923,-0.507692307692308,
-0.492307692307692,-0.476923076923077,-0.461538461538462,-0.446153846153846,
-0.430769230769231,-0.415384615384615,-0.4,-0.384615384615385,-0.369230769230769,
-0.353846153846154,-0.338461538461538,-0.323076923076923,-0.307692307692308,
-0.292307692307692,-0.276923076923077,-0.261538461538462,-0.246153846153846,
-0.230769230769231,-0.215384615384615,-0.2,-0.184615384615385,-0.169230769230769,
-0.153846153846154,-0.138461538461538,-0.123076923076923,-0.107692307692308,
-0.0923076923076923,-0.0769230769230769,-0.0615384615384615,-0.0461538461538462,
-0.0307692307692308,-0.0153846153846154,-0.00577184337450344),
 .UNSPECIFIED.)
CURVE()
GEOMETRIC_REPRESENTATION_ITEM()
RATIONAL_B_SPLINE_CURVE((1.,1.,1.,1.,1.,1.,1.,1.,1.,1.,1.,1.,1.,1.,1.,1.,
1.,1.,1.,1.,1.,1.,1.,1.,1.,1.,1.,1.,1.,1.,1.,1.,1.,1.,1.,1.,1.,1.,1.,1.,
1.,1.,1.,1.,1.,1.,1.,1.,1.,1.,1.,1.,1.,1.,1.,1.,1.,1.,1.,1.,1.,1.,1.,1.,
1.,1.,1.,1.,1.,1.))
REPRESENTATION_ITEM('')
);
#342=(
BOUNDED_CURVE()
B_SPLINE_CURVE(5,(#56045,#56046,#56047,#56048,#56049,#56050,#56051,#56052,
#56053,#56054,#56055,#56056,#56057,#56058,#56059,#56060,#56061,#56062,#56063,
#56064,#56065,#56066,#56067,#56068,#56069,#56070,#56071,#56072,#56073,#56074,
#56075,#56076,#56077,#56078,#56079,#56080,#56081,#56082,#56083,#56084,#56085,
#56086,#56087,#56088,#56089,#56090,#56091,#56092,#56093,#56094,#56095,#56096,
#56097,#56098,#56099,#56100,#56101,#56102,#56103,#56104,#56105,#56106,#56107,
#56108,#56109,#56110,#56111,#56112,#56113,#56114),.UNSPECIFIED.,.F.,.F.)
B_SPLINE_CURVE_WITH_KNOTS((6,1,1,1,1,1,1,1,1,1,1,1,1,1,1,1,1,1,1,1,1,1,
1,1,1,1,1,1,1,1,1,1,1,1,1,1,1,1,1,1,1,1,1,1,1,1,1,1,1,1,1,1,1,1,1,1,1,1,
1,1,1,1,1,1,1,6),(-0.994228156739669,-0.984615384615383,-0.969230769230768,
-0.953846153846152,-0.938461538461537,-0.923076923076922,-0.907692307692306,
-0.892307692307691,-0.876923076923076,-0.86153846153846,-0.846153846153845,
-0.83076923076923,-0.815384615384614,-0.799999999999999,-0.784615384615384,
-0.769230769230768,-0.753846153846153,-0.738461538461538,-0.723076923076922,
-0.707692307692307,-0.692307692307692,-0.676923076923076,-0.661538461538461,
-0.646153846153846,-0.63076923076923,-0.615384615384615,-0.6,-0.584615384615384,
-0.569230769230769,-0.553846153846154,-0.538461538461538,-0.523076923076923,
-0.507692307692308,-0.492307692307692,-0.476923076923077,-0.461538461538462,
-0.446153846153846,-0.430769230769231,-0.415384615384615,-0.4,-0.384615384615385,
-0.369230769230769,-0.353846153846154,-0.338461538461538,-0.323076923076923,
-0.307692307692308,-0.292307692307692,-0.276923076923077,-0.261538461538462,
-0.246153846153846,-0.230769230769231,-0.215384615384615,-0.2,-0.184615384615385,
-0.169230769230769,-0.153846153846154,-0.138461538461538,-0.123076923076923,
-0.107692307692308,-0.0923076923076923,-0.0769230769230769,-0.0615384615384615,
-0.0461538461538462,-0.0307692307692308,-0.0153846153846154,0.),
 .UNSPECIFIED.)
CURVE()
GEOMETRIC_REPRESENTATION_ITEM()
RATIONAL_B_SPLINE_CURVE((1.,1.,1.,1.,1.,1.,1.,1.,1.,1.,1.,1.,1.,1.,1.,1.,
1.,1.,1.,1.,1.,1.,1.,1.,1.,1.,1.,1.,1.,1.,1.,1.,1.,1.,1.,1.,1.,1.,1.,1.,
1.,1.,1.,1.,1.,1.,1.,1.,1.,1.,1.,1.,1.,1.,1.,1.,1.,1.,1.,1.,1.,1.,1.,1.,
1.,1.,1.,1.,1.,1.))
REPRESENTATION_ITEM('')
);
#343=(
BOUNDED_CURVE()
B_SPLINE_CURVE(5,(#56267,#56268,#56269,#56270,#56271,#56272,#56273,#56274,
#56275,#56276,#56277,#56278,#56279,#56280,#56281,#56282,#56283,#56284,#56285,
#56286,#56287,#56288,#56289,#56290,#56291,#56292,#56293,#56294,#56295,#56296,
#56297,#56298,#56299,#56300,#56301,#56302,#56303,#56304,#56305,#56306,#56307,
#56308,#56309,#56310,#56311,#56312,#56313,#56314,#56315,#56316,#56317,#56318,
#56319,#56320,#56321,#56322,#56323,#56324,#56325,#56326,#56327,#56328,#56329,
#56330,#56331,#56332,#56333,#56334,#56335,#56336),.UNSPECIFIED.,.F.,.F.)
B_SPLINE_CURVE_WITH_KNOTS((6,1,1,1,1,1,1,1,1,1,1,1,1,1,1,1,1,1,1,1,1,1,
1,1,1,1,1,1,1,1,1,1,1,1,1,1,1,1,1,1,1,1,1,1,1,1,1,1,1,1,1,1,1,1,1,1,1,1,
1,1,1,1,1,1,1,6),(-1.,-0.984615384615383,-0.969230769230768,-0.953846153846152,
-0.938461538461537,-0.923076923076922,-0.907692307692306,-0.892307692307691,
-0.876923076923076,-0.86153846153846,-0.846153846153845,-0.83076923076923,
-0.815384615384614,-0.799999999999999,-0.784615384615384,-0.769230769230768,
-0.753846153846153,-0.738461538461538,-0.723076923076922,-0.707692307692307,
-0.692307692307692,-0.676923076923076,-0.661538461538461,-0.646153846153846,
-0.63076923076923,-0.615384615384615,-0.6,-0.584615384615384,-0.569230769230769,
-0.553846153846154,-0.538461538461538,-0.523076923076923,-0.507692307692308,
-0.492307692307692,-0.476923076923077,-0.461538461538462,-0.446153846153846,
-0.430769230769231,-0.415384615384615,-0.4,-0.384615384615385,-0.369230769230769,
-0.353846153846154,-0.338461538461538,-0.323076923076923,-0.307692307692308,
-0.292307692307692,-0.276923076923077,-0.261538461538462,-0.246153846153846,
-0.230769230769231,-0.215384615384615,-0.2,-0.184615384615385,-0.169230769230769,
-0.153846153846154,-0.138461538461538,-0.123076923076923,-0.107692307692308,
-0.0923076923076923,-0.0769230769230769,-0.0615384615384615,-0.0461538461538462,
-0.0307692307692308,-0.0153846153846154,-0.00577184337450876),
 .UNSPECIFIED.)
CURVE()
GEOMETRIC_REPRESENTATION_ITEM()
RATIONAL_B_SPLINE_CURVE((1.,1.,1.,1.,1.,1.,1.,1.,1.,1.,1.,1.,1.,1.,1.,1.,
1.,1.,1.,1.,1.,1.,1.,1.,1.,1.,1.,1.,1.,1.,1.,1.,1.,1.,1.,1.,1.,1.,1.,1.,
1.,1.,1.,1.,1.,1.,1.,1.,1.,1.,1.,1.,1.,1.,1.,1.,1.,1.,1.,1.,1.,1.,1.,1.,
1.,1.,1.,1.,1.,1.))
REPRESENTATION_ITEM('')
);
#344=(
BOUNDED_CURVE()
B_SPLINE_CURVE(5,(#56487,#56488,#56489,#56490,#56491,#56492,#56493,#56494,
#56495,#56496,#56497,#56498,#56499,#56500,#56501,#56502,#56503,#56504,#56505,
#56506,#56507,#56508,#56509,#56510,#56511,#56512,#56513,#56514,#56515,#56516,
#56517,#56518,#56519,#56520,#56521,#56522,#56523,#56524,#56525,#56526,#56527,
#56528,#56529,#56530,#56531,#56532,#56533,#56534,#56535,#56536,#56537,#56538,
#56539,#56540,#56541,#56542,#56543,#56544,#56545,#56546,#56547,#56548,#56549,
#56550,#56551,#56552,#56553,#56554,#56555,#56556),.UNSPECIFIED.,.F.,.F.)
B_SPLINE_CURVE_WITH_KNOTS((6,1,1,1,1,1,1,1,1,1,1,1,1,1,1,1,1,1,1,1,1,1,
1,1,1,1,1,1,1,1,1,1,1,1,1,1,1,1,1,1,1,1,1,1,1,1,1,1,1,1,1,1,1,1,1,1,1,1,
1,1,1,1,1,1,1,6),(-0.99422815673966,-0.984615384615383,-0.969230769230768,
-0.953846153846152,-0.938461538461537,-0.923076923076922,-0.907692307692306,
-0.892307692307691,-0.876923076923076,-0.86153846153846,-0.846153846153845,
-0.83076923076923,-0.815384615384614,-0.799999999999999,-0.784615384615384,
-0.769230769230768,-0.753846153846153,-0.738461538461538,-0.723076923076922,
-0.707692307692307,-0.692307692307692,-0.676923076923076,-0.661538461538461,
-0.646153846153846,-0.63076923076923,-0.615384615384615,-0.6,-0.584615384615384,
-0.569230769230769,-0.553846153846154,-0.538461538461538,-0.523076923076923,
-0.507692307692308,-0.492307692307692,-0.476923076923077,-0.461538461538462,
-0.446153846153846,-0.430769230769231,-0.415384615384615,-0.4,-0.384615384615385,
-0.369230769230769,-0.353846153846154,-0.338461538461538,-0.323076923076923,
-0.307692307692308,-0.292307692307692,-0.276923076923077,-0.261538461538462,
-0.246153846153846,-0.230769230769231,-0.215384615384615,-0.2,-0.184615384615385,
-0.169230769230769,-0.153846153846154,-0.138461538461538,-0.123076923076923,
-0.107692307692308,-0.0923076923076923,-0.0769230769230769,-0.0615384615384615,
-0.0461538461538462,-0.0307692307692308,-0.0153846153846154,0.),
 .UNSPECIFIED.)
CURVE()
GEOMETRIC_REPRESENTATION_ITEM()
RATIONAL_B_SPLINE_CURVE((1.,1.,1.,1.,1.,1.,1.,1.,1.,1.,1.,1.,1.,1.,1.,1.,
1.,1.,1.,1.,1.,1.,1.,1.,1.,1.,1.,1.,1.,1.,1.,1.,1.,1.,1.,1.,1.,1.,1.,1.,
1.,1.,1.,1.,1.,1.,1.,1.,1.,1.,1.,1.,1.,1.,1.,1.,1.,1.,1.,1.,1.,1.,1.,1.,
1.,1.,1.,1.,1.,1.))
REPRESENTATION_ITEM('')
);
#345=(
BOUNDED_CURVE()
B_SPLINE_CURVE(5,(#56709,#56710,#56711,#56712,#56713,#56714,#56715,#56716,
#56717,#56718,#56719,#56720,#56721,#56722,#56723,#56724,#56725,#56726,#56727,
#56728,#56729,#56730,#56731,#56732,#56733,#56734,#56735,#56736,#56737,#56738,
#56739,#56740,#56741,#56742,#56743,#56744,#56745,#56746,#56747,#56748,#56749,
#56750,#56751,#56752,#56753,#56754,#56755,#56756,#56757,#56758,#56759,#56760,
#56761,#56762,#56763,#56764,#56765,#56766,#56767,#56768,#56769,#56770,#56771,
#56772,#56773,#56774,#56775,#56776,#56777,#56778),.UNSPECIFIED.,.F.,.F.)
B_SPLINE_CURVE_WITH_KNOTS((6,1,1,1,1,1,1,1,1,1,1,1,1,1,1,1,1,1,1,1,1,1,
1,1,1,1,1,1,1,1,1,1,1,1,1,1,1,1,1,1,1,1,1,1,1,1,1,1,1,1,1,1,1,1,1,1,1,1,
1,1,1,1,1,1,1,6),(-1.,-0.984615384615383,-0.969230769230768,-0.953846153846152,
-0.938461538461537,-0.923076923076922,-0.907692307692306,-0.892307692307691,
-0.876923076923076,-0.86153846153846,-0.846153846153845,-0.83076923076923,
-0.815384615384614,-0.799999999999999,-0.784615384615384,-0.769230769230768,
-0.753846153846153,-0.738461538461538,-0.723076923076922,-0.707692307692307,
-0.692307692307692,-0.676923076923076,-0.661538461538461,-0.646153846153846,
-0.63076923076923,-0.615384615384615,-0.6,-0.584615384615384,-0.569230769230769,
-0.553846153846154,-0.538461538461538,-0.523076923076923,-0.507692307692308,
-0.492307692307692,-0.476923076923077,-0.461538461538462,-0.446153846153846,
-0.430769230769231,-0.415384615384615,-0.4,-0.384615384615385,-0.369230769230769,
-0.353846153846154,-0.338461538461538,-0.323076923076923,-0.307692307692308,
-0.292307692307692,-0.276923076923077,-0.261538461538462,-0.246153846153846,
-0.230769230769231,-0.215384615384615,-0.2,-0.184615384615385,-0.169230769230769,
-0.153846153846154,-0.138461538461538,-0.123076923076923,-0.107692307692308,
-0.0923076923076923,-0.0769230769230769,-0.0615384615384615,-0.0461538461538462,
-0.0307692307692308,-0.0153846153846154,-0.00577184337451051),
 .UNSPECIFIED.)
CURVE()
GEOMETRIC_REPRESENTATION_ITEM()
RATIONAL_B_SPLINE_CURVE((1.,1.,1.,1.,1.,1.,1.,1.,1.,1.,1.,1.,1.,1.,1.,1.,
1.,1.,1.,1.,1.,1.,1.,1.,1.,1.,1.,1.,1.,1.,1.,1.,1.,1.,1.,1.,1.,1.,1.,1.,
1.,1.,1.,1.,1.,1.,1.,1.,1.,1.,1.,1.,1.,1.,1.,1.,1.,1.,1.,1.,1.,1.,1.,1.,
1.,1.,1.,1.,1.,1.))
REPRESENTATION_ITEM('')
);
#346=(
BOUNDED_CURVE()
B_SPLINE_CURVE(5,(#56929,#56930,#56931,#56932,#56933,#56934,#56935,#56936,
#56937,#56938,#56939,#56940,#56941,#56942,#56943,#56944,#56945,#56946,#56947,
#56948,#56949,#56950,#56951,#56952,#56953,#56954,#56955,#56956,#56957,#56958,
#56959,#56960,#56961,#56962,#56963,#56964,#56965,#56966,#56967,#56968,#56969,
#56970,#56971,#56972,#56973,#56974,#56975,#56976,#56977,#56978,#56979,#56980,
#56981,#56982,#56983,#56984,#56985,#56986,#56987,#56988,#56989,#56990,#56991,
#56992,#56993,#56994,#56995,#56996,#56997,#56998),.UNSPECIFIED.,.F.,.F.)
B_SPLINE_CURVE_WITH_KNOTS((6,1,1,1,1,1,1,1,1,1,1,1,1,1,1,1,1,1,1,1,1,1,
1,1,1,1,1,1,1,1,1,1,1,1,1,1,1,1,1,1,1,1,1,1,1,1,1,1,1,1,1,1,1,1,1,1,1,1,
1,1,1,1,1,1,1,6),(-0.994228156739678,-0.984615384615383,-0.969230769230768,
-0.953846153846152,-0.938461538461537,-0.923076923076922,-0.907692307692306,
-0.892307692307691,-0.876923076923076,-0.86153846153846,-0.846153846153845,
-0.83076923076923,-0.815384615384614,-0.799999999999999,-0.784615384615384,
-0.769230769230768,-0.753846153846153,-0.738461538461538,-0.723076923076922,
-0.707692307692307,-0.692307692307692,-0.676923076923076,-0.661538461538461,
-0.646153846153846,-0.63076923076923,-0.615384615384615,-0.6,-0.584615384615384,
-0.569230769230769,-0.553846153846154,-0.538461538461538,-0.523076923076923,
-0.507692307692308,-0.492307692307692,-0.476923076923077,-0.461538461538462,
-0.446153846153846,-0.430769230769231,-0.415384615384615,-0.4,-0.384615384615385,
-0.369230769230769,-0.353846153846154,-0.338461538461538,-0.323076923076923,
-0.307692307692308,-0.292307692307692,-0.276923076923077,-0.261538461538462,
-0.246153846153846,-0.230769230769231,-0.215384615384615,-0.2,-0.184615384615385,
-0.169230769230769,-0.153846153846154,-0.138461538461538,-0.123076923076923,
-0.107692307692308,-0.0923076923076923,-0.0769230769230769,-0.0615384615384615,
-0.0461538461538462,-0.0307692307692308,-0.0153846153846154,0.),
 .UNSPECIFIED.)
CURVE()
GEOMETRIC_REPRESENTATION_ITEM()
RATIONAL_B_SPLINE_CURVE((1.,1.,1.,1.,1.,1.,1.,1.,1.,1.,1.,1.,1.,1.,1.,1.,
1.,1.,1.,1.,1.,1.,1.,1.,1.,1.,1.,1.,1.,1.,1.,1.,1.,1.,1.,1.,1.,1.,1.,1.,
1.,1.,1.,1.,1.,1.,1.,1.,1.,1.,1.,1.,1.,1.,1.,1.,1.,1.,1.,1.,1.,1.,1.,1.,
1.,1.,1.,1.,1.,1.))
REPRESENTATION_ITEM('')
);
#347=(
BOUNDED_CURVE()
B_SPLINE_CURVE(5,(#57151,#57152,#57153,#57154,#57155,#57156,#57157,#57158,
#57159,#57160,#57161,#57162,#57163,#57164,#57165,#57166,#57167,#57168,#57169,
#57170,#57171,#57172,#57173,#57174,#57175,#57176,#57177,#57178,#57179,#57180,
#57181,#57182,#57183,#57184,#57185,#57186,#57187,#57188,#57189,#57190,#57191,
#57192,#57193,#57194,#57195,#57196,#57197,#57198,#57199,#57200,#57201,#57202,
#57203,#57204,#57205,#57206,#57207,#57208,#57209,#57210,#57211,#57212,#57213,
#57214,#57215,#57216,#57217,#57218,#57219,#57220),.UNSPECIFIED.,.F.,.F.)
B_SPLINE_CURVE_WITH_KNOTS((6,1,1,1,1,1,1,1,1,1,1,1,1,1,1,1,1,1,1,1,1,1,
1,1,1,1,1,1,1,1,1,1,1,1,1,1,1,1,1,1,1,1,1,1,1,1,1,1,1,1,1,1,1,1,1,1,1,1,
1,1,1,1,1,1,1,6),(-1.,-0.984615384615383,-0.969230769230768,-0.953846153846152,
-0.938461538461537,-0.923076923076922,-0.907692307692306,-0.892307692307691,
-0.876923076923076,-0.86153846153846,-0.846153846153845,-0.83076923076923,
-0.815384615384614,-0.799999999999999,-0.784615384615384,-0.769230769230768,
-0.753846153846153,-0.738461538461538,-0.723076923076922,-0.707692307692307,
-0.692307692307692,-0.676923076923076,-0.661538461538461,-0.646153846153846,
-0.63076923076923,-0.615384615384615,-0.6,-0.584615384615384,-0.569230769230769,
-0.553846153846154,-0.538461538461538,-0.523076923076923,-0.507692307692308,
-0.492307692307692,-0.476923076923077,-0.461538461538462,-0.446153846153846,
-0.430769230769231,-0.415384615384615,-0.4,-0.384615384615385,-0.369230769230769,
-0.353846153846154,-0.338461538461538,-0.323076923076923,-0.307692307692308,
-0.292307692307692,-0.276923076923077,-0.261538461538462,-0.246153846153846,
-0.230769230769231,-0.215384615384615,-0.2,-0.184615384615385,-0.169230769230769,
-0.153846153846154,-0.138461538461538,-0.123076923076923,-0.107692307692308,
-0.0923076923076923,-0.0769230769230769,-0.0615384615384615,-0.0461538461538462,
-0.0307692307692308,-0.0153846153846154,-0.0057718433745179),
 .UNSPECIFIED.)
CURVE()
GEOMETRIC_REPRESENTATION_ITEM()
RATIONAL_B_SPLINE_CURVE((1.,1.,1.,1.,1.,1.,1.,1.,1.,1.,1.,1.,1.,1.,1.,1.,
1.,1.,1.,1.,1.,1.,1.,1.,1.,1.,1.,1.,1.,1.,1.,1.,1.,1.,1.,1.,1.,1.,1.,1.,
1.,1.,1.,1.,1.,1.,1.,1.,1.,1.,1.,1.,1.,1.,1.,1.,1.,1.,1.,1.,1.,1.,1.,1.,
1.,1.,1.,1.,1.,1.))
REPRESENTATION_ITEM('')
);
#348=(
BOUNDED_CURVE()
B_SPLINE_CURVE(5,(#57371,#57372,#57373,#57374,#57375,#57376,#57377,#57378,
#57379,#57380,#57381,#57382,#57383,#57384,#57385,#57386,#57387,#57388,#57389,
#57390,#57391,#57392,#57393,#57394,#57395,#57396,#57397,#57398,#57399,#57400,
#57401,#57402,#57403,#57404,#57405,#57406,#57407,#57408,#57409,#57410,#57411,
#57412,#57413,#57414,#57415,#57416,#57417,#57418,#57419,#57420,#57421,#57422,
#57423,#57424,#57425,#57426,#57427,#57428,#57429,#57430,#57431,#57432,#57433,
#57434,#57435,#57436,#57437,#57438,#57439,#57440),.UNSPECIFIED.,.F.,.F.)
B_SPLINE_CURVE_WITH_KNOTS((6,1,1,1,1,1,1,1,1,1,1,1,1,1,1,1,1,1,1,1,1,1,
1,1,1,1,1,1,1,1,1,1,1,1,1,1,1,1,1,1,1,1,1,1,1,1,1,1,1,1,1,1,1,1,1,1,1,1,
1,1,1,1,1,1,1,6),(-0.99422815673967,-0.984615384615383,-0.969230769230768,
-0.953846153846152,-0.938461538461537,-0.923076923076922,-0.907692307692306,
-0.892307692307691,-0.876923076923076,-0.86153846153846,-0.846153846153845,
-0.83076923076923,-0.815384615384614,-0.799999999999999,-0.784615384615384,
-0.769230769230768,-0.753846153846153,-0.738461538461538,-0.723076923076922,
-0.707692307692307,-0.692307692307692,-0.676923076923076,-0.661538461538461,
-0.646153846153846,-0.63076923076923,-0.615384615384615,-0.6,-0.584615384615384,
-0.569230769230769,-0.553846153846154,-0.538461538461538,-0.523076923076923,
-0.507692307692308,-0.492307692307692,-0.476923076923077,-0.461538461538462,
-0.446153846153846,-0.430769230769231,-0.415384615384615,-0.4,-0.384615384615385,
-0.369230769230769,-0.353846153846154,-0.338461538461538,-0.323076923076923,
-0.307692307692308,-0.292307692307692,-0.276923076923077,-0.261538461538462,
-0.246153846153846,-0.230769230769231,-0.215384615384615,-0.2,-0.184615384615385,
-0.169230769230769,-0.153846153846154,-0.138461538461538,-0.123076923076923,
-0.107692307692308,-0.0923076923076923,-0.0769230769230769,-0.0615384615384615,
-0.0461538461538462,-0.0307692307692308,-0.0153846153846154,0.),
 .UNSPECIFIED.)
CURVE()
GEOMETRIC_REPRESENTATION_ITEM()
RATIONAL_B_SPLINE_CURVE((1.,1.,1.,1.,1.,1.,1.,1.,1.,1.,1.,1.,1.,1.,1.,1.,
1.,1.,1.,1.,1.,1.,1.,1.,1.,1.,1.,1.,1.,1.,1.,1.,1.,1.,1.,1.,1.,1.,1.,1.,
1.,1.,1.,1.,1.,1.,1.,1.,1.,1.,1.,1.,1.,1.,1.,1.,1.,1.,1.,1.,1.,1.,1.,1.,
1.,1.,1.,1.,1.,1.))
REPRESENTATION_ITEM('')
);
#349=(
BOUNDED_CURVE()
B_SPLINE_CURVE(5,(#57593,#57594,#57595,#57596,#57597,#57598,#57599,#57600,
#57601,#57602,#57603,#57604,#57605,#57606,#57607,#57608,#57609,#57610,#57611,
#57612,#57613,#57614,#57615,#57616,#57617,#57618,#57619,#57620,#57621,#57622,
#57623,#57624,#57625,#57626,#57627,#57628,#57629,#57630,#57631,#57632,#57633,
#57634,#57635,#57636,#57637,#57638,#57639,#57640,#57641,#57642,#57643,#57644,
#57645,#57646,#57647,#57648,#57649,#57650,#57651,#57652,#57653,#57654,#57655,
#57656,#57657,#57658,#57659,#57660,#57661,#57662),.UNSPECIFIED.,.F.,.F.)
B_SPLINE_CURVE_WITH_KNOTS((6,1,1,1,1,1,1,1,1,1,1,1,1,1,1,1,1,1,1,1,1,1,
1,1,1,1,1,1,1,1,1,1,1,1,1,1,1,1,1,1,1,1,1,1,1,1,1,1,1,1,1,1,1,1,1,1,1,1,
1,1,1,1,1,1,1,6),(-1.,-0.984615384615383,-0.969230769230768,-0.953846153846152,
-0.938461538461537,-0.923076923076922,-0.907692307692306,-0.892307692307691,
-0.876923076923076,-0.86153846153846,-0.846153846153845,-0.83076923076923,
-0.815384615384614,-0.799999999999999,-0.784615384615384,-0.769230769230768,
-0.753846153846153,-0.738461538461538,-0.723076923076922,-0.707692307692307,
-0.692307692307692,-0.676923076923076,-0.661538461538461,-0.646153846153846,
-0.63076923076923,-0.615384615384615,-0.6,-0.584615384615384,-0.569230769230769,
-0.553846153846154,-0.538461538461538,-0.523076923076923,-0.507692307692308,
-0.492307692307692,-0.476923076923077,-0.461538461538462,-0.446153846153846,
-0.430769230769231,-0.415384615384615,-0.4,-0.384615384615385,-0.369230769230769,
-0.353846153846154,-0.338461538461538,-0.323076923076923,-0.307692307692308,
-0.292307692307692,-0.276923076923077,-0.261538461538462,-0.246153846153846,
-0.230769230769231,-0.215384615384615,-0.2,-0.184615384615385,-0.169230769230769,
-0.153846153846154,-0.138461538461538,-0.123076923076923,-0.107692307692308,
-0.0923076923076923,-0.0769230769230769,-0.0615384615384615,-0.0461538461538462,
-0.0307692307692308,-0.0153846153846154,-0.00577184337452479),
 .UNSPECIFIED.)
CURVE()
GEOMETRIC_REPRESENTATION_ITEM()
RATIONAL_B_SPLINE_CURVE((1.,1.,1.,1.,1.,1.,1.,1.,1.,1.,1.,1.,1.,1.,1.,1.,
1.,1.,1.,1.,1.,1.,1.,1.,1.,1.,1.,1.,1.,1.,1.,1.,1.,1.,1.,1.,1.,1.,1.,1.,
1.,1.,1.,1.,1.,1.,1.,1.,1.,1.,1.,1.,1.,1.,1.,1.,1.,1.,1.,1.,1.,1.,1.,1.,
1.,1.,1.,1.,1.,1.))
REPRESENTATION_ITEM('')
);
#350=(
BOUNDED_CURVE()
B_SPLINE_CURVE(5,(#57813,#57814,#57815,#57816,#57817,#57818,#57819,#57820,
#57821,#57822,#57823,#57824,#57825,#57826,#57827,#57828,#57829,#57830,#57831,
#57832,#57833,#57834,#57835,#57836,#57837,#57838,#57839,#57840,#57841,#57842,
#57843,#57844,#57845,#57846,#57847,#57848,#57849,#57850,#57851,#57852,#57853,
#57854,#57855,#57856,#57857,#57858,#57859,#57860,#57861,#57862,#57863,#57864,
#57865,#57866,#57867,#57868,#57869,#57870,#57871,#57872,#57873,#57874,#57875,
#57876,#57877,#57878,#57879,#57880,#57881,#57882),.UNSPECIFIED.,.F.,.F.)
B_SPLINE_CURVE_WITH_KNOTS((6,1,1,1,1,1,1,1,1,1,1,1,1,1,1,1,1,1,1,1,1,1,
1,1,1,1,1,1,1,1,1,1,1,1,1,1,1,1,1,1,1,1,1,1,1,1,1,1,1,1,1,1,1,1,1,1,1,1,
1,1,1,1,1,1,1,6),(-0.99422815673967,-0.984615384615383,-0.969230769230768,
-0.953846153846152,-0.938461538461537,-0.923076923076922,-0.907692307692306,
-0.892307692307691,-0.876923076923076,-0.86153846153846,-0.846153846153845,
-0.83076923076923,-0.815384615384614,-0.799999999999999,-0.784615384615384,
-0.769230769230768,-0.753846153846153,-0.738461538461538,-0.723076923076922,
-0.707692307692307,-0.692307692307692,-0.676923076923076,-0.661538461538461,
-0.646153846153846,-0.63076923076923,-0.615384615384615,-0.6,-0.584615384615384,
-0.569230769230769,-0.553846153846154,-0.538461538461538,-0.523076923076923,
-0.507692307692308,-0.492307692307692,-0.476923076923077,-0.461538461538462,
-0.446153846153846,-0.430769230769231,-0.415384615384615,-0.4,-0.384615384615385,
-0.369230769230769,-0.353846153846154,-0.338461538461538,-0.323076923076923,
-0.307692307692308,-0.292307692307692,-0.276923076923077,-0.261538461538462,
-0.246153846153846,-0.230769230769231,-0.215384615384615,-0.2,-0.184615384615385,
-0.169230769230769,-0.153846153846154,-0.138461538461538,-0.123076923076923,
-0.107692307692308,-0.0923076923076923,-0.0769230769230769,-0.0615384615384615,
-0.0461538461538462,-0.0307692307692308,-0.0153846153846154,0.),
 .UNSPECIFIED.)
CURVE()
GEOMETRIC_REPRESENTATION_ITEM()
RATIONAL_B_SPLINE_CURVE((1.,1.,1.,1.,1.,1.,1.,1.,1.,1.,1.,1.,1.,1.,1.,1.,
1.,1.,1.,1.,1.,1.,1.,1.,1.,1.,1.,1.,1.,1.,1.,1.,1.,1.,1.,1.,1.,1.,1.,1.,
1.,1.,1.,1.,1.,1.,1.,1.,1.,1.,1.,1.,1.,1.,1.,1.,1.,1.,1.,1.,1.,1.,1.,1.,
1.,1.,1.,1.,1.,1.))
REPRESENTATION_ITEM('')
);
#351=(
BOUNDED_CURVE()
B_SPLINE_CURVE(5,(#58035,#58036,#58037,#58038,#58039,#58040,#58041,#58042,
#58043,#58044,#58045,#58046,#58047,#58048,#58049,#58050,#58051,#58052,#58053,
#58054,#58055,#58056,#58057,#58058,#58059,#58060,#58061,#58062,#58063,#58064,
#58065,#58066,#58067,#58068,#58069,#58070,#58071,#58072,#58073,#58074,#58075,
#58076,#58077,#58078,#58079,#58080,#58081,#58082,#58083,#58084,#58085,#58086,
#58087,#58088,#58089,#58090,#58091,#58092,#58093,#58094,#58095,#58096,#58097,
#58098,#58099,#58100,#58101,#58102,#58103,#58104),.UNSPECIFIED.,.F.,.F.)
B_SPLINE_CURVE_WITH_KNOTS((6,1,1,1,1,1,1,1,1,1,1,1,1,1,1,1,1,1,1,1,1,1,
1,1,1,1,1,1,1,1,1,1,1,1,1,1,1,1,1,1,1,1,1,1,1,1,1,1,1,1,1,1,1,1,1,1,1,1,
1,1,1,1,1,1,1,6),(-1.,-0.984615384615383,-0.969230769230768,-0.953846153846152,
-0.938461538461537,-0.923076923076922,-0.907692307692306,-0.892307692307691,
-0.876923076923076,-0.86153846153846,-0.846153846153845,-0.83076923076923,
-0.815384615384614,-0.799999999999999,-0.784615384615384,-0.769230769230768,
-0.753846153846153,-0.738461538461538,-0.723076923076922,-0.707692307692307,
-0.692307692307692,-0.676923076923076,-0.661538461538461,-0.646153846153846,
-0.63076923076923,-0.615384615384615,-0.6,-0.584615384615384,-0.569230769230769,
-0.553846153846154,-0.538461538461538,-0.523076923076923,-0.507692307692308,
-0.492307692307692,-0.476923076923077,-0.461538461538462,-0.446153846153846,
-0.430769230769231,-0.415384615384615,-0.4,-0.384615384615385,-0.369230769230769,
-0.353846153846154,-0.338461538461538,-0.323076923076923,-0.307692307692308,
-0.292307692307692,-0.276923076923077,-0.261538461538462,-0.246153846153846,
-0.230769230769231,-0.215384615384615,-0.2,-0.184615384615385,-0.169230769230769,
-0.153846153846154,-0.138461538461538,-0.123076923076923,-0.107692307692308,
-0.0923076923076923,-0.0769230769230769,-0.0615384615384615,-0.0461538461538462,
-0.0307692307692308,-0.0153846153846154,-0.0057718433745009),
 .UNSPECIFIED.)
CURVE()
GEOMETRIC_REPRESENTATION_ITEM()
RATIONAL_B_SPLINE_CURVE((1.,1.,1.,1.,1.,1.,1.,1.,1.,1.,1.,1.,1.,1.,1.,1.,
1.,1.,1.,1.,1.,1.,1.,1.,1.,1.,1.,1.,1.,1.,1.,1.,1.,1.,1.,1.,1.,1.,1.,1.,
1.,1.,1.,1.,1.,1.,1.,1.,1.,1.,1.,1.,1.,1.,1.,1.,1.,1.,1.,1.,1.,1.,1.,1.,
1.,1.,1.,1.,1.,1.))
REPRESENTATION_ITEM('')
);
#352=(
BOUNDED_CURVE()
B_SPLINE_CURVE(5,(#58255,#58256,#58257,#58258,#58259,#58260,#58261,#58262,
#58263,#58264,#58265,#58266,#58267,#58268,#58269,#58270,#58271,#58272,#58273,
#58274,#58275,#58276,#58277,#58278,#58279,#58280,#58281,#58282,#58283,#58284,
#58285,#58286,#58287,#58288,#58289,#58290,#58291,#58292,#58293,#58294,#58295,
#58296,#58297,#58298,#58299,#58300,#58301,#58302,#58303,#58304,#58305,#58306,
#58307,#58308,#58309,#58310,#58311,#58312,#58313,#58314,#58315,#58316,#58317,
#58318,#58319,#58320,#58321,#58322,#58323,#58324),.UNSPECIFIED.,.F.,.F.)
B_SPLINE_CURVE_WITH_KNOTS((6,1,1,1,1,1,1,1,1,1,1,1,1,1,1,1,1,1,1,1,1,1,
1,1,1,1,1,1,1,1,1,1,1,1,1,1,1,1,1,1,1,1,1,1,1,1,1,1,1,1,1,1,1,1,1,1,1,1,
1,1,1,1,1,1,1,6),(-0.99422815673967,-0.984615384615383,-0.969230769230768,
-0.953846153846152,-0.938461538461537,-0.923076923076922,-0.907692307692306,
-0.892307692307691,-0.876923076923076,-0.86153846153846,-0.846153846153845,
-0.83076923076923,-0.815384615384614,-0.799999999999999,-0.784615384615384,
-0.769230769230768,-0.753846153846153,-0.738461538461538,-0.723076923076922,
-0.707692307692307,-0.692307692307692,-0.676923076923076,-0.661538461538461,
-0.646153846153846,-0.63076923076923,-0.615384615384615,-0.6,-0.584615384615384,
-0.569230769230769,-0.553846153846154,-0.538461538461538,-0.523076923076923,
-0.507692307692308,-0.492307692307692,-0.476923076923077,-0.461538461538462,
-0.446153846153846,-0.430769230769231,-0.415384615384615,-0.4,-0.384615384615385,
-0.369230769230769,-0.353846153846154,-0.338461538461538,-0.323076923076923,
-0.307692307692308,-0.292307692307692,-0.276923076923077,-0.261538461538462,
-0.246153846153846,-0.230769230769231,-0.215384615384615,-0.2,-0.184615384615385,
-0.169230769230769,-0.153846153846154,-0.138461538461538,-0.123076923076923,
-0.107692307692308,-0.0923076923076923,-0.0769230769230769,-0.0615384615384615,
-0.0461538461538462,-0.0307692307692308,-0.0153846153846154,0.),
 .UNSPECIFIED.)
CURVE()
GEOMETRIC_REPRESENTATION_ITEM()
RATIONAL_B_SPLINE_CURVE((1.,1.,1.,1.,1.,1.,1.,1.,1.,1.,1.,1.,1.,1.,1.,1.,
1.,1.,1.,1.,1.,1.,1.,1.,1.,1.,1.,1.,1.,1.,1.,1.,1.,1.,1.,1.,1.,1.,1.,1.,
1.,1.,1.,1.,1.,1.,1.,1.,1.,1.,1.,1.,1.,1.,1.,1.,1.,1.,1.,1.,1.,1.,1.,1.,
1.,1.,1.,1.,1.,1.))
REPRESENTATION_ITEM('')
);
#353=(
BOUNDED_CURVE()
B_SPLINE_CURVE(5,(#58477,#58478,#58479,#58480,#58481,#58482,#58483,#58484,
#58485,#58486,#58487,#58488,#58489,#58490,#58491,#58492,#58493,#58494,#58495,
#58496,#58497,#58498,#58499,#58500,#58501,#58502,#58503,#58504,#58505,#58506,
#58507,#58508,#58509,#58510,#58511,#58512,#58513,#58514,#58515,#58516,#58517,
#58518,#58519,#58520,#58521,#58522,#58523,#58524,#58525,#58526,#58527,#58528,
#58529,#58530,#58531,#58532,#58533,#58534,#58535,#58536,#58537,#58538,#58539,
#58540,#58541,#58542,#58543,#58544,#58545,#58546),.UNSPECIFIED.,.F.,.F.)
B_SPLINE_CURVE_WITH_KNOTS((6,1,1,1,1,1,1,1,1,1,1,1,1,1,1,1,1,1,1,1,1,1,
1,1,1,1,1,1,1,1,1,1,1,1,1,1,1,1,1,1,1,1,1,1,1,1,1,1,1,1,1,1,1,1,1,1,1,1,
1,1,1,1,1,1,1,6),(-1.,-0.984615384615383,-0.969230769230768,-0.953846153846152,
-0.938461538461537,-0.923076923076922,-0.907692307692306,-0.892307692307691,
-0.876923076923076,-0.86153846153846,-0.846153846153845,-0.83076923076923,
-0.815384615384614,-0.799999999999999,-0.784615384615384,-0.769230769230768,
-0.753846153846153,-0.738461538461538,-0.723076923076922,-0.707692307692307,
-0.692307692307692,-0.676923076923076,-0.661538461538461,-0.646153846153846,
-0.63076923076923,-0.615384615384615,-0.6,-0.584615384615384,-0.569230769230769,
-0.553846153846154,-0.538461538461538,-0.523076923076923,-0.507692307692308,
-0.492307692307692,-0.476923076923077,-0.461538461538462,-0.446153846153846,
-0.430769230769231,-0.415384615384615,-0.4,-0.384615384615385,-0.369230769230769,
-0.353846153846154,-0.338461538461538,-0.323076923076923,-0.307692307692308,
-0.292307692307692,-0.276923076923077,-0.261538461538462,-0.246153846153846,
-0.230769230769231,-0.215384615384615,-0.2,-0.184615384615385,-0.169230769230769,
-0.153846153846154,-0.138461538461538,-0.123076923076923,-0.107692307692308,
-0.0923076923076923,-0.0769230769230769,-0.0615384615384615,-0.0461538461538462,
-0.0307692307692308,-0.0153846153846154,-0.00577184337450701),
 .UNSPECIFIED.)
CURVE()
GEOMETRIC_REPRESENTATION_ITEM()
RATIONAL_B_SPLINE_CURVE((1.,1.,1.,1.,1.,1.,1.,1.,1.,1.,1.,1.,1.,1.,1.,1.,
1.,1.,1.,1.,1.,1.,1.,1.,1.,1.,1.,1.,1.,1.,1.,1.,1.,1.,1.,1.,1.,1.,1.,1.,
1.,1.,1.,1.,1.,1.,1.,1.,1.,1.,1.,1.,1.,1.,1.,1.,1.,1.,1.,1.,1.,1.,1.,1.,
1.,1.,1.,1.,1.,1.))
REPRESENTATION_ITEM('')
);
#354=(
BOUNDED_CURVE()
B_SPLINE_CURVE(5,(#58697,#58698,#58699,#58700,#58701,#58702,#58703,#58704,
#58705,#58706,#58707,#58708,#58709,#58710,#58711,#58712,#58713,#58714,#58715,
#58716,#58717,#58718,#58719,#58720,#58721,#58722,#58723,#58724,#58725,#58726,
#58727,#58728,#58729,#58730,#58731,#58732,#58733,#58734,#58735,#58736,#58737,
#58738,#58739,#58740,#58741,#58742,#58743,#58744,#58745,#58746,#58747,#58748,
#58749,#58750,#58751,#58752,#58753,#58754,#58755,#58756,#58757,#58758,#58759,
#58760,#58761,#58762,#58763,#58764,#58765,#58766),.UNSPECIFIED.,.F.,.F.)
B_SPLINE_CURVE_WITH_KNOTS((6,1,1,1,1,1,1,1,1,1,1,1,1,1,1,1,1,1,1,1,1,1,
1,1,1,1,1,1,1,1,1,1,1,1,1,1,1,1,1,1,1,1,1,1,1,1,1,1,1,1,1,1,1,1,1,1,1,1,
1,1,1,1,1,1,1,6),(-0.994228156739689,-0.984615384615383,-0.969230769230768,
-0.953846153846152,-0.938461538461537,-0.923076923076922,-0.907692307692306,
-0.892307692307691,-0.876923076923076,-0.86153846153846,-0.846153846153845,
-0.83076923076923,-0.815384615384614,-0.799999999999999,-0.784615384615384,
-0.769230769230768,-0.753846153846153,-0.738461538461538,-0.723076923076922,
-0.707692307692307,-0.692307692307692,-0.676923076923076,-0.661538461538461,
-0.646153846153846,-0.63076923076923,-0.615384615384615,-0.6,-0.584615384615384,
-0.569230769230769,-0.553846153846154,-0.538461538461538,-0.523076923076923,
-0.507692307692308,-0.492307692307692,-0.476923076923077,-0.461538461538462,
-0.446153846153846,-0.430769230769231,-0.415384615384615,-0.4,-0.384615384615385,
-0.369230769230769,-0.353846153846154,-0.338461538461538,-0.323076923076923,
-0.307692307692308,-0.292307692307692,-0.276923076923077,-0.261538461538462,
-0.246153846153846,-0.230769230769231,-0.215384615384615,-0.2,-0.184615384615385,
-0.169230769230769,-0.153846153846154,-0.138461538461538,-0.123076923076923,
-0.107692307692308,-0.0923076923076923,-0.0769230769230769,-0.0615384615384615,
-0.0461538461538462,-0.0307692307692308,-0.0153846153846154,0.),
 .UNSPECIFIED.)
CURVE()
GEOMETRIC_REPRESENTATION_ITEM()
RATIONAL_B_SPLINE_CURVE((1.,1.,1.,1.,1.,1.,1.,1.,1.,1.,1.,1.,1.,1.,1.,1.,
1.,1.,1.,1.,1.,1.,1.,1.,1.,1.,1.,1.,1.,1.,1.,1.,1.,1.,1.,1.,1.,1.,1.,1.,
1.,1.,1.,1.,1.,1.,1.,1.,1.,1.,1.,1.,1.,1.,1.,1.,1.,1.,1.,1.,1.,1.,1.,1.,
1.,1.,1.,1.,1.,1.))
REPRESENTATION_ITEM('')
);
#355=(
BOUNDED_CURVE()
B_SPLINE_CURVE(5,(#58919,#58920,#58921,#58922,#58923,#58924,#58925,#58926,
#58927,#58928,#58929,#58930,#58931,#58932,#58933,#58934,#58935,#58936,#58937,
#58938,#58939,#58940,#58941,#58942,#58943,#58944,#58945,#58946,#58947,#58948,
#58949,#58950,#58951,#58952,#58953,#58954,#58955,#58956,#58957,#58958,#58959,
#58960,#58961,#58962,#58963,#58964,#58965,#58966,#58967,#58968,#58969,#58970,
#58971,#58972,#58973,#58974,#58975,#58976,#58977,#58978,#58979,#58980,#58981,
#58982,#58983,#58984,#58985,#58986,#58987,#58988),.UNSPECIFIED.,.F.,.F.)
B_SPLINE_CURVE_WITH_KNOTS((6,1,1,1,1,1,1,1,1,1,1,1,1,1,1,1,1,1,1,1,1,1,
1,1,1,1,1,1,1,1,1,1,1,1,1,1,1,1,1,1,1,1,1,1,1,1,1,1,1,1,1,1,1,1,1,1,1,1,
1,1,1,1,1,1,1,6),(-1.,-0.984615384615383,-0.969230769230768,-0.953846153846152,
-0.938461538461537,-0.923076923076922,-0.907692307692306,-0.892307692307691,
-0.876923076923076,-0.86153846153846,-0.846153846153845,-0.83076923076923,
-0.815384615384614,-0.799999999999999,-0.784615384615384,-0.769230769230768,
-0.753846153846153,-0.738461538461538,-0.723076923076922,-0.707692307692307,
-0.692307692307692,-0.676923076923076,-0.661538461538461,-0.646153846153846,
-0.63076923076923,-0.615384615384615,-0.6,-0.584615384615384,-0.569230769230769,
-0.553846153846154,-0.538461538461538,-0.523076923076923,-0.507692307692308,
-0.492307692307692,-0.476923076923077,-0.461538461538462,-0.446153846153846,
-0.430769230769231,-0.415384615384615,-0.4,-0.384615384615385,-0.369230769230769,
-0.353846153846154,-0.338461538461538,-0.323076923076923,-0.307692307692308,
-0.292307692307692,-0.276923076923077,-0.261538461538462,-0.246153846153846,
-0.230769230769231,-0.215384615384615,-0.2,-0.184615384615385,-0.169230769230769,
-0.153846153846154,-0.138461538461538,-0.123076923076923,-0.107692307692308,
-0.0923076923076923,-0.0769230769230769,-0.0615384615384615,-0.0461538461538462,
-0.0307692307692308,-0.0153846153846154,-0.00577184337452382),
 .UNSPECIFIED.)
CURVE()
GEOMETRIC_REPRESENTATION_ITEM()
RATIONAL_B_SPLINE_CURVE((1.,1.,1.,1.,1.,1.,1.,1.,1.,1.,1.,1.,1.,1.,1.,1.,
1.,1.,1.,1.,1.,1.,1.,1.,1.,1.,1.,1.,1.,1.,1.,1.,1.,1.,1.,1.,1.,1.,1.,1.,
1.,1.,1.,1.,1.,1.,1.,1.,1.,1.,1.,1.,1.,1.,1.,1.,1.,1.,1.,1.,1.,1.,1.,1.,
1.,1.,1.,1.,1.,1.))
REPRESENTATION_ITEM('')
);
#356=(
BOUNDED_CURVE()
B_SPLINE_CURVE(5,(#59139,#59140,#59141,#59142,#59143,#59144,#59145,#59146,
#59147,#59148,#59149,#59150,#59151,#59152,#59153,#59154,#59155,#59156,#59157,
#59158,#59159,#59160,#59161,#59162,#59163,#59164,#59165,#59166,#59167,#59168,
#59169,#59170,#59171,#59172,#59173,#59174,#59175,#59176,#59177,#59178,#59179,
#59180,#59181,#59182,#59183,#59184,#59185,#59186,#59187,#59188,#59189,#59190,
#59191,#59192,#59193,#59194,#59195,#59196,#59197,#59198,#59199,#59200,#59201,
#59202,#59203,#59204,#59205,#59206,#59207,#59208),.UNSPECIFIED.,.F.,.F.)
B_SPLINE_CURVE_WITH_KNOTS((6,1,1,1,1,1,1,1,1,1,1,1,1,1,1,1,1,1,1,1,1,1,
1,1,1,1,1,1,1,1,1,1,1,1,1,1,1,1,1,1,1,1,1,1,1,1,1,1,1,1,1,1,1,1,1,1,1,1,
1,1,1,1,1,1,1,6),(-0.994228156739677,-0.984615384615383,-0.969230769230768,
-0.953846153846152,-0.938461538461537,-0.923076923076922,-0.907692307692306,
-0.892307692307691,-0.876923076923076,-0.86153846153846,-0.846153846153845,
-0.83076923076923,-0.815384615384614,-0.799999999999999,-0.784615384615384,
-0.769230769230768,-0.753846153846153,-0.738461538461538,-0.723076923076922,
-0.707692307692307,-0.692307692307692,-0.676923076923076,-0.661538461538461,
-0.646153846153846,-0.63076923076923,-0.615384615384615,-0.6,-0.584615384615384,
-0.569230769230769,-0.553846153846154,-0.538461538461538,-0.523076923076923,
-0.507692307692308,-0.492307692307692,-0.476923076923077,-0.461538461538462,
-0.446153846153846,-0.430769230769231,-0.415384615384615,-0.4,-0.384615384615385,
-0.369230769230769,-0.353846153846154,-0.338461538461538,-0.323076923076923,
-0.307692307692308,-0.292307692307692,-0.276923076923077,-0.261538461538462,
-0.246153846153846,-0.230769230769231,-0.215384615384615,-0.2,-0.184615384615385,
-0.169230769230769,-0.153846153846154,-0.138461538461538,-0.123076923076923,
-0.107692307692308,-0.0923076923076923,-0.0769230769230769,-0.0615384615384615,
-0.0461538461538462,-0.0307692307692308,-0.0153846153846154,0.),
 .UNSPECIFIED.)
CURVE()
GEOMETRIC_REPRESENTATION_ITEM()
RATIONAL_B_SPLINE_CURVE((1.,1.,1.,1.,1.,1.,1.,1.,1.,1.,1.,1.,1.,1.,1.,1.,
1.,1.,1.,1.,1.,1.,1.,1.,1.,1.,1.,1.,1.,1.,1.,1.,1.,1.,1.,1.,1.,1.,1.,1.,
1.,1.,1.,1.,1.,1.,1.,1.,1.,1.,1.,1.,1.,1.,1.,1.,1.,1.,1.,1.,1.,1.,1.,1.,
1.,1.,1.,1.,1.,1.))
REPRESENTATION_ITEM('')
);
#357=(
BOUNDED_CURVE()
B_SPLINE_CURVE(5,(#59361,#59362,#59363,#59364,#59365,#59366,#59367,#59368,
#59369,#59370,#59371,#59372,#59373,#59374,#59375,#59376,#59377,#59378,#59379,
#59380,#59381,#59382,#59383,#59384,#59385,#59386,#59387,#59388,#59389,#59390,
#59391,#59392,#59393,#59394,#59395,#59396,#59397,#59398,#59399,#59400,#59401,
#59402,#59403,#59404,#59405,#59406,#59407,#59408,#59409,#59410,#59411,#59412,
#59413,#59414,#59415,#59416,#59417,#59418,#59419,#59420,#59421,#59422,#59423,
#59424,#59425,#59426,#59427,#59428,#59429,#59430),.UNSPECIFIED.,.F.,.F.)
B_SPLINE_CURVE_WITH_KNOTS((6,1,1,1,1,1,1,1,1,1,1,1,1,1,1,1,1,1,1,1,1,1,
1,1,1,1,1,1,1,1,1,1,1,1,1,1,1,1,1,1,1,1,1,1,1,1,1,1,1,1,1,1,1,1,1,1,1,1,
1,1,1,1,1,1,1,6),(-1.,-0.984615384615383,-0.969230769230768,-0.953846153846152,
-0.938461538461537,-0.923076923076922,-0.907692307692306,-0.892307692307691,
-0.876923076923076,-0.86153846153846,-0.846153846153845,-0.83076923076923,
-0.815384615384614,-0.799999999999999,-0.784615384615384,-0.769230769230768,
-0.753846153846153,-0.738461538461538,-0.723076923076922,-0.707692307692307,
-0.692307692307692,-0.676923076923076,-0.661538461538461,-0.646153846153846,
-0.63076923076923,-0.615384615384615,-0.6,-0.584615384615384,-0.569230769230769,
-0.553846153846154,-0.538461538461538,-0.523076923076923,-0.507692307692308,
-0.492307692307692,-0.476923076923077,-0.461538461538462,-0.446153846153846,
-0.430769230769231,-0.415384615384615,-0.4,-0.384615384615385,-0.369230769230769,
-0.353846153846154,-0.338461538461538,-0.323076923076923,-0.307692307692308,
-0.292307692307692,-0.276923076923077,-0.261538461538462,-0.246153846153846,
-0.230769230769231,-0.215384615384615,-0.2,-0.184615384615385,-0.169230769230769,
-0.153846153846154,-0.138461538461538,-0.123076923076923,-0.107692307692308,
-0.0923076923076923,-0.0769230769230769,-0.0615384615384615,-0.0461538461538462,
-0.0307692307692308,-0.0153846153846154,-0.0057718433744938),
 .UNSPECIFIED.)
CURVE()
GEOMETRIC_REPRESENTATION_ITEM()
RATIONAL_B_SPLINE_CURVE((1.,1.,1.,1.,1.,1.,1.,1.,1.,1.,1.,1.,1.,1.,1.,1.,
1.,1.,1.,1.,1.,1.,1.,1.,1.,1.,1.,1.,1.,1.,1.,1.,1.,1.,1.,1.,1.,1.,1.,1.,
1.,1.,1.,1.,1.,1.,1.,1.,1.,1.,1.,1.,1.,1.,1.,1.,1.,1.,1.,1.,1.,1.,1.,1.,
1.,1.,1.,1.,1.,1.))
REPRESENTATION_ITEM('')
);
#358=(
BOUNDED_CURVE()
B_SPLINE_CURVE(5,(#59581,#59582,#59583,#59584,#59585,#59586,#59587,#59588,
#59589,#59590,#59591,#59592,#59593,#59594,#59595,#59596,#59597,#59598,#59599,
#59600,#59601,#59602,#59603,#59604,#59605,#59606,#59607,#59608,#59609,#59610,
#59611,#59612,#59613,#59614,#59615,#59616,#59617,#59618,#59619,#59620,#59621,
#59622,#59623,#59624,#59625,#59626,#59627,#59628,#59629,#59630,#59631,#59632,
#59633,#59634,#59635,#59636,#59637,#59638,#59639,#59640,#59641,#59642,#59643,
#59644,#59645,#59646,#59647,#59648,#59649,#59650),.UNSPECIFIED.,.F.,.F.)
B_SPLINE_CURVE_WITH_KNOTS((6,1,1,1,1,1,1,1,1,1,1,1,1,1,1,1,1,1,1,1,1,1,
1,1,1,1,1,1,1,1,1,1,1,1,1,1,1,1,1,1,1,1,1,1,1,1,1,1,1,1,1,1,1,1,1,1,1,1,
1,1,1,1,1,1,1,6),(-0.994228156739743,-0.984615384615383,-0.969230769230768,
-0.953846153846152,-0.938461538461537,-0.923076923076922,-0.907692307692306,
-0.892307692307691,-0.876923076923076,-0.86153846153846,-0.846153846153845,
-0.83076923076923,-0.815384615384614,-0.799999999999999,-0.784615384615384,
-0.769230769230768,-0.753846153846153,-0.738461538461538,-0.723076923076922,
-0.707692307692307,-0.692307692307692,-0.676923076923076,-0.661538461538461,
-0.646153846153846,-0.63076923076923,-0.615384615384615,-0.6,-0.584615384615384,
-0.569230769230769,-0.553846153846154,-0.538461538461538,-0.523076923076923,
-0.507692307692308,-0.492307692307692,-0.476923076923077,-0.461538461538462,
-0.446153846153846,-0.430769230769231,-0.415384615384615,-0.4,-0.384615384615385,
-0.369230769230769,-0.353846153846154,-0.338461538461538,-0.323076923076923,
-0.307692307692308,-0.292307692307692,-0.276923076923077,-0.261538461538462,
-0.246153846153846,-0.230769230769231,-0.215384615384615,-0.2,-0.184615384615385,
-0.169230769230769,-0.153846153846154,-0.138461538461538,-0.123076923076923,
-0.107692307692308,-0.0923076923076923,-0.0769230769230769,-0.0615384615384615,
-0.0461538461538462,-0.0307692307692308,-0.0153846153846154,0.),
 .UNSPECIFIED.)
CURVE()
GEOMETRIC_REPRESENTATION_ITEM()
RATIONAL_B_SPLINE_CURVE((1.,1.,1.,1.,1.,1.,1.,1.,1.,1.,1.,1.,1.,1.,1.,1.,
1.,1.,1.,1.,1.,1.,1.,1.,1.,1.,1.,1.,1.,1.,1.,1.,1.,1.,1.,1.,1.,1.,1.,1.,
1.,1.,1.,1.,1.,1.,1.,1.,1.,1.,1.,1.,1.,1.,1.,1.,1.,1.,1.,1.,1.,1.,1.,1.,
1.,1.,1.,1.,1.,1.))
REPRESENTATION_ITEM('')
);
#359=(
BOUNDED_CURVE()
B_SPLINE_CURVE(5,(#59803,#59804,#59805,#59806,#59807,#59808,#59809,#59810,
#59811,#59812,#59813,#59814,#59815,#59816,#59817,#59818,#59819,#59820,#59821,
#59822,#59823,#59824,#59825,#59826,#59827,#59828,#59829,#59830,#59831,#59832,
#59833,#59834,#59835,#59836,#59837,#59838,#59839,#59840,#59841,#59842,#59843,
#59844,#59845,#59846,#59847,#59848,#59849,#59850,#59851,#59852,#59853,#59854,
#59855,#59856,#59857,#59858,#59859,#59860,#59861,#59862,#59863,#59864,#59865,
#59866,#59867,#59868,#59869,#59870,#59871,#59872),.UNSPECIFIED.,.F.,.F.)
B_SPLINE_CURVE_WITH_KNOTS((6,1,1,1,1,1,1,1,1,1,1,1,1,1,1,1,1,1,1,1,1,1,
1,1,1,1,1,1,1,1,1,1,1,1,1,1,1,1,1,1,1,1,1,1,1,1,1,1,1,1,1,1,1,1,1,1,1,1,
1,1,1,1,1,1,1,6),(-1.,-0.984615384615383,-0.969230769230768,-0.953846153846152,
-0.938461538461537,-0.923076923076922,-0.907692307692306,-0.892307692307691,
-0.876923076923076,-0.86153846153846,-0.846153846153845,-0.83076923076923,
-0.815384615384614,-0.799999999999999,-0.784615384615384,-0.769230769230768,
-0.753846153846153,-0.738461538461538,-0.723076923076922,-0.707692307692307,
-0.692307692307692,-0.676923076923076,-0.661538461538461,-0.646153846153846,
-0.63076923076923,-0.615384615384615,-0.6,-0.584615384615384,-0.569230769230769,
-0.553846153846154,-0.538461538461538,-0.523076923076923,-0.507692307692308,
-0.492307692307692,-0.476923076923077,-0.461538461538462,-0.446153846153846,
-0.430769230769231,-0.415384615384615,-0.4,-0.384615384615385,-0.369230769230769,
-0.353846153846154,-0.338461538461538,-0.323076923076923,-0.307692307692308,
-0.292307692307692,-0.276923076923077,-0.261538461538462,-0.246153846153846,
-0.230769230769231,-0.215384615384615,-0.2,-0.184615384615385,-0.169230769230769,
-0.153846153846154,-0.138461538461538,-0.123076923076923,-0.107692307692308,
-0.0923076923076923,-0.0769230769230769,-0.0615384615384615,-0.0461538461538462,
-0.0307692307692308,-0.0153846153846154,-0.0057718433745291),
 .UNSPECIFIED.)
CURVE()
GEOMETRIC_REPRESENTATION_ITEM()
RATIONAL_B_SPLINE_CURVE((1.,1.,1.,1.,1.,1.,1.,1.,1.,1.,1.,1.,1.,1.,1.,1.,
1.,1.,1.,1.,1.,1.,1.,1.,1.,1.,1.,1.,1.,1.,1.,1.,1.,1.,1.,1.,1.,1.,1.,1.,
1.,1.,1.,1.,1.,1.,1.,1.,1.,1.,1.,1.,1.,1.,1.,1.,1.,1.,1.,1.,1.,1.,1.,1.,
1.,1.,1.,1.,1.,1.))
REPRESENTATION_ITEM('')
);
#360=(
BOUNDED_CURVE()
B_SPLINE_CURVE(5,(#60023,#60024,#60025,#60026,#60027,#60028,#60029,#60030,
#60031,#60032,#60033,#60034,#60035,#60036,#60037,#60038,#60039,#60040,#60041,
#60042,#60043,#60044,#60045,#60046,#60047,#60048,#60049,#60050,#60051,#60052,
#60053,#60054,#60055,#60056,#60057,#60058,#60059,#60060,#60061,#60062,#60063,
#60064,#60065,#60066,#60067,#60068,#60069,#60070,#60071,#60072,#60073,#60074,
#60075,#60076,#60077,#60078,#60079,#60080,#60081,#60082,#60083,#60084,#60085,
#60086,#60087,#60088,#60089,#60090,#60091,#60092),.UNSPECIFIED.,.F.,.F.)
B_SPLINE_CURVE_WITH_KNOTS((6,1,1,1,1,1,1,1,1,1,1,1,1,1,1,1,1,1,1,1,1,1,
1,1,1,1,1,1,1,1,1,1,1,1,1,1,1,1,1,1,1,1,1,1,1,1,1,1,1,1,1,1,1,1,1,1,1,1,
1,1,1,1,1,1,1,6),(-0.994228156739665,-0.984615384615383,-0.969230769230768,
-0.953846153846152,-0.938461538461537,-0.923076923076922,-0.907692307692306,
-0.892307692307691,-0.876923076923076,-0.86153846153846,-0.846153846153845,
-0.83076923076923,-0.815384615384614,-0.799999999999999,-0.784615384615384,
-0.769230769230768,-0.753846153846153,-0.738461538461538,-0.723076923076922,
-0.707692307692307,-0.692307692307692,-0.676923076923076,-0.661538461538461,
-0.646153846153846,-0.63076923076923,-0.615384615384615,-0.6,-0.584615384615384,
-0.569230769230769,-0.553846153846154,-0.538461538461538,-0.523076923076923,
-0.507692307692308,-0.492307692307692,-0.476923076923077,-0.461538461538462,
-0.446153846153846,-0.430769230769231,-0.415384615384615,-0.4,-0.384615384615385,
-0.369230769230769,-0.353846153846154,-0.338461538461538,-0.323076923076923,
-0.307692307692308,-0.292307692307692,-0.276923076923077,-0.261538461538462,
-0.246153846153846,-0.230769230769231,-0.215384615384615,-0.2,-0.184615384615385,
-0.169230769230769,-0.153846153846154,-0.138461538461538,-0.123076923076923,
-0.107692307692308,-0.0923076923076923,-0.0769230769230769,-0.0615384615384615,
-0.0461538461538462,-0.0307692307692308,-0.0153846153846154,0.),
 .UNSPECIFIED.)
CURVE()
GEOMETRIC_REPRESENTATION_ITEM()
RATIONAL_B_SPLINE_CURVE((1.,1.,1.,1.,1.,1.,1.,1.,1.,1.,1.,1.,1.,1.,1.,1.,
1.,1.,1.,1.,1.,1.,1.,1.,1.,1.,1.,1.,1.,1.,1.,1.,1.,1.,1.,1.,1.,1.,1.,1.,
1.,1.,1.,1.,1.,1.,1.,1.,1.,1.,1.,1.,1.,1.,1.,1.,1.,1.,1.,1.,1.,1.,1.,1.,
1.,1.,1.,1.,1.,1.))
REPRESENTATION_ITEM('')
);
#361=(
BOUNDED_CURVE()
B_SPLINE_CURVE(5,(#60245,#60246,#60247,#60248,#60249,#60250,#60251,#60252,
#60253,#60254,#60255,#60256,#60257,#60258,#60259,#60260,#60261,#60262,#60263,
#60264,#60265,#60266,#60267,#60268,#60269,#60270,#60271,#60272,#60273,#60274,
#60275,#60276,#60277,#60278,#60279,#60280,#60281,#60282,#60283,#60284,#60285,
#60286,#60287,#60288,#60289,#60290,#60291,#60292,#60293,#60294,#60295,#60296,
#60297,#60298,#60299,#60300,#60301,#60302,#60303,#60304,#60305,#60306,#60307,
#60308,#60309,#60310,#60311,#60312,#60313,#60314),.UNSPECIFIED.,.F.,.F.)
B_SPLINE_CURVE_WITH_KNOTS((6,1,1,1,1,1,1,1,1,1,1,1,1,1,1,1,1,1,1,1,1,1,
1,1,1,1,1,1,1,1,1,1,1,1,1,1,1,1,1,1,1,1,1,1,1,1,1,1,1,1,1,1,1,1,1,1,1,1,
1,1,1,1,1,1,1,6),(-1.,-0.984615384615383,-0.969230769230768,-0.953846153846152,
-0.938461538461537,-0.923076923076922,-0.907692307692306,-0.892307692307691,
-0.876923076923076,-0.86153846153846,-0.846153846153845,-0.83076923076923,
-0.815384615384614,-0.799999999999999,-0.784615384615384,-0.769230769230768,
-0.753846153846153,-0.738461538461538,-0.723076923076922,-0.707692307692307,
-0.692307692307692,-0.676923076923076,-0.661538461538461,-0.646153846153846,
-0.63076923076923,-0.615384615384615,-0.6,-0.584615384615384,-0.569230769230769,
-0.553846153846154,-0.538461538461538,-0.523076923076923,-0.507692307692308,
-0.492307692307692,-0.476923076923077,-0.461538461538462,-0.446153846153846,
-0.430769230769231,-0.415384615384615,-0.4,-0.384615384615385,-0.369230769230769,
-0.353846153846154,-0.338461538461538,-0.323076923076923,-0.307692307692308,
-0.292307692307692,-0.276923076923077,-0.261538461538462,-0.246153846153846,
-0.230769230769231,-0.215384615384615,-0.2,-0.184615384615385,-0.169230769230769,
-0.153846153846154,-0.138461538461538,-0.123076923076923,-0.107692307692308,
-0.0923076923076923,-0.0769230769230769,-0.0615384615384615,-0.0461538461538462,
-0.0307692307692308,-0.0153846153846154,-0.00577184337450666),
 .UNSPECIFIED.)
CURVE()
GEOMETRIC_REPRESENTATION_ITEM()
RATIONAL_B_SPLINE_CURVE((1.,1.,1.,1.,1.,1.,1.,1.,1.,1.,1.,1.,1.,1.,1.,1.,
1.,1.,1.,1.,1.,1.,1.,1.,1.,1.,1.,1.,1.,1.,1.,1.,1.,1.,1.,1.,1.,1.,1.,1.,
1.,1.,1.,1.,1.,1.,1.,1.,1.,1.,1.,1.,1.,1.,1.,1.,1.,1.,1.,1.,1.,1.,1.,1.,
1.,1.,1.,1.,1.,1.))
REPRESENTATION_ITEM('')
);
#362=(
BOUNDED_CURVE()
B_SPLINE_CURVE(5,(#60465,#60466,#60467,#60468,#60469,#60470,#60471,#60472,
#60473,#60474,#60475,#60476,#60477,#60478,#60479,#60480,#60481,#60482,#60483,
#60484,#60485,#60486,#60487,#60488,#60489,#60490,#60491,#60492,#60493,#60494,
#60495,#60496,#60497,#60498,#60499,#60500,#60501,#60502,#60503,#60504,#60505,
#60506,#60507,#60508,#60509,#60510,#60511,#60512,#60513,#60514,#60515,#60516,
#60517,#60518,#60519,#60520,#60521,#60522,#60523,#60524,#60525,#60526,#60527,
#60528,#60529,#60530,#60531,#60532,#60533,#60534),.UNSPECIFIED.,.F.,.F.)
B_SPLINE_CURVE_WITH_KNOTS((6,1,1,1,1,1,1,1,1,1,1,1,1,1,1,1,1,1,1,1,1,1,
1,1,1,1,1,1,1,1,1,1,1,1,1,1,1,1,1,1,1,1,1,1,1,1,1,1,1,1,1,1,1,1,1,1,1,1,
1,1,1,1,1,1,1,6),(-0.994228156739758,-0.984615384615383,-0.969230769230768,
-0.953846153846152,-0.938461538461537,-0.923076923076922,-0.907692307692306,
-0.892307692307691,-0.876923076923076,-0.86153846153846,-0.846153846153845,
-0.83076923076923,-0.815384615384614,-0.799999999999999,-0.784615384615384,
-0.769230769230768,-0.753846153846153,-0.738461538461538,-0.723076923076922,
-0.707692307692307,-0.692307692307692,-0.676923076923076,-0.661538461538461,
-0.646153846153846,-0.63076923076923,-0.615384615384615,-0.6,-0.584615384615384,
-0.569230769230769,-0.553846153846154,-0.538461538461538,-0.523076923076923,
-0.507692307692308,-0.492307692307692,-0.476923076923077,-0.461538461538462,
-0.446153846153846,-0.430769230769231,-0.415384615384615,-0.4,-0.384615384615385,
-0.369230769230769,-0.353846153846154,-0.338461538461538,-0.323076923076923,
-0.307692307692308,-0.292307692307692,-0.276923076923077,-0.261538461538462,
-0.246153846153846,-0.230769230769231,-0.215384615384615,-0.2,-0.184615384615385,
-0.169230769230769,-0.153846153846154,-0.138461538461538,-0.123076923076923,
-0.107692307692308,-0.0923076923076923,-0.0769230769230769,-0.0615384615384615,
-0.0461538461538462,-0.0307692307692308,-0.0153846153846154,0.),
 .UNSPECIFIED.)
CURVE()
GEOMETRIC_REPRESENTATION_ITEM()
RATIONAL_B_SPLINE_CURVE((1.,1.,1.,1.,1.,1.,1.,1.,1.,1.,1.,1.,1.,1.,1.,1.,
1.,1.,1.,1.,1.,1.,1.,1.,1.,1.,1.,1.,1.,1.,1.,1.,1.,1.,1.,1.,1.,1.,1.,1.,
1.,1.,1.,1.,1.,1.,1.,1.,1.,1.,1.,1.,1.,1.,1.,1.,1.,1.,1.,1.,1.,1.,1.,1.,
1.,1.,1.,1.,1.,1.))
REPRESENTATION_ITEM('')
);
#363=(
BOUNDED_CURVE()
B_SPLINE_CURVE(5,(#60687,#60688,#60689,#60690,#60691,#60692,#60693,#60694,
#60695,#60696,#60697,#60698,#60699,#60700,#60701,#60702,#60703,#60704,#60705,
#60706,#60707,#60708,#60709,#60710,#60711,#60712,#60713,#60714,#60715,#60716,
#60717,#60718,#60719,#60720,#60721,#60722,#60723,#60724,#60725,#60726,#60727,
#60728,#60729,#60730,#60731,#60732,#60733,#60734,#60735,#60736,#60737,#60738,
#60739,#60740,#60741,#60742,#60743,#60744,#60745,#60746,#60747,#60748,#60749,
#60750,#60751,#60752,#60753,#60754,#60755,#60756),.UNSPECIFIED.,.F.,.F.)
B_SPLINE_CURVE_WITH_KNOTS((6,1,1,1,1,1,1,1,1,1,1,1,1,1,1,1,1,1,1,1,1,1,
1,1,1,1,1,1,1,1,1,1,1,1,1,1,1,1,1,1,1,1,1,1,1,1,1,1,1,1,1,1,1,1,1,1,1,1,
1,1,1,1,1,1,1,6),(-1.,-0.984615384615383,-0.969230769230768,-0.953846153846152,
-0.938461538461537,-0.923076923076922,-0.907692307692306,-0.892307692307691,
-0.876923076923076,-0.86153846153846,-0.846153846153845,-0.83076923076923,
-0.815384615384614,-0.799999999999999,-0.784615384615384,-0.769230769230768,
-0.753846153846153,-0.738461538461538,-0.723076923076922,-0.707692307692307,
-0.692307692307692,-0.676923076923076,-0.661538461538461,-0.646153846153846,
-0.63076923076923,-0.615384615384615,-0.6,-0.584615384615384,-0.569230769230769,
-0.553846153846154,-0.538461538461538,-0.523076923076923,-0.507692307692308,
-0.492307692307692,-0.476923076923077,-0.461538461538462,-0.446153846153846,
-0.430769230769231,-0.415384615384615,-0.4,-0.384615384615385,-0.369230769230769,
-0.353846153846154,-0.338461538461538,-0.323076923076923,-0.307692307692308,
-0.292307692307692,-0.276923076923077,-0.261538461538462,-0.246153846153846,
-0.230769230769231,-0.215384615384615,-0.2,-0.184615384615385,-0.169230769230769,
-0.153846153846154,-0.138461538461538,-0.123076923076923,-0.107692307692308,
-0.0923076923076923,-0.0769230769230769,-0.0615384615384615,-0.0461538461538462,
-0.0307692307692308,-0.0153846153846154,-0.00577184337451981),
 .UNSPECIFIED.)
CURVE()
GEOMETRIC_REPRESENTATION_ITEM()
RATIONAL_B_SPLINE_CURVE((1.,1.,1.,1.,1.,1.,1.,1.,1.,1.,1.,1.,1.,1.,1.,1.,
1.,1.,1.,1.,1.,1.,1.,1.,1.,1.,1.,1.,1.,1.,1.,1.,1.,1.,1.,1.,1.,1.,1.,1.,
1.,1.,1.,1.,1.,1.,1.,1.,1.,1.,1.,1.,1.,1.,1.,1.,1.,1.,1.,1.,1.,1.,1.,1.,
1.,1.,1.,1.,1.,1.))
REPRESENTATION_ITEM('')
);
#364=(
BOUNDED_CURVE()
B_SPLINE_CURVE(5,(#60907,#60908,#60909,#60910,#60911,#60912,#60913,#60914,
#60915,#60916,#60917,#60918,#60919,#60920,#60921,#60922,#60923,#60924,#60925,
#60926,#60927,#60928,#60929,#60930,#60931,#60932,#60933,#60934,#60935,#60936,
#60937,#60938,#60939,#60940,#60941,#60942,#60943,#60944,#60945,#60946,#60947,
#60948,#60949,#60950,#60951,#60952,#60953,#60954,#60955,#60956,#60957,#60958,
#60959,#60960,#60961,#60962,#60963,#60964,#60965,#60966,#60967,#60968,#60969,
#60970,#60971,#60972,#60973,#60974,#60975,#60976),.UNSPECIFIED.,.F.,.F.)
B_SPLINE_CURVE_WITH_KNOTS((6,1,1,1,1,1,1,1,1,1,1,1,1,1,1,1,1,1,1,1,1,1,
1,1,1,1,1,1,1,1,1,1,1,1,1,1,1,1,1,1,1,1,1,1,1,1,1,1,1,1,1,1,1,1,1,1,1,1,
1,1,1,1,1,1,1,6),(-0.994228156739659,-0.984615384615383,-0.969230769230768,
-0.953846153846152,-0.938461538461537,-0.923076923076922,-0.907692307692306,
-0.892307692307691,-0.876923076923076,-0.86153846153846,-0.846153846153845,
-0.83076923076923,-0.815384615384614,-0.799999999999999,-0.784615384615384,
-0.769230769230768,-0.753846153846153,-0.738461538461538,-0.723076923076922,
-0.707692307692307,-0.692307692307692,-0.676923076923076,-0.661538461538461,
-0.646153846153846,-0.63076923076923,-0.615384615384615,-0.6,-0.584615384615384,
-0.569230769230769,-0.553846153846154,-0.538461538461538,-0.523076923076923,
-0.507692307692308,-0.492307692307692,-0.476923076923077,-0.461538461538462,
-0.446153846153846,-0.430769230769231,-0.415384615384615,-0.4,-0.384615384615385,
-0.369230769230769,-0.353846153846154,-0.338461538461538,-0.323076923076923,
-0.307692307692308,-0.292307692307692,-0.276923076923077,-0.261538461538462,
-0.246153846153846,-0.230769230769231,-0.215384615384615,-0.2,-0.184615384615385,
-0.169230769230769,-0.153846153846154,-0.138461538461538,-0.123076923076923,
-0.107692307692308,-0.0923076923076923,-0.0769230769230769,-0.0615384615384615,
-0.0461538461538462,-0.0307692307692308,-0.0153846153846154,0.),
 .UNSPECIFIED.)
CURVE()
GEOMETRIC_REPRESENTATION_ITEM()
RATIONAL_B_SPLINE_CURVE((1.,1.,1.,1.,1.,1.,1.,1.,1.,1.,1.,1.,1.,1.,1.,1.,
1.,1.,1.,1.,1.,1.,1.,1.,1.,1.,1.,1.,1.,1.,1.,1.,1.,1.,1.,1.,1.,1.,1.,1.,
1.,1.,1.,1.,1.,1.,1.,1.,1.,1.,1.,1.,1.,1.,1.,1.,1.,1.,1.,1.,1.,1.,1.,1.,
1.,1.,1.,1.,1.,1.))
REPRESENTATION_ITEM('')
);
#365=(
BOUNDED_CURVE()
B_SPLINE_CURVE(5,(#61129,#61130,#61131,#61132,#61133,#61134,#61135,#61136,
#61137,#61138,#61139,#61140,#61141,#61142,#61143,#61144,#61145,#61146,#61147,
#61148,#61149,#61150,#61151,#61152,#61153,#61154,#61155,#61156,#61157,#61158,
#61159,#61160,#61161,#61162,#61163,#61164,#61165,#61166,#61167,#61168,#61169,
#61170,#61171,#61172,#61173,#61174,#61175,#61176,#61177,#61178,#61179,#61180,
#61181,#61182,#61183,#61184,#61185,#61186,#61187,#61188,#61189,#61190,#61191,
#61192,#61193,#61194,#61195,#61196,#61197,#61198),.UNSPECIFIED.,.F.,.F.)
B_SPLINE_CURVE_WITH_KNOTS((6,1,1,1,1,1,1,1,1,1,1,1,1,1,1,1,1,1,1,1,1,1,
1,1,1,1,1,1,1,1,1,1,1,1,1,1,1,1,1,1,1,1,1,1,1,1,1,1,1,1,1,1,1,1,1,1,1,1,
1,1,1,1,1,1,1,6),(-1.,-0.984615384615383,-0.969230769230768,-0.953846153846152,
-0.938461538461537,-0.923076923076922,-0.907692307692306,-0.892307692307691,
-0.876923076923076,-0.86153846153846,-0.846153846153845,-0.83076923076923,
-0.815384615384614,-0.799999999999999,-0.784615384615384,-0.769230769230768,
-0.753846153846153,-0.738461538461538,-0.723076923076922,-0.707692307692307,
-0.692307692307692,-0.676923076923076,-0.661538461538461,-0.646153846153846,
-0.63076923076923,-0.615384615384615,-0.6,-0.584615384615384,-0.569230769230769,
-0.553846153846154,-0.538461538461538,-0.523076923076923,-0.507692307692308,
-0.492307692307692,-0.476923076923077,-0.461538461538462,-0.446153846153846,
-0.430769230769231,-0.415384615384615,-0.4,-0.384615384615385,-0.369230769230769,
-0.353846153846154,-0.338461538461538,-0.323076923076923,-0.307692307692308,
-0.292307692307692,-0.276923076923077,-0.261538461538462,-0.246153846153846,
-0.230769230769231,-0.215384615384615,-0.2,-0.184615384615385,-0.169230769230769,
-0.153846153846154,-0.138461538461538,-0.123076923076923,-0.107692307692308,
-0.0923076923076923,-0.0769230769230769,-0.0615384615384615,-0.0461538461538462,
-0.0307692307692308,-0.0153846153846154,-0.00577184337450306),
 .UNSPECIFIED.)
CURVE()
GEOMETRIC_REPRESENTATION_ITEM()
RATIONAL_B_SPLINE_CURVE((1.,1.,1.,1.,1.,1.,1.,1.,1.,1.,1.,1.,1.,1.,1.,1.,
1.,1.,1.,1.,1.,1.,1.,1.,1.,1.,1.,1.,1.,1.,1.,1.,1.,1.,1.,1.,1.,1.,1.,1.,
1.,1.,1.,1.,1.,1.,1.,1.,1.,1.,1.,1.,1.,1.,1.,1.,1.,1.,1.,1.,1.,1.,1.,1.,
1.,1.,1.,1.,1.,1.))
REPRESENTATION_ITEM('')
);
#366=(
BOUNDED_CURVE()
B_SPLINE_CURVE(5,(#61349,#61350,#61351,#61352,#61353,#61354,#61355,#61356,
#61357,#61358,#61359,#61360,#61361,#61362,#61363,#61364,#61365,#61366,#61367,
#61368,#61369,#61370,#61371,#61372,#61373,#61374,#61375,#61376,#61377,#61378,
#61379,#61380,#61381,#61382,#61383,#61384,#61385,#61386,#61387,#61388,#61389,
#61390,#61391,#61392,#61393,#61394,#61395,#61396,#61397,#61398,#61399,#61400,
#61401,#61402,#61403,#61404,#61405,#61406,#61407,#61408,#61409,#61410,#61411,
#61412,#61413,#61414,#61415,#61416,#61417,#61418),.UNSPECIFIED.,.F.,.F.)
B_SPLINE_CURVE_WITH_KNOTS((6,1,1,1,1,1,1,1,1,1,1,1,1,1,1,1,1,1,1,1,1,1,
1,1,1,1,1,1,1,1,1,1,1,1,1,1,1,1,1,1,1,1,1,1,1,1,1,1,1,1,1,1,1,1,1,1,1,1,
1,1,1,1,1,1,1,6),(-0.994228156739675,-0.984615384615383,-0.969230769230768,
-0.953846153846152,-0.938461538461537,-0.923076923076922,-0.907692307692306,
-0.892307692307691,-0.876923076923076,-0.86153846153846,-0.846153846153845,
-0.83076923076923,-0.815384615384614,-0.799999999999999,-0.784615384615384,
-0.769230769230768,-0.753846153846153,-0.738461538461538,-0.723076923076922,
-0.707692307692307,-0.692307692307692,-0.676923076923076,-0.661538461538461,
-0.646153846153846,-0.63076923076923,-0.615384615384615,-0.6,-0.584615384615384,
-0.569230769230769,-0.553846153846154,-0.538461538461538,-0.523076923076923,
-0.507692307692308,-0.492307692307692,-0.476923076923077,-0.461538461538462,
-0.446153846153846,-0.430769230769231,-0.415384615384615,-0.4,-0.384615384615385,
-0.369230769230769,-0.353846153846154,-0.338461538461538,-0.323076923076923,
-0.307692307692308,-0.292307692307692,-0.276923076923077,-0.261538461538462,
-0.246153846153846,-0.230769230769231,-0.215384615384615,-0.2,-0.184615384615385,
-0.169230769230769,-0.153846153846154,-0.138461538461538,-0.123076923076923,
-0.107692307692308,-0.0923076923076923,-0.0769230769230769,-0.0615384615384615,
-0.0461538461538462,-0.0307692307692308,-0.0153846153846154,0.),
 .UNSPECIFIED.)
CURVE()
GEOMETRIC_REPRESENTATION_ITEM()
RATIONAL_B_SPLINE_CURVE((1.,1.,1.,1.,1.,1.,1.,1.,1.,1.,1.,1.,1.,1.,1.,1.,
1.,1.,1.,1.,1.,1.,1.,1.,1.,1.,1.,1.,1.,1.,1.,1.,1.,1.,1.,1.,1.,1.,1.,1.,
1.,1.,1.,1.,1.,1.,1.,1.,1.,1.,1.,1.,1.,1.,1.,1.,1.,1.,1.,1.,1.,1.,1.,1.,
1.,1.,1.,1.,1.,1.))
REPRESENTATION_ITEM('')
);
#367=(
BOUNDED_CURVE()
B_SPLINE_CURVE(5,(#61571,#61572,#61573,#61574,#61575,#61576,#61577,#61578,
#61579,#61580,#61581,#61582,#61583,#61584,#61585,#61586,#61587,#61588,#61589,
#61590,#61591,#61592,#61593,#61594,#61595,#61596,#61597,#61598,#61599,#61600,
#61601,#61602,#61603,#61604,#61605,#61606,#61607,#61608,#61609,#61610,#61611,
#61612,#61613,#61614,#61615,#61616,#61617,#61618,#61619,#61620,#61621,#61622,
#61623,#61624,#61625,#61626,#61627,#61628,#61629,#61630,#61631,#61632,#61633,
#61634,#61635,#61636,#61637,#61638,#61639,#61640),.UNSPECIFIED.,.F.,.F.)
B_SPLINE_CURVE_WITH_KNOTS((6,1,1,1,1,1,1,1,1,1,1,1,1,1,1,1,1,1,1,1,1,1,
1,1,1,1,1,1,1,1,1,1,1,1,1,1,1,1,1,1,1,1,1,1,1,1,1,1,1,1,1,1,1,1,1,1,1,1,
1,1,1,1,1,1,1,6),(-1.,-0.984615384615383,-0.969230769230768,-0.953846153846152,
-0.938461538461537,-0.923076923076922,-0.907692307692306,-0.892307692307691,
-0.876923076923076,-0.86153846153846,-0.846153846153845,-0.83076923076923,
-0.815384615384614,-0.799999999999999,-0.784615384615384,-0.769230769230768,
-0.753846153846153,-0.738461538461538,-0.723076923076922,-0.707692307692307,
-0.692307692307692,-0.676923076923076,-0.661538461538461,-0.646153846153846,
-0.63076923076923,-0.615384615384615,-0.6,-0.584615384615384,-0.569230769230769,
-0.553846153846154,-0.538461538461538,-0.523076923076923,-0.507692307692308,
-0.492307692307692,-0.476923076923077,-0.461538461538462,-0.446153846153846,
-0.430769230769231,-0.415384615384615,-0.4,-0.384615384615385,-0.369230769230769,
-0.353846153846154,-0.338461538461538,-0.323076923076923,-0.307692307692308,
-0.292307692307692,-0.276923076923077,-0.261538461538462,-0.246153846153846,
-0.230769230769231,-0.215384615384615,-0.2,-0.184615384615385,-0.169230769230769,
-0.153846153846154,-0.138461538461538,-0.123076923076923,-0.107692307692308,
-0.0923076923076923,-0.0769230769230769,-0.0615384615384615,-0.0461538461538462,
-0.0307692307692308,-0.0153846153846154,-0.00577184337450328),
 .UNSPECIFIED.)
CURVE()
GEOMETRIC_REPRESENTATION_ITEM()
RATIONAL_B_SPLINE_CURVE((1.,1.,1.,1.,1.,1.,1.,1.,1.,1.,1.,1.,1.,1.,1.,1.,
1.,1.,1.,1.,1.,1.,1.,1.,1.,1.,1.,1.,1.,1.,1.,1.,1.,1.,1.,1.,1.,1.,1.,1.,
1.,1.,1.,1.,1.,1.,1.,1.,1.,1.,1.,1.,1.,1.,1.,1.,1.,1.,1.,1.,1.,1.,1.,1.,
1.,1.,1.,1.,1.,1.))
REPRESENTATION_ITEM('')
);
#368=(
BOUNDED_CURVE()
B_SPLINE_CURVE(5,(#61793,#61794,#61795,#61796,#61797,#61798,#61799,#61800,
#61801,#61802,#61803,#61804,#61805,#61806,#61807,#61808,#61809,#61810,#61811,
#61812,#61813,#61814,#61815,#61816,#61817,#61818,#61819,#61820,#61821,#61822,
#61823,#61824,#61825,#61826,#61827,#61828,#61829,#61830,#61831,#61832,#61833,
#61834,#61835,#61836,#61837,#61838,#61839,#61840,#61841,#61842,#61843,#61844,
#61845,#61846,#61847,#61848,#61849,#61850,#61851,#61852,#61853,#61854,#61855,
#61856,#61857,#61858,#61859,#61860,#61861,#61862),.UNSPECIFIED.,.F.,.F.)
B_SPLINE_CURVE_WITH_KNOTS((6,1,1,1,1,1,1,1,1,1,1,1,1,1,1,1,1,1,1,1,1,1,
1,1,1,1,1,1,1,1,1,1,1,1,1,1,1,1,1,1,1,1,1,1,1,1,1,1,1,1,1,1,1,1,1,1,1,1,
1,1,1,1,1,1,1,6),(-0.994228156739672,-0.984615384615383,-0.969230769230768,
-0.953846153846152,-0.938461538461537,-0.923076923076922,-0.907692307692306,
-0.892307692307691,-0.876923076923076,-0.86153846153846,-0.846153846153845,
-0.83076923076923,-0.815384615384614,-0.799999999999999,-0.784615384615384,
-0.769230769230768,-0.753846153846153,-0.738461538461538,-0.723076923076922,
-0.707692307692307,-0.692307692307692,-0.676923076923076,-0.661538461538461,
-0.646153846153846,-0.63076923076923,-0.615384615384615,-0.6,-0.584615384615384,
-0.569230769230769,-0.553846153846154,-0.538461538461538,-0.523076923076923,
-0.507692307692308,-0.492307692307692,-0.476923076923077,-0.461538461538462,
-0.446153846153846,-0.430769230769231,-0.415384615384615,-0.4,-0.384615384615385,
-0.369230769230769,-0.353846153846154,-0.338461538461538,-0.323076923076923,
-0.307692307692308,-0.292307692307692,-0.276923076923077,-0.261538461538462,
-0.246153846153846,-0.230769230769231,-0.215384615384615,-0.2,-0.184615384615385,
-0.169230769230769,-0.153846153846154,-0.138461538461538,-0.123076923076923,
-0.107692307692308,-0.0923076923076923,-0.0769230769230769,-0.0615384615384615,
-0.0461538461538462,-0.0307692307692308,-0.0153846153846154,0.),
 .UNSPECIFIED.)
CURVE()
GEOMETRIC_REPRESENTATION_ITEM()
RATIONAL_B_SPLINE_CURVE((1.,1.,1.,1.,1.,1.,1.,1.,1.,1.,1.,1.,1.,1.,1.,1.,
1.,1.,1.,1.,1.,1.,1.,1.,1.,1.,1.,1.,1.,1.,1.,1.,1.,1.,1.,1.,1.,1.,1.,1.,
1.,1.,1.,1.,1.,1.,1.,1.,1.,1.,1.,1.,1.,1.,1.,1.,1.,1.,1.,1.,1.,1.,1.,1.,
1.,1.,1.,1.,1.,1.))
REPRESENTATION_ITEM('')
);
#369=(
BOUNDED_CURVE()
B_SPLINE_CURVE(5,(#62021,#62022,#62023,#62024,#62025,#62026,#62027,#62028,
#62029,#62030,#62031,#62032,#62033,#62034,#62035,#62036,#62037,#62038,#62039,
#62040,#62041,#62042,#62043,#62044,#62045,#62046,#62047,#62048,#62049,#62050,
#62051,#62052,#62053,#62054,#62055,#62056,#62057,#62058,#62059,#62060,#62061,
#62062,#62063,#62064,#62065,#62066,#62067,#62068,#62069,#62070,#62071,#62072,
#62073,#62074,#62075,#62076,#62077,#62078,#62079,#62080,#62081,#62082,#62083,
#62084,#62085,#62086,#62087,#62088,#62089,#62090),.UNSPECIFIED.,.F.,.F.)
B_SPLINE_CURVE_WITH_KNOTS((6,1,1,1,1,1,1,1,1,1,1,1,1,1,1,1,1,1,1,1,1,1,
1,1,1,1,1,1,1,1,1,1,1,1,1,1,1,1,1,1,1,1,1,1,1,1,1,1,1,1,1,1,1,1,1,1,1,1,
1,1,1,1,1,1,1,6),(-0.994228156739704,-0.984615384615383,-0.969230769230768,
-0.953846153846152,-0.938461538461537,-0.923076923076922,-0.907692307692306,
-0.892307692307691,-0.876923076923076,-0.86153846153846,-0.846153846153845,
-0.83076923076923,-0.815384615384614,-0.799999999999999,-0.784615384615384,
-0.769230769230768,-0.753846153846153,-0.738461538461538,-0.723076923076922,
-0.707692307692307,-0.692307692307692,-0.676923076923076,-0.661538461538461,
-0.646153846153846,-0.63076923076923,-0.615384615384615,-0.6,-0.584615384615384,
-0.569230769230769,-0.553846153846154,-0.538461538461538,-0.523076923076923,
-0.507692307692308,-0.492307692307692,-0.476923076923077,-0.461538461538462,
-0.446153846153846,-0.430769230769231,-0.415384615384615,-0.4,-0.384615384615385,
-0.369230769230769,-0.353846153846154,-0.338461538461538,-0.323076923076923,
-0.307692307692308,-0.292307692307692,-0.276923076923077,-0.261538461538462,
-0.246153846153846,-0.230769230769231,-0.215384615384615,-0.2,-0.184615384615385,
-0.169230769230769,-0.153846153846154,-0.138461538461538,-0.123076923076923,
-0.107692307692308,-0.0923076923076923,-0.0769230769230769,-0.0615384615384615,
-0.0461538461538462,-0.0307692307692308,-0.0153846153846154,0.),
 .UNSPECIFIED.)
CURVE()
GEOMETRIC_REPRESENTATION_ITEM()
RATIONAL_B_SPLINE_CURVE((1.,1.,1.,1.,1.,1.,1.,1.,1.,1.,1.,1.,1.,1.,1.,1.,
1.,1.,1.,1.,1.,1.,1.,1.,1.,1.,1.,1.,1.,1.,1.,1.,1.,1.,1.,1.,1.,1.,1.,1.,
1.,1.,1.,1.,1.,1.,1.,1.,1.,1.,1.,1.,1.,1.,1.,1.,1.,1.,1.,1.,1.,1.,1.,1.,
1.,1.,1.,1.,1.,1.))
REPRESENTATION_ITEM('')
);
#370=(
BOUNDED_CURVE()
B_SPLINE_CURVE(5,(#62232,#62233,#62234,#62235,#62236,#62237,#62238,#62239,
#62240,#62241,#62242,#62243,#62244,#62245,#62246,#62247,#62248,#62249,#62250,
#62251,#62252,#62253,#62254,#62255,#62256,#62257,#62258,#62259,#62260,#62261,
#62262,#62263,#62264,#62265,#62266,#62267,#62268,#62269,#62270,#62271,#62272,
#62273,#62274,#62275,#62276,#62277,#62278,#62279,#62280,#62281,#62282,#62283,
#62284,#62285,#62286,#62287,#62288,#62289,#62290,#62291,#62292,#62293,#62294,
#62295,#62296,#62297,#62298,#62299,#62300,#62301),.UNSPECIFIED.,.F.,.F.)
B_SPLINE_CURVE_WITH_KNOTS((6,1,1,1,1,1,1,1,1,1,1,1,1,1,1,1,1,1,1,1,1,1,
1,1,1,1,1,1,1,1,1,1,1,1,1,1,1,1,1,1,1,1,1,1,1,1,1,1,1,1,1,1,1,1,1,1,1,1,
1,1,1,1,1,1,1,6),(-1.,-0.984615384615383,-0.969230769230768,-0.953846153846152,
-0.938461538461537,-0.923076923076922,-0.907692307692306,-0.892307692307691,
-0.876923076923076,-0.86153846153846,-0.846153846153845,-0.83076923076923,
-0.815384615384614,-0.799999999999999,-0.784615384615384,-0.769230769230768,
-0.753846153846153,-0.738461538461538,-0.723076923076922,-0.707692307692307,
-0.692307692307692,-0.676923076923076,-0.661538461538461,-0.646153846153846,
-0.63076923076923,-0.615384615384615,-0.6,-0.584615384615384,-0.569230769230769,
-0.553846153846154,-0.538461538461538,-0.523076923076923,-0.507692307692308,
-0.492307692307692,-0.476923076923077,-0.461538461538462,-0.446153846153846,
-0.430769230769231,-0.415384615384615,-0.4,-0.384615384615385,-0.369230769230769,
-0.353846153846154,-0.338461538461538,-0.323076923076923,-0.307692307692308,
-0.292307692307692,-0.276923076923077,-0.261538461538462,-0.246153846153846,
-0.230769230769231,-0.215384615384615,-0.2,-0.184615384615385,-0.169230769230769,
-0.153846153846154,-0.138461538461538,-0.123076923076923,-0.107692307692308,
-0.0923076923076923,-0.0769230769230769,-0.0615384615384615,-0.0461538461538462,
-0.0307692307692308,-0.0153846153846154,-0.00577184337451611),
 .UNSPECIFIED.)
CURVE()
GEOMETRIC_REPRESENTATION_ITEM()
RATIONAL_B_SPLINE_CURVE((1.,1.,1.,1.,1.,1.,1.,1.,1.,1.,1.,1.,1.,1.,1.,1.,
1.,1.,1.,1.,1.,1.,1.,1.,1.,1.,1.,1.,1.,1.,1.,1.,1.,1.,1.,1.,1.,1.,1.,1.,
1.,1.,1.,1.,1.,1.,1.,1.,1.,1.,1.,1.,1.,1.,1.,1.,1.,1.,1.,1.,1.,1.,1.,1.,
1.,1.,1.,1.,1.,1.))
REPRESENTATION_ITEM('')
);
#911=B_SPLINE_CURVE_WITH_KNOTS('',3,(#44768,#44769,#44770,#44771,#44772,
#44773),.UNSPECIFIED.,.F.,.F.,(4,2,4),(0.,1.,2.),.UNSPECIFIED.);
#912=B_SPLINE_CURVE_WITH_KNOTS('',3,(#44987,#44988,#44989,#44990,#44991,
#44992),.UNSPECIFIED.,.F.,.F.,(4,2,4),(0.,1.,2.),.UNSPECIFIED.);
#913=B_SPLINE_CURVE_WITH_KNOTS('',3,(#45070,#45071,#45072,#45073,#45074,
#45075),.UNSPECIFIED.,.F.,.F.,(4,2,4),(0.,1.,2.),.UNSPECIFIED.);
#914=B_SPLINE_CURVE_WITH_KNOTS('',3,(#45429,#45430,#45431,#45432,#45433,
#45434),.UNSPECIFIED.,.F.,.F.,(4,2,4),(0.,1.,2.),.UNSPECIFIED.);
#915=B_SPLINE_CURVE_WITH_KNOTS('',3,(#45512,#45513,#45514,#45515,#45516,
#45517),.UNSPECIFIED.,.F.,.F.,(4,2,4),(0.,1.,2.),.UNSPECIFIED.);
#916=B_SPLINE_CURVE_WITH_KNOTS('',3,(#45871,#45872,#45873,#45874,#45875,
#45876),.UNSPECIFIED.,.F.,.F.,(4,2,4),(0.,1.,2.),.UNSPECIFIED.);
#917=B_SPLINE_CURVE_WITH_KNOTS('',3,(#45954,#45955,#45956,#45957,#45958,
#45959),.UNSPECIFIED.,.F.,.F.,(4,2,4),(0.,1.,2.),.UNSPECIFIED.);
#918=B_SPLINE_CURVE_WITH_KNOTS('',3,(#46313,#46314,#46315,#46316,#46317,
#46318),.UNSPECIFIED.,.F.,.F.,(4,2,4),(0.,1.,2.),.UNSPECIFIED.);
#919=B_SPLINE_CURVE_WITH_KNOTS('',3,(#46396,#46397,#46398,#46399,#46400,
#46401),.UNSPECIFIED.,.F.,.F.,(4,2,4),(0.,1.,2.),.UNSPECIFIED.);
#920=B_SPLINE_CURVE_WITH_KNOTS('',3,(#46755,#46756,#46757,#46758,#46759,
#46760),.UNSPECIFIED.,.F.,.F.,(4,2,4),(0.,1.,2.),.UNSPECIFIED.);
#921=B_SPLINE_CURVE_WITH_KNOTS('',3,(#46838,#46839,#46840,#46841,#46842,
#46843),.UNSPECIFIED.,.F.,.F.,(4,2,4),(0.,1.,2.),.UNSPECIFIED.);
#922=B_SPLINE_CURVE_WITH_KNOTS('',3,(#47197,#47198,#47199,#47200,#47201,
#47202),.UNSPECIFIED.,.F.,.F.,(4,2,4),(0.,1.,2.),.UNSPECIFIED.);
#923=B_SPLINE_CURVE_WITH_KNOTS('',3,(#47280,#47281,#47282,#47283,#47284,
#47285),.UNSPECIFIED.,.F.,.F.,(4,2,4),(0.,1.,2.),.UNSPECIFIED.);
#924=B_SPLINE_CURVE_WITH_KNOTS('',3,(#47639,#47640,#47641,#47642,#47643,
#47644),.UNSPECIFIED.,.F.,.F.,(4,2,4),(0.,1.,2.),.UNSPECIFIED.);
#925=B_SPLINE_CURVE_WITH_KNOTS('',3,(#47722,#47723,#47724,#47725,#47726,
#47727),.UNSPECIFIED.,.F.,.F.,(4,2,4),(0.,1.,2.),.UNSPECIFIED.);
#926=B_SPLINE_CURVE_WITH_KNOTS('',3,(#48081,#48082,#48083,#48084,#48085,
#48086),.UNSPECIFIED.,.F.,.F.,(4,2,4),(0.,1.,2.),.UNSPECIFIED.);
#927=B_SPLINE_CURVE_WITH_KNOTS('',3,(#48164,#48165,#48166,#48167,#48168,
#48169),.UNSPECIFIED.,.F.,.F.,(4,2,4),(0.,1.,2.),.UNSPECIFIED.);
#928=B_SPLINE_CURVE_WITH_KNOTS('',3,(#48523,#48524,#48525,#48526,#48527,
#48528),.UNSPECIFIED.,.F.,.F.,(4,2,4),(0.,1.,2.),.UNSPECIFIED.);
#929=B_SPLINE_CURVE_WITH_KNOTS('',3,(#48606,#48607,#48608,#48609,#48610,
#48611),.UNSPECIFIED.,.F.,.F.,(4,2,4),(0.,1.,2.),.UNSPECIFIED.);
#930=B_SPLINE_CURVE_WITH_KNOTS('',3,(#48965,#48966,#48967,#48968,#48969,
#48970),.UNSPECIFIED.,.F.,.F.,(4,2,4),(0.,1.,2.),.UNSPECIFIED.);
#931=B_SPLINE_CURVE_WITH_KNOTS('',3,(#49048,#49049,#49050,#49051,#49052,
#49053),.UNSPECIFIED.,.F.,.F.,(4,2,4),(0.,1.,2.),.UNSPECIFIED.);
#932=B_SPLINE_CURVE_WITH_KNOTS('',3,(#49407,#49408,#49409,#49410,#49411,
#49412),.UNSPECIFIED.,.F.,.F.,(4,2,4),(0.,1.,2.),.UNSPECIFIED.);
#933=B_SPLINE_CURVE_WITH_KNOTS('',3,(#49490,#49491,#49492,#49493,#49494,
#49495),.UNSPECIFIED.,.F.,.F.,(4,2,4),(0.,1.,2.),.UNSPECIFIED.);
#934=B_SPLINE_CURVE_WITH_KNOTS('',3,(#49849,#49850,#49851,#49852,#49853,
#49854),.UNSPECIFIED.,.F.,.F.,(4,2,4),(0.,1.,2.),.UNSPECIFIED.);
#935=B_SPLINE_CURVE_WITH_KNOTS('',3,(#49932,#49933,#49934,#49935,#49936,
#49937),.UNSPECIFIED.,.F.,.F.,(4,2,4),(0.,1.,2.),.UNSPECIFIED.);
#936=B_SPLINE_CURVE_WITH_KNOTS('',3,(#50291,#50292,#50293,#50294,#50295,
#50296),.UNSPECIFIED.,.F.,.F.,(4,2,4),(0.,1.,2.),.UNSPECIFIED.);
#937=B_SPLINE_CURVE_WITH_KNOTS('',3,(#50374,#50375,#50376,#50377,#50378,
#50379),.UNSPECIFIED.,.F.,.F.,(4,2,4),(0.,1.,2.),.UNSPECIFIED.);
#938=B_SPLINE_CURVE_WITH_KNOTS('',3,(#50733,#50734,#50735,#50736,#50737,
#50738),.UNSPECIFIED.,.F.,.F.,(4,2,4),(0.,1.,2.),.UNSPECIFIED.);
#939=B_SPLINE_CURVE_WITH_KNOTS('',3,(#50816,#50817,#50818,#50819,#50820,
#50821),.UNSPECIFIED.,.F.,.F.,(4,2,4),(0.,1.,2.),.UNSPECIFIED.);
#940=B_SPLINE_CURVE_WITH_KNOTS('',3,(#51175,#51176,#51177,#51178,#51179,
#51180),.UNSPECIFIED.,.F.,.F.,(4,2,4),(0.,1.,2.),.UNSPECIFIED.);
#941=B_SPLINE_CURVE_WITH_KNOTS('',3,(#51258,#51259,#51260,#51261,#51262,
#51263),.UNSPECIFIED.,.F.,.F.,(4,2,4),(0.,1.,2.),.UNSPECIFIED.);
#942=B_SPLINE_CURVE_WITH_KNOTS('',3,(#51617,#51618,#51619,#51620,#51621,
#51622),.UNSPECIFIED.,.F.,.F.,(4,2,4),(0.,1.,2.),.UNSPECIFIED.);
#943=B_SPLINE_CURVE_WITH_KNOTS('',3,(#51700,#51701,#51702,#51703,#51704,
#51705),.UNSPECIFIED.,.F.,.F.,(4,2,4),(0.,1.,2.),.UNSPECIFIED.);
#944=B_SPLINE_CURVE_WITH_KNOTS('',3,(#52059,#52060,#52061,#52062,#52063,
#52064),.UNSPECIFIED.,.F.,.F.,(4,2,4),(0.,1.,2.),.UNSPECIFIED.);
#945=B_SPLINE_CURVE_WITH_KNOTS('',3,(#52142,#52143,#52144,#52145,#52146,
#52147),.UNSPECIFIED.,.F.,.F.,(4,2,4),(0.,1.,2.),.UNSPECIFIED.);
#946=B_SPLINE_CURVE_WITH_KNOTS('',3,(#52501,#52502,#52503,#52504,#52505,
#52506),.UNSPECIFIED.,.F.,.F.,(4,2,4),(0.,1.,2.),.UNSPECIFIED.);
#947=B_SPLINE_CURVE_WITH_KNOTS('',3,(#52584,#52585,#52586,#52587,#52588,
#52589),.UNSPECIFIED.,.F.,.F.,(4,2,4),(0.,1.,2.),.UNSPECIFIED.);
#948=B_SPLINE_CURVE_WITH_KNOTS('',3,(#52943,#52944,#52945,#52946,#52947,
#52948),.UNSPECIFIED.,.F.,.F.,(4,2,4),(0.,1.,2.),.UNSPECIFIED.);
#949=B_SPLINE_CURVE_WITH_KNOTS('',3,(#53026,#53027,#53028,#53029,#53030,
#53031),.UNSPECIFIED.,.F.,.F.,(4,2,4),(0.,1.,2.),.UNSPECIFIED.);
#950=B_SPLINE_CURVE_WITH_KNOTS('',3,(#53385,#53386,#53387,#53388,#53389,
#53390),.UNSPECIFIED.,.F.,.F.,(4,2,4),(0.,1.,2.),.UNSPECIFIED.);
#951=B_SPLINE_CURVE_WITH_KNOTS('',3,(#53468,#53469,#53470,#53471,#53472,
#53473),.UNSPECIFIED.,.F.,.F.,(4,2,4),(0.,1.,2.),.UNSPECIFIED.);
#952=B_SPLINE_CURVE_WITH_KNOTS('',3,(#53827,#53828,#53829,#53830,#53831,
#53832),.UNSPECIFIED.,.F.,.F.,(4,2,4),(0.,1.,2.),.UNSPECIFIED.);
#953=B_SPLINE_CURVE_WITH_KNOTS('',3,(#53910,#53911,#53912,#53913,#53914,
#53915),.UNSPECIFIED.,.F.,.F.,(4,2,4),(0.,1.,2.),.UNSPECIFIED.);
#954=B_SPLINE_CURVE_WITH_KNOTS('',3,(#54269,#54270,#54271,#54272,#54273,
#54274),.UNSPECIFIED.,.F.,.F.,(4,2,4),(0.,1.,2.),.UNSPECIFIED.);
#955=B_SPLINE_CURVE_WITH_KNOTS('',3,(#54352,#54353,#54354,#54355,#54356,
#54357),.UNSPECIFIED.,.F.,.F.,(4,2,4),(0.,1.,2.),.UNSPECIFIED.);
#956=B_SPLINE_CURVE_WITH_KNOTS('',3,(#54711,#54712,#54713,#54714,#54715,
#54716),.UNSPECIFIED.,.F.,.F.,(4,2,4),(0.,1.,2.),.UNSPECIFIED.);
#957=B_SPLINE_CURVE_WITH_KNOTS('',3,(#54794,#54795,#54796,#54797,#54798,
#54799),.UNSPECIFIED.,.F.,.F.,(4,2,4),(0.,1.,2.),.UNSPECIFIED.);
#958=B_SPLINE_CURVE_WITH_KNOTS('',3,(#55153,#55154,#55155,#55156,#55157,
#55158),.UNSPECIFIED.,.F.,.F.,(4,2,4),(0.,1.,2.),.UNSPECIFIED.);
#959=B_SPLINE_CURVE_WITH_KNOTS('',3,(#55236,#55237,#55238,#55239,#55240,
#55241),.UNSPECIFIED.,.F.,.F.,(4,2,4),(0.,1.,2.),.UNSPECIFIED.);
#960=B_SPLINE_CURVE_WITH_KNOTS('',3,(#55595,#55596,#55597,#55598,#55599,
#55600),.UNSPECIFIED.,.F.,.F.,(4,2,4),(0.,1.,2.),.UNSPECIFIED.);
#961=B_SPLINE_CURVE_WITH_KNOTS('',3,(#55678,#55679,#55680,#55681,#55682,
#55683),.UNSPECIFIED.,.F.,.F.,(4,2,4),(0.,1.,2.),.UNSPECIFIED.);
#962=B_SPLINE_CURVE_WITH_KNOTS('',3,(#56037,#56038,#56039,#56040,#56041,
#56042),.UNSPECIFIED.,.F.,.F.,(4,2,4),(0.,1.,2.),.UNSPECIFIED.);
#963=B_SPLINE_CURVE_WITH_KNOTS('',3,(#56120,#56121,#56122,#56123,#56124,
#56125),.UNSPECIFIED.,.F.,.F.,(4,2,4),(0.,1.,2.),.UNSPECIFIED.);
#964=B_SPLINE_CURVE_WITH_KNOTS('',3,(#56479,#56480,#56481,#56482,#56483,
#56484),.UNSPECIFIED.,.F.,.F.,(4,2,4),(0.,1.,2.),.UNSPECIFIED.);
#965=B_SPLINE_CURVE_WITH_KNOTS('',3,(#56562,#56563,#56564,#56565,#56566,
#56567),.UNSPECIFIED.,.F.,.F.,(4,2,4),(0.,1.,2.),.UNSPECIFIED.);
#966=B_SPLINE_CURVE_WITH_KNOTS('',3,(#56921,#56922,#56923,#56924,#56925,
#56926),.UNSPECIFIED.,.F.,.F.,(4,2,4),(0.,1.,2.),.UNSPECIFIED.);
#967=B_SPLINE_CURVE_WITH_KNOTS('',3,(#57004,#57005,#57006,#57007,#57008,
#57009),.UNSPECIFIED.,.F.,.F.,(4,2,4),(0.,1.,2.),.UNSPECIFIED.);
#968=B_SPLINE_CURVE_WITH_KNOTS('',3,(#57363,#57364,#57365,#57366,#57367,
#57368),.UNSPECIFIED.,.F.,.F.,(4,2,4),(0.,1.,2.),.UNSPECIFIED.);
#969=B_SPLINE_CURVE_WITH_KNOTS('',3,(#57446,#57447,#57448,#57449,#57450,
#57451),.UNSPECIFIED.,.F.,.F.,(4,2,4),(0.,1.,2.),.UNSPECIFIED.);
#970=B_SPLINE_CURVE_WITH_KNOTS('',3,(#57805,#57806,#57807,#57808,#57809,
#57810),.UNSPECIFIED.,.F.,.F.,(4,2,4),(0.,1.,2.),.UNSPECIFIED.);
#971=B_SPLINE_CURVE_WITH_KNOTS('',3,(#57888,#57889,#57890,#57891,#57892,
#57893),.UNSPECIFIED.,.F.,.F.,(4,2,4),(0.,1.,2.),.UNSPECIFIED.);
#972=B_SPLINE_CURVE_WITH_KNOTS('',3,(#58247,#58248,#58249,#58250,#58251,
#58252),.UNSPECIFIED.,.F.,.F.,(4,2,4),(0.,1.,2.),.UNSPECIFIED.);
#973=B_SPLINE_CURVE_WITH_KNOTS('',3,(#58330,#58331,#58332,#58333,#58334,
#58335),.UNSPECIFIED.,.F.,.F.,(4,2,4),(0.,1.,2.),.UNSPECIFIED.);
#974=B_SPLINE_CURVE_WITH_KNOTS('',3,(#58689,#58690,#58691,#58692,#58693,
#58694),.UNSPECIFIED.,.F.,.F.,(4,2,4),(0.,1.,2.),.UNSPECIFIED.);
#975=B_SPLINE_CURVE_WITH_KNOTS('',3,(#58772,#58773,#58774,#58775,#58776,
#58777),.UNSPECIFIED.,.F.,.F.,(4,2,4),(0.,1.,2.),.UNSPECIFIED.);
#976=B_SPLINE_CURVE_WITH_KNOTS('',3,(#59131,#59132,#59133,#59134,#59135,
#59136),.UNSPECIFIED.,.F.,.F.,(4,2,4),(0.,1.,2.),.UNSPECIFIED.);
#977=B_SPLINE_CURVE_WITH_KNOTS('',3,(#59214,#59215,#59216,#59217,#59218,
#59219),.UNSPECIFIED.,.F.,.F.,(4,2,4),(0.,1.,2.),.UNSPECIFIED.);
#978=B_SPLINE_CURVE_WITH_KNOTS('',3,(#59573,#59574,#59575,#59576,#59577,
#59578),.UNSPECIFIED.,.F.,.F.,(4,2,4),(0.,1.,2.),.UNSPECIFIED.);
#979=B_SPLINE_CURVE_WITH_KNOTS('',3,(#59656,#59657,#59658,#59659,#59660,
#59661),.UNSPECIFIED.,.F.,.F.,(4,2,4),(0.,1.,2.),.UNSPECIFIED.);
#980=B_SPLINE_CURVE_WITH_KNOTS('',3,(#60015,#60016,#60017,#60018,#60019,
#60020),.UNSPECIFIED.,.F.,.F.,(4,2,4),(0.,1.,2.),.UNSPECIFIED.);
#981=B_SPLINE_CURVE_WITH_KNOTS('',3,(#60098,#60099,#60100,#60101,#60102,
#60103),.UNSPECIFIED.,.F.,.F.,(4,2,4),(0.,1.,2.),.UNSPECIFIED.);
#982=B_SPLINE_CURVE_WITH_KNOTS('',3,(#60457,#60458,#60459,#60460,#60461,
#60462),.UNSPECIFIED.,.F.,.F.,(4,2,4),(0.,1.,2.),.UNSPECIFIED.);
#983=B_SPLINE_CURVE_WITH_KNOTS('',3,(#60540,#60541,#60542,#60543,#60544,
#60545),.UNSPECIFIED.,.F.,.F.,(4,2,4),(0.,1.,2.),.UNSPECIFIED.);
#984=B_SPLINE_CURVE_WITH_KNOTS('',3,(#60899,#60900,#60901,#60902,#60903,
#60904),.UNSPECIFIED.,.F.,.F.,(4,2,4),(0.,1.,2.),.UNSPECIFIED.);
#985=B_SPLINE_CURVE_WITH_KNOTS('',3,(#60982,#60983,#60984,#60985,#60986,
#60987),.UNSPECIFIED.,.F.,.F.,(4,2,4),(0.,1.,2.),.UNSPECIFIED.);
#986=B_SPLINE_CURVE_WITH_KNOTS('',3,(#61341,#61342,#61343,#61344,#61345,
#61346),.UNSPECIFIED.,.F.,.F.,(4,2,4),(0.,1.,2.),.UNSPECIFIED.);
#987=B_SPLINE_CURVE_WITH_KNOTS('',3,(#61424,#61425,#61426,#61427,#61428,
#61429),.UNSPECIFIED.,.F.,.F.,(4,2,4),(0.,1.,2.),.UNSPECIFIED.);
#988=B_SPLINE_CURVE_WITH_KNOTS('',3,(#61787,#61788,#61789,#61790,#61791,
#61792),.UNSPECIFIED.,.F.,.F.,(4,2,4),(0.,1.,2.),.UNSPECIFIED.);
#989=B_SPLINE_CURVE_WITH_KNOTS('',3,(#61866,#61867,#61868,#61869,#61870,
#61871),.UNSPECIFIED.,.F.,.F.,(4,2,4),(0.,1.,2.),.UNSPECIFIED.);
#990=B_SPLINE_CURVE_WITH_KNOTS('',3,(#62013,#62014,#62015,#62016,#62017,
#62018),.UNSPECIFIED.,.F.,.F.,(4,2,4),(0.,1.,2.),.UNSPECIFIED.);
#1120=SHAPE_REPRESENTATION_RELATIONSHIP('SRR','None',#63098,#1184);
#1184=ADVANCED_BREP_SHAPE_REPRESENTATION('',(#1338),#62752);
#1263=STYLED_ITEM('',(#63455),#1338);
#1338=MANIFOLD_SOLID_BREP('Body1',#16447);
#1626=FACE_BOUND('',#4072,.T.);
#1627=FACE_BOUND('',#4076,.T.);
#1628=FACE_BOUND('',#4237,.T.);
#2045=PLANE('',#18483);
#2046=PLANE('',#18484);
#2047=PLANE('',#18485);
#2048=PLANE('',#18486);
#2049=PLANE('',#18533);
#2050=PLANE('',#18534);
#2051=PLANE('',#18537);
#2052=PLANE('',#18540);
#2053=PLANE('',#18543);
#2054=PLANE('',#18546);
#2055=PLANE('',#18549);
#2056=PLANE('',#18552);
#2057=PLANE('',#18555);
#2058=PLANE('',#18558);
#2059=PLANE('',#18561);
#2060=PLANE('',#18564);
#2061=PLANE('',#18567);
#2062=PLANE('',#18570);
#2063=PLANE('',#18573);
#2064=PLANE('',#18576);
#2065=PLANE('',#18579);
#2066=PLANE('',#18582);
#2067=PLANE('',#18585);
#2068=PLANE('',#18588);
#2069=PLANE('',#18591);
#2070=PLANE('',#18594);
#2071=PLANE('',#18597);
#2072=PLANE('',#18600);
#2073=PLANE('',#18603);
#2074=PLANE('',#18606);
#2075=PLANE('',#18609);
#2076=PLANE('',#18612);
#2077=PLANE('',#18615);
#2078=PLANE('',#18618);
#2079=PLANE('',#18621);
#2080=PLANE('',#18624);
#2081=PLANE('',#18627);
#2082=PLANE('',#18630);
#2083=PLANE('',#18633);
#2084=PLANE('',#18636);
#2085=PLANE('',#18639);
#2086=PLANE('',#18642);
#2087=PLANE('',#18645);
#2088=PLANE('',#18648);
#2089=PLANE('',#18651);
#2090=PLANE('',#18652);
#2848=FACE_OUTER_BOUND('',#4068,.T.);
#2849=FACE_OUTER_BOUND('',#4069,.T.);
#2850=FACE_OUTER_BOUND('',#4070,.T.);
#2851=FACE_OUTER_BOUND('',#4071,.T.);
#2852=FACE_OUTER_BOUND('',#4073,.T.);
#2853=FACE_OUTER_BOUND('',#4074,.T.);
#2854=FACE_OUTER_BOUND('',#4075,.T.);
#2855=FACE_OUTER_BOUND('',#4077,.T.);
#2856=FACE_OUTER_BOUND('',#4078,.T.);
#2857=FACE_OUTER_BOUND('',#4079,.T.);
#2858=FACE_OUTER_BOUND('',#4080,.T.);
#2859=FACE_OUTER_BOUND('',#4081,.T.);
#2860=FACE_OUTER_BOUND('',#4082,.T.);
#2861=FACE_OUTER_BOUND('',#4083,.T.);
#2862=FACE_OUTER_BOUND('',#4084,.T.);
#2863=FACE_OUTER_BOUND('',#4085,.T.);
#2864=FACE_OUTER_BOUND('',#4086,.T.);
#2865=FACE_OUTER_BOUND('',#4087,.T.);
#2866=FACE_OUTER_BOUND('',#4088,.T.);
#2867=FACE_OUTER_BOUND('',#4089,.T.);
#2868=FACE_OUTER_BOUND('',#4090,.T.);
#2869=FACE_OUTER_BOUND('',#4091,.T.);
#2870=FACE_OUTER_BOUND('',#4092,.T.);
#2871=FACE_OUTER_BOUND('',#4093,.T.);
#2872=FACE_OUTER_BOUND('',#4094,.T.);
#2873=FACE_OUTER_BOUND('',#4095,.T.);
#2874=FACE_OUTER_BOUND('',#4096,.T.);
#2875=FACE_OUTER_BOUND('',#4097,.T.);
#2876=FACE_OUTER_BOUND('',#4098,.T.);
#2877=FACE_OUTER_BOUND('',#4099,.T.);
#2878=FACE_OUTER_BOUND('',#4100,.T.);
#2879=FACE_OUTER_BOUND('',#4101,.T.);
#2880=FACE_OUTER_BOUND('',#4102,.T.);
#2881=FACE_OUTER_BOUND('',#4103,.T.);
#2882=FACE_OUTER_BOUND('',#4104,.T.);
#2883=FACE_OUTER_BOUND('',#4105,.T.);
#2884=FACE_OUTER_BOUND('',#4106,.T.);
#2885=FACE_OUTER_BOUND('',#4107,.T.);
#2886=FACE_OUTER_BOUND('',#4108,.T.);
#2887=FACE_OUTER_BOUND('',#4109,.T.);
#2888=FACE_OUTER_BOUND('',#4110,.T.);
#2889=FACE_OUTER_BOUND('',#4111,.T.);
#2890=FACE_OUTER_BOUND('',#4112,.T.);
#2891=FACE_OUTER_BOUND('',#4113,.T.);
#2892=FACE_OUTER_BOUND('',#4114,.T.);
#2893=FACE_OUTER_BOUND('',#4115,.T.);
#2894=FACE_OUTER_BOUND('',#4116,.T.);
#2895=FACE_OUTER_BOUND('',#4117,.T.);
#2896=FACE_OUTER_BOUND('',#4118,.T.);
#2897=FACE_OUTER_BOUND('',#4119,.T.);
#2898=FACE_OUTER_BOUND('',#4120,.T.);
#2899=FACE_OUTER_BOUND('',#4121,.T.);
#2900=FACE_OUTER_BOUND('',#4122,.T.);
#2901=FACE_OUTER_BOUND('',#4123,.T.);
#2902=FACE_OUTER_BOUND('',#4124,.T.);
#2903=FACE_OUTER_BOUND('',#4125,.T.);
#2904=FACE_OUTER_BOUND('',#4126,.T.);
#2905=FACE_OUTER_BOUND('',#4127,.T.);
#2906=FACE_OUTER_BOUND('',#4128,.T.);
#2907=FACE_OUTER_BOUND('',#4129,.T.);
#2908=FACE_OUTER_BOUND('',#4130,.T.);
#2909=FACE_OUTER_BOUND('',#4131,.T.);
#2910=FACE_OUTER_BOUND('',#4132,.T.);
#2911=FACE_OUTER_BOUND('',#4133,.T.);
#2912=FACE_OUTER_BOUND('',#4134,.T.);
#2913=FACE_OUTER_BOUND('',#4135,.T.);
#2914=FACE_OUTER_BOUND('',#4136,.T.);
#2915=FACE_OUTER_BOUND('',#4137,.T.);
#2916=FACE_OUTER_BOUND('',#4138,.T.);
#2917=FACE_OUTER_BOUND('',#4139,.T.);
#2918=FACE_OUTER_BOUND('',#4140,.T.);
#2919=FACE_OUTER_BOUND('',#4141,.T.);
#2920=FACE_OUTER_BOUND('',#4142,.T.);
#2921=FACE_OUTER_BOUND('',#4143,.T.);
#2922=FACE_OUTER_BOUND('',#4144,.T.);
#2923=FACE_OUTER_BOUND('',#4145,.T.);
#2924=FACE_OUTER_BOUND('',#4146,.T.);
#2925=FACE_OUTER_BOUND('',#4147,.T.);
#2926=FACE_OUTER_BOUND('',#4148,.T.);
#2927=FACE_OUTER_BOUND('',#4149,.T.);
#2928=FACE_OUTER_BOUND('',#4150,.T.);
#2929=FACE_OUTER_BOUND('',#4151,.T.);
#2930=FACE_OUTER_BOUND('',#4152,.T.);
#2931=FACE_OUTER_BOUND('',#4153,.T.);
#2932=FACE_OUTER_BOUND('',#4154,.T.);
#2933=FACE_OUTER_BOUND('',#4155,.T.);
#2934=FACE_OUTER_BOUND('',#4156,.T.);
#2935=FACE_OUTER_BOUND('',#4157,.T.);
#2936=FACE_OUTER_BOUND('',#4158,.T.);
#2937=FACE_OUTER_BOUND('',#4159,.T.);
#2938=FACE_OUTER_BOUND('',#4160,.T.);
#2939=FACE_OUTER_BOUND('',#4161,.T.);
#2940=FACE_OUTER_BOUND('',#4162,.T.);
#2941=FACE_OUTER_BOUND('',#4163,.T.);
#2942=FACE_OUTER_BOUND('',#4164,.T.);
#2943=FACE_OUTER_BOUND('',#4165,.T.);
#2944=FACE_OUTER_BOUND('',#4166,.T.);
#2945=FACE_OUTER_BOUND('',#4167,.T.);
#2946=FACE_OUTER_BOUND('',#4168,.T.);
#2947=FACE_OUTER_BOUND('',#4169,.T.);
#2948=FACE_OUTER_BOUND('',#4170,.T.);
#2949=FACE_OUTER_BOUND('',#4171,.T.);
#2950=FACE_OUTER_BOUND('',#4172,.T.);
#2951=FACE_OUTER_BOUND('',#4173,.T.);
#2952=FACE_OUTER_BOUND('',#4174,.T.);
#2953=FACE_OUTER_BOUND('',#4175,.T.);
#2954=FACE_OUTER_BOUND('',#4176,.T.);
#2955=FACE_OUTER_BOUND('',#4177,.T.);
#2956=FACE_OUTER_BOUND('',#4178,.T.);
#2957=FACE_OUTER_BOUND('',#4179,.T.);
#2958=FACE_OUTER_BOUND('',#4180,.T.);
#2959=FACE_OUTER_BOUND('',#4181,.T.);
#2960=FACE_OUTER_BOUND('',#4182,.T.);
#2961=FACE_OUTER_BOUND('',#4183,.T.);
#2962=FACE_OUTER_BOUND('',#4184,.T.);
#2963=FACE_OUTER_BOUND('',#4185,.T.);
#2964=FACE_OUTER_BOUND('',#4186,.T.);
#2965=FACE_OUTER_BOUND('',#4187,.T.);
#2966=FACE_OUTER_BOUND('',#4188,.T.);
#2967=FACE_OUTER_BOUND('',#4189,.T.);
#2968=FACE_OUTER_BOUND('',#4190,.T.);
#2969=FACE_OUTER_BOUND('',#4191,.T.);
#2970=FACE_OUTER_BOUND('',#4192,.T.);
#2971=FACE_OUTER_BOUND('',#4193,.T.);
#2972=FACE_OUTER_BOUND('',#4194,.T.);
#2973=FACE_OUTER_BOUND('',#4195,.T.);
#2974=FACE_OUTER_BOUND('',#4196,.T.);
#2975=FACE_OUTER_BOUND('',#4197,.T.);
#2976=FACE_OUTER_BOUND('',#4198,.T.);
#2977=FACE_OUTER_BOUND('',#4199,.T.);
#2978=FACE_OUTER_BOUND('',#4200,.T.);
#2979=FACE_OUTER_BOUND('',#4201,.T.);
#2980=FACE_OUTER_BOUND('',#4202,.T.);
#2981=FACE_OUTER_BOUND('',#4203,.T.);
#2982=FACE_OUTER_BOUND('',#4204,.T.);
#2983=FACE_OUTER_BOUND('',#4205,.T.);
#2984=FACE_OUTER_BOUND('',#4206,.T.);
#2985=FACE_OUTER_BOUND('',#4207,.T.);
#2986=FACE_OUTER_BOUND('',#4208,.T.);
#2987=FACE_OUTER_BOUND('',#4209,.T.);
#2988=FACE_OUTER_BOUND('',#4210,.T.);
#2989=FACE_OUTER_BOUND('',#4211,.T.);
#2990=FACE_OUTER_BOUND('',#4212,.T.);
#2991=FACE_OUTER_BOUND('',#4213,.T.);
#2992=FACE_OUTER_BOUND('',#4214,.T.);
#2993=FACE_OUTER_BOUND('',#4215,.T.);
#2994=FACE_OUTER_BOUND('',#4216,.T.);
#2995=FACE_OUTER_BOUND('',#4217,.T.);
#2996=FACE_OUTER_BOUND('',#4218,.T.);
#2997=FACE_OUTER_BOUND('',#4219,.T.);
#2998=FACE_OUTER_BOUND('',#4220,.T.);
#2999=FACE_OUTER_BOUND('',#4221,.T.);
#3000=FACE_OUTER_BOUND('',#4222,.T.);
#3001=FACE_OUTER_BOUND('',#4223,.T.);
#3002=FACE_OUTER_BOUND('',#4224,.T.);
#3003=FACE_OUTER_BOUND('',#4225,.T.);
#3004=FACE_OUTER_BOUND('',#4226,.T.);
#3005=FACE_OUTER_BOUND('',#4227,.T.);
#3006=FACE_OUTER_BOUND('',#4228,.T.);
#3007=FACE_OUTER_BOUND('',#4229,.T.);
#3008=FACE_OUTER_BOUND('',#4230,.T.);
#3009=FACE_OUTER_BOUND('',#4231,.T.);
#3010=FACE_OUTER_BOUND('',#4232,.T.);
#3011=FACE_OUTER_BOUND('',#4233,.T.);
#3012=FACE_OUTER_BOUND('',#4234,.T.);
#3013=FACE_OUTER_BOUND('',#4235,.T.);
#3014=FACE_OUTER_BOUND('',#4236,.T.);
#3015=FACE_OUTER_BOUND('',#4238,.T.);
#4068=EDGE_LOOP('',(#14003,#14004,#14005,#14006));
#4069=EDGE_LOOP('',(#14007,#14008,#14009,#14010));
#4070=EDGE_LOOP('',(#14011,#14012,#14013,#14014));
#4071=EDGE_LOOP('',(#14015,#14016,#14017,#14018,#14019,#14020,#14021,#14022,
#14023,#14024,#14025,#14026,#14027,#14028,#14029,#14030,#14031,#14032,#14033,
#14034,#14035,#14036,#14037,#14038,#14039,#14040,#14041,#14042,#14043,#14044,
#14045,#14046,#14047,#14048,#14049,#14050,#14051,#14052,#14053,#14054,#14055,
#14056,#14057,#14058,#14059,#14060,#14061,#14062,#14063,#14064,#14065,#14066,
#14067,#14068,#14069,#14070,#14071,#14072,#14073,#14074,#14075,#14076,#14077,
#14078,#14079,#14080,#14081,#14082,#14083,#14084,#14085,#14086,#14087,#14088,
#14089,#14090,#14091,#14092,#14093,#14094,#14095,#14096,#14097,#14098,#14099,
#14100,#14101,#14102,#14103,#14104,#14105,#14106,#14107,#14108,#14109,#14110,
#14111,#14112,#14113,#14114,#14115,#14116,#14117,#14118,#14119,#14120,#14121,
#14122,#14123,#14124,#14125,#14126,#14127,#14128,#14129,#14130,#14131,#14132,
#14133,#14134,#14135,#14136,#14137,#14138,#14139,#14140,#14141,#14142,#14143,
#14144,#14145,#14146,#14147,#14148,#14149,#14150,#14151,#14152,#14153,#14154,
#14155,#14156,#14157,#14158,#14159,#14160,#14161,#14162,#14163,#14164,#14165,
#14166,#14167,#14168,#14169,#14170,#14171,#14172,#14173,#14174));
#4072=EDGE_LOOP('',(#14175,#14176,#14177,#14178));
#4073=EDGE_LOOP('',(#14179,#14180,#14181,#14182));
#4074=EDGE_LOOP('',(#14183,#14184,#14185,#14186));
#4075=EDGE_LOOP('',(#14187));
#4076=EDGE_LOOP('',(#14188,#14189,#14190,#14191));
#4077=EDGE_LOOP('',(#14192,#14193,#14194,#14195));
#4078=EDGE_LOOP('',(#14196,#14197,#14198,#14199));
#4079=EDGE_LOOP('',(#14200,#14201,#14202,#14203));
#4080=EDGE_LOOP('',(#14204,#14205,#14206,#14207));
#4081=EDGE_LOOP('',(#14208,#14209,#14210,#14211));
#4082=EDGE_LOOP('',(#14212,#14213,#14214,#14215));
#4083=EDGE_LOOP('',(#14216,#14217,#14218,#14219));
#4084=EDGE_LOOP('',(#14220,#14221,#14222,#14223));
#4085=EDGE_LOOP('',(#14224,#14225,#14226,#14227));
#4086=EDGE_LOOP('',(#14228,#14229,#14230,#14231));
#4087=EDGE_LOOP('',(#14232,#14233,#14234,#14235));
#4088=EDGE_LOOP('',(#14236,#14237,#14238,#14239));
#4089=EDGE_LOOP('',(#14240,#14241,#14242,#14243));
#4090=EDGE_LOOP('',(#14244,#14245,#14246,#14247));
#4091=EDGE_LOOP('',(#14248,#14249,#14250,#14251));
#4092=EDGE_LOOP('',(#14252,#14253,#14254,#14255));
#4093=EDGE_LOOP('',(#14256,#14257,#14258,#14259));
#4094=EDGE_LOOP('',(#14260,#14261,#14262,#14263));
#4095=EDGE_LOOP('',(#14264,#14265,#14266,#14267));
#4096=EDGE_LOOP('',(#14268,#14269,#14270,#14271));
#4097=EDGE_LOOP('',(#14272,#14273,#14274,#14275));
#4098=EDGE_LOOP('',(#14276,#14277,#14278,#14279));
#4099=EDGE_LOOP('',(#14280,#14281,#14282,#14283));
#4100=EDGE_LOOP('',(#14284,#14285,#14286,#14287));
#4101=EDGE_LOOP('',(#14288,#14289,#14290,#14291));
#4102=EDGE_LOOP('',(#14292,#14293,#14294,#14295));
#4103=EDGE_LOOP('',(#14296,#14297,#14298,#14299));
#4104=EDGE_LOOP('',(#14300,#14301,#14302,#14303));
#4105=EDGE_LOOP('',(#14304,#14305,#14306,#14307));
#4106=EDGE_LOOP('',(#14308,#14309,#14310,#14311));
#4107=EDGE_LOOP('',(#14312,#14313,#14314,#14315));
#4108=EDGE_LOOP('',(#14316,#14317,#14318,#14319));
#4109=EDGE_LOOP('',(#14320,#14321,#14322,#14323));
#4110=EDGE_LOOP('',(#14324,#14325,#14326,#14327));
#4111=EDGE_LOOP('',(#14328,#14329,#14330,#14331));
#4112=EDGE_LOOP('',(#14332,#14333,#14334,#14335));
#4113=EDGE_LOOP('',(#14336,#14337,#14338,#14339));
#4114=EDGE_LOOP('',(#14340,#14341,#14342,#14343));
#4115=EDGE_LOOP('',(#14344,#14345,#14346,#14347));
#4116=EDGE_LOOP('',(#14348,#14349,#14350,#14351));
#4117=EDGE_LOOP('',(#14352,#14353,#14354,#14355));
#4118=EDGE_LOOP('',(#14356,#14357,#14358,#14359));
#4119=EDGE_LOOP('',(#14360,#14361,#14362,#14363));
#4120=EDGE_LOOP('',(#14364,#14365,#14366,#14367));
#4121=EDGE_LOOP('',(#14368,#14369,#14370,#14371));
#4122=EDGE_LOOP('',(#14372,#14373,#14374,#14375));
#4123=EDGE_LOOP('',(#14376,#14377,#14378,#14379));
#4124=EDGE_LOOP('',(#14380,#14381,#14382,#14383));
#4125=EDGE_LOOP('',(#14384,#14385,#14386,#14387));
#4126=EDGE_LOOP('',(#14388,#14389,#14390,#14391));
#4127=EDGE_LOOP('',(#14392,#14393,#14394,#14395));
#4128=EDGE_LOOP('',(#14396,#14397,#14398,#14399));
#4129=EDGE_LOOP('',(#14400,#14401,#14402,#14403));
#4130=EDGE_LOOP('',(#14404,#14405,#14406,#14407));
#4131=EDGE_LOOP('',(#14408,#14409,#14410,#14411));
#4132=EDGE_LOOP('',(#14412,#14413,#14414,#14415));
#4133=EDGE_LOOP('',(#14416,#14417,#14418,#14419));
#4134=EDGE_LOOP('',(#14420,#14421,#14422,#14423));
#4135=EDGE_LOOP('',(#14424,#14425,#14426,#14427));
#4136=EDGE_LOOP('',(#14428,#14429,#14430,#14431));
#4137=EDGE_LOOP('',(#14432,#14433,#14434,#14435));
#4138=EDGE_LOOP('',(#14436,#14437,#14438,#14439));
#4139=EDGE_LOOP('',(#14440,#14441,#14442,#14443));
#4140=EDGE_LOOP('',(#14444,#14445,#14446,#14447));
#4141=EDGE_LOOP('',(#14448,#14449,#14450,#14451));
#4142=EDGE_LOOP('',(#14452,#14453,#14454,#14455));
#4143=EDGE_LOOP('',(#14456,#14457,#14458,#14459));
#4144=EDGE_LOOP('',(#14460,#14461,#14462,#14463));
#4145=EDGE_LOOP('',(#14464,#14465,#14466,#14467));
#4146=EDGE_LOOP('',(#14468,#14469,#14470,#14471));
#4147=EDGE_LOOP('',(#14472,#14473,#14474,#14475));
#4148=EDGE_LOOP('',(#14476,#14477,#14478,#14479));
#4149=EDGE_LOOP('',(#14480,#14481,#14482,#14483));
#4150=EDGE_LOOP('',(#14484,#14485,#14486,#14487));
#4151=EDGE_LOOP('',(#14488,#14489,#14490,#14491));
#4152=EDGE_LOOP('',(#14492,#14493,#14494,#14495));
#4153=EDGE_LOOP('',(#14496,#14497,#14498,#14499));
#4154=EDGE_LOOP('',(#14500,#14501,#14502,#14503));
#4155=EDGE_LOOP('',(#14504,#14505,#14506,#14507));
#4156=EDGE_LOOP('',(#14508,#14509,#14510,#14511));
#4157=EDGE_LOOP('',(#14512,#14513,#14514,#14515));
#4158=EDGE_LOOP('',(#14516,#14517,#14518,#14519));
#4159=EDGE_LOOP('',(#14520,#14521,#14522,#14523));
#4160=EDGE_LOOP('',(#14524,#14525,#14526,#14527));
#4161=EDGE_LOOP('',(#14528,#14529,#14530,#14531));
#4162=EDGE_LOOP('',(#14532,#14533,#14534,#14535));
#4163=EDGE_LOOP('',(#14536,#14537,#14538,#14539));
#4164=EDGE_LOOP('',(#14540,#14541,#14542,#14543));
#4165=EDGE_LOOP('',(#14544,#14545,#14546,#14547));
#4166=EDGE_LOOP('',(#14548,#14549,#14550,#14551));
#4167=EDGE_LOOP('',(#14552,#14553,#14554,#14555));
#4168=EDGE_LOOP('',(#14556,#14557,#14558,#14559));
#4169=EDGE_LOOP('',(#14560,#14561,#14562,#14563));
#4170=EDGE_LOOP('',(#14564,#14565,#14566,#14567));
#4171=EDGE_LOOP('',(#14568,#14569,#14570,#14571));
#4172=EDGE_LOOP('',(#14572,#14573,#14574,#14575));
#4173=EDGE_LOOP('',(#14576,#14577,#14578,#14579));
#4174=EDGE_LOOP('',(#14580,#14581,#14582,#14583));
#4175=EDGE_LOOP('',(#14584,#14585,#14586,#14587));
#4176=EDGE_LOOP('',(#14588,#14589,#14590,#14591));
#4177=EDGE_LOOP('',(#14592,#14593,#14594,#14595));
#4178=EDGE_LOOP('',(#14596,#14597,#14598,#14599));
#4179=EDGE_LOOP('',(#14600,#14601,#14602,#14603));
#4180=EDGE_LOOP('',(#14604,#14605,#14606,#14607));
#4181=EDGE_LOOP('',(#14608,#14609,#14610,#14611));
#4182=EDGE_LOOP('',(#14612,#14613,#14614,#14615));
#4183=EDGE_LOOP('',(#14616,#14617,#14618,#14619));
#4184=EDGE_LOOP('',(#14620,#14621,#14622,#14623));
#4185=EDGE_LOOP('',(#14624,#14625,#14626,#14627));
#4186=EDGE_LOOP('',(#14628,#14629,#14630,#14631));
#4187=EDGE_LOOP('',(#14632,#14633,#14634,#14635));
#4188=EDGE_LOOP('',(#14636,#14637,#14638,#14639));
#4189=EDGE_LOOP('',(#14640,#14641,#14642,#14643));
#4190=EDGE_LOOP('',(#14644,#14645,#14646,#14647));
#4191=EDGE_LOOP('',(#14648,#14649,#14650,#14651));
#4192=EDGE_LOOP('',(#14652,#14653,#14654,#14655));
#4193=EDGE_LOOP('',(#14656,#14657,#14658,#14659));
#4194=EDGE_LOOP('',(#14660,#14661,#14662,#14663));
#4195=EDGE_LOOP('',(#14664,#14665,#14666,#14667));
#4196=EDGE_LOOP('',(#14668,#14669,#14670,#14671));
#4197=EDGE_LOOP('',(#14672,#14673,#14674,#14675));
#4198=EDGE_LOOP('',(#14676,#14677,#14678,#14679));
#4199=EDGE_LOOP('',(#14680,#14681,#14682,#14683));
#4200=EDGE_LOOP('',(#14684,#14685,#14686,#14687));
#4201=EDGE_LOOP('',(#14688,#14689,#14690,#14691));
#4202=EDGE_LOOP('',(#14692,#14693,#14694,#14695));
#4203=EDGE_LOOP('',(#14696,#14697,#14698,#14699));
#4204=EDGE_LOOP('',(#14700,#14701,#14702,#14703));
#4205=EDGE_LOOP('',(#14704,#14705,#14706,#14707));
#4206=EDGE_LOOP('',(#14708,#14709,#14710,#14711));
#4207=EDGE_LOOP('',(#14712,#14713,#14714,#14715));
#4208=EDGE_LOOP('',(#14716,#14717,#14718,#14719));
#4209=EDGE_LOOP('',(#14720,#14721,#14722,#14723));
#4210=EDGE_LOOP('',(#14724,#14725,#14726,#14727));
#4211=EDGE_LOOP('',(#14728,#14729,#14730,#14731));
#4212=EDGE_LOOP('',(#14732,#14733,#14734,#14735));
#4213=EDGE_LOOP('',(#14736,#14737,#14738,#14739));
#4214=EDGE_LOOP('',(#14740,#14741,#14742,#14743));
#4215=EDGE_LOOP('',(#14744,#14745,#14746,#14747));
#4216=EDGE_LOOP('',(#14748,#14749,#14750,#14751));
#4217=EDGE_LOOP('',(#14752,#14753,#14754,#14755));
#4218=EDGE_LOOP('',(#14756,#14757,#14758,#14759));
#4219=EDGE_LOOP('',(#14760,#14761,#14762,#14763));
#4220=EDGE_LOOP('',(#14764,#14765,#14766,#14767));
#4221=EDGE_LOOP('',(#14768,#14769,#14770,#14771));
#4222=EDGE_LOOP('',(#14772,#14773,#14774,#14775));
#4223=EDGE_LOOP('',(#14776,#14777,#14778,#14779));
#4224=EDGE_LOOP('',(#14780,#14781,#14782,#14783));
#4225=EDGE_LOOP('',(#14784,#14785,#14786,#14787));
#4226=EDGE_LOOP('',(#14788,#14789,#14790,#14791));
#4227=EDGE_LOOP('',(#14792,#14793,#14794,#14795));
#4228=EDGE_LOOP('',(#14796,#14797,#14798,#14799));
#4229=EDGE_LOOP('',(#14800,#14801,#14802,#14803));
#4230=EDGE_LOOP('',(#14804,#14805,#14806,#14807));
#4231=EDGE_LOOP('',(#14808,#14809,#14810,#14811));
#4232=EDGE_LOOP('',(#14812,#14813,#14814,#14815));
#4233=EDGE_LOOP('',(#14816,#14817,#14818,#14819));
#4234=EDGE_LOOP('',(#14820,#14821,#14822,#14823));
#4235=EDGE_LOOP('',(#14824,#14825,#14826,#14827));
#4236=EDGE_LOOP('',(#14828,#14829,#14830,#14831,#14832,#14833,#14834,#14835,
#14836,#14837,#14838,#14839,#14840,#14841,#14842,#14843,#14844,#14845,#14846,
#14847,#14848,#14849,#14850,#14851,#14852,#14853,#14854,#14855,#14856,#14857,
#14858,#14859,#14860,#14861,#14862,#14863,#14864,#14865,#14866,#14867,#14868,
#14869,#14870,#14871,#14872,#14873,#14874,#14875,#14876,#14877,#14878,#14879,
#14880,#14881,#14882,#14883,#14884,#14885,#14886,#14887,#14888,#14889,#14890,
#14891,#14892,#14893,#14894,#14895,#14896,#14897,#14898,#14899,#14900,#14901,
#14902,#14903,#14904,#14905,#14906,#14907,#14908,#14909,#14910,#14911,#14912,
#14913,#14914,#14915,#14916,#14917,#14918,#14919,#14920,#14921,#14922,#14923,
#14924,#14925,#14926,#14927,#14928,#14929,#14930,#14931,#14932,#14933,#14934,
#14935,#14936,#14937,#14938,#14939,#14940,#14941,#14942,#14943,#14944,#14945,
#14946,#14947,#14948,#14949,#14950,#14951,#14952,#14953,#14954,#14955,#14956,
#14957,#14958,#14959,#14960,#14961,#14962,#14963,#14964,#14965,#14966,#14967,
#14968,#14969,#14970,#14971,#14972,#14973,#14974,#14975,#14976,#14977,#14978,
#14979,#14980,#14981,#14982,#14983,#14984,#14985,#14986,#14987));
#4237=EDGE_LOOP('',(#14988));
#4238=EDGE_LOOP('',(#14989,#14990,#14991,#14992));
#5176=LINE('',#38758,#6308);
#5177=LINE('',#38760,#6309);
#5178=LINE('',#38762,#6310);
#5179=LINE('',#38763,#6311);
#5180=LINE('',#38766,#6312);
#5181=LINE('',#38768,#6313);
#5182=LINE('',#38769,#6314);
#5183=LINE('',#38772,#6315);
#5184=LINE('',#38774,#6316);
#5185=LINE('',#38775,#6317);
#5186=LINE('',#38852,#6318);
#5187=LINE('',#38998,#6319);
#5188=LINE('',#39144,#6320);
#5189=LINE('',#39290,#6321);
#5190=LINE('',#39436,#6322);
#5191=LINE('',#39582,#6323);
#5192=LINE('',#39728,#6324);
#5193=LINE('',#39874,#6325);
#5194=LINE('',#40020,#6326);
#5195=LINE('',#40166,#6327);
#5196=LINE('',#40312,#6328);
#5197=LINE('',#40458,#6329);
#5198=LINE('',#40604,#6330);
#5199=LINE('',#40750,#6331);
#5200=LINE('',#40896,#6332);
#5201=LINE('',#41042,#6333);
#5202=LINE('',#41188,#6334);
#5203=LINE('',#41334,#6335);
#5204=LINE('',#41480,#6336);
#5205=LINE('',#41626,#6337);
#5206=LINE('',#41772,#6338);
#5207=LINE('',#41918,#6339);
#5208=LINE('',#42064,#6340);
#5209=LINE('',#42210,#6341);
#5210=LINE('',#42356,#6342);
#5211=LINE('',#42502,#6343);
#5212=LINE('',#42648,#6344);
#5213=LINE('',#42794,#6345);
#5214=LINE('',#42940,#6346);
#5215=LINE('',#43086,#6347);
#5216=LINE('',#43232,#6348);
#5217=LINE('',#43378,#6349);
#5218=LINE('',#43524,#6350);
#5219=LINE('',#43670,#6351);
#5220=LINE('',#43816,#6352);
#5221=LINE('',#43962,#6353);
#5222=LINE('',#44108,#6354);
#5223=LINE('',#44254,#6355);
#5224=LINE('',#44400,#6356);
#5225=LINE('',#44546,#6357);
#5226=LINE('',#44624,#6358);
#5227=LINE('',#44845,#6359);
#5228=LINE('',#44994,#6360);
#5229=LINE('',#45066,#6361);
#5230=LINE('',#45287,#6362);
#5231=LINE('',#45436,#6363);
#5232=LINE('',#45508,#6364);
#5233=LINE('',#45729,#6365);
#5234=LINE('',#45878,#6366);
#5235=LINE('',#45950,#6367);
#5236=LINE('',#46171,#6368);
#5237=LINE('',#46320,#6369);
#5238=LINE('',#46392,#6370);
#5239=LINE('',#46613,#6371);
#5240=LINE('',#46762,#6372);
#5241=LINE('',#46834,#6373);
#5242=LINE('',#47055,#6374);
#5243=LINE('',#47204,#6375);
#5244=LINE('',#47276,#6376);
#5245=LINE('',#47497,#6377);
#5246=LINE('',#47646,#6378);
#5247=LINE('',#47718,#6379);
#5248=LINE('',#47939,#6380);
#5249=LINE('',#48088,#6381);
#5250=LINE('',#48160,#6382);
#5251=LINE('',#48381,#6383);
#5252=LINE('',#48530,#6384);
#5253=LINE('',#48602,#6385);
#5254=LINE('',#48823,#6386);
#5255=LINE('',#48972,#6387);
#5256=LINE('',#49044,#6388);
#5257=LINE('',#49265,#6389);
#5258=LINE('',#49414,#6390);
#5259=LINE('',#49486,#6391);
#5260=LINE('',#49707,#6392);
#5261=LINE('',#49856,#6393);
#5262=LINE('',#49928,#6394);
#5263=LINE('',#50149,#6395);
#5264=LINE('',#50298,#6396);
#5265=LINE('',#50370,#6397);
#5266=LINE('',#50591,#6398);
#5267=LINE('',#50740,#6399);
#5268=LINE('',#50812,#6400);
#5269=LINE('',#51033,#6401);
#5270=LINE('',#51182,#6402);
#5271=LINE('',#51254,#6403);
#5272=LINE('',#51475,#6404);
#5273=LINE('',#51624,#6405);
#5274=LINE('',#51696,#6406);
#5275=LINE('',#51917,#6407);
#5276=LINE('',#52066,#6408);
#5277=LINE('',#52138,#6409);
#5278=LINE('',#52359,#6410);
#5279=LINE('',#52508,#6411);
#5280=LINE('',#52580,#6412);
#5281=LINE('',#52801,#6413);
#5282=LINE('',#52950,#6414);
#5283=LINE('',#53022,#6415);
#5284=LINE('',#53243,#6416);
#5285=LINE('',#53392,#6417);
#5286=LINE('',#53464,#6418);
#5287=LINE('',#53685,#6419);
#5288=LINE('',#53834,#6420);
#5289=LINE('',#53906,#6421);
#5290=LINE('',#54127,#6422);
#5291=LINE('',#54276,#6423);
#5292=LINE('',#54348,#6424);
#5293=LINE('',#54569,#6425);
#5294=LINE('',#54718,#6426);
#5295=LINE('',#54790,#6427);
#5296=LINE('',#55011,#6428);
#5297=LINE('',#55160,#6429);
#5298=LINE('',#55232,#6430);
#5299=LINE('',#55453,#6431);
#5300=LINE('',#55602,#6432);
#5301=LINE('',#55674,#6433);
#5302=LINE('',#55895,#6434);
#5303=LINE('',#56044,#6435);
#5304=LINE('',#56116,#6436);
#5305=LINE('',#56337,#6437);
#5306=LINE('',#56486,#6438);
#5307=LINE('',#56558,#6439);
#5308=LINE('',#56779,#6440);
#5309=LINE('',#56928,#6441);
#5310=LINE('',#57000,#6442);
#5311=LINE('',#57221,#6443);
#5312=LINE('',#57370,#6444);
#5313=LINE('',#57442,#6445);
#5314=LINE('',#57663,#6446);
#5315=LINE('',#57812,#6447);
#5316=LINE('',#57884,#6448);
#5317=LINE('',#58105,#6449);
#5318=LINE('',#58254,#6450);
#5319=LINE('',#58326,#6451);
#5320=LINE('',#58547,#6452);
#5321=LINE('',#58696,#6453);
#5322=LINE('',#58768,#6454);
#5323=LINE('',#58989,#6455);
#5324=LINE('',#59138,#6456);
#5325=LINE('',#59210,#6457);
#5326=LINE('',#59431,#6458);
#5327=LINE('',#59580,#6459);
#5328=LINE('',#59652,#6460);
#5329=LINE('',#59873,#6461);
#5330=LINE('',#60022,#6462);
#5331=LINE('',#60094,#6463);
#5332=LINE('',#60315,#6464);
#5333=LINE('',#60464,#6465);
#5334=LINE('',#60536,#6466);
#5335=LINE('',#60757,#6467);
#5336=LINE('',#60906,#6468);
#5337=LINE('',#60978,#6469);
#5338=LINE('',#61199,#6470);
#5339=LINE('',#61348,#6471);
#5340=LINE('',#61420,#6472);
#5341=LINE('',#61641,#6473);
#5342=LINE('',#61644,#6474);
#5343=LINE('',#61645,#6475);
#5344=LINE('',#62020,#6476);
#5345=LINE('',#62302,#6477);
#5346=LINE('',#62304,#6478);
#6308=VECTOR('',#22373,1.);
#6309=VECTOR('',#22374,1.);
#6310=VECTOR('',#22375,1.);
#6311=VECTOR('',#22376,1.);
#6312=VECTOR('',#22379,1.);
#6313=VECTOR('',#22380,1.);
#6314=VECTOR('',#22381,1.);
#6315=VECTOR('',#22384,1.);
#6316=VECTOR('',#22385,1.);
#6317=VECTOR('',#22386,1.);
#6318=VECTOR('',#22391,1.);
#6319=VECTOR('',#22394,1.);
#6320=VECTOR('',#22397,1.);
#6321=VECTOR('',#22400,1.);
#6322=VECTOR('',#22403,1.);
#6323=VECTOR('',#22406,1.);
#6324=VECTOR('',#22409,1.);
#6325=VECTOR('',#22412,1.);
#6326=VECTOR('',#22415,1.);
#6327=VECTOR('',#22418,1.);
#6328=VECTOR('',#22421,1.);
#6329=VECTOR('',#22424,1.);
#6330=VECTOR('',#22427,1.);
#6331=VECTOR('',#22430,1.);
#6332=VECTOR('',#22433,1.);
#6333=VECTOR('',#22436,1.);
#6334=VECTOR('',#22439,1.);
#6335=VECTOR('',#22442,1.);
#6336=VECTOR('',#22445,1.);
#6337=VECTOR('',#22448,1.);
#6338=VECTOR('',#22451,1.);
#6339=VECTOR('',#22454,1.);
#6340=VECTOR('',#22457,1.);
#6341=VECTOR('',#22460,1.);
#6342=VECTOR('',#22463,1.);
#6343=VECTOR('',#22466,1.);
#6344=VECTOR('',#22469,1.);
#6345=VECTOR('',#22472,1.);
#6346=VECTOR('',#22475,1.);
#6347=VECTOR('',#22478,1.);
#6348=VECTOR('',#22481,1.);
#6349=VECTOR('',#22484,1.);
#6350=VECTOR('',#22487,1.);
#6351=VECTOR('',#22490,1.);
#6352=VECTOR('',#22493,1.);
#6353=VECTOR('',#22496,1.);
#6354=VECTOR('',#22499,1.);
#6355=VECTOR('',#22502,1.);
#6356=VECTOR('',#22505,1.);
#6357=VECTOR('',#22508,1.);
#6358=VECTOR('',#22519,2.);
#6359=VECTOR('',#22524,1.);
#6360=VECTOR('',#22525,1.);
#6361=VECTOR('',#22528,1.);
#6362=VECTOR('',#22533,1.);
#6363=VECTOR('',#22534,1.);
#6364=VECTOR('',#22537,1.);
#6365=VECTOR('',#22542,1.);
#6366=VECTOR('',#22543,1.);
#6367=VECTOR('',#22546,1.);
#6368=VECTOR('',#22551,1.);
#6369=VECTOR('',#22552,1.);
#6370=VECTOR('',#22555,1.);
#6371=VECTOR('',#22560,1.);
#6372=VECTOR('',#22561,1.);
#6373=VECTOR('',#22564,1.);
#6374=VECTOR('',#22569,1.);
#6375=VECTOR('',#22570,1.);
#6376=VECTOR('',#22573,1.);
#6377=VECTOR('',#22578,1.);
#6378=VECTOR('',#22579,1.);
#6379=VECTOR('',#22582,1.);
#6380=VECTOR('',#22587,1.);
#6381=VECTOR('',#22588,1.);
#6382=VECTOR('',#22591,1.);
#6383=VECTOR('',#22596,1.);
#6384=VECTOR('',#22597,1.);
#6385=VECTOR('',#22600,1.);
#6386=VECTOR('',#22605,1.);
#6387=VECTOR('',#22606,1.);
#6388=VECTOR('',#22609,1.);
#6389=VECTOR('',#22614,1.);
#6390=VECTOR('',#22615,1.);
#6391=VECTOR('',#22618,1.);
#6392=VECTOR('',#22623,1.);
#6393=VECTOR('',#22624,1.);
#6394=VECTOR('',#22627,1.);
#6395=VECTOR('',#22632,1.);
#6396=VECTOR('',#22633,1.);
#6397=VECTOR('',#22636,1.);
#6398=VECTOR('',#22641,1.);
#6399=VECTOR('',#22642,1.);
#6400=VECTOR('',#22645,1.);
#6401=VECTOR('',#22650,1.);
#6402=VECTOR('',#22651,1.);
#6403=VECTOR('',#22654,1.);
#6404=VECTOR('',#22659,1.);
#6405=VECTOR('',#22660,1.);
#6406=VECTOR('',#22663,1.);
#6407=VECTOR('',#22668,1.);
#6408=VECTOR('',#22669,1.);
#6409=VECTOR('',#22672,1.);
#6410=VECTOR('',#22677,1.);
#6411=VECTOR('',#22678,1.);
#6412=VECTOR('',#22681,1.);
#6413=VECTOR('',#22686,1.);
#6414=VECTOR('',#22687,1.);
#6415=VECTOR('',#22690,1.);
#6416=VECTOR('',#22695,1.);
#6417=VECTOR('',#22696,1.);
#6418=VECTOR('',#22699,1.);
#6419=VECTOR('',#22704,1.);
#6420=VECTOR('',#22705,1.);
#6421=VECTOR('',#22708,1.);
#6422=VECTOR('',#22713,1.);
#6423=VECTOR('',#22714,1.);
#6424=VECTOR('',#22717,1.);
#6425=VECTOR('',#22722,1.);
#6426=VECTOR('',#22723,1.);
#6427=VECTOR('',#22726,1.);
#6428=VECTOR('',#22731,1.);
#6429=VECTOR('',#22732,1.);
#6430=VECTOR('',#22735,1.);
#6431=VECTOR('',#22740,1.);
#6432=VECTOR('',#22741,1.);
#6433=VECTOR('',#22744,1.);
#6434=VECTOR('',#22749,1.);
#6435=VECTOR('',#22750,1.);
#6436=VECTOR('',#22753,1.);
#6437=VECTOR('',#22758,1.);
#6438=VECTOR('',#22759,1.);
#6439=VECTOR('',#22762,1.);
#6440=VECTOR('',#22767,1.);
#6441=VECTOR('',#22768,1.);
#6442=VECTOR('',#22771,1.);
#6443=VECTOR('',#22776,1.);
#6444=VECTOR('',#22777,1.);
#6445=VECTOR('',#22780,1.);
#6446=VECTOR('',#22785,1.);
#6447=VECTOR('',#22786,1.);
#6448=VECTOR('',#22789,1.);
#6449=VECTOR('',#22794,1.);
#6450=VECTOR('',#22795,1.);
#6451=VECTOR('',#22798,1.);
#6452=VECTOR('',#22803,1.);
#6453=VECTOR('',#22804,1.);
#6454=VECTOR('',#22807,1.);
#6455=VECTOR('',#22812,1.);
#6456=VECTOR('',#22813,1.);
#6457=VECTOR('',#22816,1.);
#6458=VECTOR('',#22821,1.);
#6459=VECTOR('',#22822,1.);
#6460=VECTOR('',#22825,1.);
#6461=VECTOR('',#22830,1.);
#6462=VECTOR('',#22831,1.);
#6463=VECTOR('',#22834,1.);
#6464=VECTOR('',#22839,1.);
#6465=VECTOR('',#22840,1.);
#6466=VECTOR('',#22843,1.);
#6467=VECTOR('',#22848,1.);
#6468=VECTOR('',#22849,1.);
#6469=VECTOR('',#22852,1.);
#6470=VECTOR('',#22857,1.);
#6471=VECTOR('',#22858,1.);
#6472=VECTOR('',#22861,1.);
#6473=VECTOR('',#22866,1.);
#6474=VECTOR('',#22869,1.);
#6475=VECTOR('',#22870,1.);
#6476=VECTOR('',#22875,1.);
#6477=VECTOR('',#22876,1.);
#6478=VECTOR('',#22879,1.);
#7112=CIRCLE('',#18487,3.75);
#7113=CIRCLE('',#18488,3.75);
#7114=CIRCLE('',#18489,3.75);
#7115=CIRCLE('',#18490,3.75);
#7116=CIRCLE('',#18491,3.75);
#7117=CIRCLE('',#18492,3.75);
#7118=CIRCLE('',#18493,3.75);
#7119=CIRCLE('',#18494,3.75);
#7120=CIRCLE('',#18495,3.75);
#7121=CIRCLE('',#18496,3.75);
#7122=CIRCLE('',#18497,3.75);
#7123=CIRCLE('',#18498,3.75);
#7124=CIRCLE('',#18499,3.75);
#7125=CIRCLE('',#18500,3.75);
#7126=CIRCLE('',#18501,3.75);
#7127=CIRCLE('',#18502,3.75);
#7128=CIRCLE('',#18503,3.75);
#7129=CIRCLE('',#18504,3.75);
#7130=CIRCLE('',#18505,3.75);
#7131=CIRCLE('',#18506,3.75);
#7132=CIRCLE('',#18507,3.75);
#7133=CIRCLE('',#18508,3.75);
#7134=CIRCLE('',#18509,3.75);
#7135=CIRCLE('',#18510,3.75);
#7136=CIRCLE('',#18511,3.75);
#7137=CIRCLE('',#18512,3.75);
#7138=CIRCLE('',#18513,3.75);
#7139=CIRCLE('',#18514,3.75);
#7140=CIRCLE('',#18515,3.75);
#7141=CIRCLE('',#18516,3.75);
#7142=CIRCLE('',#18517,3.75);
#7143=CIRCLE('',#18518,3.75);
#7144=CIRCLE('',#18519,3.75);
#7145=CIRCLE('',#18520,3.75);
#7146=CIRCLE('',#18521,3.75);
#7147=CIRCLE('',#18522,3.75);
#7148=CIRCLE('',#18523,3.75);
#7149=CIRCLE('',#18524,3.75);
#7150=CIRCLE('',#18525,3.75);
#7151=CIRCLE('',#18526,3.75);
#7152=CIRCLE('',#18527,1.);
#7153=CIRCLE('',#18529,1.);
#7154=CIRCLE('',#18531,2.);
#7155=CIRCLE('',#18532,2.);
#7156=CIRCLE('',#18536,3.75);
#7157=CIRCLE('',#18539,3.75);
#7158=CIRCLE('',#18542,3.75);
#7159=CIRCLE('',#18545,3.75);
#7160=CIRCLE('',#18548,3.75);
#7161=CIRCLE('',#18551,3.75);
#7162=CIRCLE('',#18554,3.75);
#7163=CIRCLE('',#18557,3.75);
#7164=CIRCLE('',#18560,3.75);
#7165=CIRCLE('',#18563,3.75);
#7166=CIRCLE('',#18566,3.75);
#7167=CIRCLE('',#18569,3.75);
#7168=CIRCLE('',#18572,3.75);
#7169=CIRCLE('',#18575,3.75);
#7170=CIRCLE('',#18578,3.75);
#7171=CIRCLE('',#18581,3.75);
#7172=CIRCLE('',#18584,3.75);
#7173=CIRCLE('',#18587,3.75);
#7174=CIRCLE('',#18590,3.75);
#7175=CIRCLE('',#18593,3.75);
#7176=CIRCLE('',#18596,3.75);
#7177=CIRCLE('',#18599,3.75);
#7178=CIRCLE('',#18602,3.75);
#7179=CIRCLE('',#18605,3.75);
#7180=CIRCLE('',#18608,3.75);
#7181=CIRCLE('',#18611,3.75);
#7182=CIRCLE('',#18614,3.75);
#7183=CIRCLE('',#18617,3.75);
#7184=CIRCLE('',#18620,3.75);
#7185=CIRCLE('',#18623,3.75);
#7186=CIRCLE('',#18626,3.75);
#7187=CIRCLE('',#18629,3.75);
#7188=CIRCLE('',#18632,3.75);
#7189=CIRCLE('',#18635,3.75);
#7190=CIRCLE('',#18638,3.75);
#7191=CIRCLE('',#18641,3.75);
#7192=CIRCLE('',#18644,3.75);
#7193=CIRCLE('',#18647,3.75);
#7194=CIRCLE('',#18650,3.75);
#7195=CIRCLE('',#18653,3.75);
#8283=VERTEX_POINT('',#38756);
#8284=VERTEX_POINT('',#38757);
#8285=VERTEX_POINT('',#38759);
#8286=VERTEX_POINT('',#38761);
#8287=VERTEX_POINT('',#38765);
#8288=VERTEX_POINT('',#38767);
#8289=VERTEX_POINT('',#38771);
#8290=VERTEX_POINT('',#38773);
#8291=VERTEX_POINT('',#38777);
#8292=VERTEX_POINT('',#38778);
#8293=VERTEX_POINT('',#38780);
#8294=VERTEX_POINT('',#38851);
#8295=VERTEX_POINT('',#38853);
#8296=VERTEX_POINT('',#38924);
#8297=VERTEX_POINT('',#38926);
#8298=VERTEX_POINT('',#38997);
#8299=VERTEX_POINT('',#38999);
#8300=VERTEX_POINT('',#39070);
#8301=VERTEX_POINT('',#39072);
#8302=VERTEX_POINT('',#39143);
#8303=VERTEX_POINT('',#39145);
#8304=VERTEX_POINT('',#39216);
#8305=VERTEX_POINT('',#39218);
#8306=VERTEX_POINT('',#39289);
#8307=VERTEX_POINT('',#39291);
#8308=VERTEX_POINT('',#39362);
#8309=VERTEX_POINT('',#39364);
#8310=VERTEX_POINT('',#39435);
#8311=VERTEX_POINT('',#39437);
#8312=VERTEX_POINT('',#39508);
#8313=VERTEX_POINT('',#39510);
#8314=VERTEX_POINT('',#39581);
#8315=VERTEX_POINT('',#39583);
#8316=VERTEX_POINT('',#39654);
#8317=VERTEX_POINT('',#39656);
#8318=VERTEX_POINT('',#39727);
#8319=VERTEX_POINT('',#39729);
#8320=VERTEX_POINT('',#39800);
#8321=VERTEX_POINT('',#39802);
#8322=VERTEX_POINT('',#39873);
#8323=VERTEX_POINT('',#39875);
#8324=VERTEX_POINT('',#39946);
#8325=VERTEX_POINT('',#39948);
#8326=VERTEX_POINT('',#40019);
#8327=VERTEX_POINT('',#40021);
#8328=VERTEX_POINT('',#40092);
#8329=VERTEX_POINT('',#40094);
#8330=VERTEX_POINT('',#40165);
#8331=VERTEX_POINT('',#40167);
#8332=VERTEX_POINT('',#40238);
#8333=VERTEX_POINT('',#40240);
#8334=VERTEX_POINT('',#40311);
#8335=VERTEX_POINT('',#40313);
#8336=VERTEX_POINT('',#40384);
#8337=VERTEX_POINT('',#40386);
#8338=VERTEX_POINT('',#40457);
#8339=VERTEX_POINT('',#40459);
#8340=VERTEX_POINT('',#40530);
#8341=VERTEX_POINT('',#40532);
#8342=VERTEX_POINT('',#40603);
#8343=VERTEX_POINT('',#40605);
#8344=VERTEX_POINT('',#40676);
#8345=VERTEX_POINT('',#40678);
#8346=VERTEX_POINT('',#40749);
#8347=VERTEX_POINT('',#40751);
#8348=VERTEX_POINT('',#40822);
#8349=VERTEX_POINT('',#40824);
#8350=VERTEX_POINT('',#40895);
#8351=VERTEX_POINT('',#40897);
#8352=VERTEX_POINT('',#40968);
#8353=VERTEX_POINT('',#40970);
#8354=VERTEX_POINT('',#41041);
#8355=VERTEX_POINT('',#41043);
#8356=VERTEX_POINT('',#41114);
#8357=VERTEX_POINT('',#41116);
#8358=VERTEX_POINT('',#41187);
#8359=VERTEX_POINT('',#41189);
#8360=VERTEX_POINT('',#41260);
#8361=VERTEX_POINT('',#41262);
#8362=VERTEX_POINT('',#41333);
#8363=VERTEX_POINT('',#41335);
#8364=VERTEX_POINT('',#41406);
#8365=VERTEX_POINT('',#41408);
#8366=VERTEX_POINT('',#41479);
#8367=VERTEX_POINT('',#41481);
#8368=VERTEX_POINT('',#41552);
#8369=VERTEX_POINT('',#41554);
#8370=VERTEX_POINT('',#41625);
#8371=VERTEX_POINT('',#41627);
#8372=VERTEX_POINT('',#41698);
#8373=VERTEX_POINT('',#41700);
#8374=VERTEX_POINT('',#41771);
#8375=VERTEX_POINT('',#41773);
#8376=VERTEX_POINT('',#41844);
#8377=VERTEX_POINT('',#41846);
#8378=VERTEX_POINT('',#41917);
#8379=VERTEX_POINT('',#41919);
#8380=VERTEX_POINT('',#41990);
#8381=VERTEX_POINT('',#41992);
#8382=VERTEX_POINT('',#42063);
#8383=VERTEX_POINT('',#42065);
#8384=VERTEX_POINT('',#42136);
#8385=VERTEX_POINT('',#42138);
#8386=VERTEX_POINT('',#42209);
#8387=VERTEX_POINT('',#42211);
#8388=VERTEX_POINT('',#42282);
#8389=VERTEX_POINT('',#42284);
#8390=VERTEX_POINT('',#42355);
#8391=VERTEX_POINT('',#42357);
#8392=VERTEX_POINT('',#42428);
#8393=VERTEX_POINT('',#42430);
#8394=VERTEX_POINT('',#42501);
#8395=VERTEX_POINT('',#42503);
#8396=VERTEX_POINT('',#42574);
#8397=VERTEX_POINT('',#42576);
#8398=VERTEX_POINT('',#42647);
#8399=VERTEX_POINT('',#42649);
#8400=VERTEX_POINT('',#42720);
#8401=VERTEX_POINT('',#42722);
#8402=VERTEX_POINT('',#42793);
#8403=VERTEX_POINT('',#42795);
#8404=VERTEX_POINT('',#42866);
#8405=VERTEX_POINT('',#42868);
#8406=VERTEX_POINT('',#42939);
#8407=VERTEX_POINT('',#42941);
#8408=VERTEX_POINT('',#43012);
#8409=VERTEX_POINT('',#43014);
#8410=VERTEX_POINT('',#43085);
#8411=VERTEX_POINT('',#43087);
#8412=VERTEX_POINT('',#43158);
#8413=VERTEX_POINT('',#43160);
#8414=VERTEX_POINT('',#43231);
#8415=VERTEX_POINT('',#43233);
#8416=VERTEX_POINT('',#43304);
#8417=VERTEX_POINT('',#43306);
#8418=VERTEX_POINT('',#43377);
#8419=VERTEX_POINT('',#43379);
#8420=VERTEX_POINT('',#43450);
#8421=VERTEX_POINT('',#43452);
#8422=VERTEX_POINT('',#43523);
#8423=VERTEX_POINT('',#43525);
#8424=VERTEX_POINT('',#43596);
#8425=VERTEX_POINT('',#43598);
#8426=VERTEX_POINT('',#43669);
#8427=VERTEX_POINT('',#43671);
#8428=VERTEX_POINT('',#43742);
#8429=VERTEX_POINT('',#43744);
#8430=VERTEX_POINT('',#43815);
#8431=VERTEX_POINT('',#43817);
#8432=VERTEX_POINT('',#43888);
#8433=VERTEX_POINT('',#43890);
#8434=VERTEX_POINT('',#43961);
#8435=VERTEX_POINT('',#43963);
#8436=VERTEX_POINT('',#44034);
#8437=VERTEX_POINT('',#44036);
#8438=VERTEX_POINT('',#44107);
#8439=VERTEX_POINT('',#44109);
#8440=VERTEX_POINT('',#44180);
#8441=VERTEX_POINT('',#44182);
#8442=VERTEX_POINT('',#44253);
#8443=VERTEX_POINT('',#44255);
#8444=VERTEX_POINT('',#44326);
#8445=VERTEX_POINT('',#44328);
#8446=VERTEX_POINT('',#44399);
#8447=VERTEX_POINT('',#44401);
#8448=VERTEX_POINT('',#44472);
#8449=VERTEX_POINT('',#44474);
#8450=VERTEX_POINT('',#44545);
#8451=VERTEX_POINT('',#44621);
#8452=VERTEX_POINT('',#44623);
#8453=VERTEX_POINT('',#44767);
#8454=VERTEX_POINT('',#44774);
#8455=VERTEX_POINT('',#44986);
#8456=VERTEX_POINT('',#44993);
#8457=VERTEX_POINT('',#45068);
#8458=VERTEX_POINT('',#45216);
#8459=VERTEX_POINT('',#45428);
#8460=VERTEX_POINT('',#45435);
#8461=VERTEX_POINT('',#45510);
#8462=VERTEX_POINT('',#45658);
#8463=VERTEX_POINT('',#45870);
#8464=VERTEX_POINT('',#45877);
#8465=VERTEX_POINT('',#45952);
#8466=VERTEX_POINT('',#46100);
#8467=VERTEX_POINT('',#46312);
#8468=VERTEX_POINT('',#46319);
#8469=VERTEX_POINT('',#46394);
#8470=VERTEX_POINT('',#46542);
#8471=VERTEX_POINT('',#46754);
#8472=VERTEX_POINT('',#46761);
#8473=VERTEX_POINT('',#46836);
#8474=VERTEX_POINT('',#46984);
#8475=VERTEX_POINT('',#47196);
#8476=VERTEX_POINT('',#47203);
#8477=VERTEX_POINT('',#47278);
#8478=VERTEX_POINT('',#47426);
#8479=VERTEX_POINT('',#47638);
#8480=VERTEX_POINT('',#47645);
#8481=VERTEX_POINT('',#47720);
#8482=VERTEX_POINT('',#47868);
#8483=VERTEX_POINT('',#48080);
#8484=VERTEX_POINT('',#48087);
#8485=VERTEX_POINT('',#48162);
#8486=VERTEX_POINT('',#48310);
#8487=VERTEX_POINT('',#48522);
#8488=VERTEX_POINT('',#48529);
#8489=VERTEX_POINT('',#48604);
#8490=VERTEX_POINT('',#48752);
#8491=VERTEX_POINT('',#48964);
#8492=VERTEX_POINT('',#48971);
#8493=VERTEX_POINT('',#49046);
#8494=VERTEX_POINT('',#49194);
#8495=VERTEX_POINT('',#49406);
#8496=VERTEX_POINT('',#49413);
#8497=VERTEX_POINT('',#49488);
#8498=VERTEX_POINT('',#49636);
#8499=VERTEX_POINT('',#49848);
#8500=VERTEX_POINT('',#49855);
#8501=VERTEX_POINT('',#49930);
#8502=VERTEX_POINT('',#50078);
#8503=VERTEX_POINT('',#50290);
#8504=VERTEX_POINT('',#50297);
#8505=VERTEX_POINT('',#50372);
#8506=VERTEX_POINT('',#50520);
#8507=VERTEX_POINT('',#50732);
#8508=VERTEX_POINT('',#50739);
#8509=VERTEX_POINT('',#50814);
#8510=VERTEX_POINT('',#50962);
#8511=VERTEX_POINT('',#51174);
#8512=VERTEX_POINT('',#51181);
#8513=VERTEX_POINT('',#51256);
#8514=VERTEX_POINT('',#51404);
#8515=VERTEX_POINT('',#51616);
#8516=VERTEX_POINT('',#51623);
#8517=VERTEX_POINT('',#51698);
#8518=VERTEX_POINT('',#51846);
#8519=VERTEX_POINT('',#52058);
#8520=VERTEX_POINT('',#52065);
#8521=VERTEX_POINT('',#52140);
#8522=VERTEX_POINT('',#52288);
#8523=VERTEX_POINT('',#52500);
#8524=VERTEX_POINT('',#52507);
#8525=VERTEX_POINT('',#52582);
#8526=VERTEX_POINT('',#52730);
#8527=VERTEX_POINT('',#52942);
#8528=VERTEX_POINT('',#52949);
#8529=VERTEX_POINT('',#53024);
#8530=VERTEX_POINT('',#53172);
#8531=VERTEX_POINT('',#53384);
#8532=VERTEX_POINT('',#53391);
#8533=VERTEX_POINT('',#53466);
#8534=VERTEX_POINT('',#53614);
#8535=VERTEX_POINT('',#53826);
#8536=VERTEX_POINT('',#53833);
#8537=VERTEX_POINT('',#53908);
#8538=VERTEX_POINT('',#54056);
#8539=VERTEX_POINT('',#54268);
#8540=VERTEX_POINT('',#54275);
#8541=VERTEX_POINT('',#54350);
#8542=VERTEX_POINT('',#54498);
#8543=VERTEX_POINT('',#54710);
#8544=VERTEX_POINT('',#54717);
#8545=VERTEX_POINT('',#54792);
#8546=VERTEX_POINT('',#54940);
#8547=VERTEX_POINT('',#55152);
#8548=VERTEX_POINT('',#55159);
#8549=VERTEX_POINT('',#55234);
#8550=VERTEX_POINT('',#55382);
#8551=VERTEX_POINT('',#55594);
#8552=VERTEX_POINT('',#55601);
#8553=VERTEX_POINT('',#55676);
#8554=VERTEX_POINT('',#55824);
#8555=VERTEX_POINT('',#56036);
#8556=VERTEX_POINT('',#56043);
#8557=VERTEX_POINT('',#56118);
#8558=VERTEX_POINT('',#56266);
#8559=VERTEX_POINT('',#56478);
#8560=VERTEX_POINT('',#56485);
#8561=VERTEX_POINT('',#56560);
#8562=VERTEX_POINT('',#56708);
#8563=VERTEX_POINT('',#56920);
#8564=VERTEX_POINT('',#56927);
#8565=VERTEX_POINT('',#57002);
#8566=VERTEX_POINT('',#57150);
#8567=VERTEX_POINT('',#57362);
#8568=VERTEX_POINT('',#57369);
#8569=VERTEX_POINT('',#57444);
#8570=VERTEX_POINT('',#57592);
#8571=VERTEX_POINT('',#57804);
#8572=VERTEX_POINT('',#57811);
#8573=VERTEX_POINT('',#57886);
#8574=VERTEX_POINT('',#58034);
#8575=VERTEX_POINT('',#58246);
#8576=VERTEX_POINT('',#58253);
#8577=VERTEX_POINT('',#58328);
#8578=VERTEX_POINT('',#58476);
#8579=VERTEX_POINT('',#58688);
#8580=VERTEX_POINT('',#58695);
#8581=VERTEX_POINT('',#58770);
#8582=VERTEX_POINT('',#58918);
#8583=VERTEX_POINT('',#59130);
#8584=VERTEX_POINT('',#59137);
#8585=VERTEX_POINT('',#59212);
#8586=VERTEX_POINT('',#59360);
#8587=VERTEX_POINT('',#59572);
#8588=VERTEX_POINT('',#59579);
#8589=VERTEX_POINT('',#59654);
#8590=VERTEX_POINT('',#59802);
#8591=VERTEX_POINT('',#60014);
#8592=VERTEX_POINT('',#60021);
#8593=VERTEX_POINT('',#60096);
#8594=VERTEX_POINT('',#60244);
#8595=VERTEX_POINT('',#60456);
#8596=VERTEX_POINT('',#60463);
#8597=VERTEX_POINT('',#60538);
#8598=VERTEX_POINT('',#60686);
#8599=VERTEX_POINT('',#60898);
#8600=VERTEX_POINT('',#60905);
#8601=VERTEX_POINT('',#60980);
#8602=VERTEX_POINT('',#61128);
#8603=VERTEX_POINT('',#61340);
#8604=VERTEX_POINT('',#61347);
#8605=VERTEX_POINT('',#61422);
#8606=VERTEX_POINT('',#61570);
#8607=VERTEX_POINT('',#61643);
#8608=VERTEX_POINT('',#61786);
#8609=VERTEX_POINT('',#61864);
#8610=VERTEX_POINT('',#62012);
#8611=VERTEX_POINT('',#62019);
#8612=VERTEX_POINT('',#62231);
#10253=EDGE_CURVE('',#8283,#8284,#5176,.T.);
#10254=EDGE_CURVE('',#8285,#8283,#5177,.T.);
#10255=EDGE_CURVE('',#8286,#8285,#5178,.T.);
#10256=EDGE_CURVE('',#8284,#8286,#5179,.T.);
#10257=EDGE_CURVE('',#8287,#8283,#5180,.T.);
#10258=EDGE_CURVE('',#8287,#8288,#5181,.T.);
#10259=EDGE_CURVE('',#8285,#8288,#5182,.T.);
#10260=EDGE_CURVE('',#8289,#8287,#5183,.T.);
#10261=EDGE_CURVE('',#8290,#8289,#5184,.T.);
#10262=EDGE_CURVE('',#8288,#8290,#5185,.T.);
#10263=EDGE_CURVE('',#8291,#8292,#7112,.T.);
#10264=EDGE_CURVE('',#8292,#8293,#211,.T.);
#10265=EDGE_CURVE('',#8293,#8294,#5186,.T.);
#10266=EDGE_CURVE('',#8294,#8295,#212,.T.);
#10267=EDGE_CURVE('',#8295,#8296,#7113,.T.);
#10268=EDGE_CURVE('',#8296,#8297,#213,.T.);
#10269=EDGE_CURVE('',#8297,#8298,#5187,.T.);
#10270=EDGE_CURVE('',#8298,#8299,#214,.T.);
#10271=EDGE_CURVE('',#8299,#8300,#7114,.T.);
#10272=EDGE_CURVE('',#8300,#8301,#215,.T.);
#10273=EDGE_CURVE('',#8301,#8302,#5188,.T.);
#10274=EDGE_CURVE('',#8302,#8303,#216,.T.);
#10275=EDGE_CURVE('',#8303,#8304,#7115,.T.);
#10276=EDGE_CURVE('',#8304,#8305,#217,.T.);
#10277=EDGE_CURVE('',#8305,#8306,#5189,.T.);
#10278=EDGE_CURVE('',#8306,#8307,#218,.T.);
#10279=EDGE_CURVE('',#8307,#8308,#7116,.T.);
#10280=EDGE_CURVE('',#8308,#8309,#219,.T.);
#10281=EDGE_CURVE('',#8309,#8310,#5190,.T.);
#10282=EDGE_CURVE('',#8310,#8311,#220,.T.);
#10283=EDGE_CURVE('',#8311,#8312,#7117,.T.);
#10284=EDGE_CURVE('',#8312,#8313,#221,.T.);
#10285=EDGE_CURVE('',#8313,#8314,#5191,.T.);
#10286=EDGE_CURVE('',#8314,#8315,#222,.T.);
#10287=EDGE_CURVE('',#8315,#8316,#7118,.T.);
#10288=EDGE_CURVE('',#8316,#8317,#223,.T.);
#10289=EDGE_CURVE('',#8317,#8318,#5192,.T.);
#10290=EDGE_CURVE('',#8318,#8319,#224,.T.);
#10291=EDGE_CURVE('',#8319,#8320,#7119,.T.);
#10292=EDGE_CURVE('',#8320,#8321,#225,.T.);
#10293=EDGE_CURVE('',#8321,#8322,#5193,.T.);
#10294=EDGE_CURVE('',#8322,#8323,#226,.T.);
#10295=EDGE_CURVE('',#8323,#8324,#7120,.T.);
#10296=EDGE_CURVE('',#8324,#8325,#227,.T.);
#10297=EDGE_CURVE('',#8325,#8326,#5194,.T.);
#10298=EDGE_CURVE('',#8326,#8327,#228,.T.);
#10299=EDGE_CURVE('',#8327,#8328,#7121,.T.);
#10300=EDGE_CURVE('',#8328,#8329,#229,.T.);
#10301=EDGE_CURVE('',#8329,#8330,#5195,.T.);
#10302=EDGE_CURVE('',#8330,#8331,#230,.T.);
#10303=EDGE_CURVE('',#8331,#8332,#7122,.T.);
#10304=EDGE_CURVE('',#8332,#8333,#231,.T.);
#10305=EDGE_CURVE('',#8333,#8334,#5196,.T.);
#10306=EDGE_CURVE('',#8334,#8335,#232,.T.);
#10307=EDGE_CURVE('',#8335,#8336,#7123,.T.);
#10308=EDGE_CURVE('',#8336,#8337,#233,.T.);
#10309=EDGE_CURVE('',#8337,#8338,#5197,.T.);
#10310=EDGE_CURVE('',#8338,#8339,#234,.T.);
#10311=EDGE_CURVE('',#8339,#8340,#7124,.T.);
#10312=EDGE_CURVE('',#8340,#8341,#235,.T.);
#10313=EDGE_CURVE('',#8341,#8342,#5198,.T.);
#10314=EDGE_CURVE('',#8342,#8343,#236,.T.);
#10315=EDGE_CURVE('',#8343,#8344,#7125,.T.);
#10316=EDGE_CURVE('',#8344,#8345,#237,.T.);
#10317=EDGE_CURVE('',#8345,#8346,#5199,.T.);
#10318=EDGE_CURVE('',#8346,#8347,#238,.T.);
#10319=EDGE_CURVE('',#8347,#8348,#7126,.T.);
#10320=EDGE_CURVE('',#8348,#8349,#239,.T.);
#10321=EDGE_CURVE('',#8349,#8350,#5200,.T.);
#10322=EDGE_CURVE('',#8350,#8351,#240,.T.);
#10323=EDGE_CURVE('',#8351,#8352,#7127,.T.);
#10324=EDGE_CURVE('',#8352,#8353,#241,.T.);
#10325=EDGE_CURVE('',#8353,#8354,#5201,.T.);
#10326=EDGE_CURVE('',#8354,#8355,#242,.T.);
#10327=EDGE_CURVE('',#8355,#8356,#7128,.T.);
#10328=EDGE_CURVE('',#8356,#8357,#243,.T.);
#10329=EDGE_CURVE('',#8357,#8358,#5202,.T.);
#10330=EDGE_CURVE('',#8358,#8359,#244,.T.);
#10331=EDGE_CURVE('',#8359,#8360,#7129,.T.);
#10332=EDGE_CURVE('',#8360,#8361,#245,.T.);
#10333=EDGE_CURVE('',#8361,#8362,#5203,.T.);
#10334=EDGE_CURVE('',#8362,#8363,#246,.T.);
#10335=EDGE_CURVE('',#8363,#8364,#7130,.T.);
#10336=EDGE_CURVE('',#8364,#8365,#247,.T.);
#10337=EDGE_CURVE('',#8365,#8366,#5204,.T.);
#10338=EDGE_CURVE('',#8366,#8367,#248,.T.);
#10339=EDGE_CURVE('',#8367,#8368,#7131,.T.);
#10340=EDGE_CURVE('',#8368,#8369,#249,.T.);
#10341=EDGE_CURVE('',#8369,#8370,#5205,.T.);
#10342=EDGE_CURVE('',#8370,#8371,#250,.T.);
#10343=EDGE_CURVE('',#8371,#8372,#7132,.T.);
#10344=EDGE_CURVE('',#8372,#8373,#251,.T.);
#10345=EDGE_CURVE('',#8373,#8374,#5206,.T.);
#10346=EDGE_CURVE('',#8374,#8375,#252,.T.);
#10347=EDGE_CURVE('',#8375,#8376,#7133,.T.);
#10348=EDGE_CURVE('',#8376,#8377,#253,.T.);
#10349=EDGE_CURVE('',#8377,#8378,#5207,.T.);
#10350=EDGE_CURVE('',#8378,#8379,#254,.T.);
#10351=EDGE_CURVE('',#8379,#8380,#7134,.T.);
#10352=EDGE_CURVE('',#8380,#8381,#255,.T.);
#10353=EDGE_CURVE('',#8381,#8382,#5208,.T.);
#10354=EDGE_CURVE('',#8382,#8383,#256,.T.);
#10355=EDGE_CURVE('',#8383,#8384,#7135,.T.);
#10356=EDGE_CURVE('',#8384,#8385,#257,.T.);
#10357=EDGE_CURVE('',#8385,#8386,#5209,.T.);
#10358=EDGE_CURVE('',#8386,#8387,#258,.T.);
#10359=EDGE_CURVE('',#8387,#8388,#7136,.T.);
#10360=EDGE_CURVE('',#8388,#8389,#259,.T.);
#10361=EDGE_CURVE('',#8389,#8390,#5210,.T.);
#10362=EDGE_CURVE('',#8390,#8391,#260,.T.);
#10363=EDGE_CURVE('',#8391,#8392,#7137,.T.);
#10364=EDGE_CURVE('',#8392,#8393,#261,.T.);
#10365=EDGE_CURVE('',#8393,#8394,#5211,.T.);
#10366=EDGE_CURVE('',#8394,#8395,#262,.T.);
#10367=EDGE_CURVE('',#8395,#8396,#7138,.T.);
#10368=EDGE_CURVE('',#8396,#8397,#263,.T.);
#10369=EDGE_CURVE('',#8397,#8398,#5212,.T.);
#10370=EDGE_CURVE('',#8398,#8399,#264,.T.);
#10371=EDGE_CURVE('',#8399,#8400,#7139,.T.);
#10372=EDGE_CURVE('',#8400,#8401,#265,.T.);
#10373=EDGE_CURVE('',#8401,#8402,#5213,.T.);
#10374=EDGE_CURVE('',#8402,#8403,#266,.T.);
#10375=EDGE_CURVE('',#8403,#8404,#7140,.T.);
#10376=EDGE_CURVE('',#8404,#8405,#267,.T.);
#10377=EDGE_CURVE('',#8405,#8406,#5214,.T.);
#10378=EDGE_CURVE('',#8406,#8407,#268,.T.);
#10379=EDGE_CURVE('',#8407,#8408,#7141,.T.);
#10380=EDGE_CURVE('',#8408,#8409,#269,.T.);
#10381=EDGE_CURVE('',#8409,#8410,#5215,.T.);
#10382=EDGE_CURVE('',#8410,#8411,#270,.T.);
#10383=EDGE_CURVE('',#8411,#8412,#7142,.T.);
#10384=EDGE_CURVE('',#8412,#8413,#271,.T.);
#10385=EDGE_CURVE('',#8413,#8414,#5216,.T.);
#10386=EDGE_CURVE('',#8414,#8415,#272,.T.);
#10387=EDGE_CURVE('',#8415,#8416,#7143,.T.);
#10388=EDGE_CURVE('',#8416,#8417,#273,.T.);
#10389=EDGE_CURVE('',#8417,#8418,#5217,.T.);
#10390=EDGE_CURVE('',#8418,#8419,#274,.T.);
#10391=EDGE_CURVE('',#8419,#8420,#7144,.T.);
#10392=EDGE_CURVE('',#8420,#8421,#275,.T.);
#10393=EDGE_CURVE('',#8421,#8422,#5218,.T.);
#10394=EDGE_CURVE('',#8422,#8423,#276,.T.);
#10395=EDGE_CURVE('',#8423,#8424,#7145,.T.);
#10396=EDGE_CURVE('',#8424,#8425,#277,.T.);
#10397=EDGE_CURVE('',#8425,#8426,#5219,.T.);
#10398=EDGE_CURVE('',#8426,#8427,#278,.T.);
#10399=EDGE_CURVE('',#8427,#8428,#7146,.T.);
#10400=EDGE_CURVE('',#8428,#8429,#279,.T.);
#10401=EDGE_CURVE('',#8429,#8430,#5220,.T.);
#10402=EDGE_CURVE('',#8430,#8431,#280,.T.);
#10403=EDGE_CURVE('',#8431,#8432,#7147,.T.);
#10404=EDGE_CURVE('',#8432,#8433,#281,.T.);
#10405=EDGE_CURVE('',#8433,#8434,#5221,.T.);
#10406=EDGE_CURVE('',#8434,#8435,#282,.T.);
#10407=EDGE_CURVE('',#8435,#8436,#7148,.T.);
#10408=EDGE_CURVE('',#8436,#8437,#283,.T.);
#10409=EDGE_CURVE('',#8437,#8438,#5222,.T.);
#10410=EDGE_CURVE('',#8438,#8439,#284,.T.);
#10411=EDGE_CURVE('',#8439,#8440,#7149,.T.);
#10412=EDGE_CURVE('',#8440,#8441,#285,.T.);
#10413=EDGE_CURVE('',#8441,#8442,#5223,.T.);
#10414=EDGE_CURVE('',#8442,#8443,#286,.T.);
#10415=EDGE_CURVE('',#8443,#8444,#7150,.T.);
#10416=EDGE_CURVE('',#8444,#8445,#287,.T.);
#10417=EDGE_CURVE('',#8445,#8446,#5224,.T.);
#10418=EDGE_CURVE('',#8446,#8447,#288,.T.);
#10419=EDGE_CURVE('',#8447,#8448,#7151,.T.);
#10420=EDGE_CURVE('',#8448,#8449,#289,.T.);
#10421=EDGE_CURVE('',#8449,#8450,#5225,.T.);
#10422=EDGE_CURVE('',#8450,#8291,#290,.T.);
#10423=EDGE_CURVE('',#8290,#8286,#7152,.T.);
#10424=EDGE_CURVE('',#8284,#8289,#7153,.T.);
#10425=EDGE_CURVE('',#8451,#8451,#7154,.T.);
#10426=EDGE_CURVE('',#8451,#8452,#5226,.T.);
#10427=EDGE_CURVE('',#8452,#8452,#7155,.T.);
#10428=EDGE_CURVE('',#8453,#8448,#911,.T.);
#10429=EDGE_CURVE('',#8454,#8453,#291,.T.);
#10430=EDGE_CURVE('',#8449,#8454,#5227,.T.);
#10431=EDGE_CURVE('',#8291,#8455,#912,.T.);
#10432=EDGE_CURVE('',#8450,#8456,#5228,.T.);
#10433=EDGE_CURVE('',#8455,#8456,#292,.T.);
#10434=EDGE_CURVE('',#8456,#8454,#5229,.T.);
#10435=EDGE_CURVE('',#8457,#8455,#7156,.T.);
#10436=EDGE_CURVE('',#8457,#8292,#913,.T.);
#10437=EDGE_CURVE('',#8458,#8457,#293,.T.);
#10438=EDGE_CURVE('',#8293,#8458,#5230,.T.);
#10439=EDGE_CURVE('',#8295,#8459,#914,.T.);
#10440=EDGE_CURVE('',#8294,#8460,#5231,.T.);
#10441=EDGE_CURVE('',#8459,#8460,#294,.T.);
#10442=EDGE_CURVE('',#8460,#8458,#5232,.T.);
#10443=EDGE_CURVE('',#8461,#8459,#7157,.T.);
#10444=EDGE_CURVE('',#8461,#8296,#915,.T.);
#10445=EDGE_CURVE('',#8462,#8461,#295,.T.);
#10446=EDGE_CURVE('',#8297,#8462,#5233,.T.);
#10447=EDGE_CURVE('',#8299,#8463,#916,.T.);
#10448=EDGE_CURVE('',#8298,#8464,#5234,.T.);
#10449=EDGE_CURVE('',#8463,#8464,#296,.T.);
#10450=EDGE_CURVE('',#8464,#8462,#5235,.T.);
#10451=EDGE_CURVE('',#8465,#8463,#7158,.T.);
#10452=EDGE_CURVE('',#8465,#8300,#917,.T.);
#10453=EDGE_CURVE('',#8466,#8465,#297,.T.);
#10454=EDGE_CURVE('',#8301,#8466,#5236,.T.);
#10455=EDGE_CURVE('',#8303,#8467,#918,.T.);
#10456=EDGE_CURVE('',#8302,#8468,#5237,.T.);
#10457=EDGE_CURVE('',#8467,#8468,#298,.T.);
#10458=EDGE_CURVE('',#8468,#8466,#5238,.T.);
#10459=EDGE_CURVE('',#8469,#8467,#7159,.T.);
#10460=EDGE_CURVE('',#8469,#8304,#919,.T.);
#10461=EDGE_CURVE('',#8470,#8469,#299,.T.);
#10462=EDGE_CURVE('',#8305,#8470,#5239,.T.);
#10463=EDGE_CURVE('',#8307,#8471,#920,.T.);
#10464=EDGE_CURVE('',#8306,#8472,#5240,.T.);
#10465=EDGE_CURVE('',#8471,#8472,#300,.T.);
#10466=EDGE_CURVE('',#8472,#8470,#5241,.T.);
#10467=EDGE_CURVE('',#8473,#8471,#7160,.T.);
#10468=EDGE_CURVE('',#8473,#8308,#921,.T.);
#10469=EDGE_CURVE('',#8474,#8473,#301,.T.);
#10470=EDGE_CURVE('',#8309,#8474,#5242,.T.);
#10471=EDGE_CURVE('',#8311,#8475,#922,.T.);
#10472=EDGE_CURVE('',#8310,#8476,#5243,.T.);
#10473=EDGE_CURVE('',#8475,#8476,#302,.T.);
#10474=EDGE_CURVE('',#8476,#8474,#5244,.T.);
#10475=EDGE_CURVE('',#8477,#8475,#7161,.T.);
#10476=EDGE_CURVE('',#8477,#8312,#923,.T.);
#10477=EDGE_CURVE('',#8478,#8477,#303,.T.);
#10478=EDGE_CURVE('',#8313,#8478,#5245,.T.);
#10479=EDGE_CURVE('',#8315,#8479,#924,.T.);
#10480=EDGE_CURVE('',#8314,#8480,#5246,.T.);
#10481=EDGE_CURVE('',#8479,#8480,#304,.T.);
#10482=EDGE_CURVE('',#8480,#8478,#5247,.T.);
#10483=EDGE_CURVE('',#8481,#8479,#7162,.T.);
#10484=EDGE_CURVE('',#8481,#8316,#925,.T.);
#10485=EDGE_CURVE('',#8482,#8481,#305,.T.);
#10486=EDGE_CURVE('',#8317,#8482,#5248,.T.);
#10487=EDGE_CURVE('',#8319,#8483,#926,.T.);
#10488=EDGE_CURVE('',#8318,#8484,#5249,.T.);
#10489=EDGE_CURVE('',#8483,#8484,#306,.T.);
#10490=EDGE_CURVE('',#8484,#8482,#5250,.T.);
#10491=EDGE_CURVE('',#8485,#8483,#7163,.T.);
#10492=EDGE_CURVE('',#8485,#8320,#927,.T.);
#10493=EDGE_CURVE('',#8486,#8485,#307,.T.);
#10494=EDGE_CURVE('',#8321,#8486,#5251,.T.);
#10495=EDGE_CURVE('',#8323,#8487,#928,.T.);
#10496=EDGE_CURVE('',#8322,#8488,#5252,.T.);
#10497=EDGE_CURVE('',#8487,#8488,#308,.T.);
#10498=EDGE_CURVE('',#8488,#8486,#5253,.T.);
#10499=EDGE_CURVE('',#8489,#8487,#7164,.T.);
#10500=EDGE_CURVE('',#8489,#8324,#929,.T.);
#10501=EDGE_CURVE('',#8490,#8489,#309,.T.);
#10502=EDGE_CURVE('',#8325,#8490,#5254,.T.);
#10503=EDGE_CURVE('',#8327,#8491,#930,.T.);
#10504=EDGE_CURVE('',#8326,#8492,#5255,.T.);
#10505=EDGE_CURVE('',#8491,#8492,#310,.T.);
#10506=EDGE_CURVE('',#8492,#8490,#5256,.T.);
#10507=EDGE_CURVE('',#8493,#8491,#7165,.T.);
#10508=EDGE_CURVE('',#8493,#8328,#931,.T.);
#10509=EDGE_CURVE('',#8494,#8493,#311,.T.);
#10510=EDGE_CURVE('',#8329,#8494,#5257,.T.);
#10511=EDGE_CURVE('',#8331,#8495,#932,.T.);
#10512=EDGE_CURVE('',#8330,#8496,#5258,.T.);
#10513=EDGE_CURVE('',#8495,#8496,#312,.T.);
#10514=EDGE_CURVE('',#8496,#8494,#5259,.T.);
#10515=EDGE_CURVE('',#8497,#8495,#7166,.T.);
#10516=EDGE_CURVE('',#8497,#8332,#933,.T.);
#10517=EDGE_CURVE('',#8498,#8497,#313,.T.);
#10518=EDGE_CURVE('',#8333,#8498,#5260,.T.);
#10519=EDGE_CURVE('',#8335,#8499,#934,.T.);
#10520=EDGE_CURVE('',#8334,#8500,#5261,.T.);
#10521=EDGE_CURVE('',#8499,#8500,#314,.T.);
#10522=EDGE_CURVE('',#8500,#8498,#5262,.T.);
#10523=EDGE_CURVE('',#8501,#8499,#7167,.T.);
#10524=EDGE_CURVE('',#8501,#8336,#935,.T.);
#10525=EDGE_CURVE('',#8502,#8501,#315,.T.);
#10526=EDGE_CURVE('',#8337,#8502,#5263,.T.);
#10527=EDGE_CURVE('',#8339,#8503,#936,.T.);
#10528=EDGE_CURVE('',#8338,#8504,#5264,.T.);
#10529=EDGE_CURVE('',#8503,#8504,#316,.T.);
#10530=EDGE_CURVE('',#8504,#8502,#5265,.T.);
#10531=EDGE_CURVE('',#8505,#8503,#7168,.T.);
#10532=EDGE_CURVE('',#8505,#8340,#937,.T.);
#10533=EDGE_CURVE('',#8506,#8505,#317,.T.);
#10534=EDGE_CURVE('',#8341,#8506,#5266,.T.);
#10535=EDGE_CURVE('',#8343,#8507,#938,.T.);
#10536=EDGE_CURVE('',#8342,#8508,#5267,.T.);
#10537=EDGE_CURVE('',#8507,#8508,#318,.T.);
#10538=EDGE_CURVE('',#8508,#8506,#5268,.T.);
#10539=EDGE_CURVE('',#8509,#8507,#7169,.T.);
#10540=EDGE_CURVE('',#8509,#8344,#939,.T.);
#10541=EDGE_CURVE('',#8510,#8509,#319,.T.);
#10542=EDGE_CURVE('',#8345,#8510,#5269,.T.);
#10543=EDGE_CURVE('',#8347,#8511,#940,.T.);
#10544=EDGE_CURVE('',#8346,#8512,#5270,.T.);
#10545=EDGE_CURVE('',#8511,#8512,#320,.T.);
#10546=EDGE_CURVE('',#8512,#8510,#5271,.T.);
#10547=EDGE_CURVE('',#8513,#8511,#7170,.T.);
#10548=EDGE_CURVE('',#8513,#8348,#941,.T.);
#10549=EDGE_CURVE('',#8514,#8513,#321,.T.);
#10550=EDGE_CURVE('',#8349,#8514,#5272,.T.);
#10551=EDGE_CURVE('',#8351,#8515,#942,.T.);
#10552=EDGE_CURVE('',#8350,#8516,#5273,.T.);
#10553=EDGE_CURVE('',#8515,#8516,#322,.T.);
#10554=EDGE_CURVE('',#8516,#8514,#5274,.T.);
#10555=EDGE_CURVE('',#8517,#8515,#7171,.T.);
#10556=EDGE_CURVE('',#8517,#8352,#943,.T.);
#10557=EDGE_CURVE('',#8518,#8517,#323,.T.);
#10558=EDGE_CURVE('',#8353,#8518,#5275,.T.);
#10559=EDGE_CURVE('',#8355,#8519,#944,.T.);
#10560=EDGE_CURVE('',#8354,#8520,#5276,.T.);
#10561=EDGE_CURVE('',#8519,#8520,#324,.T.);
#10562=EDGE_CURVE('',#8520,#8518,#5277,.T.);
#10563=EDGE_CURVE('',#8521,#8519,#7172,.T.);
#10564=EDGE_CURVE('',#8521,#8356,#945,.T.);
#10565=EDGE_CURVE('',#8522,#8521,#325,.T.);
#10566=EDGE_CURVE('',#8357,#8522,#5278,.T.);
#10567=EDGE_CURVE('',#8359,#8523,#946,.T.);
#10568=EDGE_CURVE('',#8358,#8524,#5279,.T.);
#10569=EDGE_CURVE('',#8523,#8524,#326,.T.);
#10570=EDGE_CURVE('',#8524,#8522,#5280,.T.);
#10571=EDGE_CURVE('',#8525,#8523,#7173,.T.);
#10572=EDGE_CURVE('',#8525,#8360,#947,.T.);
#10573=EDGE_CURVE('',#8526,#8525,#327,.T.);
#10574=EDGE_CURVE('',#8361,#8526,#5281,.T.);
#10575=EDGE_CURVE('',#8363,#8527,#948,.T.);
#10576=EDGE_CURVE('',#8362,#8528,#5282,.T.);
#10577=EDGE_CURVE('',#8527,#8528,#328,.T.);
#10578=EDGE_CURVE('',#8528,#8526,#5283,.T.);
#10579=EDGE_CURVE('',#8529,#8527,#7174,.T.);
#10580=EDGE_CURVE('',#8529,#8364,#949,.T.);
#10581=EDGE_CURVE('',#8530,#8529,#329,.T.);
#10582=EDGE_CURVE('',#8365,#8530,#5284,.T.);
#10583=EDGE_CURVE('',#8367,#8531,#950,.T.);
#10584=EDGE_CURVE('',#8366,#8532,#5285,.T.);
#10585=EDGE_CURVE('',#8531,#8532,#330,.T.);
#10586=EDGE_CURVE('',#8532,#8530,#5286,.T.);
#10587=EDGE_CURVE('',#8533,#8531,#7175,.T.);
#10588=EDGE_CURVE('',#8533,#8368,#951,.T.);
#10589=EDGE_CURVE('',#8534,#8533,#331,.T.);
#10590=EDGE_CURVE('',#8369,#8534,#5287,.T.);
#10591=EDGE_CURVE('',#8371,#8535,#952,.T.);
#10592=EDGE_CURVE('',#8370,#8536,#5288,.T.);
#10593=EDGE_CURVE('',#8535,#8536,#332,.T.);
#10594=EDGE_CURVE('',#8536,#8534,#5289,.T.);
#10595=EDGE_CURVE('',#8537,#8535,#7176,.T.);
#10596=EDGE_CURVE('',#8537,#8372,#953,.T.);
#10597=EDGE_CURVE('',#8538,#8537,#333,.T.);
#10598=EDGE_CURVE('',#8373,#8538,#5290,.T.);
#10599=EDGE_CURVE('',#8375,#8539,#954,.T.);
#10600=EDGE_CURVE('',#8374,#8540,#5291,.T.);
#10601=EDGE_CURVE('',#8539,#8540,#334,.T.);
#10602=EDGE_CURVE('',#8540,#8538,#5292,.T.);
#10603=EDGE_CURVE('',#8541,#8539,#7177,.T.);
#10604=EDGE_CURVE('',#8541,#8376,#955,.T.);
#10605=EDGE_CURVE('',#8542,#8541,#335,.T.);
#10606=EDGE_CURVE('',#8377,#8542,#5293,.T.);
#10607=EDGE_CURVE('',#8379,#8543,#956,.T.);
#10608=EDGE_CURVE('',#8378,#8544,#5294,.T.);
#10609=EDGE_CURVE('',#8543,#8544,#336,.T.);
#10610=EDGE_CURVE('',#8544,#8542,#5295,.T.);
#10611=EDGE_CURVE('',#8545,#8543,#7178,.T.);
#10612=EDGE_CURVE('',#8545,#8380,#957,.T.);
#10613=EDGE_CURVE('',#8546,#8545,#337,.T.);
#10614=EDGE_CURVE('',#8381,#8546,#5296,.T.);
#10615=EDGE_CURVE('',#8383,#8547,#958,.T.);
#10616=EDGE_CURVE('',#8382,#8548,#5297,.T.);
#10617=EDGE_CURVE('',#8547,#8548,#338,.T.);
#10618=EDGE_CURVE('',#8548,#8546,#5298,.T.);
#10619=EDGE_CURVE('',#8549,#8547,#7179,.T.);
#10620=EDGE_CURVE('',#8549,#8384,#959,.T.);
#10621=EDGE_CURVE('',#8550,#8549,#339,.T.);
#10622=EDGE_CURVE('',#8385,#8550,#5299,.T.);
#10623=EDGE_CURVE('',#8387,#8551,#960,.T.);
#10624=EDGE_CURVE('',#8386,#8552,#5300,.T.);
#10625=EDGE_CURVE('',#8551,#8552,#340,.T.);
#10626=EDGE_CURVE('',#8552,#8550,#5301,.T.);
#10627=EDGE_CURVE('',#8553,#8551,#7180,.T.);
#10628=EDGE_CURVE('',#8553,#8388,#961,.T.);
#10629=EDGE_CURVE('',#8554,#8553,#341,.T.);
#10630=EDGE_CURVE('',#8389,#8554,#5302,.T.);
#10631=EDGE_CURVE('',#8391,#8555,#962,.T.);
#10632=EDGE_CURVE('',#8390,#8556,#5303,.T.);
#10633=EDGE_CURVE('',#8555,#8556,#342,.T.);
#10634=EDGE_CURVE('',#8556,#8554,#5304,.T.);
#10635=EDGE_CURVE('',#8557,#8555,#7181,.T.);
#10636=EDGE_CURVE('',#8557,#8392,#963,.T.);
#10637=EDGE_CURVE('',#8558,#8557,#343,.T.);
#10638=EDGE_CURVE('',#8393,#8558,#5305,.T.);
#10639=EDGE_CURVE('',#8395,#8559,#964,.T.);
#10640=EDGE_CURVE('',#8394,#8560,#5306,.T.);
#10641=EDGE_CURVE('',#8559,#8560,#344,.T.);
#10642=EDGE_CURVE('',#8560,#8558,#5307,.T.);
#10643=EDGE_CURVE('',#8561,#8559,#7182,.T.);
#10644=EDGE_CURVE('',#8561,#8396,#965,.T.);
#10645=EDGE_CURVE('',#8562,#8561,#345,.T.);
#10646=EDGE_CURVE('',#8397,#8562,#5308,.T.);
#10647=EDGE_CURVE('',#8399,#8563,#966,.T.);
#10648=EDGE_CURVE('',#8398,#8564,#5309,.T.);
#10649=EDGE_CURVE('',#8563,#8564,#346,.T.);
#10650=EDGE_CURVE('',#8564,#8562,#5310,.T.);
#10651=EDGE_CURVE('',#8565,#8563,#7183,.T.);
#10652=EDGE_CURVE('',#8565,#8400,#967,.T.);
#10653=EDGE_CURVE('',#8566,#8565,#347,.T.);
#10654=EDGE_CURVE('',#8401,#8566,#5311,.T.);
#10655=EDGE_CURVE('',#8403,#8567,#968,.T.);
#10656=EDGE_CURVE('',#8402,#8568,#5312,.T.);
#10657=EDGE_CURVE('',#8567,#8568,#348,.T.);
#10658=EDGE_CURVE('',#8568,#8566,#5313,.T.);
#10659=EDGE_CURVE('',#8569,#8567,#7184,.T.);
#10660=EDGE_CURVE('',#8569,#8404,#969,.T.);
#10661=EDGE_CURVE('',#8570,#8569,#349,.T.);
#10662=EDGE_CURVE('',#8405,#8570,#5314,.T.);
#10663=EDGE_CURVE('',#8407,#8571,#970,.T.);
#10664=EDGE_CURVE('',#8406,#8572,#5315,.T.);
#10665=EDGE_CURVE('',#8571,#8572,#350,.T.);
#10666=EDGE_CURVE('',#8572,#8570,#5316,.T.);
#10667=EDGE_CURVE('',#8573,#8571,#7185,.T.);
#10668=EDGE_CURVE('',#8573,#8408,#971,.T.);
#10669=EDGE_CURVE('',#8574,#8573,#351,.T.);
#10670=EDGE_CURVE('',#8409,#8574,#5317,.T.);
#10671=EDGE_CURVE('',#8411,#8575,#972,.T.);
#10672=EDGE_CURVE('',#8410,#8576,#5318,.T.);
#10673=EDGE_CURVE('',#8575,#8576,#352,.T.);
#10674=EDGE_CURVE('',#8576,#8574,#5319,.T.);
#10675=EDGE_CURVE('',#8577,#8575,#7186,.T.);
#10676=EDGE_CURVE('',#8577,#8412,#973,.T.);
#10677=EDGE_CURVE('',#8578,#8577,#353,.T.);
#10678=EDGE_CURVE('',#8413,#8578,#5320,.T.);
#10679=EDGE_CURVE('',#8415,#8579,#974,.T.);
#10680=EDGE_CURVE('',#8414,#8580,#5321,.T.);
#10681=EDGE_CURVE('',#8579,#8580,#354,.T.);
#10682=EDGE_CURVE('',#8580,#8578,#5322,.T.);
#10683=EDGE_CURVE('',#8581,#8579,#7187,.T.);
#10684=EDGE_CURVE('',#8581,#8416,#975,.T.);
#10685=EDGE_CURVE('',#8582,#8581,#355,.T.);
#10686=EDGE_CURVE('',#8417,#8582,#5323,.T.);
#10687=EDGE_CURVE('',#8419,#8583,#976,.T.);
#10688=EDGE_CURVE('',#8418,#8584,#5324,.T.);
#10689=EDGE_CURVE('',#8583,#8584,#356,.T.);
#10690=EDGE_CURVE('',#8584,#8582,#5325,.T.);
#10691=EDGE_CURVE('',#8585,#8583,#7188,.T.);
#10692=EDGE_CURVE('',#8585,#8420,#977,.T.);
#10693=EDGE_CURVE('',#8586,#8585,#357,.T.);
#10694=EDGE_CURVE('',#8421,#8586,#5326,.T.);
#10695=EDGE_CURVE('',#8423,#8587,#978,.T.);
#10696=EDGE_CURVE('',#8422,#8588,#5327,.T.);
#10697=EDGE_CURVE('',#8587,#8588,#358,.T.);
#10698=EDGE_CURVE('',#8588,#8586,#5328,.T.);
#10699=EDGE_CURVE('',#8589,#8587,#7189,.T.);
#10700=EDGE_CURVE('',#8589,#8424,#979,.T.);
#10701=EDGE_CURVE('',#8590,#8589,#359,.T.);
#10702=EDGE_CURVE('',#8425,#8590,#5329,.T.);
#10703=EDGE_CURVE('',#8427,#8591,#980,.T.);
#10704=EDGE_CURVE('',#8426,#8592,#5330,.T.);
#10705=EDGE_CURVE('',#8591,#8592,#360,.T.);
#10706=EDGE_CURVE('',#8592,#8590,#5331,.T.);
#10707=EDGE_CURVE('',#8593,#8591,#7190,.T.);
#10708=EDGE_CURVE('',#8593,#8428,#981,.T.);
#10709=EDGE_CURVE('',#8594,#8593,#361,.T.);
#10710=EDGE_CURVE('',#8429,#8594,#5332,.T.);
#10711=EDGE_CURVE('',#8431,#8595,#982,.T.);
#10712=EDGE_CURVE('',#8430,#8596,#5333,.T.);
#10713=EDGE_CURVE('',#8595,#8596,#362,.T.);
#10714=EDGE_CURVE('',#8596,#8594,#5334,.T.);
#10715=EDGE_CURVE('',#8597,#8595,#7191,.T.);
#10716=EDGE_CURVE('',#8597,#8432,#983,.T.);
#10717=EDGE_CURVE('',#8598,#8597,#363,.T.);
#10718=EDGE_CURVE('',#8433,#8598,#5335,.T.);
#10719=EDGE_CURVE('',#8435,#8599,#984,.T.);
#10720=EDGE_CURVE('',#8434,#8600,#5336,.T.);
#10721=EDGE_CURVE('',#8599,#8600,#364,.T.);
#10722=EDGE_CURVE('',#8600,#8598,#5337,.T.);
#10723=EDGE_CURVE('',#8601,#8599,#7192,.T.);
#10724=EDGE_CURVE('',#8601,#8436,#985,.T.);
#10725=EDGE_CURVE('',#8602,#8601,#365,.T.);
#10726=EDGE_CURVE('',#8437,#8602,#5338,.T.);
#10727=EDGE_CURVE('',#8439,#8603,#986,.T.);
#10728=EDGE_CURVE('',#8438,#8604,#5339,.T.);
#10729=EDGE_CURVE('',#8603,#8604,#366,.T.);
#10730=EDGE_CURVE('',#8604,#8602,#5340,.T.);
#10731=EDGE_CURVE('',#8605,#8603,#7193,.T.);
#10732=EDGE_CURVE('',#8605,#8440,#987,.T.);
#10733=EDGE_CURVE('',#8606,#8605,#367,.T.);
#10734=EDGE_CURVE('',#8441,#8606,#5341,.T.);
#10735=EDGE_CURVE('',#8607,#8606,#5342,.T.);
#10736=EDGE_CURVE('',#8442,#8607,#5343,.T.);
#10737=EDGE_CURVE('',#8443,#8608,#988,.T.);
#10738=EDGE_CURVE('',#8608,#8607,#368,.T.);
#10739=EDGE_CURVE('',#8609,#8608,#7194,.T.);
#10740=EDGE_CURVE('',#8609,#8444,#989,.T.);
#10741=EDGE_CURVE('',#8447,#8610,#990,.T.);
#10742=EDGE_CURVE('',#8446,#8611,#5344,.T.);
#10743=EDGE_CURVE('',#8610,#8611,#369,.T.);
#10744=EDGE_CURVE('',#8612,#8609,#370,.T.);
#10745=EDGE_CURVE('',#8445,#8612,#5345,.T.);
#10746=EDGE_CURVE('',#8611,#8612,#5346,.T.);
#10747=EDGE_CURVE('',#8453,#8610,#7195,.T.);
#14003=ORIENTED_EDGE('',*,*,#10253,.F.);
#14004=ORIENTED_EDGE('',*,*,#10254,.F.);
#14005=ORIENTED_EDGE('',*,*,#10255,.F.);
#14006=ORIENTED_EDGE('',*,*,#10256,.F.);
#14007=ORIENTED_EDGE('',*,*,#10257,.F.);
#14008=ORIENTED_EDGE('',*,*,#10258,.T.);
#14009=ORIENTED_EDGE('',*,*,#10259,.F.);
#14010=ORIENTED_EDGE('',*,*,#10254,.T.);
#14011=ORIENTED_EDGE('',*,*,#10260,.F.);
#14012=ORIENTED_EDGE('',*,*,#10261,.F.);
#14013=ORIENTED_EDGE('',*,*,#10262,.F.);
#14014=ORIENTED_EDGE('',*,*,#10258,.F.);
#14015=ORIENTED_EDGE('',*,*,#10263,.T.);
#14016=ORIENTED_EDGE('',*,*,#10264,.T.);
#14017=ORIENTED_EDGE('',*,*,#10265,.T.);
#14018=ORIENTED_EDGE('',*,*,#10266,.T.);
#14019=ORIENTED_EDGE('',*,*,#10267,.T.);
#14020=ORIENTED_EDGE('',*,*,#10268,.T.);
#14021=ORIENTED_EDGE('',*,*,#10269,.T.);
#14022=ORIENTED_EDGE('',*,*,#10270,.T.);
#14023=ORIENTED_EDGE('',*,*,#10271,.T.);
#14024=ORIENTED_EDGE('',*,*,#10272,.T.);
#14025=ORIENTED_EDGE('',*,*,#10273,.T.);
#14026=ORIENTED_EDGE('',*,*,#10274,.T.);
#14027=ORIENTED_EDGE('',*,*,#10275,.T.);
#14028=ORIENTED_EDGE('',*,*,#10276,.T.);
#14029=ORIENTED_EDGE('',*,*,#10277,.T.);
#14030=ORIENTED_EDGE('',*,*,#10278,.T.);
#14031=ORIENTED_EDGE('',*,*,#10279,.T.);
#14032=ORIENTED_EDGE('',*,*,#10280,.T.);
#14033=ORIENTED_EDGE('',*,*,#10281,.T.);
#14034=ORIENTED_EDGE('',*,*,#10282,.T.);
#14035=ORIENTED_EDGE('',*,*,#10283,.T.);
#14036=ORIENTED_EDGE('',*,*,#10284,.T.);
#14037=ORIENTED_EDGE('',*,*,#10285,.T.);
#14038=ORIENTED_EDGE('',*,*,#10286,.T.);
#14039=ORIENTED_EDGE('',*,*,#10287,.T.);
#14040=ORIENTED_EDGE('',*,*,#10288,.T.);
#14041=ORIENTED_EDGE('',*,*,#10289,.T.);
#14042=ORIENTED_EDGE('',*,*,#10290,.T.);
#14043=ORIENTED_EDGE('',*,*,#10291,.T.);
#14044=ORIENTED_EDGE('',*,*,#10292,.T.);
#14045=ORIENTED_EDGE('',*,*,#10293,.T.);
#14046=ORIENTED_EDGE('',*,*,#10294,.T.);
#14047=ORIENTED_EDGE('',*,*,#10295,.T.);
#14048=ORIENTED_EDGE('',*,*,#10296,.T.);
#14049=ORIENTED_EDGE('',*,*,#10297,.T.);
#14050=ORIENTED_EDGE('',*,*,#10298,.T.);
#14051=ORIENTED_EDGE('',*,*,#10299,.T.);
#14052=ORIENTED_EDGE('',*,*,#10300,.T.);
#14053=ORIENTED_EDGE('',*,*,#10301,.T.);
#14054=ORIENTED_EDGE('',*,*,#10302,.T.);
#14055=ORIENTED_EDGE('',*,*,#10303,.T.);
#14056=ORIENTED_EDGE('',*,*,#10304,.T.);
#14057=ORIENTED_EDGE('',*,*,#10305,.T.);
#14058=ORIENTED_EDGE('',*,*,#10306,.T.);
#14059=ORIENTED_EDGE('',*,*,#10307,.T.);
#14060=ORIENTED_EDGE('',*,*,#10308,.T.);
#14061=ORIENTED_EDGE('',*,*,#10309,.T.);
#14062=ORIENTED_EDGE('',*,*,#10310,.T.);
#14063=ORIENTED_EDGE('',*,*,#10311,.T.);
#14064=ORIENTED_EDGE('',*,*,#10312,.T.);
#14065=ORIENTED_EDGE('',*,*,#10313,.T.);
#14066=ORIENTED_EDGE('',*,*,#10314,.T.);
#14067=ORIENTED_EDGE('',*,*,#10315,.T.);
#14068=ORIENTED_EDGE('',*,*,#10316,.T.);
#14069=ORIENTED_EDGE('',*,*,#10317,.T.);
#14070=ORIENTED_EDGE('',*,*,#10318,.T.);
#14071=ORIENTED_EDGE('',*,*,#10319,.T.);
#14072=ORIENTED_EDGE('',*,*,#10320,.T.);
#14073=ORIENTED_EDGE('',*,*,#10321,.T.);
#14074=ORIENTED_EDGE('',*,*,#10322,.T.);
#14075=ORIENTED_EDGE('',*,*,#10323,.T.);
#14076=ORIENTED_EDGE('',*,*,#10324,.T.);
#14077=ORIENTED_EDGE('',*,*,#10325,.T.);
#14078=ORIENTED_EDGE('',*,*,#10326,.T.);
#14079=ORIENTED_EDGE('',*,*,#10327,.T.);
#14080=ORIENTED_EDGE('',*,*,#10328,.T.);
#14081=ORIENTED_EDGE('',*,*,#10329,.T.);
#14082=ORIENTED_EDGE('',*,*,#10330,.T.);
#14083=ORIENTED_EDGE('',*,*,#10331,.T.);
#14084=ORIENTED_EDGE('',*,*,#10332,.T.);
#14085=ORIENTED_EDGE('',*,*,#10333,.T.);
#14086=ORIENTED_EDGE('',*,*,#10334,.T.);
#14087=ORIENTED_EDGE('',*,*,#10335,.T.);
#14088=ORIENTED_EDGE('',*,*,#10336,.T.);
#14089=ORIENTED_EDGE('',*,*,#10337,.T.);
#14090=ORIENTED_EDGE('',*,*,#10338,.T.);
#14091=ORIENTED_EDGE('',*,*,#10339,.T.);
#14092=ORIENTED_EDGE('',*,*,#10340,.T.);
#14093=ORIENTED_EDGE('',*,*,#10341,.T.);
#14094=ORIENTED_EDGE('',*,*,#10342,.T.);
#14095=ORIENTED_EDGE('',*,*,#10343,.T.);
#14096=ORIENTED_EDGE('',*,*,#10344,.T.);
#14097=ORIENTED_EDGE('',*,*,#10345,.T.);
#14098=ORIENTED_EDGE('',*,*,#10346,.T.);
#14099=ORIENTED_EDGE('',*,*,#10347,.T.);
#14100=ORIENTED_EDGE('',*,*,#10348,.T.);
#14101=ORIENTED_EDGE('',*,*,#10349,.T.);
#14102=ORIENTED_EDGE('',*,*,#10350,.T.);
#14103=ORIENTED_EDGE('',*,*,#10351,.T.);
#14104=ORIENTED_EDGE('',*,*,#10352,.T.);
#14105=ORIENTED_EDGE('',*,*,#10353,.T.);
#14106=ORIENTED_EDGE('',*,*,#10354,.T.);
#14107=ORIENTED_EDGE('',*,*,#10355,.T.);
#14108=ORIENTED_EDGE('',*,*,#10356,.T.);
#14109=ORIENTED_EDGE('',*,*,#10357,.T.);
#14110=ORIENTED_EDGE('',*,*,#10358,.T.);
#14111=ORIENTED_EDGE('',*,*,#10359,.T.);
#14112=ORIENTED_EDGE('',*,*,#10360,.T.);
#14113=ORIENTED_EDGE('',*,*,#10361,.T.);
#14114=ORIENTED_EDGE('',*,*,#10362,.T.);
#14115=ORIENTED_EDGE('',*,*,#10363,.T.);
#14116=ORIENTED_EDGE('',*,*,#10364,.T.);
#14117=ORIENTED_EDGE('',*,*,#10365,.T.);
#14118=ORIENTED_EDGE('',*,*,#10366,.T.);
#14119=ORIENTED_EDGE('',*,*,#10367,.T.);
#14120=ORIENTED_EDGE('',*,*,#10368,.T.);
#14121=ORIENTED_EDGE('',*,*,#10369,.T.);
#14122=ORIENTED_EDGE('',*,*,#10370,.T.);
#14123=ORIENTED_EDGE('',*,*,#10371,.T.);
#14124=ORIENTED_EDGE('',*,*,#10372,.T.);
#14125=ORIENTED_EDGE('',*,*,#10373,.T.);
#14126=ORIENTED_EDGE('',*,*,#10374,.T.);
#14127=ORIENTED_EDGE('',*,*,#10375,.T.);
#14128=ORIENTED_EDGE('',*,*,#10376,.T.);
#14129=ORIENTED_EDGE('',*,*,#10377,.T.);
#14130=ORIENTED_EDGE('',*,*,#10378,.T.);
#14131=ORIENTED_EDGE('',*,*,#10379,.T.);
#14132=ORIENTED_EDGE('',*,*,#10380,.T.);
#14133=ORIENTED_EDGE('',*,*,#10381,.T.);
#14134=ORIENTED_EDGE('',*,*,#10382,.T.);
#14135=ORIENTED_EDGE('',*,*,#10383,.T.);
#14136=ORIENTED_EDGE('',*,*,#10384,.T.);
#14137=ORIENTED_EDGE('',*,*,#10385,.T.);
#14138=ORIENTED_EDGE('',*,*,#10386,.T.);
#14139=ORIENTED_EDGE('',*,*,#10387,.T.);
#14140=ORIENTED_EDGE('',*,*,#10388,.T.);
#14141=ORIENTED_EDGE('',*,*,#10389,.T.);
#14142=ORIENTED_EDGE('',*,*,#10390,.T.);
#14143=ORIENTED_EDGE('',*,*,#10391,.T.);
#14144=ORIENTED_EDGE('',*,*,#10392,.T.);
#14145=ORIENTED_EDGE('',*,*,#10393,.T.);
#14146=ORIENTED_EDGE('',*,*,#10394,.T.);
#14147=ORIENTED_EDGE('',*,*,#10395,.T.);
#14148=ORIENTED_EDGE('',*,*,#10396,.T.);
#14149=ORIENTED_EDGE('',*,*,#10397,.T.);
#14150=ORIENTED_EDGE('',*,*,#10398,.T.);
#14151=ORIENTED_EDGE('',*,*,#10399,.T.);
#14152=ORIENTED_EDGE('',*,*,#10400,.T.);
#14153=ORIENTED_EDGE('',*,*,#10401,.T.);
#14154=ORIENTED_EDGE('',*,*,#10402,.T.);
#14155=ORIENTED_EDGE('',*,*,#10403,.T.);
#14156=ORIENTED_EDGE('',*,*,#10404,.T.);
#14157=ORIENTED_EDGE('',*,*,#10405,.T.);
#14158=ORIENTED_EDGE('',*,*,#10406,.T.);
#14159=ORIENTED_EDGE('',*,*,#10407,.T.);
#14160=ORIENTED_EDGE('',*,*,#10408,.T.);
#14161=ORIENTED_EDGE('',*,*,#10409,.T.);
#14162=ORIENTED_EDGE('',*,*,#10410,.T.);
#14163=ORIENTED_EDGE('',*,*,#10411,.T.);
#14164=ORIENTED_EDGE('',*,*,#10412,.T.);
#14165=ORIENTED_EDGE('',*,*,#10413,.T.);
#14166=ORIENTED_EDGE('',*,*,#10414,.T.);
#14167=ORIENTED_EDGE('',*,*,#10415,.T.);
#14168=ORIENTED_EDGE('',*,*,#10416,.T.);
#14169=ORIENTED_EDGE('',*,*,#10417,.T.);
#14170=ORIENTED_EDGE('',*,*,#10418,.T.);
#14171=ORIENTED_EDGE('',*,*,#10419,.T.);
#14172=ORIENTED_EDGE('',*,*,#10420,.T.);
#14173=ORIENTED_EDGE('',*,*,#10421,.T.);
#14174=ORIENTED_EDGE('',*,*,#10422,.T.);
#14175=ORIENTED_EDGE('',*,*,#10255,.T.);
#14176=ORIENTED_EDGE('',*,*,#10259,.T.);
#14177=ORIENTED_EDGE('',*,*,#10262,.T.);
#14178=ORIENTED_EDGE('',*,*,#10423,.T.);
#14179=ORIENTED_EDGE('',*,*,#10256,.T.);
#14180=ORIENTED_EDGE('',*,*,#10423,.F.);
#14181=ORIENTED_EDGE('',*,*,#10261,.T.);
#14182=ORIENTED_EDGE('',*,*,#10424,.F.);
#14183=ORIENTED_EDGE('',*,*,#10425,.F.);
#14184=ORIENTED_EDGE('',*,*,#10426,.T.);
#14185=ORIENTED_EDGE('',*,*,#10427,.F.);
#14186=ORIENTED_EDGE('',*,*,#10426,.F.);
#14187=ORIENTED_EDGE('',*,*,#10425,.T.);
#14188=ORIENTED_EDGE('',*,*,#10253,.T.);
#14189=ORIENTED_EDGE('',*,*,#10424,.T.);
#14190=ORIENTED_EDGE('',*,*,#10260,.T.);
#14191=ORIENTED_EDGE('',*,*,#10257,.T.);
#14192=ORIENTED_EDGE('',*,*,#10428,.F.);
#14193=ORIENTED_EDGE('',*,*,#10429,.F.);
#14194=ORIENTED_EDGE('',*,*,#10430,.F.);
#14195=ORIENTED_EDGE('',*,*,#10420,.F.);
#14196=ORIENTED_EDGE('',*,*,#10431,.F.);
#14197=ORIENTED_EDGE('',*,*,#10422,.F.);
#14198=ORIENTED_EDGE('',*,*,#10432,.T.);
#14199=ORIENTED_EDGE('',*,*,#10433,.F.);
#14200=ORIENTED_EDGE('',*,*,#10430,.T.);
#14201=ORIENTED_EDGE('',*,*,#10434,.F.);
#14202=ORIENTED_EDGE('',*,*,#10432,.F.);
#14203=ORIENTED_EDGE('',*,*,#10421,.F.);
#14204=ORIENTED_EDGE('',*,*,#10431,.T.);
#14205=ORIENTED_EDGE('',*,*,#10435,.F.);
#14206=ORIENTED_EDGE('',*,*,#10436,.T.);
#14207=ORIENTED_EDGE('',*,*,#10263,.F.);
#14208=ORIENTED_EDGE('',*,*,#10436,.F.);
#14209=ORIENTED_EDGE('',*,*,#10437,.F.);
#14210=ORIENTED_EDGE('',*,*,#10438,.F.);
#14211=ORIENTED_EDGE('',*,*,#10264,.F.);
#14212=ORIENTED_EDGE('',*,*,#10439,.F.);
#14213=ORIENTED_EDGE('',*,*,#10266,.F.);
#14214=ORIENTED_EDGE('',*,*,#10440,.T.);
#14215=ORIENTED_EDGE('',*,*,#10441,.F.);
#14216=ORIENTED_EDGE('',*,*,#10438,.T.);
#14217=ORIENTED_EDGE('',*,*,#10442,.F.);
#14218=ORIENTED_EDGE('',*,*,#10440,.F.);
#14219=ORIENTED_EDGE('',*,*,#10265,.F.);
#14220=ORIENTED_EDGE('',*,*,#10439,.T.);
#14221=ORIENTED_EDGE('',*,*,#10443,.F.);
#14222=ORIENTED_EDGE('',*,*,#10444,.T.);
#14223=ORIENTED_EDGE('',*,*,#10267,.F.);
#14224=ORIENTED_EDGE('',*,*,#10444,.F.);
#14225=ORIENTED_EDGE('',*,*,#10445,.F.);
#14226=ORIENTED_EDGE('',*,*,#10446,.F.);
#14227=ORIENTED_EDGE('',*,*,#10268,.F.);
#14228=ORIENTED_EDGE('',*,*,#10447,.F.);
#14229=ORIENTED_EDGE('',*,*,#10270,.F.);
#14230=ORIENTED_EDGE('',*,*,#10448,.T.);
#14231=ORIENTED_EDGE('',*,*,#10449,.F.);
#14232=ORIENTED_EDGE('',*,*,#10446,.T.);
#14233=ORIENTED_EDGE('',*,*,#10450,.F.);
#14234=ORIENTED_EDGE('',*,*,#10448,.F.);
#14235=ORIENTED_EDGE('',*,*,#10269,.F.);
#14236=ORIENTED_EDGE('',*,*,#10447,.T.);
#14237=ORIENTED_EDGE('',*,*,#10451,.F.);
#14238=ORIENTED_EDGE('',*,*,#10452,.T.);
#14239=ORIENTED_EDGE('',*,*,#10271,.F.);
#14240=ORIENTED_EDGE('',*,*,#10452,.F.);
#14241=ORIENTED_EDGE('',*,*,#10453,.F.);
#14242=ORIENTED_EDGE('',*,*,#10454,.F.);
#14243=ORIENTED_EDGE('',*,*,#10272,.F.);
#14244=ORIENTED_EDGE('',*,*,#10455,.F.);
#14245=ORIENTED_EDGE('',*,*,#10274,.F.);
#14246=ORIENTED_EDGE('',*,*,#10456,.T.);
#14247=ORIENTED_EDGE('',*,*,#10457,.F.);
#14248=ORIENTED_EDGE('',*,*,#10454,.T.);
#14249=ORIENTED_EDGE('',*,*,#10458,.F.);
#14250=ORIENTED_EDGE('',*,*,#10456,.F.);
#14251=ORIENTED_EDGE('',*,*,#10273,.F.);
#14252=ORIENTED_EDGE('',*,*,#10455,.T.);
#14253=ORIENTED_EDGE('',*,*,#10459,.F.);
#14254=ORIENTED_EDGE('',*,*,#10460,.T.);
#14255=ORIENTED_EDGE('',*,*,#10275,.F.);
#14256=ORIENTED_EDGE('',*,*,#10460,.F.);
#14257=ORIENTED_EDGE('',*,*,#10461,.F.);
#14258=ORIENTED_EDGE('',*,*,#10462,.F.);
#14259=ORIENTED_EDGE('',*,*,#10276,.F.);
#14260=ORIENTED_EDGE('',*,*,#10463,.F.);
#14261=ORIENTED_EDGE('',*,*,#10278,.F.);
#14262=ORIENTED_EDGE('',*,*,#10464,.T.);
#14263=ORIENTED_EDGE('',*,*,#10465,.F.);
#14264=ORIENTED_EDGE('',*,*,#10462,.T.);
#14265=ORIENTED_EDGE('',*,*,#10466,.F.);
#14266=ORIENTED_EDGE('',*,*,#10464,.F.);
#14267=ORIENTED_EDGE('',*,*,#10277,.F.);
#14268=ORIENTED_EDGE('',*,*,#10463,.T.);
#14269=ORIENTED_EDGE('',*,*,#10467,.F.);
#14270=ORIENTED_EDGE('',*,*,#10468,.T.);
#14271=ORIENTED_EDGE('',*,*,#10279,.F.);
#14272=ORIENTED_EDGE('',*,*,#10468,.F.);
#14273=ORIENTED_EDGE('',*,*,#10469,.F.);
#14274=ORIENTED_EDGE('',*,*,#10470,.F.);
#14275=ORIENTED_EDGE('',*,*,#10280,.F.);
#14276=ORIENTED_EDGE('',*,*,#10471,.F.);
#14277=ORIENTED_EDGE('',*,*,#10282,.F.);
#14278=ORIENTED_EDGE('',*,*,#10472,.T.);
#14279=ORIENTED_EDGE('',*,*,#10473,.F.);
#14280=ORIENTED_EDGE('',*,*,#10470,.T.);
#14281=ORIENTED_EDGE('',*,*,#10474,.F.);
#14282=ORIENTED_EDGE('',*,*,#10472,.F.);
#14283=ORIENTED_EDGE('',*,*,#10281,.F.);
#14284=ORIENTED_EDGE('',*,*,#10471,.T.);
#14285=ORIENTED_EDGE('',*,*,#10475,.F.);
#14286=ORIENTED_EDGE('',*,*,#10476,.T.);
#14287=ORIENTED_EDGE('',*,*,#10283,.F.);
#14288=ORIENTED_EDGE('',*,*,#10476,.F.);
#14289=ORIENTED_EDGE('',*,*,#10477,.F.);
#14290=ORIENTED_EDGE('',*,*,#10478,.F.);
#14291=ORIENTED_EDGE('',*,*,#10284,.F.);
#14292=ORIENTED_EDGE('',*,*,#10479,.F.);
#14293=ORIENTED_EDGE('',*,*,#10286,.F.);
#14294=ORIENTED_EDGE('',*,*,#10480,.T.);
#14295=ORIENTED_EDGE('',*,*,#10481,.F.);
#14296=ORIENTED_EDGE('',*,*,#10478,.T.);
#14297=ORIENTED_EDGE('',*,*,#10482,.F.);
#14298=ORIENTED_EDGE('',*,*,#10480,.F.);
#14299=ORIENTED_EDGE('',*,*,#10285,.F.);
#14300=ORIENTED_EDGE('',*,*,#10479,.T.);
#14301=ORIENTED_EDGE('',*,*,#10483,.F.);
#14302=ORIENTED_EDGE('',*,*,#10484,.T.);
#14303=ORIENTED_EDGE('',*,*,#10287,.F.);
#14304=ORIENTED_EDGE('',*,*,#10484,.F.);
#14305=ORIENTED_EDGE('',*,*,#10485,.F.);
#14306=ORIENTED_EDGE('',*,*,#10486,.F.);
#14307=ORIENTED_EDGE('',*,*,#10288,.F.);
#14308=ORIENTED_EDGE('',*,*,#10487,.F.);
#14309=ORIENTED_EDGE('',*,*,#10290,.F.);
#14310=ORIENTED_EDGE('',*,*,#10488,.T.);
#14311=ORIENTED_EDGE('',*,*,#10489,.F.);
#14312=ORIENTED_EDGE('',*,*,#10486,.T.);
#14313=ORIENTED_EDGE('',*,*,#10490,.F.);
#14314=ORIENTED_EDGE('',*,*,#10488,.F.);
#14315=ORIENTED_EDGE('',*,*,#10289,.F.);
#14316=ORIENTED_EDGE('',*,*,#10487,.T.);
#14317=ORIENTED_EDGE('',*,*,#10491,.F.);
#14318=ORIENTED_EDGE('',*,*,#10492,.T.);
#14319=ORIENTED_EDGE('',*,*,#10291,.F.);
#14320=ORIENTED_EDGE('',*,*,#10492,.F.);
#14321=ORIENTED_EDGE('',*,*,#10493,.F.);
#14322=ORIENTED_EDGE('',*,*,#10494,.F.);
#14323=ORIENTED_EDGE('',*,*,#10292,.F.);
#14324=ORIENTED_EDGE('',*,*,#10495,.F.);
#14325=ORIENTED_EDGE('',*,*,#10294,.F.);
#14326=ORIENTED_EDGE('',*,*,#10496,.T.);
#14327=ORIENTED_EDGE('',*,*,#10497,.F.);
#14328=ORIENTED_EDGE('',*,*,#10494,.T.);
#14329=ORIENTED_EDGE('',*,*,#10498,.F.);
#14330=ORIENTED_EDGE('',*,*,#10496,.F.);
#14331=ORIENTED_EDGE('',*,*,#10293,.F.);
#14332=ORIENTED_EDGE('',*,*,#10495,.T.);
#14333=ORIENTED_EDGE('',*,*,#10499,.F.);
#14334=ORIENTED_EDGE('',*,*,#10500,.T.);
#14335=ORIENTED_EDGE('',*,*,#10295,.F.);
#14336=ORIENTED_EDGE('',*,*,#10500,.F.);
#14337=ORIENTED_EDGE('',*,*,#10501,.F.);
#14338=ORIENTED_EDGE('',*,*,#10502,.F.);
#14339=ORIENTED_EDGE('',*,*,#10296,.F.);
#14340=ORIENTED_EDGE('',*,*,#10503,.F.);
#14341=ORIENTED_EDGE('',*,*,#10298,.F.);
#14342=ORIENTED_EDGE('',*,*,#10504,.T.);
#14343=ORIENTED_EDGE('',*,*,#10505,.F.);
#14344=ORIENTED_EDGE('',*,*,#10502,.T.);
#14345=ORIENTED_EDGE('',*,*,#10506,.F.);
#14346=ORIENTED_EDGE('',*,*,#10504,.F.);
#14347=ORIENTED_EDGE('',*,*,#10297,.F.);
#14348=ORIENTED_EDGE('',*,*,#10503,.T.);
#14349=ORIENTED_EDGE('',*,*,#10507,.F.);
#14350=ORIENTED_EDGE('',*,*,#10508,.T.);
#14351=ORIENTED_EDGE('',*,*,#10299,.F.);
#14352=ORIENTED_EDGE('',*,*,#10508,.F.);
#14353=ORIENTED_EDGE('',*,*,#10509,.F.);
#14354=ORIENTED_EDGE('',*,*,#10510,.F.);
#14355=ORIENTED_EDGE('',*,*,#10300,.F.);
#14356=ORIENTED_EDGE('',*,*,#10511,.F.);
#14357=ORIENTED_EDGE('',*,*,#10302,.F.);
#14358=ORIENTED_EDGE('',*,*,#10512,.T.);
#14359=ORIENTED_EDGE('',*,*,#10513,.F.);
#14360=ORIENTED_EDGE('',*,*,#10510,.T.);
#14361=ORIENTED_EDGE('',*,*,#10514,.F.);
#14362=ORIENTED_EDGE('',*,*,#10512,.F.);
#14363=ORIENTED_EDGE('',*,*,#10301,.F.);
#14364=ORIENTED_EDGE('',*,*,#10511,.T.);
#14365=ORIENTED_EDGE('',*,*,#10515,.F.);
#14366=ORIENTED_EDGE('',*,*,#10516,.T.);
#14367=ORIENTED_EDGE('',*,*,#10303,.F.);
#14368=ORIENTED_EDGE('',*,*,#10516,.F.);
#14369=ORIENTED_EDGE('',*,*,#10517,.F.);
#14370=ORIENTED_EDGE('',*,*,#10518,.F.);
#14371=ORIENTED_EDGE('',*,*,#10304,.F.);
#14372=ORIENTED_EDGE('',*,*,#10519,.F.);
#14373=ORIENTED_EDGE('',*,*,#10306,.F.);
#14374=ORIENTED_EDGE('',*,*,#10520,.T.);
#14375=ORIENTED_EDGE('',*,*,#10521,.F.);
#14376=ORIENTED_EDGE('',*,*,#10518,.T.);
#14377=ORIENTED_EDGE('',*,*,#10522,.F.);
#14378=ORIENTED_EDGE('',*,*,#10520,.F.);
#14379=ORIENTED_EDGE('',*,*,#10305,.F.);
#14380=ORIENTED_EDGE('',*,*,#10519,.T.);
#14381=ORIENTED_EDGE('',*,*,#10523,.F.);
#14382=ORIENTED_EDGE('',*,*,#10524,.T.);
#14383=ORIENTED_EDGE('',*,*,#10307,.F.);
#14384=ORIENTED_EDGE('',*,*,#10524,.F.);
#14385=ORIENTED_EDGE('',*,*,#10525,.F.);
#14386=ORIENTED_EDGE('',*,*,#10526,.F.);
#14387=ORIENTED_EDGE('',*,*,#10308,.F.);
#14388=ORIENTED_EDGE('',*,*,#10527,.F.);
#14389=ORIENTED_EDGE('',*,*,#10310,.F.);
#14390=ORIENTED_EDGE('',*,*,#10528,.T.);
#14391=ORIENTED_EDGE('',*,*,#10529,.F.);
#14392=ORIENTED_EDGE('',*,*,#10526,.T.);
#14393=ORIENTED_EDGE('',*,*,#10530,.F.);
#14394=ORIENTED_EDGE('',*,*,#10528,.F.);
#14395=ORIENTED_EDGE('',*,*,#10309,.F.);
#14396=ORIENTED_EDGE('',*,*,#10527,.T.);
#14397=ORIENTED_EDGE('',*,*,#10531,.F.);
#14398=ORIENTED_EDGE('',*,*,#10532,.T.);
#14399=ORIENTED_EDGE('',*,*,#10311,.F.);
#14400=ORIENTED_EDGE('',*,*,#10532,.F.);
#14401=ORIENTED_EDGE('',*,*,#10533,.F.);
#14402=ORIENTED_EDGE('',*,*,#10534,.F.);
#14403=ORIENTED_EDGE('',*,*,#10312,.F.);
#14404=ORIENTED_EDGE('',*,*,#10535,.F.);
#14405=ORIENTED_EDGE('',*,*,#10314,.F.);
#14406=ORIENTED_EDGE('',*,*,#10536,.T.);
#14407=ORIENTED_EDGE('',*,*,#10537,.F.);
#14408=ORIENTED_EDGE('',*,*,#10534,.T.);
#14409=ORIENTED_EDGE('',*,*,#10538,.F.);
#14410=ORIENTED_EDGE('',*,*,#10536,.F.);
#14411=ORIENTED_EDGE('',*,*,#10313,.F.);
#14412=ORIENTED_EDGE('',*,*,#10535,.T.);
#14413=ORIENTED_EDGE('',*,*,#10539,.F.);
#14414=ORIENTED_EDGE('',*,*,#10540,.T.);
#14415=ORIENTED_EDGE('',*,*,#10315,.F.);
#14416=ORIENTED_EDGE('',*,*,#10540,.F.);
#14417=ORIENTED_EDGE('',*,*,#10541,.F.);
#14418=ORIENTED_EDGE('',*,*,#10542,.F.);
#14419=ORIENTED_EDGE('',*,*,#10316,.F.);
#14420=ORIENTED_EDGE('',*,*,#10543,.F.);
#14421=ORIENTED_EDGE('',*,*,#10318,.F.);
#14422=ORIENTED_EDGE('',*,*,#10544,.T.);
#14423=ORIENTED_EDGE('',*,*,#10545,.F.);
#14424=ORIENTED_EDGE('',*,*,#10542,.T.);
#14425=ORIENTED_EDGE('',*,*,#10546,.F.);
#14426=ORIENTED_EDGE('',*,*,#10544,.F.);
#14427=ORIENTED_EDGE('',*,*,#10317,.F.);
#14428=ORIENTED_EDGE('',*,*,#10543,.T.);
#14429=ORIENTED_EDGE('',*,*,#10547,.F.);
#14430=ORIENTED_EDGE('',*,*,#10548,.T.);
#14431=ORIENTED_EDGE('',*,*,#10319,.F.);
#14432=ORIENTED_EDGE('',*,*,#10548,.F.);
#14433=ORIENTED_EDGE('',*,*,#10549,.F.);
#14434=ORIENTED_EDGE('',*,*,#10550,.F.);
#14435=ORIENTED_EDGE('',*,*,#10320,.F.);
#14436=ORIENTED_EDGE('',*,*,#10551,.F.);
#14437=ORIENTED_EDGE('',*,*,#10322,.F.);
#14438=ORIENTED_EDGE('',*,*,#10552,.T.);
#14439=ORIENTED_EDGE('',*,*,#10553,.F.);
#14440=ORIENTED_EDGE('',*,*,#10550,.T.);
#14441=ORIENTED_EDGE('',*,*,#10554,.F.);
#14442=ORIENTED_EDGE('',*,*,#10552,.F.);
#14443=ORIENTED_EDGE('',*,*,#10321,.F.);
#14444=ORIENTED_EDGE('',*,*,#10551,.T.);
#14445=ORIENTED_EDGE('',*,*,#10555,.F.);
#14446=ORIENTED_EDGE('',*,*,#10556,.T.);
#14447=ORIENTED_EDGE('',*,*,#10323,.F.);
#14448=ORIENTED_EDGE('',*,*,#10556,.F.);
#14449=ORIENTED_EDGE('',*,*,#10557,.F.);
#14450=ORIENTED_EDGE('',*,*,#10558,.F.);
#14451=ORIENTED_EDGE('',*,*,#10324,.F.);
#14452=ORIENTED_EDGE('',*,*,#10559,.F.);
#14453=ORIENTED_EDGE('',*,*,#10326,.F.);
#14454=ORIENTED_EDGE('',*,*,#10560,.T.);
#14455=ORIENTED_EDGE('',*,*,#10561,.F.);
#14456=ORIENTED_EDGE('',*,*,#10558,.T.);
#14457=ORIENTED_EDGE('',*,*,#10562,.F.);
#14458=ORIENTED_EDGE('',*,*,#10560,.F.);
#14459=ORIENTED_EDGE('',*,*,#10325,.F.);
#14460=ORIENTED_EDGE('',*,*,#10559,.T.);
#14461=ORIENTED_EDGE('',*,*,#10563,.F.);
#14462=ORIENTED_EDGE('',*,*,#10564,.T.);
#14463=ORIENTED_EDGE('',*,*,#10327,.F.);
#14464=ORIENTED_EDGE('',*,*,#10564,.F.);
#14465=ORIENTED_EDGE('',*,*,#10565,.F.);
#14466=ORIENTED_EDGE('',*,*,#10566,.F.);
#14467=ORIENTED_EDGE('',*,*,#10328,.F.);
#14468=ORIENTED_EDGE('',*,*,#10567,.F.);
#14469=ORIENTED_EDGE('',*,*,#10330,.F.);
#14470=ORIENTED_EDGE('',*,*,#10568,.T.);
#14471=ORIENTED_EDGE('',*,*,#10569,.F.);
#14472=ORIENTED_EDGE('',*,*,#10566,.T.);
#14473=ORIENTED_EDGE('',*,*,#10570,.F.);
#14474=ORIENTED_EDGE('',*,*,#10568,.F.);
#14475=ORIENTED_EDGE('',*,*,#10329,.F.);
#14476=ORIENTED_EDGE('',*,*,#10567,.T.);
#14477=ORIENTED_EDGE('',*,*,#10571,.F.);
#14478=ORIENTED_EDGE('',*,*,#10572,.T.);
#14479=ORIENTED_EDGE('',*,*,#10331,.F.);
#14480=ORIENTED_EDGE('',*,*,#10572,.F.);
#14481=ORIENTED_EDGE('',*,*,#10573,.F.);
#14482=ORIENTED_EDGE('',*,*,#10574,.F.);
#14483=ORIENTED_EDGE('',*,*,#10332,.F.);
#14484=ORIENTED_EDGE('',*,*,#10575,.F.);
#14485=ORIENTED_EDGE('',*,*,#10334,.F.);
#14486=ORIENTED_EDGE('',*,*,#10576,.T.);
#14487=ORIENTED_EDGE('',*,*,#10577,.F.);
#14488=ORIENTED_EDGE('',*,*,#10574,.T.);
#14489=ORIENTED_EDGE('',*,*,#10578,.F.);
#14490=ORIENTED_EDGE('',*,*,#10576,.F.);
#14491=ORIENTED_EDGE('',*,*,#10333,.F.);
#14492=ORIENTED_EDGE('',*,*,#10575,.T.);
#14493=ORIENTED_EDGE('',*,*,#10579,.F.);
#14494=ORIENTED_EDGE('',*,*,#10580,.T.);
#14495=ORIENTED_EDGE('',*,*,#10335,.F.);
#14496=ORIENTED_EDGE('',*,*,#10580,.F.);
#14497=ORIENTED_EDGE('',*,*,#10581,.F.);
#14498=ORIENTED_EDGE('',*,*,#10582,.F.);
#14499=ORIENTED_EDGE('',*,*,#10336,.F.);
#14500=ORIENTED_EDGE('',*,*,#10583,.F.);
#14501=ORIENTED_EDGE('',*,*,#10338,.F.);
#14502=ORIENTED_EDGE('',*,*,#10584,.T.);
#14503=ORIENTED_EDGE('',*,*,#10585,.F.);
#14504=ORIENTED_EDGE('',*,*,#10582,.T.);
#14505=ORIENTED_EDGE('',*,*,#10586,.F.);
#14506=ORIENTED_EDGE('',*,*,#10584,.F.);
#14507=ORIENTED_EDGE('',*,*,#10337,.F.);
#14508=ORIENTED_EDGE('',*,*,#10583,.T.);
#14509=ORIENTED_EDGE('',*,*,#10587,.F.);
#14510=ORIENTED_EDGE('',*,*,#10588,.T.);
#14511=ORIENTED_EDGE('',*,*,#10339,.F.);
#14512=ORIENTED_EDGE('',*,*,#10588,.F.);
#14513=ORIENTED_EDGE('',*,*,#10589,.F.);
#14514=ORIENTED_EDGE('',*,*,#10590,.F.);
#14515=ORIENTED_EDGE('',*,*,#10340,.F.);
#14516=ORIENTED_EDGE('',*,*,#10591,.F.);
#14517=ORIENTED_EDGE('',*,*,#10342,.F.);
#14518=ORIENTED_EDGE('',*,*,#10592,.T.);
#14519=ORIENTED_EDGE('',*,*,#10593,.F.);
#14520=ORIENTED_EDGE('',*,*,#10590,.T.);
#14521=ORIENTED_EDGE('',*,*,#10594,.F.);
#14522=ORIENTED_EDGE('',*,*,#10592,.F.);
#14523=ORIENTED_EDGE('',*,*,#10341,.F.);
#14524=ORIENTED_EDGE('',*,*,#10591,.T.);
#14525=ORIENTED_EDGE('',*,*,#10595,.F.);
#14526=ORIENTED_EDGE('',*,*,#10596,.T.);
#14527=ORIENTED_EDGE('',*,*,#10343,.F.);
#14528=ORIENTED_EDGE('',*,*,#10596,.F.);
#14529=ORIENTED_EDGE('',*,*,#10597,.F.);
#14530=ORIENTED_EDGE('',*,*,#10598,.F.);
#14531=ORIENTED_EDGE('',*,*,#10344,.F.);
#14532=ORIENTED_EDGE('',*,*,#10599,.F.);
#14533=ORIENTED_EDGE('',*,*,#10346,.F.);
#14534=ORIENTED_EDGE('',*,*,#10600,.T.);
#14535=ORIENTED_EDGE('',*,*,#10601,.F.);
#14536=ORIENTED_EDGE('',*,*,#10598,.T.);
#14537=ORIENTED_EDGE('',*,*,#10602,.F.);
#14538=ORIENTED_EDGE('',*,*,#10600,.F.);
#14539=ORIENTED_EDGE('',*,*,#10345,.F.);
#14540=ORIENTED_EDGE('',*,*,#10599,.T.);
#14541=ORIENTED_EDGE('',*,*,#10603,.F.);
#14542=ORIENTED_EDGE('',*,*,#10604,.T.);
#14543=ORIENTED_EDGE('',*,*,#10347,.F.);
#14544=ORIENTED_EDGE('',*,*,#10604,.F.);
#14545=ORIENTED_EDGE('',*,*,#10605,.F.);
#14546=ORIENTED_EDGE('',*,*,#10606,.F.);
#14547=ORIENTED_EDGE('',*,*,#10348,.F.);
#14548=ORIENTED_EDGE('',*,*,#10607,.F.);
#14549=ORIENTED_EDGE('',*,*,#10350,.F.);
#14550=ORIENTED_EDGE('',*,*,#10608,.T.);
#14551=ORIENTED_EDGE('',*,*,#10609,.F.);
#14552=ORIENTED_EDGE('',*,*,#10606,.T.);
#14553=ORIENTED_EDGE('',*,*,#10610,.F.);
#14554=ORIENTED_EDGE('',*,*,#10608,.F.);
#14555=ORIENTED_EDGE('',*,*,#10349,.F.);
#14556=ORIENTED_EDGE('',*,*,#10607,.T.);
#14557=ORIENTED_EDGE('',*,*,#10611,.F.);
#14558=ORIENTED_EDGE('',*,*,#10612,.T.);
#14559=ORIENTED_EDGE('',*,*,#10351,.F.);
#14560=ORIENTED_EDGE('',*,*,#10612,.F.);
#14561=ORIENTED_EDGE('',*,*,#10613,.F.);
#14562=ORIENTED_EDGE('',*,*,#10614,.F.);
#14563=ORIENTED_EDGE('',*,*,#10352,.F.);
#14564=ORIENTED_EDGE('',*,*,#10615,.F.);
#14565=ORIENTED_EDGE('',*,*,#10354,.F.);
#14566=ORIENTED_EDGE('',*,*,#10616,.T.);
#14567=ORIENTED_EDGE('',*,*,#10617,.F.);
#14568=ORIENTED_EDGE('',*,*,#10614,.T.);
#14569=ORIENTED_EDGE('',*,*,#10618,.F.);
#14570=ORIENTED_EDGE('',*,*,#10616,.F.);
#14571=ORIENTED_EDGE('',*,*,#10353,.F.);
#14572=ORIENTED_EDGE('',*,*,#10615,.T.);
#14573=ORIENTED_EDGE('',*,*,#10619,.F.);
#14574=ORIENTED_EDGE('',*,*,#10620,.T.);
#14575=ORIENTED_EDGE('',*,*,#10355,.F.);
#14576=ORIENTED_EDGE('',*,*,#10620,.F.);
#14577=ORIENTED_EDGE('',*,*,#10621,.F.);
#14578=ORIENTED_EDGE('',*,*,#10622,.F.);
#14579=ORIENTED_EDGE('',*,*,#10356,.F.);
#14580=ORIENTED_EDGE('',*,*,#10623,.F.);
#14581=ORIENTED_EDGE('',*,*,#10358,.F.);
#14582=ORIENTED_EDGE('',*,*,#10624,.T.);
#14583=ORIENTED_EDGE('',*,*,#10625,.F.);
#14584=ORIENTED_EDGE('',*,*,#10622,.T.);
#14585=ORIENTED_EDGE('',*,*,#10626,.F.);
#14586=ORIENTED_EDGE('',*,*,#10624,.F.);
#14587=ORIENTED_EDGE('',*,*,#10357,.F.);
#14588=ORIENTED_EDGE('',*,*,#10623,.T.);
#14589=ORIENTED_EDGE('',*,*,#10627,.F.);
#14590=ORIENTED_EDGE('',*,*,#10628,.T.);
#14591=ORIENTED_EDGE('',*,*,#10359,.F.);
#14592=ORIENTED_EDGE('',*,*,#10628,.F.);
#14593=ORIENTED_EDGE('',*,*,#10629,.F.);
#14594=ORIENTED_EDGE('',*,*,#10630,.F.);
#14595=ORIENTED_EDGE('',*,*,#10360,.F.);
#14596=ORIENTED_EDGE('',*,*,#10631,.F.);
#14597=ORIENTED_EDGE('',*,*,#10362,.F.);
#14598=ORIENTED_EDGE('',*,*,#10632,.T.);
#14599=ORIENTED_EDGE('',*,*,#10633,.F.);
#14600=ORIENTED_EDGE('',*,*,#10630,.T.);
#14601=ORIENTED_EDGE('',*,*,#10634,.F.);
#14602=ORIENTED_EDGE('',*,*,#10632,.F.);
#14603=ORIENTED_EDGE('',*,*,#10361,.F.);
#14604=ORIENTED_EDGE('',*,*,#10631,.T.);
#14605=ORIENTED_EDGE('',*,*,#10635,.F.);
#14606=ORIENTED_EDGE('',*,*,#10636,.T.);
#14607=ORIENTED_EDGE('',*,*,#10363,.F.);
#14608=ORIENTED_EDGE('',*,*,#10636,.F.);
#14609=ORIENTED_EDGE('',*,*,#10637,.F.);
#14610=ORIENTED_EDGE('',*,*,#10638,.F.);
#14611=ORIENTED_EDGE('',*,*,#10364,.F.);
#14612=ORIENTED_EDGE('',*,*,#10639,.F.);
#14613=ORIENTED_EDGE('',*,*,#10366,.F.);
#14614=ORIENTED_EDGE('',*,*,#10640,.T.);
#14615=ORIENTED_EDGE('',*,*,#10641,.F.);
#14616=ORIENTED_EDGE('',*,*,#10638,.T.);
#14617=ORIENTED_EDGE('',*,*,#10642,.F.);
#14618=ORIENTED_EDGE('',*,*,#10640,.F.);
#14619=ORIENTED_EDGE('',*,*,#10365,.F.);
#14620=ORIENTED_EDGE('',*,*,#10639,.T.);
#14621=ORIENTED_EDGE('',*,*,#10643,.F.);
#14622=ORIENTED_EDGE('',*,*,#10644,.T.);
#14623=ORIENTED_EDGE('',*,*,#10367,.F.);
#14624=ORIENTED_EDGE('',*,*,#10644,.F.);
#14625=ORIENTED_EDGE('',*,*,#10645,.F.);
#14626=ORIENTED_EDGE('',*,*,#10646,.F.);
#14627=ORIENTED_EDGE('',*,*,#10368,.F.);
#14628=ORIENTED_EDGE('',*,*,#10647,.F.);
#14629=ORIENTED_EDGE('',*,*,#10370,.F.);
#14630=ORIENTED_EDGE('',*,*,#10648,.T.);
#14631=ORIENTED_EDGE('',*,*,#10649,.F.);
#14632=ORIENTED_EDGE('',*,*,#10646,.T.);
#14633=ORIENTED_EDGE('',*,*,#10650,.F.);
#14634=ORIENTED_EDGE('',*,*,#10648,.F.);
#14635=ORIENTED_EDGE('',*,*,#10369,.F.);
#14636=ORIENTED_EDGE('',*,*,#10647,.T.);
#14637=ORIENTED_EDGE('',*,*,#10651,.F.);
#14638=ORIENTED_EDGE('',*,*,#10652,.T.);
#14639=ORIENTED_EDGE('',*,*,#10371,.F.);
#14640=ORIENTED_EDGE('',*,*,#10652,.F.);
#14641=ORIENTED_EDGE('',*,*,#10653,.F.);
#14642=ORIENTED_EDGE('',*,*,#10654,.F.);
#14643=ORIENTED_EDGE('',*,*,#10372,.F.);
#14644=ORIENTED_EDGE('',*,*,#10655,.F.);
#14645=ORIENTED_EDGE('',*,*,#10374,.F.);
#14646=ORIENTED_EDGE('',*,*,#10656,.T.);
#14647=ORIENTED_EDGE('',*,*,#10657,.F.);
#14648=ORIENTED_EDGE('',*,*,#10654,.T.);
#14649=ORIENTED_EDGE('',*,*,#10658,.F.);
#14650=ORIENTED_EDGE('',*,*,#10656,.F.);
#14651=ORIENTED_EDGE('',*,*,#10373,.F.);
#14652=ORIENTED_EDGE('',*,*,#10655,.T.);
#14653=ORIENTED_EDGE('',*,*,#10659,.F.);
#14654=ORIENTED_EDGE('',*,*,#10660,.T.);
#14655=ORIENTED_EDGE('',*,*,#10375,.F.);
#14656=ORIENTED_EDGE('',*,*,#10660,.F.);
#14657=ORIENTED_EDGE('',*,*,#10661,.F.);
#14658=ORIENTED_EDGE('',*,*,#10662,.F.);
#14659=ORIENTED_EDGE('',*,*,#10376,.F.);
#14660=ORIENTED_EDGE('',*,*,#10663,.F.);
#14661=ORIENTED_EDGE('',*,*,#10378,.F.);
#14662=ORIENTED_EDGE('',*,*,#10664,.T.);
#14663=ORIENTED_EDGE('',*,*,#10665,.F.);
#14664=ORIENTED_EDGE('',*,*,#10662,.T.);
#14665=ORIENTED_EDGE('',*,*,#10666,.F.);
#14666=ORIENTED_EDGE('',*,*,#10664,.F.);
#14667=ORIENTED_EDGE('',*,*,#10377,.F.);
#14668=ORIENTED_EDGE('',*,*,#10663,.T.);
#14669=ORIENTED_EDGE('',*,*,#10667,.F.);
#14670=ORIENTED_EDGE('',*,*,#10668,.T.);
#14671=ORIENTED_EDGE('',*,*,#10379,.F.);
#14672=ORIENTED_EDGE('',*,*,#10668,.F.);
#14673=ORIENTED_EDGE('',*,*,#10669,.F.);
#14674=ORIENTED_EDGE('',*,*,#10670,.F.);
#14675=ORIENTED_EDGE('',*,*,#10380,.F.);
#14676=ORIENTED_EDGE('',*,*,#10671,.F.);
#14677=ORIENTED_EDGE('',*,*,#10382,.F.);
#14678=ORIENTED_EDGE('',*,*,#10672,.T.);
#14679=ORIENTED_EDGE('',*,*,#10673,.F.);
#14680=ORIENTED_EDGE('',*,*,#10670,.T.);
#14681=ORIENTED_EDGE('',*,*,#10674,.F.);
#14682=ORIENTED_EDGE('',*,*,#10672,.F.);
#14683=ORIENTED_EDGE('',*,*,#10381,.F.);
#14684=ORIENTED_EDGE('',*,*,#10671,.T.);
#14685=ORIENTED_EDGE('',*,*,#10675,.F.);
#14686=ORIENTED_EDGE('',*,*,#10676,.T.);
#14687=ORIENTED_EDGE('',*,*,#10383,.F.);
#14688=ORIENTED_EDGE('',*,*,#10676,.F.);
#14689=ORIENTED_EDGE('',*,*,#10677,.F.);
#14690=ORIENTED_EDGE('',*,*,#10678,.F.);
#14691=ORIENTED_EDGE('',*,*,#10384,.F.);
#14692=ORIENTED_EDGE('',*,*,#10679,.F.);
#14693=ORIENTED_EDGE('',*,*,#10386,.F.);
#14694=ORIENTED_EDGE('',*,*,#10680,.T.);
#14695=ORIENTED_EDGE('',*,*,#10681,.F.);
#14696=ORIENTED_EDGE('',*,*,#10678,.T.);
#14697=ORIENTED_EDGE('',*,*,#10682,.F.);
#14698=ORIENTED_EDGE('',*,*,#10680,.F.);
#14699=ORIENTED_EDGE('',*,*,#10385,.F.);
#14700=ORIENTED_EDGE('',*,*,#10679,.T.);
#14701=ORIENTED_EDGE('',*,*,#10683,.F.);
#14702=ORIENTED_EDGE('',*,*,#10684,.T.);
#14703=ORIENTED_EDGE('',*,*,#10387,.F.);
#14704=ORIENTED_EDGE('',*,*,#10684,.F.);
#14705=ORIENTED_EDGE('',*,*,#10685,.F.);
#14706=ORIENTED_EDGE('',*,*,#10686,.F.);
#14707=ORIENTED_EDGE('',*,*,#10388,.F.);
#14708=ORIENTED_EDGE('',*,*,#10687,.F.);
#14709=ORIENTED_EDGE('',*,*,#10390,.F.);
#14710=ORIENTED_EDGE('',*,*,#10688,.T.);
#14711=ORIENTED_EDGE('',*,*,#10689,.F.);
#14712=ORIENTED_EDGE('',*,*,#10686,.T.);
#14713=ORIENTED_EDGE('',*,*,#10690,.F.);
#14714=ORIENTED_EDGE('',*,*,#10688,.F.);
#14715=ORIENTED_EDGE('',*,*,#10389,.F.);
#14716=ORIENTED_EDGE('',*,*,#10687,.T.);
#14717=ORIENTED_EDGE('',*,*,#10691,.F.);
#14718=ORIENTED_EDGE('',*,*,#10692,.T.);
#14719=ORIENTED_EDGE('',*,*,#10391,.F.);
#14720=ORIENTED_EDGE('',*,*,#10692,.F.);
#14721=ORIENTED_EDGE('',*,*,#10693,.F.);
#14722=ORIENTED_EDGE('',*,*,#10694,.F.);
#14723=ORIENTED_EDGE('',*,*,#10392,.F.);
#14724=ORIENTED_EDGE('',*,*,#10695,.F.);
#14725=ORIENTED_EDGE('',*,*,#10394,.F.);
#14726=ORIENTED_EDGE('',*,*,#10696,.T.);
#14727=ORIENTED_EDGE('',*,*,#10697,.F.);
#14728=ORIENTED_EDGE('',*,*,#10694,.T.);
#14729=ORIENTED_EDGE('',*,*,#10698,.F.);
#14730=ORIENTED_EDGE('',*,*,#10696,.F.);
#14731=ORIENTED_EDGE('',*,*,#10393,.F.);
#14732=ORIENTED_EDGE('',*,*,#10695,.T.);
#14733=ORIENTED_EDGE('',*,*,#10699,.F.);
#14734=ORIENTED_EDGE('',*,*,#10700,.T.);
#14735=ORIENTED_EDGE('',*,*,#10395,.F.);
#14736=ORIENTED_EDGE('',*,*,#10700,.F.);
#14737=ORIENTED_EDGE('',*,*,#10701,.F.);
#14738=ORIENTED_EDGE('',*,*,#10702,.F.);
#14739=ORIENTED_EDGE('',*,*,#10396,.F.);
#14740=ORIENTED_EDGE('',*,*,#10703,.F.);
#14741=ORIENTED_EDGE('',*,*,#10398,.F.);
#14742=ORIENTED_EDGE('',*,*,#10704,.T.);
#14743=ORIENTED_EDGE('',*,*,#10705,.F.);
#14744=ORIENTED_EDGE('',*,*,#10702,.T.);
#14745=ORIENTED_EDGE('',*,*,#10706,.F.);
#14746=ORIENTED_EDGE('',*,*,#10704,.F.);
#14747=ORIENTED_EDGE('',*,*,#10397,.F.);
#14748=ORIENTED_EDGE('',*,*,#10703,.T.);
#14749=ORIENTED_EDGE('',*,*,#10707,.F.);
#14750=ORIENTED_EDGE('',*,*,#10708,.T.);
#14751=ORIENTED_EDGE('',*,*,#10399,.F.);
#14752=ORIENTED_EDGE('',*,*,#10708,.F.);
#14753=ORIENTED_EDGE('',*,*,#10709,.F.);
#14754=ORIENTED_EDGE('',*,*,#10710,.F.);
#14755=ORIENTED_EDGE('',*,*,#10400,.F.);
#14756=ORIENTED_EDGE('',*,*,#10711,.F.);
#14757=ORIENTED_EDGE('',*,*,#10402,.F.);
#14758=ORIENTED_EDGE('',*,*,#10712,.T.);
#14759=ORIENTED_EDGE('',*,*,#10713,.F.);
#14760=ORIENTED_EDGE('',*,*,#10710,.T.);
#14761=ORIENTED_EDGE('',*,*,#10714,.F.);
#14762=ORIENTED_EDGE('',*,*,#10712,.F.);
#14763=ORIENTED_EDGE('',*,*,#10401,.F.);
#14764=ORIENTED_EDGE('',*,*,#10711,.T.);
#14765=ORIENTED_EDGE('',*,*,#10715,.F.);
#14766=ORIENTED_EDGE('',*,*,#10716,.T.);
#14767=ORIENTED_EDGE('',*,*,#10403,.F.);
#14768=ORIENTED_EDGE('',*,*,#10716,.F.);
#14769=ORIENTED_EDGE('',*,*,#10717,.F.);
#14770=ORIENTED_EDGE('',*,*,#10718,.F.);
#14771=ORIENTED_EDGE('',*,*,#10404,.F.);
#14772=ORIENTED_EDGE('',*,*,#10719,.F.);
#14773=ORIENTED_EDGE('',*,*,#10406,.F.);
#14774=ORIENTED_EDGE('',*,*,#10720,.T.);
#14775=ORIENTED_EDGE('',*,*,#10721,.F.);
#14776=ORIENTED_EDGE('',*,*,#10718,.T.);
#14777=ORIENTED_EDGE('',*,*,#10722,.F.);
#14778=ORIENTED_EDGE('',*,*,#10720,.F.);
#14779=ORIENTED_EDGE('',*,*,#10405,.F.);
#14780=ORIENTED_EDGE('',*,*,#10719,.T.);
#14781=ORIENTED_EDGE('',*,*,#10723,.F.);
#14782=ORIENTED_EDGE('',*,*,#10724,.T.);
#14783=ORIENTED_EDGE('',*,*,#10407,.F.);
#14784=ORIENTED_EDGE('',*,*,#10724,.F.);
#14785=ORIENTED_EDGE('',*,*,#10725,.F.);
#14786=ORIENTED_EDGE('',*,*,#10726,.F.);
#14787=ORIENTED_EDGE('',*,*,#10408,.F.);
#14788=ORIENTED_EDGE('',*,*,#10727,.F.);
#14789=ORIENTED_EDGE('',*,*,#10410,.F.);
#14790=ORIENTED_EDGE('',*,*,#10728,.T.);
#14791=ORIENTED_EDGE('',*,*,#10729,.F.);
#14792=ORIENTED_EDGE('',*,*,#10726,.T.);
#14793=ORIENTED_EDGE('',*,*,#10730,.F.);
#14794=ORIENTED_EDGE('',*,*,#10728,.F.);
#14795=ORIENTED_EDGE('',*,*,#10409,.F.);
#14796=ORIENTED_EDGE('',*,*,#10727,.T.);
#14797=ORIENTED_EDGE('',*,*,#10731,.F.);
#14798=ORIENTED_EDGE('',*,*,#10732,.T.);
#14799=ORIENTED_EDGE('',*,*,#10411,.F.);
#14800=ORIENTED_EDGE('',*,*,#10732,.F.);
#14801=ORIENTED_EDGE('',*,*,#10733,.F.);
#14802=ORIENTED_EDGE('',*,*,#10734,.F.);
#14803=ORIENTED_EDGE('',*,*,#10412,.F.);
#14804=ORIENTED_EDGE('',*,*,#10734,.T.);
#14805=ORIENTED_EDGE('',*,*,#10735,.F.);
#14806=ORIENTED_EDGE('',*,*,#10736,.F.);
#14807=ORIENTED_EDGE('',*,*,#10413,.F.);
#14808=ORIENTED_EDGE('',*,*,#10737,.F.);
#14809=ORIENTED_EDGE('',*,*,#10414,.F.);
#14810=ORIENTED_EDGE('',*,*,#10736,.T.);
#14811=ORIENTED_EDGE('',*,*,#10738,.F.);
#14812=ORIENTED_EDGE('',*,*,#10737,.T.);
#14813=ORIENTED_EDGE('',*,*,#10739,.F.);
#14814=ORIENTED_EDGE('',*,*,#10740,.T.);
#14815=ORIENTED_EDGE('',*,*,#10415,.F.);
#14816=ORIENTED_EDGE('',*,*,#10741,.F.);
#14817=ORIENTED_EDGE('',*,*,#10418,.F.);
#14818=ORIENTED_EDGE('',*,*,#10742,.T.);
#14819=ORIENTED_EDGE('',*,*,#10743,.F.);
#14820=ORIENTED_EDGE('',*,*,#10740,.F.);
#14821=ORIENTED_EDGE('',*,*,#10744,.F.);
#14822=ORIENTED_EDGE('',*,*,#10745,.F.);
#14823=ORIENTED_EDGE('',*,*,#10416,.F.);
#14824=ORIENTED_EDGE('',*,*,#10745,.T.);
#14825=ORIENTED_EDGE('',*,*,#10746,.F.);
#14826=ORIENTED_EDGE('',*,*,#10742,.F.);
#14827=ORIENTED_EDGE('',*,*,#10417,.F.);
#14828=ORIENTED_EDGE('',*,*,#10433,.T.);
#14829=ORIENTED_EDGE('',*,*,#10434,.T.);
#14830=ORIENTED_EDGE('',*,*,#10429,.T.);
#14831=ORIENTED_EDGE('',*,*,#10747,.T.);
#14832=ORIENTED_EDGE('',*,*,#10743,.T.);
#14833=ORIENTED_EDGE('',*,*,#10746,.T.);
#14834=ORIENTED_EDGE('',*,*,#10744,.T.);
#14835=ORIENTED_EDGE('',*,*,#10739,.T.);
#14836=ORIENTED_EDGE('',*,*,#10738,.T.);
#14837=ORIENTED_EDGE('',*,*,#10735,.T.);
#14838=ORIENTED_EDGE('',*,*,#10733,.T.);
#14839=ORIENTED_EDGE('',*,*,#10731,.T.);
#14840=ORIENTED_EDGE('',*,*,#10729,.T.);
#14841=ORIENTED_EDGE('',*,*,#10730,.T.);
#14842=ORIENTED_EDGE('',*,*,#10725,.T.);
#14843=ORIENTED_EDGE('',*,*,#10723,.T.);
#14844=ORIENTED_EDGE('',*,*,#10721,.T.);
#14845=ORIENTED_EDGE('',*,*,#10722,.T.);
#14846=ORIENTED_EDGE('',*,*,#10717,.T.);
#14847=ORIENTED_EDGE('',*,*,#10715,.T.);
#14848=ORIENTED_EDGE('',*,*,#10713,.T.);
#14849=ORIENTED_EDGE('',*,*,#10714,.T.);
#14850=ORIENTED_EDGE('',*,*,#10709,.T.);
#14851=ORIENTED_EDGE('',*,*,#10707,.T.);
#14852=ORIENTED_EDGE('',*,*,#10705,.T.);
#14853=ORIENTED_EDGE('',*,*,#10706,.T.);
#14854=ORIENTED_EDGE('',*,*,#10701,.T.);
#14855=ORIENTED_EDGE('',*,*,#10699,.T.);
#14856=ORIENTED_EDGE('',*,*,#10697,.T.);
#14857=ORIENTED_EDGE('',*,*,#10698,.T.);
#14858=ORIENTED_EDGE('',*,*,#10693,.T.);
#14859=ORIENTED_EDGE('',*,*,#10691,.T.);
#14860=ORIENTED_EDGE('',*,*,#10689,.T.);
#14861=ORIENTED_EDGE('',*,*,#10690,.T.);
#14862=ORIENTED_EDGE('',*,*,#10685,.T.);
#14863=ORIENTED_EDGE('',*,*,#10683,.T.);
#14864=ORIENTED_EDGE('',*,*,#10681,.T.);
#14865=ORIENTED_EDGE('',*,*,#10682,.T.);
#14866=ORIENTED_EDGE('',*,*,#10677,.T.);
#14867=ORIENTED_EDGE('',*,*,#10675,.T.);
#14868=ORIENTED_EDGE('',*,*,#10673,.T.);
#14869=ORIENTED_EDGE('',*,*,#10674,.T.);
#14870=ORIENTED_EDGE('',*,*,#10669,.T.);
#14871=ORIENTED_EDGE('',*,*,#10667,.T.);
#14872=ORIENTED_EDGE('',*,*,#10665,.T.);
#14873=ORIENTED_EDGE('',*,*,#10666,.T.);
#14874=ORIENTED_EDGE('',*,*,#10661,.T.);
#14875=ORIENTED_EDGE('',*,*,#10659,.T.);
#14876=ORIENTED_EDGE('',*,*,#10657,.T.);
#14877=ORIENTED_EDGE('',*,*,#10658,.T.);
#14878=ORIENTED_EDGE('',*,*,#10653,.T.);
#14879=ORIENTED_EDGE('',*,*,#10651,.T.);
#14880=ORIENTED_EDGE('',*,*,#10649,.T.);
#14881=ORIENTED_EDGE('',*,*,#10650,.T.);
#14882=ORIENTED_EDGE('',*,*,#10645,.T.);
#14883=ORIENTED_EDGE('',*,*,#10643,.T.);
#14884=ORIENTED_EDGE('',*,*,#10641,.T.);
#14885=ORIENTED_EDGE('',*,*,#10642,.T.);
#14886=ORIENTED_EDGE('',*,*,#10637,.T.);
#14887=ORIENTED_EDGE('',*,*,#10635,.T.);
#14888=ORIENTED_EDGE('',*,*,#10633,.T.);
#14889=ORIENTED_EDGE('',*,*,#10634,.T.);
#14890=ORIENTED_EDGE('',*,*,#10629,.T.);
#14891=ORIENTED_EDGE('',*,*,#10627,.T.);
#14892=ORIENTED_EDGE('',*,*,#10625,.T.);
#14893=ORIENTED_EDGE('',*,*,#10626,.T.);
#14894=ORIENTED_EDGE('',*,*,#10621,.T.);
#14895=ORIENTED_EDGE('',*,*,#10619,.T.);
#14896=ORIENTED_EDGE('',*,*,#10617,.T.);
#14897=ORIENTED_EDGE('',*,*,#10618,.T.);
#14898=ORIENTED_EDGE('',*,*,#10613,.T.);
#14899=ORIENTED_EDGE('',*,*,#10611,.T.);
#14900=ORIENTED_EDGE('',*,*,#10609,.T.);
#14901=ORIENTED_EDGE('',*,*,#10610,.T.);
#14902=ORIENTED_EDGE('',*,*,#10605,.T.);
#14903=ORIENTED_EDGE('',*,*,#10603,.T.);
#14904=ORIENTED_EDGE('',*,*,#10601,.T.);
#14905=ORIENTED_EDGE('',*,*,#10602,.T.);
#14906=ORIENTED_EDGE('',*,*,#10597,.T.);
#14907=ORIENTED_EDGE('',*,*,#10595,.T.);
#14908=ORIENTED_EDGE('',*,*,#10593,.T.);
#14909=ORIENTED_EDGE('',*,*,#10594,.T.);
#14910=ORIENTED_EDGE('',*,*,#10589,.T.);
#14911=ORIENTED_EDGE('',*,*,#10587,.T.);
#14912=ORIENTED_EDGE('',*,*,#10585,.T.);
#14913=ORIENTED_EDGE('',*,*,#10586,.T.);
#14914=ORIENTED_EDGE('',*,*,#10581,.T.);
#14915=ORIENTED_EDGE('',*,*,#10579,.T.);
#14916=ORIENTED_EDGE('',*,*,#10577,.T.);
#14917=ORIENTED_EDGE('',*,*,#10578,.T.);
#14918=ORIENTED_EDGE('',*,*,#10573,.T.);
#14919=ORIENTED_EDGE('',*,*,#10571,.T.);
#14920=ORIENTED_EDGE('',*,*,#10569,.T.);
#14921=ORIENTED_EDGE('',*,*,#10570,.T.);
#14922=ORIENTED_EDGE('',*,*,#10565,.T.);
#14923=ORIENTED_EDGE('',*,*,#10563,.T.);
#14924=ORIENTED_EDGE('',*,*,#10561,.T.);
#14925=ORIENTED_EDGE('',*,*,#10562,.T.);
#14926=ORIENTED_EDGE('',*,*,#10557,.T.);
#14927=ORIENTED_EDGE('',*,*,#10555,.T.);
#14928=ORIENTED_EDGE('',*,*,#10553,.T.);
#14929=ORIENTED_EDGE('',*,*,#10554,.T.);
#14930=ORIENTED_EDGE('',*,*,#10549,.T.);
#14931=ORIENTED_EDGE('',*,*,#10547,.T.);
#14932=ORIENTED_EDGE('',*,*,#10545,.T.);
#14933=ORIENTED_EDGE('',*,*,#10546,.T.);
#14934=ORIENTED_EDGE('',*,*,#10541,.T.);
#14935=ORIENTED_EDGE('',*,*,#10539,.T.);
#14936=ORIENTED_EDGE('',*,*,#10537,.T.);
#14937=ORIENTED_EDGE('',*,*,#10538,.T.);
#14938=ORIENTED_EDGE('',*,*,#10533,.T.);
#14939=ORIENTED_EDGE('',*,*,#10531,.T.);
#14940=ORIENTED_EDGE('',*,*,#10529,.T.);
#14941=ORIENTED_EDGE('',*,*,#10530,.T.);
#14942=ORIENTED_EDGE('',*,*,#10525,.T.);
#14943=ORIENTED_EDGE('',*,*,#10523,.T.);
#14944=ORIENTED_EDGE('',*,*,#10521,.T.);
#14945=ORIENTED_EDGE('',*,*,#10522,.T.);
#14946=ORIENTED_EDGE('',*,*,#10517,.T.);
#14947=ORIENTED_EDGE('',*,*,#10515,.T.);
#14948=ORIENTED_EDGE('',*,*,#10513,.T.);
#14949=ORIENTED_EDGE('',*,*,#10514,.T.);
#14950=ORIENTED_EDGE('',*,*,#10509,.T.);
#14951=ORIENTED_EDGE('',*,*,#10507,.T.);
#14952=ORIENTED_EDGE('',*,*,#10505,.T.);
#14953=ORIENTED_EDGE('',*,*,#10506,.T.);
#14954=ORIENTED_EDGE('',*,*,#10501,.T.);
#14955=ORIENTED_EDGE('',*,*,#10499,.T.);
#14956=ORIENTED_EDGE('',*,*,#10497,.T.);
#14957=ORIENTED_EDGE('',*,*,#10498,.T.);
#14958=ORIENTED_EDGE('',*,*,#10493,.T.);
#14959=ORIENTED_EDGE('',*,*,#10491,.T.);
#14960=ORIENTED_EDGE('',*,*,#10489,.T.);
#14961=ORIENTED_EDGE('',*,*,#10490,.T.);
#14962=ORIENTED_EDGE('',*,*,#10485,.T.);
#14963=ORIENTED_EDGE('',*,*,#10483,.T.);
#14964=ORIENTED_EDGE('',*,*,#10481,.T.);
#14965=ORIENTED_EDGE('',*,*,#10482,.T.);
#14966=ORIENTED_EDGE('',*,*,#10477,.T.);
#14967=ORIENTED_EDGE('',*,*,#10475,.T.);
#14968=ORIENTED_EDGE('',*,*,#10473,.T.);
#14969=ORIENTED_EDGE('',*,*,#10474,.T.);
#14970=ORIENTED_EDGE('',*,*,#10469,.T.);
#14971=ORIENTED_EDGE('',*,*,#10467,.T.);
#14972=ORIENTED_EDGE('',*,*,#10465,.T.);
#14973=ORIENTED_EDGE('',*,*,#10466,.T.);
#14974=ORIENTED_EDGE('',*,*,#10461,.T.);
#14975=ORIENTED_EDGE('',*,*,#10459,.T.);
#14976=ORIENTED_EDGE('',*,*,#10457,.T.);
#14977=ORIENTED_EDGE('',*,*,#10458,.T.);
#14978=ORIENTED_EDGE('',*,*,#10453,.T.);
#14979=ORIENTED_EDGE('',*,*,#10451,.T.);
#14980=ORIENTED_EDGE('',*,*,#10449,.T.);
#14981=ORIENTED_EDGE('',*,*,#10450,.T.);
#14982=ORIENTED_EDGE('',*,*,#10445,.T.);
#14983=ORIENTED_EDGE('',*,*,#10443,.T.);
#14984=ORIENTED_EDGE('',*,*,#10441,.T.);
#14985=ORIENTED_EDGE('',*,*,#10442,.T.);
#14986=ORIENTED_EDGE('',*,*,#10437,.T.);
#14987=ORIENTED_EDGE('',*,*,#10435,.T.);
#14988=ORIENTED_EDGE('',*,*,#10427,.T.);
#14989=ORIENTED_EDGE('',*,*,#10428,.T.);
#14990=ORIENTED_EDGE('',*,*,#10419,.F.);
#14991=ORIENTED_EDGE('',*,*,#10741,.T.);
#14992=ORIENTED_EDGE('',*,*,#10747,.F.);
#15386=CYLINDRICAL_SURFACE('',#18528,1.);
#15387=CYLINDRICAL_SURFACE('',#18530,2.);
#15388=CYLINDRICAL_SURFACE('',#18535,3.75);
#15389=CYLINDRICAL_SURFACE('',#18538,3.75);
#15390=CYLINDRICAL_SURFACE('',#18541,3.75);
#15391=CYLINDRICAL_SURFACE('',#18544,3.75);
#15392=CYLINDRICAL_SURFACE('',#18547,3.75);
#15393=CYLINDRICAL_SURFACE('',#18550,3.75);
#15394=CYLINDRICAL_SURFACE('',#18553,3.75);
#15395=CYLINDRICAL_SURFACE('',#18556,3.75);
#15396=CYLINDRICAL_SURFACE('',#18559,3.75);
#15397=CYLINDRICAL_SURFACE('',#18562,3.75);
#15398=CYLINDRICAL_SURFACE('',#18565,3.75);
#15399=CYLINDRICAL_SURFACE('',#18568,3.75);
#15400=CYLINDRICAL_SURFACE('',#18571,3.75);
#15401=CYLINDRICAL_SURFACE('',#18574,3.75);
#15402=CYLINDRICAL_SURFACE('',#18577,3.75);
#15403=CYLINDRICAL_SURFACE('',#18580,3.75);
#15404=CYLINDRICAL_SURFACE('',#18583,3.75);
#15405=CYLINDRICAL_SURFACE('',#18586,3.75);
#15406=CYLINDRICAL_SURFACE('',#18589,3.75);
#15407=CYLINDRICAL_SURFACE('',#18592,3.75);
#15408=CYLINDRICAL_SURFACE('',#18595,3.75);
#15409=CYLINDRICAL_SURFACE('',#18598,3.75);
#15410=CYLINDRICAL_SURFACE('',#18601,3.75);
#15411=CYLINDRICAL_SURFACE('',#18604,3.75);
#15412=CYLINDRICAL_SURFACE('',#18607,3.75);
#15413=CYLINDRICAL_SURFACE('',#18610,3.75);
#15414=CYLINDRICAL_SURFACE('',#18613,3.75);
#15415=CYLINDRICAL_SURFACE('',#18616,3.75);
#15416=CYLINDRICAL_SURFACE('',#18619,3.75);
#15417=CYLINDRICAL_SURFACE('',#18622,3.75);
#15418=CYLINDRICAL_SURFACE('',#18625,3.75);
#15419=CYLINDRICAL_SURFACE('',#18628,3.75);
#15420=CYLINDRICAL_SURFACE('',#18631,3.75);
#15421=CYLINDRICAL_SURFACE('',#18634,3.75);
#15422=CYLINDRICAL_SURFACE('',#18637,3.75);
#15423=CYLINDRICAL_SURFACE('',#18640,3.75);
#15424=CYLINDRICAL_SURFACE('',#18643,3.75);
#15425=CYLINDRICAL_SURFACE('',#18646,3.75);
#15426=CYLINDRICAL_SURFACE('',#18649,3.75);
#15427=CYLINDRICAL_SURFACE('',#18654,3.75);
#16158=ADVANCED_FACE('',(#2848),#2045,.F.);
#16159=ADVANCED_FACE('',(#2849),#2046,.F.);
#16160=ADVANCED_FACE('',(#2850),#2047,.F.);
#16161=ADVANCED_FACE('',(#2851,#1626),#2048,.F.);
#16162=ADVANCED_FACE('',(#2852),#15386,.F.);
#16163=ADVANCED_FACE('',(#2853),#15387,.T.);
#16164=ADVANCED_FACE('',(#2854,#1627),#2049,.T.);
#16165=ADVANCED_FACE('',(#2855),#51,.T.);
#16166=ADVANCED_FACE('',(#2856),#52,.T.);
#16167=ADVANCED_FACE('',(#2857),#2050,.T.);
#16168=ADVANCED_FACE('',(#2858),#15388,.T.);
#16169=ADVANCED_FACE('',(#2859),#53,.T.);
#16170=ADVANCED_FACE('',(#2860),#54,.T.);
#16171=ADVANCED_FACE('',(#2861),#2051,.T.);
#16172=ADVANCED_FACE('',(#2862),#15389,.T.);
#16173=ADVANCED_FACE('',(#2863),#55,.T.);
#16174=ADVANCED_FACE('',(#2864),#56,.T.);
#16175=ADVANCED_FACE('',(#2865),#2052,.T.);
#16176=ADVANCED_FACE('',(#2866),#15390,.T.);
#16177=ADVANCED_FACE('',(#2867),#57,.T.);
#16178=ADVANCED_FACE('',(#2868),#58,.T.);
#16179=ADVANCED_FACE('',(#2869),#2053,.T.);
#16180=ADVANCED_FACE('',(#2870),#15391,.T.);
#16181=ADVANCED_FACE('',(#2871),#59,.T.);
#16182=ADVANCED_FACE('',(#2872),#60,.T.);
#16183=ADVANCED_FACE('',(#2873),#2054,.T.);
#16184=ADVANCED_FACE('',(#2874),#15392,.T.);
#16185=ADVANCED_FACE('',(#2875),#61,.T.);
#16186=ADVANCED_FACE('',(#2876),#62,.T.);
#16187=ADVANCED_FACE('',(#2877),#2055,.T.);
#16188=ADVANCED_FACE('',(#2878),#15393,.T.);
#16189=ADVANCED_FACE('',(#2879),#63,.T.);
#16190=ADVANCED_FACE('',(#2880),#64,.T.);
#16191=ADVANCED_FACE('',(#2881),#2056,.T.);
#16192=ADVANCED_FACE('',(#2882),#15394,.T.);
#16193=ADVANCED_FACE('',(#2883),#65,.T.);
#16194=ADVANCED_FACE('',(#2884),#66,.T.);
#16195=ADVANCED_FACE('',(#2885),#2057,.T.);
#16196=ADVANCED_FACE('',(#2886),#15395,.T.);
#16197=ADVANCED_FACE('',(#2887),#67,.T.);
#16198=ADVANCED_FACE('',(#2888),#68,.T.);
#16199=ADVANCED_FACE('',(#2889),#2058,.T.);
#16200=ADVANCED_FACE('',(#2890),#15396,.T.);
#16201=ADVANCED_FACE('',(#2891),#69,.T.);
#16202=ADVANCED_FACE('',(#2892),#70,.T.);
#16203=ADVANCED_FACE('',(#2893),#2059,.T.);
#16204=ADVANCED_FACE('',(#2894),#15397,.T.);
#16205=ADVANCED_FACE('',(#2895),#71,.T.);
#16206=ADVANCED_FACE('',(#2896),#72,.T.);
#16207=ADVANCED_FACE('',(#2897),#2060,.T.);
#16208=ADVANCED_FACE('',(#2898),#15398,.T.);
#16209=ADVANCED_FACE('',(#2899),#73,.T.);
#16210=ADVANCED_FACE('',(#2900),#74,.T.);
#16211=ADVANCED_FACE('',(#2901),#2061,.T.);
#16212=ADVANCED_FACE('',(#2902),#15399,.T.);
#16213=ADVANCED_FACE('',(#2903),#75,.T.);
#16214=ADVANCED_FACE('',(#2904),#76,.T.);
#16215=ADVANCED_FACE('',(#2905),#2062,.T.);
#16216=ADVANCED_FACE('',(#2906),#15400,.T.);
#16217=ADVANCED_FACE('',(#2907),#77,.T.);
#16218=ADVANCED_FACE('',(#2908),#78,.T.);
#16219=ADVANCED_FACE('',(#2909),#2063,.T.);
#16220=ADVANCED_FACE('',(#2910),#15401,.T.);
#16221=ADVANCED_FACE('',(#2911),#79,.T.);
#16222=ADVANCED_FACE('',(#2912),#80,.T.);
#16223=ADVANCED_FACE('',(#2913),#2064,.T.);
#16224=ADVANCED_FACE('',(#2914),#15402,.T.);
#16225=ADVANCED_FACE('',(#2915),#81,.T.);
#16226=ADVANCED_FACE('',(#2916),#82,.T.);
#16227=ADVANCED_FACE('',(#2917),#2065,.T.);
#16228=ADVANCED_FACE('',(#2918),#15403,.T.);
#16229=ADVANCED_FACE('',(#2919),#83,.T.);
#16230=ADVANCED_FACE('',(#2920),#84,.T.);
#16231=ADVANCED_FACE('',(#2921),#2066,.T.);
#16232=ADVANCED_FACE('',(#2922),#15404,.T.);
#16233=ADVANCED_FACE('',(#2923),#85,.T.);
#16234=ADVANCED_FACE('',(#2924),#86,.T.);
#16235=ADVANCED_FACE('',(#2925),#2067,.T.);
#16236=ADVANCED_FACE('',(#2926),#15405,.T.);
#16237=ADVANCED_FACE('',(#2927),#87,.T.);
#16238=ADVANCED_FACE('',(#2928),#88,.T.);
#16239=ADVANCED_FACE('',(#2929),#2068,.T.);
#16240=ADVANCED_FACE('',(#2930),#15406,.T.);
#16241=ADVANCED_FACE('',(#2931),#89,.T.);
#16242=ADVANCED_FACE('',(#2932),#90,.T.);
#16243=ADVANCED_FACE('',(#2933),#2069,.T.);
#16244=ADVANCED_FACE('',(#2934),#15407,.T.);
#16245=ADVANCED_FACE('',(#2935),#91,.T.);
#16246=ADVANCED_FACE('',(#2936),#92,.T.);
#16247=ADVANCED_FACE('',(#2937),#2070,.T.);
#16248=ADVANCED_FACE('',(#2938),#15408,.T.);
#16249=ADVANCED_FACE('',(#2939),#93,.T.);
#16250=ADVANCED_FACE('',(#2940),#94,.T.);
#16251=ADVANCED_FACE('',(#2941),#2071,.T.);
#16252=ADVANCED_FACE('',(#2942),#15409,.T.);
#16253=ADVANCED_FACE('',(#2943),#95,.T.);
#16254=ADVANCED_FACE('',(#2944),#96,.T.);
#16255=ADVANCED_FACE('',(#2945),#2072,.T.);
#16256=ADVANCED_FACE('',(#2946),#15410,.T.);
#16257=ADVANCED_FACE('',(#2947),#97,.T.);
#16258=ADVANCED_FACE('',(#2948),#98,.T.);
#16259=ADVANCED_FACE('',(#2949),#2073,.T.);
#16260=ADVANCED_FACE('',(#2950),#15411,.T.);
#16261=ADVANCED_FACE('',(#2951),#99,.T.);
#16262=ADVANCED_FACE('',(#2952),#100,.T.);
#16263=ADVANCED_FACE('',(#2953),#2074,.T.);
#16264=ADVANCED_FACE('',(#2954),#15412,.T.);
#16265=ADVANCED_FACE('',(#2955),#101,.T.);
#16266=ADVANCED_FACE('',(#2956),#102,.T.);
#16267=ADVANCED_FACE('',(#2957),#2075,.T.);
#16268=ADVANCED_FACE('',(#2958),#15413,.T.);
#16269=ADVANCED_FACE('',(#2959),#103,.T.);
#16270=ADVANCED_FACE('',(#2960),#104,.T.);
#16271=ADVANCED_FACE('',(#2961),#2076,.T.);
#16272=ADVANCED_FACE('',(#2962),#15414,.T.);
#16273=ADVANCED_FACE('',(#2963),#105,.T.);
#16274=ADVANCED_FACE('',(#2964),#106,.T.);
#16275=ADVANCED_FACE('',(#2965),#2077,.T.);
#16276=ADVANCED_FACE('',(#2966),#15415,.T.);
#16277=ADVANCED_FACE('',(#2967),#107,.T.);
#16278=ADVANCED_FACE('',(#2968),#108,.T.);
#16279=ADVANCED_FACE('',(#2969),#2078,.T.);
#16280=ADVANCED_FACE('',(#2970),#15416,.T.);
#16281=ADVANCED_FACE('',(#2971),#109,.T.);
#16282=ADVANCED_FACE('',(#2972),#110,.T.);
#16283=ADVANCED_FACE('',(#2973),#2079,.T.);
#16284=ADVANCED_FACE('',(#2974),#15417,.T.);
#16285=ADVANCED_FACE('',(#2975),#111,.T.);
#16286=ADVANCED_FACE('',(#2976),#112,.T.);
#16287=ADVANCED_FACE('',(#2977),#2080,.T.);
#16288=ADVANCED_FACE('',(#2978),#15418,.T.);
#16289=ADVANCED_FACE('',(#2979),#113,.T.);
#16290=ADVANCED_FACE('',(#2980),#114,.T.);
#16291=ADVANCED_FACE('',(#2981),#2081,.T.);
#16292=ADVANCED_FACE('',(#2982),#15419,.T.);
#16293=ADVANCED_FACE('',(#2983),#115,.T.);
#16294=ADVANCED_FACE('',(#2984),#116,.T.);
#16295=ADVANCED_FACE('',(#2985),#2082,.T.);
#16296=ADVANCED_FACE('',(#2986),#15420,.T.);
#16297=ADVANCED_FACE('',(#2987),#117,.T.);
#16298=ADVANCED_FACE('',(#2988),#118,.T.);
#16299=ADVANCED_FACE('',(#2989),#2083,.T.);
#16300=ADVANCED_FACE('',(#2990),#15421,.T.);
#16301=ADVANCED_FACE('',(#2991),#119,.T.);
#16302=ADVANCED_FACE('',(#2992),#120,.T.);
#16303=ADVANCED_FACE('',(#2993),#2084,.T.);
#16304=ADVANCED_FACE('',(#2994),#15422,.T.);
#16305=ADVANCED_FACE('',(#2995),#121,.T.);
#16306=ADVANCED_FACE('',(#2996),#122,.T.);
#16307=ADVANCED_FACE('',(#2997),#2085,.T.);
#16308=ADVANCED_FACE('',(#2998),#15423,.T.);
#16309=ADVANCED_FACE('',(#2999),#123,.T.);
#16310=ADVANCED_FACE('',(#3000),#124,.T.);
#16311=ADVANCED_FACE('',(#3001),#2086,.T.);
#16312=ADVANCED_FACE('',(#3002),#15424,.T.);
#16313=ADVANCED_FACE('',(#3003),#125,.T.);
#16314=ADVANCED_FACE('',(#3004),#126,.T.);
#16315=ADVANCED_FACE('',(#3005),#2087,.T.);
#16316=ADVANCED_FACE('',(#3006),#15425,.T.);
#16317=ADVANCED_FACE('',(#3007),#127,.T.);
#16318=ADVANCED_FACE('',(#3008),#2088,.T.);
#16319=ADVANCED_FACE('',(#3009),#128,.T.);
#16320=ADVANCED_FACE('',(#3010),#15426,.T.);
#16321=ADVANCED_FACE('',(#3011),#129,.T.);
#16322=ADVANCED_FACE('',(#3012),#130,.T.);
#16323=ADVANCED_FACE('',(#3013),#2089,.T.);
#16324=ADVANCED_FACE('',(#3014,#1628),#2090,.T.);
#16325=ADVANCED_FACE('',(#3015),#15427,.T.);
#16447=CLOSED_SHELL('',(#16158,#16159,#16160,#16161,#16162,#16163,#16164,
#16165,#16166,#16167,#16168,#16169,#16170,#16171,#16172,#16173,#16174,#16175,
#16176,#16177,#16178,#16179,#16180,#16181,#16182,#16183,#16184,#16185,#16186,
#16187,#16188,#16189,#16190,#16191,#16192,#16193,#16194,#16195,#16196,#16197,
#16198,#16199,#16200,#16201,#16202,#16203,#16204,#16205,#16206,#16207,#16208,
#16209,#16210,#16211,#16212,#16213,#16214,#16215,#16216,#16217,#16218,#16219,
#16220,#16221,#16222,#16223,#16224,#16225,#16226,#16227,#16228,#16229,#16230,
#16231,#16232,#16233,#16234,#16235,#16236,#16237,#16238,#16239,#16240,#16241,
#16242,#16243,#16244,#16245,#16246,#16247,#16248,#16249,#16250,#16251,#16252,
#16253,#16254,#16255,#16256,#16257,#16258,#16259,#16260,#16261,#16262,#16263,
#16264,#16265,#16266,#16267,#16268,#16269,#16270,#16271,#16272,#16273,#16274,
#16275,#16276,#16277,#16278,#16279,#16280,#16281,#16282,#16283,#16284,#16285,
#16286,#16287,#16288,#16289,#16290,#16291,#16292,#16293,#16294,#16295,#16296,
#16297,#16298,#16299,#16300,#16301,#16302,#16303,#16304,#16305,#16306,#16307,
#16308,#16309,#16310,#16311,#16312,#16313,#16314,#16315,#16316,#16317,#16318,
#16319,#16320,#16321,#16322,#16323,#16324,#16325));
#18482=AXIS2_PLACEMENT_3D('',#38754,#22369,#22370);
#18483=AXIS2_PLACEMENT_3D('',#38755,#22371,#22372);
#18484=AXIS2_PLACEMENT_3D('',#38764,#22377,#22378);
#18485=AXIS2_PLACEMENT_3D('',#38770,#22382,#22383);
#18486=AXIS2_PLACEMENT_3D('',#38776,#22387,#22388);
#18487=AXIS2_PLACEMENT_3D('',#38779,#22389,#22390);
#18488=AXIS2_PLACEMENT_3D('',#38925,#22392,#22393);
#18489=AXIS2_PLACEMENT_3D('',#39071,#22395,#22396);
#18490=AXIS2_PLACEMENT_3D('',#39217,#22398,#22399);
#18491=AXIS2_PLACEMENT_3D('',#39363,#22401,#22402);
#18492=AXIS2_PLACEMENT_3D('',#39509,#22404,#22405);
#18493=AXIS2_PLACEMENT_3D('',#39655,#22407,#22408);
#18494=AXIS2_PLACEMENT_3D('',#39801,#22410,#22411);
#18495=AXIS2_PLACEMENT_3D('',#39947,#22413,#22414);
#18496=AXIS2_PLACEMENT_3D('',#40093,#22416,#22417);
#18497=AXIS2_PLACEMENT_3D('',#40239,#22419,#22420);
#18498=AXIS2_PLACEMENT_3D('',#40385,#22422,#22423);
#18499=AXIS2_PLACEMENT_3D('',#40531,#22425,#22426);
#18500=AXIS2_PLACEMENT_3D('',#40677,#22428,#22429);
#18501=AXIS2_PLACEMENT_3D('',#40823,#22431,#22432);
#18502=AXIS2_PLACEMENT_3D('',#40969,#22434,#22435);
#18503=AXIS2_PLACEMENT_3D('',#41115,#22437,#22438);
#18504=AXIS2_PLACEMENT_3D('',#41261,#22440,#22441);
#18505=AXIS2_PLACEMENT_3D('',#41407,#22443,#22444);
#18506=AXIS2_PLACEMENT_3D('',#41553,#22446,#22447);
#18507=AXIS2_PLACEMENT_3D('',#41699,#22449,#22450);
#18508=AXIS2_PLACEMENT_3D('',#41845,#22452,#22453);
#18509=AXIS2_PLACEMENT_3D('',#41991,#22455,#22456);
#18510=AXIS2_PLACEMENT_3D('',#42137,#22458,#22459);
#18511=AXIS2_PLACEMENT_3D('',#42283,#22461,#22462);
#18512=AXIS2_PLACEMENT_3D('',#42429,#22464,#22465);
#18513=AXIS2_PLACEMENT_3D('',#42575,#22467,#22468);
#18514=AXIS2_PLACEMENT_3D('',#42721,#22470,#22471);
#18515=AXIS2_PLACEMENT_3D('',#42867,#22473,#22474);
#18516=AXIS2_PLACEMENT_3D('',#43013,#22476,#22477);
#18517=AXIS2_PLACEMENT_3D('',#43159,#22479,#22480);
#18518=AXIS2_PLACEMENT_3D('',#43305,#22482,#22483);
#18519=AXIS2_PLACEMENT_3D('',#43451,#22485,#22486);
#18520=AXIS2_PLACEMENT_3D('',#43597,#22488,#22489);
#18521=AXIS2_PLACEMENT_3D('',#43743,#22491,#22492);
#18522=AXIS2_PLACEMENT_3D('',#43889,#22494,#22495);
#18523=AXIS2_PLACEMENT_3D('',#44035,#22497,#22498);
#18524=AXIS2_PLACEMENT_3D('',#44181,#22500,#22501);
#18525=AXIS2_PLACEMENT_3D('',#44327,#22503,#22504);
#18526=AXIS2_PLACEMENT_3D('',#44473,#22506,#22507);
#18527=AXIS2_PLACEMENT_3D('',#44617,#22509,#22510);
#18528=AXIS2_PLACEMENT_3D('',#44618,#22511,#22512);
#18529=AXIS2_PLACEMENT_3D('',#44619,#22513,#22514);
#18530=AXIS2_PLACEMENT_3D('',#44620,#22515,#22516);
#18531=AXIS2_PLACEMENT_3D('',#44622,#22517,#22518);
#18532=AXIS2_PLACEMENT_3D('',#44625,#22520,#22521);
#18533=AXIS2_PLACEMENT_3D('',#44626,#22522,#22523);
#18534=AXIS2_PLACEMENT_3D('',#45065,#22526,#22527);
#18535=AXIS2_PLACEMENT_3D('',#45067,#22529,#22530);
#18536=AXIS2_PLACEMENT_3D('',#45069,#22531,#22532);
#18537=AXIS2_PLACEMENT_3D('',#45507,#22535,#22536);
#18538=AXIS2_PLACEMENT_3D('',#45509,#22538,#22539);
#18539=AXIS2_PLACEMENT_3D('',#45511,#22540,#22541);
#18540=AXIS2_PLACEMENT_3D('',#45949,#22544,#22545);
#18541=AXIS2_PLACEMENT_3D('',#45951,#22547,#22548);
#18542=AXIS2_PLACEMENT_3D('',#45953,#22549,#22550);
#18543=AXIS2_PLACEMENT_3D('',#46391,#22553,#22554);
#18544=AXIS2_PLACEMENT_3D('',#46393,#22556,#22557);
#18545=AXIS2_PLACEMENT_3D('',#46395,#22558,#22559);
#18546=AXIS2_PLACEMENT_3D('',#46833,#22562,#22563);
#18547=AXIS2_PLACEMENT_3D('',#46835,#22565,#22566);
#18548=AXIS2_PLACEMENT_3D('',#46837,#22567,#22568);
#18549=AXIS2_PLACEMENT_3D('',#47275,#22571,#22572);
#18550=AXIS2_PLACEMENT_3D('',#47277,#22574,#22575);
#18551=AXIS2_PLACEMENT_3D('',#47279,#22576,#22577);
#18552=AXIS2_PLACEMENT_3D('',#47717,#22580,#22581);
#18553=AXIS2_PLACEMENT_3D('',#47719,#22583,#22584);
#18554=AXIS2_PLACEMENT_3D('',#47721,#22585,#22586);
#18555=AXIS2_PLACEMENT_3D('',#48159,#22589,#22590);
#18556=AXIS2_PLACEMENT_3D('',#48161,#22592,#22593);
#18557=AXIS2_PLACEMENT_3D('',#48163,#22594,#22595);
#18558=AXIS2_PLACEMENT_3D('',#48601,#22598,#22599);
#18559=AXIS2_PLACEMENT_3D('',#48603,#22601,#22602);
#18560=AXIS2_PLACEMENT_3D('',#48605,#22603,#22604);
#18561=AXIS2_PLACEMENT_3D('',#49043,#22607,#22608);
#18562=AXIS2_PLACEMENT_3D('',#49045,#22610,#22611);
#18563=AXIS2_PLACEMENT_3D('',#49047,#22612,#22613);
#18564=AXIS2_PLACEMENT_3D('',#49485,#22616,#22617);
#18565=AXIS2_PLACEMENT_3D('',#49487,#22619,#22620);
#18566=AXIS2_PLACEMENT_3D('',#49489,#22621,#22622);
#18567=AXIS2_PLACEMENT_3D('',#49927,#22625,#22626);
#18568=AXIS2_PLACEMENT_3D('',#49929,#22628,#22629);
#18569=AXIS2_PLACEMENT_3D('',#49931,#22630,#22631);
#18570=AXIS2_PLACEMENT_3D('',#50369,#22634,#22635);
#18571=AXIS2_PLACEMENT_3D('',#50371,#22637,#22638);
#18572=AXIS2_PLACEMENT_3D('',#50373,#22639,#22640);
#18573=AXIS2_PLACEMENT_3D('',#50811,#22643,#22644);
#18574=AXIS2_PLACEMENT_3D('',#50813,#22646,#22647);
#18575=AXIS2_PLACEMENT_3D('',#50815,#22648,#22649);
#18576=AXIS2_PLACEMENT_3D('',#51253,#22652,#22653);
#18577=AXIS2_PLACEMENT_3D('',#51255,#22655,#22656);
#18578=AXIS2_PLACEMENT_3D('',#51257,#22657,#22658);
#18579=AXIS2_PLACEMENT_3D('',#51695,#22661,#22662);
#18580=AXIS2_PLACEMENT_3D('',#51697,#22664,#22665);
#18581=AXIS2_PLACEMENT_3D('',#51699,#22666,#22667);
#18582=AXIS2_PLACEMENT_3D('',#52137,#22670,#22671);
#18583=AXIS2_PLACEMENT_3D('',#52139,#22673,#22674);
#18584=AXIS2_PLACEMENT_3D('',#52141,#22675,#22676);
#18585=AXIS2_PLACEMENT_3D('',#52579,#22679,#22680);
#18586=AXIS2_PLACEMENT_3D('',#52581,#22682,#22683);
#18587=AXIS2_PLACEMENT_3D('',#52583,#22684,#22685);
#18588=AXIS2_PLACEMENT_3D('',#53021,#22688,#22689);
#18589=AXIS2_PLACEMENT_3D('',#53023,#22691,#22692);
#18590=AXIS2_PLACEMENT_3D('',#53025,#22693,#22694);
#18591=AXIS2_PLACEMENT_3D('',#53463,#22697,#22698);
#18592=AXIS2_PLACEMENT_3D('',#53465,#22700,#22701);
#18593=AXIS2_PLACEMENT_3D('',#53467,#22702,#22703);
#18594=AXIS2_PLACEMENT_3D('',#53905,#22706,#22707);
#18595=AXIS2_PLACEMENT_3D('',#53907,#22709,#22710);
#18596=AXIS2_PLACEMENT_3D('',#53909,#22711,#22712);
#18597=AXIS2_PLACEMENT_3D('',#54347,#22715,#22716);
#18598=AXIS2_PLACEMENT_3D('',#54349,#22718,#22719);
#18599=AXIS2_PLACEMENT_3D('',#54351,#22720,#22721);
#18600=AXIS2_PLACEMENT_3D('',#54789,#22724,#22725);
#18601=AXIS2_PLACEMENT_3D('',#54791,#22727,#22728);
#18602=AXIS2_PLACEMENT_3D('',#54793,#22729,#22730);
#18603=AXIS2_PLACEMENT_3D('',#55231,#22733,#22734);
#18604=AXIS2_PLACEMENT_3D('',#55233,#22736,#22737);
#18605=AXIS2_PLACEMENT_3D('',#55235,#22738,#22739);
#18606=AXIS2_PLACEMENT_3D('',#55673,#22742,#22743);
#18607=AXIS2_PLACEMENT_3D('',#55675,#22745,#22746);
#18608=AXIS2_PLACEMENT_3D('',#55677,#22747,#22748);
#18609=AXIS2_PLACEMENT_3D('',#56115,#22751,#22752);
#18610=AXIS2_PLACEMENT_3D('',#56117,#22754,#22755);
#18611=AXIS2_PLACEMENT_3D('',#56119,#22756,#22757);
#18612=AXIS2_PLACEMENT_3D('',#56557,#22760,#22761);
#18613=AXIS2_PLACEMENT_3D('',#56559,#22763,#22764);
#18614=AXIS2_PLACEMENT_3D('',#56561,#22765,#22766);
#18615=AXIS2_PLACEMENT_3D('',#56999,#22769,#22770);
#18616=AXIS2_PLACEMENT_3D('',#57001,#22772,#22773);
#18617=AXIS2_PLACEMENT_3D('',#57003,#22774,#22775);
#18618=AXIS2_PLACEMENT_3D('',#57441,#22778,#22779);
#18619=AXIS2_PLACEMENT_3D('',#57443,#22781,#22782);
#18620=AXIS2_PLACEMENT_3D('',#57445,#22783,#22784);
#18621=AXIS2_PLACEMENT_3D('',#57883,#22787,#22788);
#18622=AXIS2_PLACEMENT_3D('',#57885,#22790,#22791);
#18623=AXIS2_PLACEMENT_3D('',#57887,#22792,#22793);
#18624=AXIS2_PLACEMENT_3D('',#58325,#22796,#22797);
#18625=AXIS2_PLACEMENT_3D('',#58327,#22799,#22800);
#18626=AXIS2_PLACEMENT_3D('',#58329,#22801,#22802);
#18627=AXIS2_PLACEMENT_3D('',#58767,#22805,#22806);
#18628=AXIS2_PLACEMENT_3D('',#58769,#22808,#22809);
#18629=AXIS2_PLACEMENT_3D('',#58771,#22810,#22811);
#18630=AXIS2_PLACEMENT_3D('',#59209,#22814,#22815);
#18631=AXIS2_PLACEMENT_3D('',#59211,#22817,#22818);
#18632=AXIS2_PLACEMENT_3D('',#59213,#22819,#22820);
#18633=AXIS2_PLACEMENT_3D('',#59651,#22823,#22824);
#18634=AXIS2_PLACEMENT_3D('',#59653,#22826,#22827);
#18635=AXIS2_PLACEMENT_3D('',#59655,#22828,#22829);
#18636=AXIS2_PLACEMENT_3D('',#60093,#22832,#22833);
#18637=AXIS2_PLACEMENT_3D('',#60095,#22835,#22836);
#18638=AXIS2_PLACEMENT_3D('',#60097,#22837,#22838);
#18639=AXIS2_PLACEMENT_3D('',#60535,#22841,#22842);
#18640=AXIS2_PLACEMENT_3D('',#60537,#22844,#22845);
#18641=AXIS2_PLACEMENT_3D('',#60539,#22846,#22847);
#18642=AXIS2_PLACEMENT_3D('',#60977,#22850,#22851);
#18643=AXIS2_PLACEMENT_3D('',#60979,#22853,#22854);
#18644=AXIS2_PLACEMENT_3D('',#60981,#22855,#22856);
#18645=AXIS2_PLACEMENT_3D('',#61419,#22859,#22860);
#18646=AXIS2_PLACEMENT_3D('',#61421,#22862,#22863);
#18647=AXIS2_PLACEMENT_3D('',#61423,#22864,#22865);
#18648=AXIS2_PLACEMENT_3D('',#61642,#22867,#22868);
#18649=AXIS2_PLACEMENT_3D('',#61863,#22871,#22872);
#18650=AXIS2_PLACEMENT_3D('',#61865,#22873,#22874);
#18651=AXIS2_PLACEMENT_3D('',#62303,#22877,#22878);
#18652=AXIS2_PLACEMENT_3D('',#62305,#22880,#22881);
#18653=AXIS2_PLACEMENT_3D('',#62306,#22882,#22883);
#18654=AXIS2_PLACEMENT_3D('',#62307,#22884,#22885);
#22369=DIRECTION('axis',(0.,0.,1.));
#22370=DIRECTION('refdir',(1.,0.,0.));
#22371=DIRECTION('center_axis',(1.,0.,0.));
#22372=DIRECTION('ref_axis',(0.,0.,-1.));
#22373=DIRECTION('',(0.,0.,1.));
#22374=DIRECTION('',(0.,1.,0.));
#22375=DIRECTION('',(0.,0.,-1.));
#22376=DIRECTION('',(0.,-1.,0.));
#22377=DIRECTION('center_axis',(0.,0.,-1.));
#22378=DIRECTION('ref_axis',(-1.,0.,0.));
#22379=DIRECTION('',(1.,0.,0.));
#22380=DIRECTION('',(0.,-1.,0.));
#22381=DIRECTION('',(-1.,0.,0.));
#22382=DIRECTION('center_axis',(-1.,0.,0.));
#22383=DIRECTION('ref_axis',(0.,0.,1.));
#22384=DIRECTION('',(0.,0.,-1.));
#22385=DIRECTION('',(0.,1.,0.));
#22386=DIRECTION('',(0.,0.,1.));
#22387=DIRECTION('center_axis',(0.,1.,0.));
#22388=DIRECTION('ref_axis',(1.,0.,0.));
#22389=DIRECTION('center_axis',(0.,-1.,0.));
#22390=DIRECTION('ref_axis',(1.,0.,0.));
#22391=DIRECTION('',(-0.309016994374948,0.,0.951056516295154));
#22392=DIRECTION('center_axis',(0.,-1.,0.));
#22393=DIRECTION('ref_axis',(1.,0.,0.));
#22394=DIRECTION('',(-0.453990499739547,0.,0.891006524188368));
#22395=DIRECTION('center_axis',(0.,-1.,0.));
#22396=DIRECTION('ref_axis',(1.,0.,0.));
#22397=DIRECTION('',(-0.587785252292473,0.,0.809016994374947));
#22398=DIRECTION('center_axis',(0.,-1.,0.));
#22399=DIRECTION('ref_axis',(1.,0.,0.));
#22400=DIRECTION('',(-0.707106781186548,0.,0.707106781186547));
#22401=DIRECTION('center_axis',(0.,-1.,0.));
#22402=DIRECTION('ref_axis',(1.,0.,0.));
#22403=DIRECTION('',(-0.809016994374948,0.,0.587785252292473));
#22404=DIRECTION('center_axis',(0.,-1.,0.));
#22405=DIRECTION('ref_axis',(1.,0.,0.));
#22406=DIRECTION('',(-0.891006524188368,0.,0.453990499739547));
#22407=DIRECTION('center_axis',(0.,-1.,0.));
#22408=DIRECTION('ref_axis',(1.,0.,0.));
#22409=DIRECTION('',(-0.951056516295154,0.,0.309016994374947));
#22410=DIRECTION('center_axis',(0.,-1.,0.));
#22411=DIRECTION('ref_axis',(1.,0.,0.));
#22412=DIRECTION('',(-0.987688340595138,0.,0.156434465040231));
#22413=DIRECTION('center_axis',(0.,-1.,0.));
#22414=DIRECTION('ref_axis',(1.,0.,0.));
#22415=DIRECTION('',(-1.,0.,-1.83697019872103E-16));
#22416=DIRECTION('center_axis',(0.,-1.,0.));
#22417=DIRECTION('ref_axis',(1.,0.,0.));
#22418=DIRECTION('',(-0.987688340595138,0.,-0.156434465040231));
#22419=DIRECTION('center_axis',(0.,-1.,0.));
#22420=DIRECTION('ref_axis',(1.,0.,0.));
#22421=DIRECTION('',(-0.951056516295154,0.,-0.309016994374948));
#22422=DIRECTION('center_axis',(0.,-1.,0.));
#22423=DIRECTION('ref_axis',(1.,0.,0.));
#22424=DIRECTION('',(-0.891006524188368,0.,-0.453990499739547));
#22425=DIRECTION('center_axis',(0.,-1.,0.));
#22426=DIRECTION('ref_axis',(1.,0.,0.));
#22427=DIRECTION('',(-0.809016994374947,0.,-0.587785252292473));
#22428=DIRECTION('center_axis',(0.,-1.,0.));
#22429=DIRECTION('ref_axis',(1.,0.,0.));
#22430=DIRECTION('',(-0.707106781186547,0.,-0.707106781186548));
#22431=DIRECTION('center_axis',(0.,-1.,0.));
#22432=DIRECTION('ref_axis',(1.,0.,0.));
#22433=DIRECTION('',(-0.587785252292473,0.,-0.809016994374948));
#22434=DIRECTION('center_axis',(0.,-1.,0.));
#22435=DIRECTION('ref_axis',(1.,0.,0.));
#22436=DIRECTION('',(-0.453990499739547,0.,-0.891006524188368));
#22437=DIRECTION('center_axis',(0.,-1.,0.));
#22438=DIRECTION('ref_axis',(1.,0.,0.));
#22439=DIRECTION('',(-0.309016994374947,0.,-0.951056516295154));
#22440=DIRECTION('center_axis',(0.,-1.,0.));
#22441=DIRECTION('ref_axis',(1.,0.,0.));
#22442=DIRECTION('',(-0.156434465040231,0.,-0.987688340595138));
#22443=DIRECTION('center_axis',(0.,-1.,0.));
#22444=DIRECTION('ref_axis',(1.,0.,0.));
#22445=DIRECTION('',(1.22464679914735E-16,0.,-1.));
#22446=DIRECTION('center_axis',(0.,-1.,0.));
#22447=DIRECTION('ref_axis',(1.,0.,0.));
#22448=DIRECTION('',(0.156434465040231,0.,-0.987688340595138));
#22449=DIRECTION('center_axis',(0.,-1.,0.));
#22450=DIRECTION('ref_axis',(1.,0.,0.));
#22451=DIRECTION('',(0.309016994374948,0.,-0.951056516295154));
#22452=DIRECTION('center_axis',(0.,-1.,0.));
#22453=DIRECTION('ref_axis',(1.,0.,0.));
#22454=DIRECTION('',(0.453990499739547,0.,-0.891006524188368));
#22455=DIRECTION('center_axis',(0.,-1.,0.));
#22456=DIRECTION('ref_axis',(1.,0.,0.));
#22457=DIRECTION('',(0.587785252292473,0.,-0.809016994374947));
#22458=DIRECTION('center_axis',(0.,-1.,0.));
#22459=DIRECTION('ref_axis',(1.,0.,0.));
#22460=DIRECTION('',(0.707106781186548,0.,-0.707106781186547));
#22461=DIRECTION('center_axis',(0.,-1.,0.));
#22462=DIRECTION('ref_axis',(1.,0.,0.));
#22463=DIRECTION('',(0.809016994374948,0.,-0.587785252292473));
#22464=DIRECTION('center_axis',(0.,-1.,0.));
#22465=DIRECTION('ref_axis',(1.,0.,0.));
#22466=DIRECTION('',(0.891006524188368,0.,-0.453990499739547));
#22467=DIRECTION('center_axis',(0.,-1.,0.));
#22468=DIRECTION('ref_axis',(1.,0.,0.));
#22469=DIRECTION('',(0.951056516295154,0.,-0.309016994374947));
#22470=DIRECTION('center_axis',(0.,-1.,0.));
#22471=DIRECTION('ref_axis',(1.,0.,0.));
#22472=DIRECTION('',(0.987688340595138,0.,-0.156434465040231));
#22473=DIRECTION('center_axis',(0.,-1.,0.));
#22474=DIRECTION('ref_axis',(1.,0.,0.));
#22475=DIRECTION('',(1.,0.,6.12323399573677E-17));
#22476=DIRECTION('center_axis',(0.,-1.,0.));
#22477=DIRECTION('ref_axis',(1.,0.,0.));
#22478=DIRECTION('',(0.987688340595138,0.,0.156434465040231));
#22479=DIRECTION('center_axis',(0.,-1.,0.));
#22480=DIRECTION('ref_axis',(1.,0.,0.));
#22481=DIRECTION('',(0.951056516295154,0.,0.309016994374948));
#22482=DIRECTION('center_axis',(0.,-1.,0.));
#22483=DIRECTION('ref_axis',(1.,0.,0.));
#22484=DIRECTION('',(0.891006524188368,0.,0.453990499739547));
#22485=DIRECTION('center_axis',(0.,-1.,0.));
#22486=DIRECTION('ref_axis',(1.,0.,0.));
#22487=DIRECTION('',(0.809016994374947,0.,0.587785252292473));
#22488=DIRECTION('center_axis',(0.,-1.,0.));
#22489=DIRECTION('ref_axis',(1.,0.,0.));
#22490=DIRECTION('',(0.707106781186547,0.,0.707106781186548));
#22491=DIRECTION('center_axis',(0.,-1.,0.));
#22492=DIRECTION('ref_axis',(1.,0.,0.));
#22493=DIRECTION('',(0.587785252292473,0.,0.809016994374947));
#22494=DIRECTION('center_axis',(0.,-1.,0.));
#22495=DIRECTION('ref_axis',(1.,0.,0.));
#22496=DIRECTION('',(0.453990499739547,0.,0.891006524188368));
#22497=DIRECTION('center_axis',(0.,-1.,0.));
#22498=DIRECTION('ref_axis',(1.,0.,0.));
#22499=DIRECTION('',(0.309016994374947,0.,0.951056516295154));
#22500=DIRECTION('center_axis',(0.,-1.,0.));
#22501=DIRECTION('ref_axis',(1.,0.,0.));
#22502=DIRECTION('',(0.156434465040231,0.,0.987688340595138));
#22503=DIRECTION('center_axis',(0.,-1.,0.));
#22504=DIRECTION('ref_axis',(1.,0.,0.));
#22505=DIRECTION('',(0.,0.,1.));
#22506=DIRECTION('center_axis',(0.,-1.,0.));
#22507=DIRECTION('ref_axis',(1.,0.,0.));
#22508=DIRECTION('',(-0.156434465040231,0.,0.987688340595138));
#22509=DIRECTION('center_axis',(0.,1.,0.));
#22510=DIRECTION('ref_axis',(1.,0.,0.));
#22511=DIRECTION('center_axis',(0.,1.,0.));
#22512=DIRECTION('ref_axis',(6.12323399573677E-17,0.,1.));
#22513=DIRECTION('center_axis',(0.,-1.,0.));
#22514=DIRECTION('ref_axis',(1.,0.,0.));
#22515=DIRECTION('center_axis',(0.,1.,0.));
#22516=DIRECTION('ref_axis',(1.,0.,0.));
#22517=DIRECTION('center_axis',(0.,1.,0.));
#22518=DIRECTION('ref_axis',(1.,0.,0.));
#22519=DIRECTION('',(0.,-1.,0.));
#22520=DIRECTION('center_axis',(0.,-1.,0.));
#22521=DIRECTION('ref_axis',(1.,0.,0.));
#22522=DIRECTION('center_axis',(0.,1.,0.));
#22523=DIRECTION('ref_axis',(1.,0.,0.));
#22524=DIRECTION('',(0.,1.,0.));
#22525=DIRECTION('',(0.,1.,0.));
#22526=DIRECTION('center_axis',(0.987688340595138,0.,0.156434465040231));
#22527=DIRECTION('ref_axis',(0.156434465040231,0.,-0.987688340595138));
#22528=DIRECTION('',(0.156434465040231,0.,-0.987688340595138));
#22529=DIRECTION('center_axis',(0.,1.,0.));
#22530=DIRECTION('ref_axis',(1.,0.,0.));
#22531=DIRECTION('center_axis',(0.,1.,0.));
#22532=DIRECTION('ref_axis',(1.,0.,0.));
#22533=DIRECTION('',(0.,1.,0.));
#22534=DIRECTION('',(0.,1.,0.));
#22535=DIRECTION('center_axis',(0.951056516295154,0.,0.309016994374948));
#22536=DIRECTION('ref_axis',(0.309016994374948,0.,-0.951056516295154));
#22537=DIRECTION('',(0.309016994374948,0.,-0.951056516295154));
#22538=DIRECTION('center_axis',(0.,1.,0.));
#22539=DIRECTION('ref_axis',(1.,0.,0.));
#22540=DIRECTION('center_axis',(0.,1.,0.));
#22541=DIRECTION('ref_axis',(1.,0.,0.));
#22542=DIRECTION('',(0.,1.,0.));
#22543=DIRECTION('',(0.,1.,0.));
#22544=DIRECTION('center_axis',(0.891006524188368,0.,0.453990499739547));
#22545=DIRECTION('ref_axis',(0.453990499739547,0.,-0.891006524188368));
#22546=DIRECTION('',(0.453990499739547,0.,-0.891006524188368));
#22547=DIRECTION('center_axis',(0.,1.,0.));
#22548=DIRECTION('ref_axis',(1.,0.,0.));
#22549=DIRECTION('center_axis',(0.,1.,0.));
#22550=DIRECTION('ref_axis',(1.,0.,0.));
#22551=DIRECTION('',(0.,1.,0.));
#22552=DIRECTION('',(0.,1.,0.));
#22553=DIRECTION('center_axis',(0.809016994374947,0.,0.587785252292473));
#22554=DIRECTION('ref_axis',(0.587785252292473,0.,-0.809016994374947));
#22555=DIRECTION('',(0.587785252292473,0.,-0.809016994374947));
#22556=DIRECTION('center_axis',(0.,1.,0.));
#22557=DIRECTION('ref_axis',(1.,0.,0.));
#22558=DIRECTION('center_axis',(0.,1.,0.));
#22559=DIRECTION('ref_axis',(1.,0.,0.));
#22560=DIRECTION('',(0.,1.,0.));
#22561=DIRECTION('',(0.,1.,0.));
#22562=DIRECTION('center_axis',(0.707106781186547,0.,0.707106781186548));
#22563=DIRECTION('ref_axis',(0.707106781186548,0.,-0.707106781186547));
#22564=DIRECTION('',(0.707106781186548,0.,-0.707106781186547));
#22565=DIRECTION('center_axis',(0.,1.,0.));
#22566=DIRECTION('ref_axis',(1.,0.,0.));
#22567=DIRECTION('center_axis',(0.,1.,0.));
#22568=DIRECTION('ref_axis',(1.,0.,0.));
#22569=DIRECTION('',(0.,1.,0.));
#22570=DIRECTION('',(0.,1.,0.));
#22571=DIRECTION('center_axis',(0.587785252292473,0.,0.809016994374948));
#22572=DIRECTION('ref_axis',(0.809016994374948,0.,-0.587785252292473));
#22573=DIRECTION('',(0.809016994374948,0.,-0.587785252292473));
#22574=DIRECTION('center_axis',(0.,1.,0.));
#22575=DIRECTION('ref_axis',(1.,0.,0.));
#22576=DIRECTION('center_axis',(0.,1.,0.));
#22577=DIRECTION('ref_axis',(1.,0.,0.));
#22578=DIRECTION('',(0.,1.,0.));
#22579=DIRECTION('',(0.,1.,0.));
#22580=DIRECTION('center_axis',(0.453990499739547,0.,0.891006524188368));
#22581=DIRECTION('ref_axis',(0.891006524188368,0.,-0.453990499739547));
#22582=DIRECTION('',(0.891006524188368,0.,-0.453990499739547));
#22583=DIRECTION('center_axis',(0.,1.,0.));
#22584=DIRECTION('ref_axis',(1.,0.,0.));
#22585=DIRECTION('center_axis',(0.,1.,0.));
#22586=DIRECTION('ref_axis',(1.,0.,0.));
#22587=DIRECTION('',(0.,1.,0.));
#22588=DIRECTION('',(0.,1.,0.));
#22589=DIRECTION('center_axis',(0.309016994374947,0.,0.951056516295154));
#22590=DIRECTION('ref_axis',(0.951056516295154,0.,-0.309016994374947));
#22591=DIRECTION('',(0.951056516295154,0.,-0.309016994374947));
#22592=DIRECTION('center_axis',(0.,1.,0.));
#22593=DIRECTION('ref_axis',(1.,0.,0.));
#22594=DIRECTION('center_axis',(0.,1.,0.));
#22595=DIRECTION('ref_axis',(1.,0.,0.));
#22596=DIRECTION('',(0.,1.,0.));
#22597=DIRECTION('',(0.,1.,0.));
#22598=DIRECTION('center_axis',(0.156434465040231,0.,0.987688340595138));
#22599=DIRECTION('ref_axis',(0.987688340595138,0.,-0.156434465040231));
#22600=DIRECTION('',(0.987688340595138,0.,-0.156434465040231));
#22601=DIRECTION('center_axis',(0.,1.,0.));
#22602=DIRECTION('ref_axis',(1.,0.,0.));
#22603=DIRECTION('center_axis',(0.,1.,0.));
#22604=DIRECTION('ref_axis',(1.,0.,0.));
#22605=DIRECTION('',(0.,1.,0.));
#22606=DIRECTION('',(0.,1.,0.));
#22607=DIRECTION('center_axis',(-1.83697019872103E-16,0.,1.));
#22608=DIRECTION('ref_axis',(1.,0.,1.83697019872103E-16));
#22609=DIRECTION('',(1.,0.,1.83697019872103E-16));
#22610=DIRECTION('center_axis',(0.,1.,0.));
#22611=DIRECTION('ref_axis',(1.,0.,0.));
#22612=DIRECTION('center_axis',(0.,1.,0.));
#22613=DIRECTION('ref_axis',(1.,0.,0.));
#22614=DIRECTION('',(0.,1.,0.));
#22615=DIRECTION('',(0.,1.,0.));
#22616=DIRECTION('center_axis',(-0.156434465040231,0.,0.987688340595138));
#22617=DIRECTION('ref_axis',(0.987688340595138,0.,0.156434465040231));
#22618=DIRECTION('',(0.987688340595138,0.,0.156434465040231));
#22619=DIRECTION('center_axis',(0.,1.,0.));
#22620=DIRECTION('ref_axis',(1.,0.,0.));
#22621=DIRECTION('center_axis',(0.,1.,0.));
#22622=DIRECTION('ref_axis',(1.,0.,0.));
#22623=DIRECTION('',(0.,1.,0.));
#22624=DIRECTION('',(0.,1.,0.));
#22625=DIRECTION('center_axis',(-0.309016994374948,0.,0.951056516295154));
#22626=DIRECTION('ref_axis',(0.951056516295154,0.,0.309016994374948));
#22627=DIRECTION('',(0.951056516295154,0.,0.309016994374948));
#22628=DIRECTION('center_axis',(0.,1.,0.));
#22629=DIRECTION('ref_axis',(1.,0.,0.));
#22630=DIRECTION('center_axis',(0.,1.,0.));
#22631=DIRECTION('ref_axis',(1.,0.,0.));
#22632=DIRECTION('',(0.,1.,0.));
#22633=DIRECTION('',(0.,1.,0.));
#22634=DIRECTION('center_axis',(-0.453990499739547,0.,0.891006524188368));
#22635=DIRECTION('ref_axis',(0.891006524188368,0.,0.453990499739547));
#22636=DIRECTION('',(0.891006524188368,0.,0.453990499739547));
#22637=DIRECTION('center_axis',(0.,1.,0.));
#22638=DIRECTION('ref_axis',(1.,0.,0.));
#22639=DIRECTION('center_axis',(0.,1.,0.));
#22640=DIRECTION('ref_axis',(1.,0.,0.));
#22641=DIRECTION('',(0.,1.,0.));
#22642=DIRECTION('',(0.,1.,0.));
#22643=DIRECTION('center_axis',(-0.587785252292473,0.,0.809016994374947));
#22644=DIRECTION('ref_axis',(0.809016994374947,0.,0.587785252292473));
#22645=DIRECTION('',(0.809016994374947,0.,0.587785252292473));
#22646=DIRECTION('center_axis',(0.,1.,0.));
#22647=DIRECTION('ref_axis',(1.,0.,0.));
#22648=DIRECTION('center_axis',(0.,1.,0.));
#22649=DIRECTION('ref_axis',(1.,0.,0.));
#22650=DIRECTION('',(0.,1.,0.));
#22651=DIRECTION('',(0.,1.,0.));
#22652=DIRECTION('center_axis',(-0.707106781186548,0.,0.707106781186547));
#22653=DIRECTION('ref_axis',(0.707106781186547,0.,0.707106781186548));
#22654=DIRECTION('',(0.707106781186547,0.,0.707106781186548));
#22655=DIRECTION('center_axis',(0.,1.,0.));
#22656=DIRECTION('ref_axis',(1.,0.,0.));
#22657=DIRECTION('center_axis',(0.,1.,0.));
#22658=DIRECTION('ref_axis',(1.,0.,0.));
#22659=DIRECTION('',(0.,1.,0.));
#22660=DIRECTION('',(0.,1.,0.));
#22661=DIRECTION('center_axis',(-0.809016994374948,0.,0.587785252292473));
#22662=DIRECTION('ref_axis',(0.587785252292473,0.,0.809016994374948));
#22663=DIRECTION('',(0.587785252292473,0.,0.809016994374948));
#22664=DIRECTION('center_axis',(0.,1.,0.));
#22665=DIRECTION('ref_axis',(1.,0.,0.));
#22666=DIRECTION('center_axis',(0.,1.,0.));
#22667=DIRECTION('ref_axis',(1.,0.,0.));
#22668=DIRECTION('',(0.,1.,0.));
#22669=DIRECTION('',(0.,1.,0.));
#22670=DIRECTION('center_axis',(-0.891006524188368,0.,0.453990499739547));
#22671=DIRECTION('ref_axis',(0.453990499739547,0.,0.891006524188368));
#22672=DIRECTION('',(0.453990499739547,0.,0.891006524188368));
#22673=DIRECTION('center_axis',(0.,1.,0.));
#22674=DIRECTION('ref_axis',(1.,0.,0.));
#22675=DIRECTION('center_axis',(0.,1.,0.));
#22676=DIRECTION('ref_axis',(1.,0.,0.));
#22677=DIRECTION('',(0.,1.,0.));
#22678=DIRECTION('',(0.,1.,0.));
#22679=DIRECTION('center_axis',(-0.951056516295154,0.,0.309016994374947));
#22680=DIRECTION('ref_axis',(0.309016994374947,0.,0.951056516295154));
#22681=DIRECTION('',(0.309016994374947,0.,0.951056516295154));
#22682=DIRECTION('center_axis',(0.,1.,0.));
#22683=DIRECTION('ref_axis',(1.,0.,0.));
#22684=DIRECTION('center_axis',(0.,1.,0.));
#22685=DIRECTION('ref_axis',(1.,0.,0.));
#22686=DIRECTION('',(0.,1.,0.));
#22687=DIRECTION('',(0.,1.,0.));
#22688=DIRECTION('center_axis',(-0.987688340595138,0.,0.156434465040231));
#22689=DIRECTION('ref_axis',(0.156434465040231,0.,0.987688340595138));
#22690=DIRECTION('',(0.156434465040231,0.,0.987688340595138));
#22691=DIRECTION('center_axis',(0.,1.,0.));
#22692=DIRECTION('ref_axis',(1.,0.,0.));
#22693=DIRECTION('center_axis',(0.,1.,0.));
#22694=DIRECTION('ref_axis',(1.,0.,0.));
#22695=DIRECTION('',(0.,1.,0.));
#22696=DIRECTION('',(0.,1.,0.));
#22697=DIRECTION('center_axis',(-1.,0.,-1.22464679914735E-16));
#22698=DIRECTION('ref_axis',(-1.22464679914735E-16,0.,1.));
#22699=DIRECTION('',(-1.22464679914735E-16,0.,1.));
#22700=DIRECTION('center_axis',(0.,1.,0.));
#22701=DIRECTION('ref_axis',(1.,0.,0.));
#22702=DIRECTION('center_axis',(0.,1.,0.));
#22703=DIRECTION('ref_axis',(1.,0.,0.));
#22704=DIRECTION('',(0.,1.,0.));
#22705=DIRECTION('',(0.,1.,0.));
#22706=DIRECTION('center_axis',(-0.987688340595138,0.,-0.156434465040231));
#22707=DIRECTION('ref_axis',(-0.156434465040231,0.,0.987688340595138));
#22708=DIRECTION('',(-0.156434465040231,0.,0.987688340595138));
#22709=DIRECTION('center_axis',(0.,1.,0.));
#22710=DIRECTION('ref_axis',(1.,0.,0.));
#22711=DIRECTION('center_axis',(0.,1.,0.));
#22712=DIRECTION('ref_axis',(1.,0.,0.));
#22713=DIRECTION('',(0.,1.,0.));
#22714=DIRECTION('',(0.,1.,0.));
#22715=DIRECTION('center_axis',(-0.951056516295154,0.,-0.309016994374948));
#22716=DIRECTION('ref_axis',(-0.309016994374948,0.,0.951056516295154));
#22717=DIRECTION('',(-0.309016994374948,0.,0.951056516295154));
#22718=DIRECTION('center_axis',(0.,1.,0.));
#22719=DIRECTION('ref_axis',(1.,0.,0.));
#22720=DIRECTION('center_axis',(0.,1.,0.));
#22721=DIRECTION('ref_axis',(1.,0.,0.));
#22722=DIRECTION('',(0.,1.,0.));
#22723=DIRECTION('',(0.,1.,0.));
#22724=DIRECTION('center_axis',(-0.891006524188368,0.,-0.453990499739547));
#22725=DIRECTION('ref_axis',(-0.453990499739547,0.,0.891006524188368));
#22726=DIRECTION('',(-0.453990499739547,0.,0.891006524188368));
#22727=DIRECTION('center_axis',(0.,1.,0.));
#22728=DIRECTION('ref_axis',(1.,0.,0.));
#22729=DIRECTION('center_axis',(0.,1.,0.));
#22730=DIRECTION('ref_axis',(1.,0.,0.));
#22731=DIRECTION('',(0.,1.,0.));
#22732=DIRECTION('',(0.,1.,0.));
#22733=DIRECTION('center_axis',(-0.809016994374947,0.,-0.587785252292473));
#22734=DIRECTION('ref_axis',(-0.587785252292473,0.,0.809016994374947));
#22735=DIRECTION('',(-0.587785252292473,0.,0.809016994374947));
#22736=DIRECTION('center_axis',(0.,1.,0.));
#22737=DIRECTION('ref_axis',(1.,0.,0.));
#22738=DIRECTION('center_axis',(0.,1.,0.));
#22739=DIRECTION('ref_axis',(1.,0.,0.));
#22740=DIRECTION('',(0.,1.,0.));
#22741=DIRECTION('',(0.,1.,0.));
#22742=DIRECTION('center_axis',(-0.707106781186547,0.,-0.707106781186548));
#22743=DIRECTION('ref_axis',(-0.707106781186548,0.,0.707106781186547));
#22744=DIRECTION('',(-0.707106781186548,0.,0.707106781186547));
#22745=DIRECTION('center_axis',(0.,1.,0.));
#22746=DIRECTION('ref_axis',(1.,0.,0.));
#22747=DIRECTION('center_axis',(0.,1.,0.));
#22748=DIRECTION('ref_axis',(1.,0.,0.));
#22749=DIRECTION('',(0.,1.,0.));
#22750=DIRECTION('',(0.,1.,0.));
#22751=DIRECTION('center_axis',(-0.587785252292473,0.,-0.809016994374948));
#22752=DIRECTION('ref_axis',(-0.809016994374948,0.,0.587785252292473));
#22753=DIRECTION('',(-0.809016994374948,0.,0.587785252292473));
#22754=DIRECTION('center_axis',(0.,1.,0.));
#22755=DIRECTION('ref_axis',(1.,0.,0.));
#22756=DIRECTION('center_axis',(0.,1.,0.));
#22757=DIRECTION('ref_axis',(1.,0.,0.));
#22758=DIRECTION('',(0.,1.,0.));
#22759=DIRECTION('',(0.,1.,0.));
#22760=DIRECTION('center_axis',(-0.453990499739547,0.,-0.891006524188368));
#22761=DIRECTION('ref_axis',(-0.891006524188368,0.,0.453990499739547));
#22762=DIRECTION('',(-0.891006524188368,0.,0.453990499739547));
#22763=DIRECTION('center_axis',(0.,1.,0.));
#22764=DIRECTION('ref_axis',(1.,0.,0.));
#22765=DIRECTION('center_axis',(0.,1.,0.));
#22766=DIRECTION('ref_axis',(1.,0.,0.));
#22767=DIRECTION('',(0.,1.,0.));
#22768=DIRECTION('',(0.,1.,0.));
#22769=DIRECTION('center_axis',(-0.309016994374947,0.,-0.951056516295154));
#22770=DIRECTION('ref_axis',(-0.951056516295154,0.,0.309016994374947));
#22771=DIRECTION('',(-0.951056516295154,0.,0.309016994374947));
#22772=DIRECTION('center_axis',(0.,1.,0.));
#22773=DIRECTION('ref_axis',(1.,0.,0.));
#22774=DIRECTION('center_axis',(0.,1.,0.));
#22775=DIRECTION('ref_axis',(1.,0.,0.));
#22776=DIRECTION('',(0.,1.,0.));
#22777=DIRECTION('',(0.,1.,0.));
#22778=DIRECTION('center_axis',(-0.156434465040231,0.,-0.987688340595138));
#22779=DIRECTION('ref_axis',(-0.987688340595138,0.,0.156434465040231));
#22780=DIRECTION('',(-0.987688340595138,0.,0.156434465040231));
#22781=DIRECTION('center_axis',(0.,1.,0.));
#22782=DIRECTION('ref_axis',(1.,0.,0.));
#22783=DIRECTION('center_axis',(0.,1.,0.));
#22784=DIRECTION('ref_axis',(1.,0.,0.));
#22785=DIRECTION('',(0.,1.,0.));
#22786=DIRECTION('',(0.,1.,0.));
#22787=DIRECTION('center_axis',(6.12323399573677E-17,0.,-1.));
#22788=DIRECTION('ref_axis',(-1.,0.,-6.12323399573677E-17));
#22789=DIRECTION('',(-1.,0.,-6.12323399573677E-17));
#22790=DIRECTION('center_axis',(0.,1.,0.));
#22791=DIRECTION('ref_axis',(1.,0.,0.));
#22792=DIRECTION('center_axis',(0.,1.,0.));
#22793=DIRECTION('ref_axis',(1.,0.,0.));
#22794=DIRECTION('',(0.,1.,0.));
#22795=DIRECTION('',(0.,1.,0.));
#22796=DIRECTION('center_axis',(0.156434465040231,0.,-0.987688340595138));
#22797=DIRECTION('ref_axis',(-0.987688340595138,0.,-0.156434465040231));
#22798=DIRECTION('',(-0.987688340595138,0.,-0.156434465040231));
#22799=DIRECTION('center_axis',(0.,1.,0.));
#22800=DIRECTION('ref_axis',(1.,0.,0.));
#22801=DIRECTION('center_axis',(0.,1.,0.));
#22802=DIRECTION('ref_axis',(1.,0.,0.));
#22803=DIRECTION('',(0.,1.,0.));
#22804=DIRECTION('',(0.,1.,0.));
#22805=DIRECTION('center_axis',(0.309016994374948,0.,-0.951056516295154));
#22806=DIRECTION('ref_axis',(-0.951056516295154,0.,-0.309016994374948));
#22807=DIRECTION('',(-0.951056516295154,0.,-0.309016994374948));
#22808=DIRECTION('center_axis',(0.,1.,0.));
#22809=DIRECTION('ref_axis',(1.,0.,0.));
#22810=DIRECTION('center_axis',(0.,1.,0.));
#22811=DIRECTION('ref_axis',(1.,0.,0.));
#22812=DIRECTION('',(0.,1.,0.));
#22813=DIRECTION('',(0.,1.,0.));
#22814=DIRECTION('center_axis',(0.453990499739547,0.,-0.891006524188368));
#22815=DIRECTION('ref_axis',(-0.891006524188368,0.,-0.453990499739547));
#22816=DIRECTION('',(-0.891006524188368,0.,-0.453990499739547));
#22817=DIRECTION('center_axis',(0.,1.,0.));
#22818=DIRECTION('ref_axis',(1.,0.,0.));
#22819=DIRECTION('center_axis',(0.,1.,0.));
#22820=DIRECTION('ref_axis',(1.,0.,0.));
#22821=DIRECTION('',(0.,1.,0.));
#22822=DIRECTION('',(0.,1.,0.));
#22823=DIRECTION('center_axis',(0.587785252292473,0.,-0.809016994374947));
#22824=DIRECTION('ref_axis',(-0.809016994374947,0.,-0.587785252292473));
#22825=DIRECTION('',(-0.809016994374947,0.,-0.587785252292473));
#22826=DIRECTION('center_axis',(0.,1.,0.));
#22827=DIRECTION('ref_axis',(1.,0.,0.));
#22828=DIRECTION('center_axis',(0.,1.,0.));
#22829=DIRECTION('ref_axis',(1.,0.,0.));
#22830=DIRECTION('',(0.,1.,0.));
#22831=DIRECTION('',(0.,1.,0.));
#22832=DIRECTION('center_axis',(0.707106781186548,0.,-0.707106781186547));
#22833=DIRECTION('ref_axis',(-0.707106781186547,0.,-0.707106781186548));
#22834=DIRECTION('',(-0.707106781186547,0.,-0.707106781186548));
#22835=DIRECTION('center_axis',(0.,1.,0.));
#22836=DIRECTION('ref_axis',(1.,0.,0.));
#22837=DIRECTION('center_axis',(0.,1.,0.));
#22838=DIRECTION('ref_axis',(1.,0.,0.));
#22839=DIRECTION('',(0.,1.,0.));
#22840=DIRECTION('',(0.,1.,0.));
#22841=DIRECTION('center_axis',(0.809016994374947,0.,-0.587785252292473));
#22842=DIRECTION('ref_axis',(-0.587785252292473,0.,-0.809016994374947));
#22843=DIRECTION('',(-0.587785252292473,0.,-0.809016994374947));
#22844=DIRECTION('center_axis',(0.,1.,0.));
#22845=DIRECTION('ref_axis',(1.,0.,0.));
#22846=DIRECTION('center_axis',(0.,1.,0.));
#22847=DIRECTION('ref_axis',(1.,0.,0.));
#22848=DIRECTION('',(0.,1.,0.));
#22849=DIRECTION('',(0.,1.,0.));
#22850=DIRECTION('center_axis',(0.891006524188368,0.,-0.453990499739547));
#22851=DIRECTION('ref_axis',(-0.453990499739547,0.,-0.891006524188368));
#22852=DIRECTION('',(-0.453990499739547,0.,-0.891006524188368));
#22853=DIRECTION('center_axis',(0.,1.,0.));
#22854=DIRECTION('ref_axis',(1.,0.,0.));
#22855=DIRECTION('center_axis',(0.,1.,0.));
#22856=DIRECTION('ref_axis',(1.,0.,0.));
#22857=DIRECTION('',(0.,1.,0.));
#22858=DIRECTION('',(0.,1.,0.));
#22859=DIRECTION('center_axis',(0.951056516295154,0.,-0.309016994374947));
#22860=DIRECTION('ref_axis',(-0.309016994374947,0.,-0.951056516295154));
#22861=DIRECTION('',(-0.309016994374947,0.,-0.951056516295154));
#22862=DIRECTION('center_axis',(0.,1.,0.));
#22863=DIRECTION('ref_axis',(1.,0.,0.));
#22864=DIRECTION('center_axis',(0.,1.,0.));
#22865=DIRECTION('ref_axis',(1.,0.,0.));
#22866=DIRECTION('',(0.,1.,0.));
#22867=DIRECTION('center_axis',(0.987688340595138,0.,-0.156434465040231));
#22868=DIRECTION('ref_axis',(-0.156434465040231,0.,-0.987688340595138));
#22869=DIRECTION('',(-0.156434465040231,0.,-0.987688340595138));
#22870=DIRECTION('',(0.,1.,0.));
#22871=DIRECTION('center_axis',(0.,1.,0.));
#22872=DIRECTION('ref_axis',(1.,0.,0.));
#22873=DIRECTION('center_axis',(0.,1.,0.));
#22874=DIRECTION('ref_axis',(1.,0.,0.));
#22875=DIRECTION('',(0.,1.,0.));
#22876=DIRECTION('',(0.,1.,0.));
#22877=DIRECTION('center_axis',(1.,0.,0.));
#22878=DIRECTION('ref_axis',(0.,0.,-1.));
#22879=DIRECTION('',(0.,0.,-1.));
#22880=DIRECTION('center_axis',(0.,1.,0.));
#22881=DIRECTION('ref_axis',(1.,0.,0.));
#22882=DIRECTION('center_axis',(0.,1.,0.));
#22883=DIRECTION('ref_axis',(1.,0.,0.));
#22884=DIRECTION('center_axis',(0.,1.,0.));
#22885=DIRECTION('ref_axis',(1.,0.,0.));
#38754=CARTESIAN_POINT('',(0.,0.,0.));
#38755=CARTESIAN_POINT('Origin',(0.3,0.,0.));
#38756=CARTESIAN_POINT('',(0.3,2.2,-1.28));
#38757=CARTESIAN_POINT('',(0.3,2.2,-0.953939201416946));
#38758=CARTESIAN_POINT('',(0.3,2.2,0.));
#38759=CARTESIAN_POINT('',(0.3,-1.,-1.28));
#38760=CARTESIAN_POINT('',(0.3,0.,-1.28));
#38761=CARTESIAN_POINT('',(0.3,-1.,-0.953939201416946));
#38762=CARTESIAN_POINT('',(0.3,-1.,0.));
#38763=CARTESIAN_POINT('',(0.3,0.,-0.953939201416946));
#38764=CARTESIAN_POINT('Origin',(0.3,0.,-1.28));
#38765=CARTESIAN_POINT('',(-0.3,2.2,-1.28));
#38766=CARTESIAN_POINT('',(0.15,2.2,-1.28));
#38767=CARTESIAN_POINT('',(-0.3,-1.,-1.28));
#38768=CARTESIAN_POINT('',(-0.3,0.,-1.28));
#38769=CARTESIAN_POINT('',(0.15,-1.,-1.28));
#38770=CARTESIAN_POINT('Origin',(-0.3,0.,-1.28));
#38771=CARTESIAN_POINT('',(-0.3,2.2,-0.953939201416946));
#38772=CARTESIAN_POINT('',(-0.3,2.2,-0.64));
#38773=CARTESIAN_POINT('',(-0.3,-1.,-0.953939201416946));
#38774=CARTESIAN_POINT('',(-0.3,0.,-0.953939201416946));
#38775=CARTESIAN_POINT('',(-0.3,-1.,-0.64));
#38776=CARTESIAN_POINT('Origin',(0.,-1.,0.));
#38777=CARTESIAN_POINT('',(3.66661143271685,-1.,0.786422660831985));
#38778=CARTESIAN_POINT('',(3.62400312501245,-1.,0.963899035117249));
#38779=CARTESIAN_POINT('Origin',(0.,-1.,0.));
#38780=CARTESIAN_POINT('',(4.01728681790024,-1.,1.22531898815164));
#38781=CARTESIAN_POINT('Ctrl Pts',(3.62400312501245,-1.,0.963899035117249));
#38782=CARTESIAN_POINT('Ctrl Pts',(3.6240482887845,-1.,0.963880158555582));
#38783=CARTESIAN_POINT('Ctrl Pts',(3.62424461507588,-1.,0.963861297423241));
#38784=CARTESIAN_POINT('Ctrl Pts',(3.62489305727662,-1.,0.963957782642844));
#38785=CARTESIAN_POINT('Ctrl Pts',(3.62652618145335,-1.,0.964373850166458));
#38786=CARTESIAN_POINT('Ctrl Pts',(3.62988252139846,-1.,0.965395153165294));
#38787=CARTESIAN_POINT('Ctrl Pts',(3.63492122081143,-1.,0.967052554541386));
#38788=CARTESIAN_POINT('Ctrl Pts',(3.64113946505766,-1.,0.969195124675866));
#38789=CARTESIAN_POINT('Ctrl Pts',(3.64819756447455,-1.,0.971722122061341));
#38790=CARTESIAN_POINT('Ctrl Pts',(3.65571576735126,-1.,0.974519971354849));
#38791=CARTESIAN_POINT('Ctrl Pts',(3.66333049637475,-1.,0.977478312751618));
#38792=CARTESIAN_POINT('Ctrl Pts',(3.67074983340361,-1.,0.980505922458267));
#38793=CARTESIAN_POINT('Ctrl Pts',(3.67782408841715,-1.,0.98355079147042));
#38794=CARTESIAN_POINT('Ctrl Pts',(3.68455317926068,-1.,0.986602639863838));
#38795=CARTESIAN_POINT('Ctrl Pts',(3.69102682138846,-1.,0.989676715398559));
#38796=CARTESIAN_POINT('Ctrl Pts',(3.69738123415662,-1.,0.992802218332011));
#38797=CARTESIAN_POINT('Ctrl Pts',(3.70375282282138,-1.,0.996009819772518));
#38798=CARTESIAN_POINT('Ctrl Pts',(3.71022439713938,-1.,0.999317260756531));
#38799=CARTESIAN_POINT('Ctrl Pts',(3.71680667125118,-1.,1.00272423396822));
#38800=CARTESIAN_POINT('Ctrl Pts',(3.72346803750595,-1.,1.0062200073571));
#38801=CARTESIAN_POINT('Ctrl Pts',(3.73015276704426,-1.,1.00978798539496));
#38802=CARTESIAN_POINT('Ctrl Pts',(3.73680245055734,-1.,1.01341114319903));
#38803=CARTESIAN_POINT('Ctrl Pts',(3.74337942504959,-1.,1.01707794311079));
#38804=CARTESIAN_POINT('Ctrl Pts',(3.74987777155834,-1.,1.02078510487428));
#38805=CARTESIAN_POINT('Ctrl Pts',(3.75631037456194,-1.,1.0245342944466));
#38806=CARTESIAN_POINT('Ctrl Pts',(3.76270122291232,-1.,1.02833014458181));
#38807=CARTESIAN_POINT('Ctrl Pts',(3.76907609832522,-1.,1.0321778660492));
#38808=CARTESIAN_POINT('Ctrl Pts',(3.77545283140445,-1.,1.03608074678013));
#38809=CARTESIAN_POINT('Ctrl Pts',(3.78183535008192,-1.,1.04003862055804));
#38810=CARTESIAN_POINT('Ctrl Pts',(3.78821910787195,-1.,1.04404924374426));
#38811=CARTESIAN_POINT('Ctrl Pts',(3.79459440308793,-1.,1.04810913267641));
#38812=CARTESIAN_POINT('Ctrl Pts',(3.80095039790678,-1.,1.05221457990015));
#38813=CARTESIAN_POINT('Ctrl Pts',(3.80727913637784,-1.,1.05636266918643));
#38814=CARTESIAN_POINT('Ctrl Pts',(3.81357866117485,-1.,1.06055206187298));
#38815=CARTESIAN_POINT('Ctrl Pts',(3.81985083953012,-1.,1.06478244038931));
#38816=CARTESIAN_POINT('Ctrl Pts',(3.82609989967278,-1.,1.0690541318036));
#38817=CARTESIAN_POINT('Ctrl Pts',(3.83233071195145,-1.,1.0733676663346));
#38818=CARTESIAN_POINT('Ctrl Pts',(3.83854714117486,-1.,1.07772335353856));
#38819=CARTESIAN_POINT('Ctrl Pts',(3.84475048030615,-1.,1.08212087917986));
#38820=CARTESIAN_POINT('Ctrl Pts',(3.8509402522269,-1.,1.08655950846377));
#38821=CARTESIAN_POINT('Ctrl Pts',(3.85711487933911,-1.,1.09103825516288));
#38822=CARTESIAN_POINT('Ctrl Pts',(3.86327241021242,-1.,1.09555606505012));
#38823=CARTESIAN_POINT('Ctrl Pts',(3.86941120134872,-1.,1.10011198761203));
#38824=CARTESIAN_POINT('Ctrl Pts',(3.87553067187566,-1.,1.10470536603303));
#38825=CARTESIAN_POINT('Ctrl Pts',(3.88163105531791,-1.,1.10933577224029));
#38826=CARTESIAN_POINT('Ctrl Pts',(3.88771308285229,-1.,1.11400292434447));
#38827=CARTESIAN_POINT('Ctrl Pts',(3.89377768340362,-1.,1.11870660794609));
#38828=CARTESIAN_POINT('Ctrl Pts',(3.89982569749978,-1.,1.12344660099029));
#38829=CARTESIAN_POINT('Ctrl Pts',(3.90585753318622,-1.,1.12822258281518));
#38830=CARTESIAN_POINT('Ctrl Pts',(3.91187321145495,-1.,1.13303414693849));
#38831=CARTESIAN_POINT('Ctrl Pts',(3.91787251936688,-1.,1.13788084225511));
#38832=CARTESIAN_POINT('Ctrl Pts',(3.92385513133937,-1.,1.14276220561575));
#38833=CARTESIAN_POINT('Ctrl Pts',(3.92982073294334,-1.,1.14767779451147));
#38834=CARTESIAN_POINT('Ctrl Pts',(3.9357691705651,-1.,1.15262722716391));
#38835=CARTESIAN_POINT('Ctrl Pts',(3.94170046685542,-1.,1.15761018341061));
#38836=CARTESIAN_POINT('Ctrl Pts',(3.9476147478092,-1.,1.16262637999261));
#38837=CARTESIAN_POINT('Ctrl Pts',(3.95351219510062,-1.,1.16767555244495));
#38838=CARTESIAN_POINT('Ctrl Pts',(3.95939299213164,-1.,1.17275743590327));
#38839=CARTESIAN_POINT('Ctrl Pts',(3.96525726357682,-1.,1.17787174135446));
#38840=CARTESIAN_POINT('Ctrl Pts',(3.9711050516465,-1.,1.18301815039596));
#38841=CARTESIAN_POINT('Ctrl Pts',(3.97693634766926,-1.,1.18819633715285));
#38842=CARTESIAN_POINT('Ctrl Pts',(3.98275111052015,-1.,1.19340598349307));
#38843=CARTESIAN_POINT('Ctrl Pts',(3.98854928957287,-1.,1.19864679609596));
#38844=CARTESIAN_POINT('Ctrl Pts',(3.99433084800649,-1.,1.2039185237544));
#38845=CARTESIAN_POINT('Ctrl Pts',(4.00009577952534,-1.,1.20922097030107));
#38846=CARTESIAN_POINT('Ctrl Pts',(4.00584409524937,-1.,1.21455398918813));
#38847=CARTESIAN_POINT('Ctrl Pts',(4.01042947142681,-1.,1.21884478244983));
#38848=CARTESIAN_POINT('Ctrl Pts',(4.01386104434674,-1.,1.22207656456199));
#38849=CARTESIAN_POINT('Ctrl Pts',(4.0161454457032,-1.,1.22423716681447));
#38850=CARTESIAN_POINT('Ctrl Pts',(4.01728681790024,-1.,1.22531898815164));
#38851=CARTESIAN_POINT('',(3.97027773754922,-1.,1.36999806084573));
#38852=CARTESIAN_POINT('',(4.01728681790024,-1.,1.22531898815164));
#38853=CARTESIAN_POINT('',(3.4984457533445,-1.,1.35032489087101));
#38854=CARTESIAN_POINT('Ctrl Pts',(3.97027773754922,-1.,1.36999806084573));
#38855=CARTESIAN_POINT('Ctrl Pts',(3.9687184694131,-1.,1.37020239094614));
#38856=CARTESIAN_POINT('Ctrl Pts',(3.96560037974645,-1.,1.37060761745635));
#38857=CARTESIAN_POINT('Ctrl Pts',(3.96092458506535,-1.,1.3712051561502));
#38858=CARTESIAN_POINT('Ctrl Pts',(3.95469287280914,-1.,1.37198126432386));
#38859=CARTESIAN_POINT('Ctrl Pts',(3.94690771785133,-1.,1.37291699202807));
#38860=CARTESIAN_POINT('Ctrl Pts',(3.93912709040818,-1.,1.37381821967165));
#38861=CARTESIAN_POINT('Ctrl Pts',(3.93135106761844,-1.,1.37468482215751));
#38862=CARTESIAN_POINT('Ctrl Pts',(3.92357976987672,-1.,1.37551664448242));
#38863=CARTESIAN_POINT('Ctrl Pts',(3.91581337462644,-1.,1.37631350505797));
#38864=CARTESIAN_POINT('Ctrl Pts',(3.90805209523486,-1.,1.3770751963402));
#38865=CARTESIAN_POINT('Ctrl Pts',(3.90029615196727,-1.,1.37780148512792));
#38866=CARTESIAN_POINT('Ctrl Pts',(3.89254574338496,-1.,1.3784921128802));
#38867=CARTESIAN_POINT('Ctrl Pts',(3.88480102249277,-1.,1.37914679719383));
#38868=CARTESIAN_POINT('Ctrl Pts',(3.87706205830532,-1.,1.37976523097073));
#38869=CARTESIAN_POINT('Ctrl Pts',(3.86932885813068,-1.,1.38034709213014));
#38870=CARTESIAN_POINT('Ctrl Pts',(3.86160143043959,-1.,1.3808920599299));
#38871=CARTESIAN_POINT('Ctrl Pts',(3.85387983979481,-1.,1.3813998311505));
#38872=CARTESIAN_POINT('Ctrl Pts',(3.84616425605764,-1.,1.38187013346109));
#38873=CARTESIAN_POINT('Ctrl Pts',(3.83845502790746,-1.,1.38230274828822));
#38874=CARTESIAN_POINT('Ctrl Pts',(3.8307526698229,-1.,1.38269750245138));
#38875=CARTESIAN_POINT('Ctrl Pts',(3.82305771743829,-1.,1.38305421262763));
#38876=CARTESIAN_POINT('Ctrl Pts',(3.81537060817811,-1.,1.38337263902782));
#38877=CARTESIAN_POINT('Ctrl Pts',(3.80769156398411,-1.,1.3836524404622));
#38878=CARTESIAN_POINT('Ctrl Pts',(3.80002044322111,-1.,1.38389311766682));
#38879=CARTESIAN_POINT('Ctrl Pts',(3.79235669640841,-1.,1.38409399694566));
#38880=CARTESIAN_POINT('Ctrl Pts',(3.78469969805082,-1.,1.38425435883756));
#38881=CARTESIAN_POINT('Ctrl Pts',(3.77704902230418,-1.,1.38437354551428));
#38882=CARTESIAN_POINT('Ctrl Pts',(3.76940473185779,-1.,1.38445107339518));
#38883=CARTESIAN_POINT('Ctrl Pts',(3.76176768271367,-1.,1.3844867525335));
#38884=CARTESIAN_POINT('Ctrl Pts',(3.7541397631875,-1.,1.38448077997163));
#38885=CARTESIAN_POINT('Ctrl Pts',(3.74652317167876,-1.,1.38443344984394));
#38886=CARTESIAN_POINT('Ctrl Pts',(3.73891976418104,-1.,1.38434489156458));
#38887=CARTESIAN_POINT('Ctrl Pts',(3.73133035859282,-1.,1.38421479111531));
#38888=CARTESIAN_POINT('Ctrl Pts',(3.72375409358803,-1.,1.3840421342895));
#38889=CARTESIAN_POINT('Ctrl Pts',(3.7161876605181,-1.,1.38382489984586));
#38890=CARTESIAN_POINT('Ctrl Pts',(3.70862680753347,-1.,1.38356065402124));
#38891=CARTESIAN_POINT('Ctrl Pts',(3.701067921679,-1.,1.38324717612865));
#38892=CARTESIAN_POINT('Ctrl Pts',(3.69350967899526,-1.,1.38288311171651));
#38893=CARTESIAN_POINT('Ctrl Pts',(3.68595444983837,-1.,1.38246852827182));
#38894=CARTESIAN_POINT('Ctrl Pts',(3.67841038482414,-1.,1.3820057429062));
#38895=CARTESIAN_POINT('Ctrl Pts',(3.67088843112262,-1.,1.38149812653868));
#38896=CARTESIAN_POINT('Ctrl Pts',(3.66339848520857,-1.,1.38094856333552));
#38897=CARTESIAN_POINT('Ctrl Pts',(3.6559455440439,-1.,1.38035791051213));
#38898=CARTESIAN_POINT('Ctrl Pts',(3.64852652756456,-1.,1.37972372481603));
#38899=CARTESIAN_POINT('Ctrl Pts',(3.64112507791141,-1.,1.37903818567359));
#38900=CARTESIAN_POINT('Ctrl Pts',(3.63371727442486,-1.,1.37829035457339));
#38901=CARTESIAN_POINT('Ctrl Pts',(3.62628098665145,-1.,1.37746987919881));
#38902=CARTESIAN_POINT('Ctrl Pts',(3.6188048116042,-1.,1.37657053403107));
#38903=CARTESIAN_POINT('Ctrl Pts',(3.61129546591064,-1.,1.37559314436634));
#38904=CARTESIAN_POINT('Ctrl Pts',(3.60379020123988,-1.,1.37455051379623));
#38905=CARTESIAN_POINT('Ctrl Pts',(3.59634627869048,-1.,1.37346320103157));
#38906=CARTESIAN_POINT('Ctrl Pts',(3.58901853846365,-1.,1.37235053660976));
#38907=CARTESIAN_POINT('Ctrl Pts',(3.58183885982715,-1.,1.37122241663062));
#38908=CARTESIAN_POINT('Ctrl Pts',(3.57479875549486,-1.,1.37007229485659));
#38909=CARTESIAN_POINT('Ctrl Pts',(3.5678208030466,-1.,1.36886584973389));
#38910=CARTESIAN_POINT('Ctrl Pts',(3.56077662028649,-1.,1.36754771771233));
#38911=CARTESIAN_POINT('Ctrl Pts',(3.55353883995949,-1.,1.3660614545677));
#38912=CARTESIAN_POINT('Ctrl Pts',(3.54602591832973,-1.,1.36436666257598));
#38913=CARTESIAN_POINT('Ctrl Pts',(3.53824396424961,-1.,1.36245507339307));
#38914=CARTESIAN_POINT('Ctrl Pts',(3.530344649616,-1.,1.36037259643734));
#38915=CARTESIAN_POINT('Ctrl Pts',(3.52261776116748,-1.,1.35821701528836));
#38916=CARTESIAN_POINT('Ctrl Pts',(3.51542230699556,-1.,1.35611275237152));
#38917=CARTESIAN_POINT('Ctrl Pts',(3.50913227059999,-1.,1.35419113575956));
#38918=CARTESIAN_POINT('Ctrl Pts',(3.50408168106261,-1.,1.35257032843486));
#38919=CARTESIAN_POINT('Ctrl Pts',(3.5007660381649,-1.,1.35142377279517));
#38920=CARTESIAN_POINT('Ctrl Pts',(3.49920025459723,-1.,1.35080045218587));
#38921=CARTESIAN_POINT('Ctrl Pts',(3.49861894124827,-1.,1.35049736560527));
#38922=CARTESIAN_POINT('Ctrl Pts',(3.49847119623846,-1.,1.35036670892966));
#38923=CARTESIAN_POINT('Ctrl Pts',(3.4984457533445,-1.,1.35032489087101));
#38924=CARTESIAN_POINT('',(3.42859860294378,-1.,1.51895082866166));
#38925=CARTESIAN_POINT('Origin',(0.,-1.,0.));
#38926=CARTESIAN_POINT('',(3.77614523045147,-1.,1.83867539237861));
#38927=CARTESIAN_POINT('Ctrl Pts',(3.42859860294378,-1.,1.51895082866166));
#38928=CARTESIAN_POINT('Ctrl Pts',(3.42864616361967,-1.,1.51893924967231));
#38929=CARTESIAN_POINT('Ctrl Pts',(3.42884302333978,-1.,1.51895133295017));
#38930=CARTESIAN_POINT('Ctrl Pts',(3.42946838852728,-1.,1.51914806898539));
#38931=CARTESIAN_POINT('Ctrl Pts',(3.4310163189349,-1.,1.5198144909343));
#38932=CARTESIAN_POINT('Ctrl Pts',(3.43417156977749,-1.,1.52134826724227));
#38933=CARTESIAN_POINT('Ctrl Pts',(3.43888895974182,-1.,1.52377348950429));
#38934=CARTESIAN_POINT('Ctrl Pts',(3.44469547527,-1.,1.52686242875717));
#38935=CARTESIAN_POINT('Ctrl Pts',(3.45127136828667,-1.,1.530462444618));
#38936=CARTESIAN_POINT('Ctrl Pts',(3.45825932955273,-1.,1.53440195378902));
#38937=CARTESIAN_POINT('Ctrl Pts',(3.46531752207222,-1.,1.53851507915533));
#38938=CARTESIAN_POINT('Ctrl Pts',(3.47217189224576,-1.,1.54266605398152));
#38939=CARTESIAN_POINT('Ctrl Pts',(3.47868272898599,-1.,1.54678009290207));
#38940=CARTESIAN_POINT('Ctrl Pts',(3.48485155928414,-1.,1.55084702970382));
#38941=CARTESIAN_POINT('Ctrl Pts',(3.49076460877317,-1.,1.5548959590107));
#38942=CARTESIAN_POINT('Ctrl Pts',(3.49655185179623,-1.,1.55897703097859));
#38943=CARTESIAN_POINT('Ctrl Pts',(3.50234321621607,-1.,1.56314187758689));
#38944=CARTESIAN_POINT('Ctrl Pts',(3.50821771695427,-1.,1.56742097575041));
#38945=CARTESIAN_POINT('Ctrl Pts',(3.51418598431733,-1.,1.57181569799774));
#38946=CARTESIAN_POINT('Ctrl Pts',(3.52021847865961,-1.,1.5763104998818));
#38947=CARTESIAN_POINT('Ctrl Pts',(3.52626275334899,-1.,1.58088027227856));
#38948=CARTESIAN_POINT('Ctrl Pts',(3.53226378147068,-1.,1.58549906268083));
#38949=CARTESIAN_POINT('Ctrl Pts',(3.53818616861045,-1.,1.59014958368725));
#38950=CARTESIAN_POINT('Ctrl Pts',(3.544024581823,-1.,1.5948276694975));
#38951=CARTESIAN_POINT('Ctrl Pts',(3.54979148634426,-1.,1.59953698113444));
#38952=CARTESIAN_POINT('Ctrl Pts',(3.55550985096117,-1.,1.60428584699848));
#38953=CARTESIAN_POINT('Ctrl Pts',(3.56120432482986,-1.,1.60908344685459));
#38954=CARTESIAN_POINT('Ctrl Pts',(3.56689200468404,-1.,1.61393581747522));
#38955=CARTESIAN_POINT('Ctrl Pts',(3.57257679609826,-1.,1.61884340915412));
#38956=CARTESIAN_POINT('Ctrl Pts',(3.57825455954405,-1.,1.62380329464851));
#38957=CARTESIAN_POINT('Ctrl Pts',(3.5839162577435,-1.,1.62881051550748));
#38958=CARTESIAN_POINT('Ctrl Pts',(3.58955176627876,-1.,1.63385971451259));
#38959=CARTESIAN_POINT('Ctrl Pts',(3.59515368334887,-1.,1.63894676675349));
#38960=CARTESIAN_POINT('Ctrl Pts',(3.6007202851384,-1.,1.6440700438558));
#38961=CARTESIAN_POINT('Ctrl Pts',(3.60625346556992,-1.,1.64922952425833));
#38962=CARTESIAN_POINT('Ctrl Pts',(3.61175734965129,-1.,1.65442619244327));
#38963=CARTESIAN_POINT('Ctrl Pts',(3.61723666482457,-1.,1.65966133399186));
#38964=CARTESIAN_POINT('Ctrl Pts',(3.62269517989104,-1.,1.66493585923853));
#38965=CARTESIAN_POINT('Ctrl Pts',(3.62813422105257,-1.,1.67024966008037));
#38966=CARTESIAN_POINT('Ctrl Pts',(3.63355343201211,-1.,1.67560193613145));
#38967=CARTESIAN_POINT('Ctrl Pts',(3.63895140887443,-1.,1.68099146651577));
#38968=CARTESIAN_POINT('Ctrl Pts',(3.64432638915199,-1.,1.68641690471455));
#38969=CARTESIAN_POINT('Ctrl Pts',(3.64967689827393,-1.,1.691877054817));
#38970=CARTESIAN_POINT('Ctrl Pts',(3.65500246526798,-1.,1.69737117722559));
#38971=CARTESIAN_POINT('Ctrl Pts',(3.6603033877491,-1.,1.70289888566904));
#38972=CARTESIAN_POINT('Ctrl Pts',(3.6655804319893,-1.,1.70846001610983));
#38973=CARTESIAN_POINT('Ctrl Pts',(3.67083454901629,-1.,1.71405450210392));
#38974=CARTESIAN_POINT('Ctrl Pts',(3.67606660374665,-1.,1.71968225581787));
#38975=CARTESIAN_POINT('Ctrl Pts',(3.68127704936472,-1.,1.72534302437003));
#38976=CARTESIAN_POINT('Ctrl Pts',(3.68646597019188,-1.,1.73103640956647));
#38977=CARTESIAN_POINT('Ctrl Pts',(3.69163322647906,-1.,1.73676193254493));
#38978=CARTESIAN_POINT('Ctrl Pts',(3.6967785691046,-1.,1.74251908492589));
#38979=CARTESIAN_POINT('Ctrl Pts',(3.70190175673422,-1.,1.74830738046092));
#38980=CARTESIAN_POINT('Ctrl Pts',(3.70700269736876,-1.,1.75412641804148));
#38981=CARTESIAN_POINT('Ctrl Pts',(3.71208146346454,-1.,1.75997588499021));
#38982=CARTESIAN_POINT('Ctrl Pts',(3.71713822377675,-1.,1.76585552124549));
#38983=CARTESIAN_POINT('Ctrl Pts',(3.72217319911429,-1.,1.77176509401846));
#38984=CARTESIAN_POINT('Ctrl Pts',(3.72718661205504,-1.,1.77770437039606));
#38985=CARTESIAN_POINT('Ctrl Pts',(3.73217863095022,-1.,1.78367308442682));
#38986=CARTESIAN_POINT('Ctrl Pts',(3.73714934729962,-1.,1.78967092823139));
#38987=CARTESIAN_POINT('Ctrl Pts',(3.74209880351667,-1.,1.79569757859041));
#38988=CARTESIAN_POINT('Ctrl Pts',(3.74702700874954,-1.,1.80175271485519));
#38989=CARTESIAN_POINT('Ctrl Pts',(3.75193395888069,-1.,1.80783603939662));
#38990=CARTESIAN_POINT('Ctrl Pts',(3.75681965683995,-1.,1.81394729834032));
#38991=CARTESIAN_POINT('Ctrl Pts',(3.76168412709652,-1.,1.82008629694924));
#38992=CARTESIAN_POINT('Ctrl Pts',(3.76652740355856,-1.,1.82625289221933));
#38993=CARTESIAN_POINT('Ctrl Pts',(3.77038509819777,-1.,1.83120816956515));
#38994=CARTESIAN_POINT('Ctrl Pts',(3.77326886065484,-1.,1.83493697935064));
#38995=CARTESIAN_POINT('Ctrl Pts',(3.77518714458232,-1.,1.83742834010821));
#38996=CARTESIAN_POINT('Ctrl Pts',(3.77614523045147,-1.,1.83867539237861));
#38997=CARTESIAN_POINT('',(3.70708211654725,-1.,1.97421938526992));
#38998=CARTESIAN_POINT('',(3.77614523045147,-1.,1.83867539237861));
#38999=CARTESIAN_POINT('',(3.24413672884902,-1.,1.88097764062542));
#39000=CARTESIAN_POINT('Ctrl Pts',(3.70708211654725,-1.,1.97421938526992));
#39001=CARTESIAN_POINT('Ctrl Pts',(3.7055100813194,-1.,1.974177276451));
#39002=CARTESIAN_POINT('Ctrl Pts',(3.70236698911837,-1.,1.97408973726149));
#39003=CARTESIAN_POINT('Ctrl Pts',(3.69765528558292,-1.,1.97394846382289));
#39004=CARTESIAN_POINT('Ctrl Pts',(3.69137888597855,-1.,1.97374016224397));
#39005=CARTESIAN_POINT('Ctrl Pts',(3.68354319913416,-1.,1.97344650303631));
#39006=CARTESIAN_POINT('Ctrl Pts',(3.67571738106175,-1.,1.97311947678035));
#39007=CARTESIAN_POINT('Ctrl Pts',(3.66790152751984,-1.,1.9727589719863));
#39008=CARTESIAN_POINT('Ctrl Pts',(3.66009578166865,-1.,1.97236485439317));
#39009=CARTESIAN_POINT('Ctrl Pts',(3.65230034717364,-1.,1.97193697240645));
#39010=CARTESIAN_POINT('Ctrl Pts',(3.64451546724221,-1.,1.97147515441539));
#39011=CARTESIAN_POINT('Ctrl Pts',(3.63674139590853,-1.,1.97097920454698));
#39012=CARTESIAN_POINT('Ctrl Pts',(3.62897836973397,-1.,1.97044889850518));
#39013=CARTESIAN_POINT('Ctrl Pts',(3.62122658401722,-1.,1.96988398129888));
#39014=CARTESIAN_POINT('Ctrl Pts',(3.61348615496393,-1.,1.96928416040712));
#39015=CARTESIAN_POINT('Ctrl Pts',(3.60575714017676,-1.,1.96864911885775));
#39016=CARTESIAN_POINT('Ctrl Pts',(3.59803959819725,-1.,1.96797854118257));
#39017=CARTESIAN_POINT('Ctrl Pts',(3.5903336402273,-1.,1.96727213799507));
#39018=CARTESIAN_POINT('Ctrl Pts',(3.58263947663884,-1.,1.9665296668894));
#39019=CARTESIAN_POINT('Ctrl Pts',(3.57495748601088,-1.,1.96575096652857));
#39020=CARTESIAN_POINT('Ctrl Pts',(3.56728820357933,-1.,1.96493594634643));
#39021=CARTESIAN_POINT('Ctrl Pts',(3.55963218706201,-1.,1.96408450906868));
#39022=CARTESIAN_POINT('Ctrl Pts',(3.55198990600929,-1.,1.96319648628667));
#39023=CARTESIAN_POINT('Ctrl Pts',(3.54436163300425,-1.,1.96227157573058));
#39024=CARTESIAN_POINT('Ctrl Pts',(3.53674730625759,-1.,1.96130926212661));
#39025=CARTESIAN_POINT('Ctrl Pts',(3.52914648844289,-1.,1.96030879411534));
#39026=CARTESIAN_POINT('Ctrl Pts',(3.52155867431438,-1.,1.95926936324436));
#39027=CARTESIAN_POINT('Ctrl Pts',(3.51398354617772,-1.,1.95819025316768));
#39028=CARTESIAN_POINT('Ctrl Pts',(3.50642124159913,-1.,1.95707099606514));
#39029=CARTESIAN_POINT('Ctrl Pts',(3.49887263575602,-1.,1.9559115382367));
#39030=CARTESIAN_POINT('Ctrl Pts',(3.49133956289154,-1.,1.95471236969653));
#39031=CARTESIAN_POINT('Ctrl Pts',(3.48382414832648,-1.,1.95347412486316));
#39032=CARTESIAN_POINT('Ctrl Pts',(3.47632820495926,-1.,1.95219722189878));
#39033=CARTESIAN_POINT('Ctrl Pts',(3.4688525897419,-1.,1.95088147859876));
#39034=CARTESIAN_POINT('Ctrl Pts',(3.46139661060959,-1.,1.94952575850196));
#39035=CARTESIAN_POINT('Ctrl Pts',(3.45395731584051,-1.,1.94812754766524));
#39036=CARTESIAN_POINT('Ctrl Pts',(3.44653088665685,-1.,1.94668377715332));
#39037=CARTESIAN_POINT('Ctrl Pts',(3.43911410197693,-1.,1.94519168842883));
#39038=CARTESIAN_POINT('Ctrl Pts',(3.43170586602436,-1.,1.94364973660285));
#39039=CARTESIAN_POINT('Ctrl Pts',(3.42430850941497,-1.,1.94205835913692));
#39040=CARTESIAN_POINT('Ctrl Pts',(3.41692971994082,-1.,1.94042111965237));
#39041=CARTESIAN_POINT('Ctrl Pts',(3.40957978266622,-1.,1.93874306008132));
#39042=CARTESIAN_POINT('Ctrl Pts',(3.40226802104093,-1.,1.93702857723089));
#39043=CARTESIAN_POINT('Ctrl Pts',(3.39499923640789,-1.,1.93527929945982));
#39044=CARTESIAN_POINT('Ctrl Pts',(3.38777076883267,-1.,1.93349233176794));
#39045=CARTESIAN_POINT('Ctrl Pts',(3.38056768525577,-1.,1.93165739093292));
#39046=CARTESIAN_POINT('Ctrl Pts',(3.37336807068078,-1.,1.92975993109897));
#39047=CARTESIAN_POINT('Ctrl Pts',(3.36615168657597,-1.,1.92778626543803));
#39048=CARTESIAN_POINT('Ctrl Pts',(3.35890824422976,-1.,1.92572846125763));
#39049=CARTESIAN_POINT('Ctrl Pts',(3.35164424847206,-1.,1.92358838440518));
#39050=CARTESIAN_POINT('Ctrl Pts',(3.34439448941915,-1.,1.92138450828378));
#39051=CARTESIAN_POINT('Ctrl Pts',(3.33721230709948,-1.,1.91914609610173));
#39052=CARTESIAN_POINT('Ctrl Pts',(3.33014884257812,-1.,1.91690081930297));
#39053=CARTESIAN_POINT('Ctrl Pts',(3.32323403454507,-1.,1.91466343916612));
#39054=CARTESIAN_POINT('Ctrl Pts',(3.31646052426395,-1.,1.91242616234459));
#39055=CARTESIAN_POINT('Ctrl Pts',(3.30975721158694,-1.,1.91014297830502));
#39056=CARTESIAN_POINT('Ctrl Pts',(3.30300595568341,-1.,1.90773912171424));
#39057=CARTESIAN_POINT('Ctrl Pts',(3.29608978722258,-1.,1.9051389186417));
#39058=CARTESIAN_POINT('Ctrl Pts',(3.28893448600364,-1.,1.9022897124757));
#39059=CARTESIAN_POINT('Ctrl Pts',(3.28154737912287,-1.,1.89918429230425));
#39060=CARTESIAN_POINT('Ctrl Pts',(3.27407108932908,-1.,1.89589172903662));
#39061=CARTESIAN_POINT('Ctrl Pts',(3.2667765388833,-1.,1.89255393500769));
#39062=CARTESIAN_POINT('Ctrl Pts',(3.2599988519361,-1.,1.88934996203508));
#39063=CARTESIAN_POINT('Ctrl Pts',(3.25408686339298,-1.,1.88646802523372));
#39064=CARTESIAN_POINT('Ctrl Pts',(3.24935200512055,-1.,1.88407708646435));
#39065=CARTESIAN_POINT('Ctrl Pts',(3.24625654410705,-1.,1.88242596600422));
#39066=CARTESIAN_POINT('Ctrl Pts',(3.24480754675942,-1.,1.88156537699118));
#39067=CARTESIAN_POINT('Ctrl Pts',(3.24428080352952,-1.,1.88117508446657));
#39068=CARTESIAN_POINT('Ctrl Pts',(3.2441553167131,-1.,1.88102292397987));
#39069=CARTESIAN_POINT('Ctrl Pts',(3.24413672884902,-1.,1.88097764062542));
#39070=CARTESIAN_POINT('',(3.14877060440425,-1.,2.03660101169564));
#39071=CARTESIAN_POINT('Origin',(0.,-1.,0.));
#39072=CARTESIAN_POINT('',(3.44202241512147,-1.,2.40675750623143));
#39073=CARTESIAN_POINT('Ctrl Pts',(3.14877060440425,-1.,2.03660101169564));
#39074=CARTESIAN_POINT('Ctrl Pts',(3.1488193908823,-1.,2.03659701539175));
#39075=CARTESIAN_POINT('Ctrl Pts',(3.14901193669147,-1.,2.03663974554941));
#39076=CARTESIAN_POINT('Ctrl Pts',(3.14959882629936,-1.,2.03693188810614));
#39077=CARTESIAN_POINT('Ctrl Pts',(3.15102344775396,-1.,2.03783225496023));
#39078=CARTESIAN_POINT('Ctrl Pts',(3.1538999167466,-1.,2.03984073791432));
#39079=CARTESIAN_POINT('Ctrl Pts',(3.15817983946525,-1.,2.04297406404132));
#39080=CARTESIAN_POINT('Ctrl Pts',(3.16343165059235,-1.,2.0469333124766));
#39081=CARTESIAN_POINT('Ctrl Pts',(3.16936341689859,-1.,2.05151770247452));
#39082=CARTESIAN_POINT('Ctrl Pts',(3.17564906975592,-1.,2.05650186773279));
#39083=CARTESIAN_POINT('Ctrl Pts',(3.18197692964677,-1.,2.06166849827143));
#39084=CARTESIAN_POINT('Ctrl Pts',(3.18809755562297,-1.,2.06684062744065));
#39085=CARTESIAN_POINT('Ctrl Pts',(3.19388465568113,-1.,2.07192253497765));
#39086=CARTESIAN_POINT('Ctrl Pts',(3.19934132835879,-1.,2.0769044187063));
#39087=CARTESIAN_POINT('Ctrl Pts',(3.20454818630635,-1.,2.08182850370816));
#39088=CARTESIAN_POINT('Ctrl Pts',(3.20962575845433,-1.,2.08676465517435));
#39089=CARTESIAN_POINT('Ctrl Pts',(3.2146942960168,-1.,2.0917841946046));
#39090=CARTESIAN_POINT('Ctrl Pts',(3.21982707347067,-1.,2.09692958434933));
#39091=CARTESIAN_POINT('Ctrl Pts',(3.22503437553496,-1.,2.10220384298534));
#39092=CARTESIAN_POINT('Ctrl Pts',(3.23028945793334,-1.,2.1075869964248));
#39093=CARTESIAN_POINT('Ctrl Pts',(3.23554444767115,-1.,2.11304604021784));
#39094=CARTESIAN_POINT('Ctrl Pts',(3.24074905517282,-1.,2.11854673326972));
#39095=CARTESIAN_POINT('Ctrl Pts',(3.24587102613347,-1.,2.12406646410943));
#39096=CARTESIAN_POINT('Ctrl Pts',(3.25090574493994,-1.,2.1296002839681));
#39097=CARTESIAN_POINT('Ctrl Pts',(3.25586495065027,-1.,2.13515375878786));
#39098=CARTESIAN_POINT('Ctrl Pts',(3.26077002641868,-1.,2.14073870754258));
#39099=CARTESIAN_POINT('Ctrl Pts',(3.26564388189764,-1.,2.14636805295663));
#39100=CARTESIAN_POINT('Ctrl Pts',(3.27050245897244,-1.,2.15205043199818));
#39101=CARTESIAN_POINT('Ctrl Pts',(3.27534954469206,-1.,2.15778690038359));
#39102=CARTESIAN_POINT('Ctrl Pts',(3.28018150841414,-1.,2.16357391934434));
#39103=CARTESIAN_POINT('Ctrl Pts',(3.2849901997973,-1.,2.16940517773459));
#39104=CARTESIAN_POINT('Ctrl Pts',(3.28976645712566,-1.,2.17527380048422));
#39105=CARTESIAN_POINT('Ctrl Pts',(3.29450361500484,-1.,2.18117455557062));
#39106=CARTESIAN_POINT('Ctrl Pts',(3.29920022557635,-1.,2.18710556500325));
#39107=CARTESIAN_POINT('Ctrl Pts',(3.30385816281831,-1.,2.19306710376112));
#39108=CARTESIAN_POINT('Ctrl Pts',(3.30848134694596,-1.,2.19906078949925));
#39109=CARTESIAN_POINT('Ctrl Pts',(3.3130742460895,-1.,2.20508863150608));
#39110=CARTESIAN_POINT('Ctrl Pts',(3.31764044024231,-1.,2.21115211847872));
#39111=CARTESIAN_POINT('Ctrl Pts',(3.32218125618955,-1.,2.21725135110889));
#39112=CARTESIAN_POINT('Ctrl Pts',(3.32669646722871,-1.,2.22338548312759));
#39113=CARTESIAN_POINT('Ctrl Pts',(3.33118487773593,-1.,2.22955308907221));
#39114=CARTESIAN_POINT('Ctrl Pts',(3.33564495756478,-1.,2.2357525632881));
#39115=CARTESIAN_POINT('Ctrl Pts',(3.34007543738044,-1.,2.24198249391437));
#39116=CARTESIAN_POINT('Ctrl Pts',(3.34447596770768,-1.,2.24824207678288));
#39117=CARTESIAN_POINT('Ctrl Pts',(3.34884690292342,-1.,2.25453097693524));
#39118=CARTESIAN_POINT('Ctrl Pts',(3.35318902552676,-1.,2.26084915222484));
#39119=CARTESIAN_POINT('Ctrl Pts',(3.35750328523077,-1.,2.26719668579921));
#39120=CARTESIAN_POINT('Ctrl Pts',(3.36179055004369,-1.,2.27357362620902));
#39121=CARTESIAN_POINT('Ctrl Pts',(3.36605130712978,-1.,2.27997979457968));
#39122=CARTESIAN_POINT('Ctrl Pts',(3.37028570206357,-1.,2.28641481081045));
#39123=CARTESIAN_POINT('Ctrl Pts',(3.37449367172707,-1.,2.2928781800731));
#39124=CARTESIAN_POINT('Ctrl Pts',(3.37867504959382,-1.,2.29936936127588));
#39125=CARTESIAN_POINT('Ctrl Pts',(3.38282967336676,-1.,2.30588783640389));
#39126=CARTESIAN_POINT('Ctrl Pts',(3.38695751492659,-1.,2.31243319489505));
#39127=CARTESIAN_POINT('Ctrl Pts',(3.39105869475112,-1.,2.31900513925627));
#39128=CARTESIAN_POINT('Ctrl Pts',(3.39513342020045,-1.,2.32560343902683));
#39129=CARTESIAN_POINT('Ctrl Pts',(3.39918194578115,-1.,2.33222789882601));
#39130=CARTESIAN_POINT('Ctrl Pts',(3.40320452776646,-1.,2.33887832342715));
#39131=CARTESIAN_POINT('Ctrl Pts',(3.40720137403888,-1.,2.34555447648901));
#39132=CARTESIAN_POINT('Ctrl Pts',(3.41117262313464,-1.,2.35225606823649));
#39133=CARTESIAN_POINT('Ctrl Pts',(3.4151183675076,-1.,2.35898278606449));
#39134=CARTESIAN_POINT('Ctrl Pts',(3.41903866635384,-1.,2.36573431470314));
#39135=CARTESIAN_POINT('Ctrl Pts',(3.42293356216595,-1.,2.37251035954351));
#39136=CARTESIAN_POINT('Ctrl Pts',(3.42680309755241,-1.,2.37931067029517));
#39137=CARTESIAN_POINT('Ctrl Pts',(3.43064732714472,-1.,2.38613505844641));
#39138=CARTESIAN_POINT('Ctrl Pts',(3.43446630680436,-1.,2.39298338805823));
#39139=CARTESIAN_POINT('Ctrl Pts',(3.43750133066036,-1.,2.39848113411429));
#39140=CARTESIAN_POINT('Ctrl Pts',(3.43976627485223,-1.,2.40261515590099));
#39141=CARTESIAN_POINT('Ctrl Pts',(3.44127120683402,-1.,2.40537592959345));
#39142=CARTESIAN_POINT('Ctrl Pts',(3.44202241512147,-1.,2.40675750623143));
#39143=CARTESIAN_POINT('',(3.35260583073571,-1.,2.52982887637028));
#39144=CARTESIAN_POINT('',(3.44202241512147,-1.,2.40675750623143));
#39145=CARTESIAN_POINT('',(2.90994629141676,-1.,2.36531447826074));
#39146=CARTESIAN_POINT('Ctrl Pts',(3.35260583073571,-1.,2.52982887637028));
#39147=CARTESIAN_POINT('Ctrl Pts',(3.35105973714071,-1.,2.5295413654909));
#39148=CARTESIAN_POINT('Ctrl Pts',(3.34796903576663,-1.,2.52896321610703));
#39149=CARTESIAN_POINT('Ctrl Pts',(3.34333744115511,-1.,2.52808660915689));
#39150=CARTESIAN_POINT('Ctrl Pts',(3.33717089999103,-1.,2.52689902690158));
#39151=CARTESIAN_POINT('Ctrl Pts',(3.32947762187533,-1.,2.52538321164634));
#39152=CARTESIAN_POINT('Ctrl Pts',(3.32179931078699,-1.,2.5238359839626));
#39153=CARTESIAN_POINT('Ctrl Pts',(3.31413607874645,-1.,2.52225724871313));
#39154=CARTESIAN_POINT('Ctrl Pts',(3.30648808815442,-1.,2.52064689568511));
#39155=CARTESIAN_POINT('Ctrl Pts',(3.29885556388352,-1.,2.51900480701069));
#39156=CARTESIAN_POINT('Ctrl Pts',(3.2912387729927,-1.,2.51733085123797));
#39157=CARTESIAN_POINT('Ctrl Pts',(3.28363799702982,-1.,2.51562487464514));
#39158=CARTESIAN_POINT('Ctrl Pts',(3.27605350473142,-1.,2.513886692704));
#39159=CARTESIAN_POINT('Ctrl Pts',(3.26848552888115,-1.,2.51211608411423));
#39160=CARTESIAN_POINT('Ctrl Pts',(3.26093423001434,-1.,2.51031277813486));
#39161=CARTESIAN_POINT('Ctrl Pts',(3.25339971460982,-1.,2.50847647070723));
#39162=CARTESIAN_POINT('Ctrl Pts',(3.24588208983849,-1.,2.506606859405));
#39163=CARTESIAN_POINT('Ctrl Pts',(3.23838151080319,-1.,2.5047036758003));
#39164=CARTESIAN_POINT('Ctrl Pts',(3.23089822320646,-1.,2.50276671338111));
#39165=CARTESIAN_POINT('Ctrl Pts',(3.22343262620503,-1.,2.50079587201958));
#39166=CARTESIAN_POINT('Ctrl Pts',(3.21598526261286,-1.,2.4987911459939));
#39167=CARTESIAN_POINT('Ctrl Pts',(3.20855669849836,-1.,2.4967525264737));
#39168=CARTESIAN_POINT('Ctrl Pts',(3.20114742397588,-1.,2.49467992057755));
#39169=CARTESIAN_POINT('Ctrl Pts',(3.19375775555798,-1.,2.49257307239848));
#39170=CARTESIAN_POINT('Ctrl Pts',(3.18638771282266,-1.,2.49043146334059));
#39171=CARTESIAN_POINT('Ctrl Pts',(3.17903698136622,-1.,2.48825428288201));
#39172=CARTESIAN_POINT('Ctrl Pts',(3.17170518863313,-1.,2.48604065348587));
#39173=CARTESIAN_POINT('Ctrl Pts',(3.16439213290161,-1.,2.48378981792725));
#39174=CARTESIAN_POINT('Ctrl Pts',(3.15709802322739,-1.,2.48150133566571));
#39175=CARTESIAN_POINT('Ctrl Pts',(3.14982373241352,-1.,2.47917529057029));
#39176=CARTESIAN_POINT('Ctrl Pts',(3.1425709954655,-1.,2.47681245356109));
#39177=CARTESIAN_POINT('Ctrl Pts',(3.13534181229295,-1.,2.47441378371932));
#39178=CARTESIAN_POINT('Ctrl Pts',(3.12813790805952,-1.,2.47197997765871));
#39179=CARTESIAN_POINT('Ctrl Pts',(3.12096015766983,-1.,2.46951098947469));
#39180=CARTESIAN_POINT('Ctrl Pts',(3.11380805536122,-1.,2.46700558843506));
#39181=CARTESIAN_POINT('Ctrl Pts',(3.1066790790198,-1.,2.46446082979646));
#39182=CARTESIAN_POINT('Ctrl Pts',(3.09956993697052,-1.,2.46187308501884));
#39183=CARTESIAN_POINT('Ctrl Pts',(3.09247787931887,-1.,2.4592391256388));
#39184=CARTESIAN_POINT('Ctrl Pts',(3.08540206545315,-1.,2.45655725437039));
#39185=CARTESIAN_POINT('Ctrl Pts',(3.07834472886139,-1.,2.4538282678779));
#39186=CARTESIAN_POINT('Ctrl Pts',(3.07131290521297,-1.,2.45105688854422));
#39187=CARTESIAN_POINT('Ctrl Pts',(3.06431596421405,-1.,2.44824970516544));
#39188=CARTESIAN_POINT('Ctrl Pts',(3.05736242671506,-1.,2.44541251892556));
#39189=CARTESIAN_POINT('Ctrl Pts',(3.05045678021504,-1.,2.44254768923105));
#39190=CARTESIAN_POINT('Ctrl Pts',(3.04359685040555,-1.,2.43965194061857));
#39191=CARTESIAN_POINT('Ctrl Pts',(3.03676949672821,-1.,2.43671278042414));
#39192=CARTESIAN_POINT('Ctrl Pts',(3.02995534946978,-1.,2.43371241361488));
#39193=CARTESIAN_POINT('Ctrl Pts',(3.02313656036004,-1.,2.43063415586637));
#39194=CARTESIAN_POINT('Ctrl Pts',(3.01630420830504,-1.,2.42746856264168));
#39195=CARTESIAN_POINT('Ctrl Pts',(3.00946442616658,-1.,2.42421849439613));
#39196=CARTESIAN_POINT('Ctrl Pts',(3.00264868585996,-1.,2.42090763946779));
#39197=CARTESIAN_POINT('Ctrl Pts',(2.99590509293503,-1.,2.41757324500514));
#39198=CARTESIAN_POINT('Ctrl Pts',(2.98927983005796,-1.,2.41425064199586));
#39199=CARTESIAN_POINT('Ctrl Pts',(2.98280015815107,-1.,2.41095909342571));
#39200=CARTESIAN_POINT('Ctrl Pts',(2.97646002822422,-1.,2.40768975073713));
#39201=CARTESIAN_POINT('Ctrl Pts',(2.9701964131236,-1.,2.40438604734919));
#39202=CARTESIAN_POINT('Ctrl Pts',(2.96390432240312,-1.,2.4009556571164));
#39203=CARTESIAN_POINT('Ctrl Pts',(2.95748006482942,-1.,2.39730553974517));
#39204=CARTESIAN_POINT('Ctrl Pts',(2.95085857128439,-1.,2.39337207631667));
#39205=CARTESIAN_POINT('Ctrl Pts',(2.94404820669076,-1.,2.38914929090759));
#39206=CARTESIAN_POINT('Ctrl Pts',(2.93717903280391,-1.,2.38472771516311));
#39207=CARTESIAN_POINT('Ctrl Pts',(2.93049643640206,-1.,2.38028989582073));
#39208=CARTESIAN_POINT('Ctrl Pts',(2.92430340582608,-1.,2.3760651052403));
#39209=CARTESIAN_POINT('Ctrl Pts',(2.91891503791411,-1.,2.37229381109821));
#39210=CARTESIAN_POINT('Ctrl Pts',(2.9146124988314,-1.,2.36919161373173));
#39211=CARTESIAN_POINT('Ctrl Pts',(2.91181344022548,-1.,2.36707658451664));
#39212=CARTESIAN_POINT('Ctrl Pts',(2.91051690822156,-1.,2.36599991765749));
#39213=CARTESIAN_POINT('Ctrl Pts',(2.91005770527719,-1.,2.36553202948613));
#39214=CARTESIAN_POINT('Ctrl Pts',(2.90995756655606,-1.,2.36536211188453));
#39215=CARTESIAN_POINT('Ctrl Pts',(2.90994629141676,-1.,2.36531447826074));
#39216=CARTESIAN_POINT('',(2.79140942341378,-1.,2.50410331873042));
#39217=CARTESIAN_POINT('Origin',(0.,-1.,0.));
#39218=CARTESIAN_POINT('',(3.02314558451372,-1.,2.91557726271063));
#39219=CARTESIAN_POINT('Ctrl Pts',(2.79140942341378,-1.,2.50410331873043));
#39220=CARTESIAN_POINT('Ctrl Pts',(2.79145823440899,-1.,2.50410700351427));
#39221=CARTESIAN_POINT('Ctrl Pts',(2.79164172519039,-1.,2.50417932839343));
#39222=CARTESIAN_POINT('Ctrl Pts',(2.79217568804874,-1.,2.50455968395235));
#39223=CARTESIAN_POINT('Ctrl Pts',(2.79344192164204,-1.,2.50567182569153));
#39224=CARTESIAN_POINT('Ctrl Pts',(2.7959687805717,-1.,2.50810555977564));
#39225=CARTESIAN_POINT('Ctrl Pts',(2.79970585014308,-1.,2.51186983687947));
#39226=CARTESIAN_POINT('Ctrl Pts',(2.80427363984939,-1.,2.51660190466067));
#39227=CARTESIAN_POINT('Ctrl Pts',(2.80941521967234,-1.,2.52205778589922));
#39228=CARTESIAN_POINT('Ctrl Pts',(2.8148437904867,-1.,2.52796388055457));
#39229=CARTESIAN_POINT('Ctrl Pts',(2.82028550483744,-1.,2.53405679667463));
#39230=CARTESIAN_POINT('Ctrl Pts',(2.82552167649157,-1.,2.54012272520141));
#39231=CARTESIAN_POINT('Ctrl Pts',(2.83044254225794,-1.,2.54604736792542));
#39232=CARTESIAN_POINT('Ctrl Pts',(2.83505269592412,-1.,2.55182152806964));
#39233=CARTESIAN_POINT('Ctrl Pts',(2.83942515220699,-1.,2.55749952145165));
#39234=CARTESIAN_POINT('Ctrl Pts',(2.84366802680211,-1.,2.56316920798489));
#39235=CARTESIAN_POINT('Ctrl Pts',(2.84788893329091,-1.,2.56891984251743));
#39236=CARTESIAN_POINT('Ctrl Pts',(2.85215360144482,-1.,2.57480482727128));
#39237=CARTESIAN_POINT('Ctrl Pts',(2.85647171715147,-1.,2.58082875254407));
#39238=CARTESIAN_POINT('Ctrl Pts',(2.86081999003668,-1.,2.5869677064356));
#39239=CARTESIAN_POINT('Ctrl Pts',(2.86515629953528,-1.,2.59318160184921));
#39240=CARTESIAN_POINT('Ctrl Pts',(2.86943633170712,-1.,2.59942875223202));
#39241=CARTESIAN_POINT('Ctrl Pts',(2.87363176656475,-1.,2.6056817788128));
#39242=CARTESIAN_POINT('Ctrl Pts',(2.87773881947885,-1.,2.61193507170928));
#39243=CARTESIAN_POINT('Ctrl Pts',(2.88176821427502,-1.,2.61819596473087));
#39244=CARTESIAN_POINT('Ctrl Pts',(2.88573922195049,-1.,2.62447947640253));
#39245=CARTESIAN_POINT('Ctrl Pts',(2.88967244854243,-1.,2.63080195420771));
#39246=CARTESIAN_POINT('Ctrl Pts',(2.89358228854557,-1.,2.63717442263944));
#39247=CARTESIAN_POINT('Ctrl Pts',(2.89747231723361,-1.,2.64359851684146));
#39248=CARTESIAN_POINT('Ctrl Pts',(2.90133950224879,-1.,2.65007017365576));
#39249=CARTESIAN_POINT('Ctrl Pts',(2.90517678087467,-1.,2.65658188464287));
#39250=CARTESIAN_POINT('Ctrl Pts',(2.90897617968921,-1.,2.66312542616809));
#39251=CARTESIAN_POINT('Ctrl Pts',(2.91273193382876,-1.,2.66969458792627));
#39252=CARTESIAN_POINT('Ctrl Pts',(2.91644290704281,-1.,2.67628728855309));
#39253=CARTESIAN_POINT('Ctrl Pts',(2.92011090722152,-1.,2.68290409279689));
#39254=CARTESIAN_POINT('Ctrl Pts',(2.92373955325876,-1.,2.68954721165342));
#39255=CARTESIAN_POINT('Ctrl Pts',(2.92733294395268,-1.,2.69621932864302));
#39256=CARTESIAN_POINT('Ctrl Pts',(2.93089438233746,-1.,2.70292247416881));
#39257=CARTESIAN_POINT('Ctrl Pts',(2.93442516311167,-1.,2.70965695523776));
#39258=CARTESIAN_POINT('Ctrl Pts',(2.93792519474955,-1.,2.71642190053575));
#39259=CARTESIAN_POINT('Ctrl Pts',(2.94139351933882,-1.,2.72321571511322));
#39260=CARTESIAN_POINT('Ctrl Pts',(2.94482887675139,-1.,2.73003657371613));
#39261=CARTESIAN_POINT('Ctrl Pts',(2.94823023414381,-1.,2.73688288329825));
#39262=CARTESIAN_POINT('Ctrl Pts',(2.95159737214304,-1.,2.7437537949221));
#39263=CARTESIAN_POINT('Ctrl Pts',(2.95493069316211,-1.,2.75064903318996));
#39264=CARTESIAN_POINT('Ctrl Pts',(2.9582309766594,-1.,2.75756867888393));
#39265=CARTESIAN_POINT('Ctrl Pts',(2.96149914764832,-1.,2.76451296269571));
#39266=CARTESIAN_POINT('Ctrl Pts',(2.96473605585548,-1.,2.77148206836464));
#39267=CARTESIAN_POINT('Ctrl Pts',(2.9679422104295,-1.,2.77847589542767));
#39268=CARTESIAN_POINT('Ctrl Pts',(2.97111781461349,-1.,2.78549409123657));
#39269=CARTESIAN_POINT('Ctrl Pts',(2.97426288347475,-1.,2.79253615718147));
#39270=CARTESIAN_POINT('Ctrl Pts',(2.97737733718242,-1.,2.79960153278186));
#39271=CARTESIAN_POINT('Ctrl Pts',(2.98046109647299,-1.,2.80668968101162));
#39272=CARTESIAN_POINT('Ctrl Pts',(2.9835141977994,-1.,2.81380019196454));
#39273=CARTESIAN_POINT('Ctrl Pts',(2.98653680669434,-1.,2.82093279065704));
#39274=CARTESIAN_POINT('Ctrl Pts',(2.98952916401699,-1.,2.82808728190402));
#39275=CARTESIAN_POINT('Ctrl Pts',(2.99249155170479,-1.,2.83526351254383));
#39276=CARTESIAN_POINT('Ctrl Pts',(2.995424253416,-1.,2.84246132984334));
#39277=CARTESIAN_POINT('Ctrl Pts',(2.99832751144566,-1.,2.84968053289104));
#39278=CARTESIAN_POINT('Ctrl Pts',(3.0012015079552,-1.,2.85692085715129));
#39279=CARTESIAN_POINT('Ctrl Pts',(3.00404638316245,-1.,2.86418200833065));
#39280=CARTESIAN_POINT('Ctrl Pts',(3.00686224485374,-1.,2.87146368430104));
#39281=CARTESIAN_POINT('Ctrl Pts',(3.0096491810855,-1.,2.87876560072799));
#39282=CARTESIAN_POINT('Ctrl Pts',(3.01240727309568,-1.,2.88608751706796));
#39283=CARTESIAN_POINT('Ctrl Pts',(3.01513660433291,-1.,2.8934292556764));
#39284=CARTESIAN_POINT('Ctrl Pts',(3.01783725123646,-1.,2.90079069102661));
#39285=CARTESIAN_POINT('Ctrl Pts',(3.01997487194926,-1.,2.90669553303902));
#39286=CARTESIAN_POINT('Ctrl Pts',(3.02156522743299,-1.,2.91113297349052));
#39287=CARTESIAN_POINT('Ctrl Pts',(3.02261975104912,-1.,2.91409518070707));
#39288=CARTESIAN_POINT('Ctrl Pts',(3.02314558451372,-1.,2.91557726271063));
#39289=CARTESIAN_POINT('',(2.91557726271063,-1.,3.02314558451372));
#39290=CARTESIAN_POINT('',(3.02314558451372,-1.,2.91557726271063));
#39291=CARTESIAN_POINT('',(2.50410331873176,-1.,2.79140942341258));
#39292=CARTESIAN_POINT('Ctrl Pts',(2.91557726271063,-1.,3.02314558451372));
#39293=CARTESIAN_POINT('Ctrl Pts',(2.91409518070399,-1.,3.02261975104593));
#39294=CARTESIAN_POINT('Ctrl Pts',(2.91113297348212,-1.,3.02156522742431));
#39295=CARTESIAN_POINT('Ctrl Pts',(2.90669553302526,-1.,3.01997487193503));
#39296=CARTESIAN_POINT('Ctrl Pts',(2.9007906910105,-1.,3.01783725121981));
#39297=CARTESIAN_POINT('Ctrl Pts',(2.89342925566321,-1.,3.01513660431928));
#39298=CARTESIAN_POINT('Ctrl Pts',(2.8860875170608,-1.,3.01240727308829));
#39299=CARTESIAN_POINT('Ctrl Pts',(2.87876560072727,-1.,3.00964918108476));
#39300=CARTESIAN_POINT('Ctrl Pts',(2.87146368430501,-1.,3.00686224485784));
#39301=CARTESIAN_POINT('Ctrl Pts',(2.86418200833667,-1.,3.00404638316867));
#39302=CARTESIAN_POINT('Ctrl Pts',(2.85692085715685,-1.,3.00120150796095));
#39303=CARTESIAN_POINT('Ctrl Pts',(2.84968053289451,-1.,2.99832751144925));
#39304=CARTESIAN_POINT('Ctrl Pts',(2.84246132984415,-1.,2.99542425341685));
#39305=CARTESIAN_POINT('Ctrl Pts',(2.83526351254248,-1.,2.9924915517034));
#39306=CARTESIAN_POINT('Ctrl Pts',(2.82808728190157,-1.,2.98952916401446));
#39307=CARTESIAN_POINT('Ctrl Pts',(2.82093279065457,-1.,2.9865368066918));
#39308=CARTESIAN_POINT('Ctrl Pts',(2.81380019196286,-1.,2.98351419779767));
#39309=CARTESIAN_POINT('Ctrl Pts',(2.80668968101106,-1.,2.98046109647241));
#39310=CARTESIAN_POINT('Ctrl Pts',(2.7996015327823,-1.,2.97737733718287));
#39311=CARTESIAN_POINT('Ctrl Pts',(2.79253615718248,-1.,2.9742628834758));
#39312=CARTESIAN_POINT('Ctrl Pts',(2.78549409123769,-1.,2.97111781461465));
#39313=CARTESIAN_POINT('Ctrl Pts',(2.7784758954285,-1.,2.96794221043036));
#39314=CARTESIAN_POINT('Ctrl Pts',(2.77148206836498,-1.,2.96473605585583));
#39315=CARTESIAN_POINT('Ctrl Pts',(2.76451296269557,-1.,2.96149914764818));
#39316=CARTESIAN_POINT('Ctrl Pts',(2.7575686788835,-1.,2.95823097665896));
#39317=CARTESIAN_POINT('Ctrl Pts',(2.75064903318947,-1.,2.95493069316161));
#39318=CARTESIAN_POINT('Ctrl Pts',(2.74375379492172,-1.,2.95159737214266));
#39319=CARTESIAN_POINT('Ctrl Pts',(2.73688288329808,-1.,2.94823023414364));
#39320=CARTESIAN_POINT('Ctrl Pts',(2.73003657371616,-1.,2.94482887675143));
#39321=CARTESIAN_POINT('Ctrl Pts',(2.72321571511337,-1.,2.94139351933897));
#39322=CARTESIAN_POINT('Ctrl Pts',(2.71642190053592,-1.,2.93792519474972));
#39323=CARTESIAN_POINT('Ctrl Pts',(2.70965695523787,-1.,2.93442516311179));
#39324=CARTESIAN_POINT('Ctrl Pts',(2.70292247416885,-1.,2.9308943823375));
#39325=CARTESIAN_POINT('Ctrl Pts',(2.69621932864301,-1.,2.92733294395267));
#39326=CARTESIAN_POINT('Ctrl Pts',(2.68954721165339,-1.,2.92373955325875));
#39327=CARTESIAN_POINT('Ctrl Pts',(2.68290409279688,-1.,2.92011090722152));
#39328=CARTESIAN_POINT('Ctrl Pts',(2.67628728855312,-1.,2.91644290704285));
#39329=CARTESIAN_POINT('Ctrl Pts',(2.66969458792631,-1.,2.91273193382882));
#39330=CARTESIAN_POINT('Ctrl Pts',(2.6631254261681,-1.,2.90897617968923));
#39331=CARTESIAN_POINT('Ctrl Pts',(2.65658188464282,-1.,2.90517678087461));
#39332=CARTESIAN_POINT('Ctrl Pts',(2.65007017365564,-1.,2.90133950224867));
#39333=CARTESIAN_POINT('Ctrl Pts',(2.64359851684131,-1.,2.89747231723345));
#39334=CARTESIAN_POINT('Ctrl Pts',(2.63717442263932,-1.,2.89358228854544));
#39335=CARTESIAN_POINT('Ctrl Pts',(2.63080195420767,-1.,2.88967244854239));
#39336=CARTESIAN_POINT('Ctrl Pts',(2.62447947640262,-1.,2.88573922195059));
#39337=CARTESIAN_POINT('Ctrl Pts',(2.61819596473108,-1.,2.88176821427525));
#39338=CARTESIAN_POINT('Ctrl Pts',(2.61193507170955,-1.,2.87773881947916));
#39339=CARTESIAN_POINT('Ctrl Pts',(2.60568177881303,-1.,2.87363176656501));
#39340=CARTESIAN_POINT('Ctrl Pts',(2.5994287522321,-1.,2.86943633170722));
#39341=CARTESIAN_POINT('Ctrl Pts',(2.59318160184908,-1.,2.86515629953513));
#39342=CARTESIAN_POINT('Ctrl Pts',(2.58696770643524,-1.,2.86081999003629));
#39343=CARTESIAN_POINT('Ctrl Pts',(2.58082875254357,-1.,2.85647171715092));
#39344=CARTESIAN_POINT('Ctrl Pts',(2.57480482727081,-1.,2.85215360144431));
#39345=CARTESIAN_POINT('Ctrl Pts',(2.56891984251721,-1.,2.84788893329067));
#39346=CARTESIAN_POINT('Ctrl Pts',(2.56316920798513,-1.,2.84366802680237));
#39347=CARTESIAN_POINT('Ctrl Pts',(2.55749952145241,-1.,2.83942515220782));
#39348=CARTESIAN_POINT('Ctrl Pts',(2.55182152807077,-1.,2.83505269592536));
#39349=CARTESIAN_POINT('Ctrl Pts',(2.54604736792655,-1.,2.83044254225917));
#39350=CARTESIAN_POINT('Ctrl Pts',(2.54012272520199,-1.,2.8255216764922));
#39351=CARTESIAN_POINT('Ctrl Pts',(2.53405679667412,-1.,2.82028550483689));
#39352=CARTESIAN_POINT('Ctrl Pts',(2.52796388055278,-1.,2.81484379048475));
#39353=CARTESIAN_POINT('Ctrl Pts',(2.52205778589653,-1.,2.80941521966941));
#39354=CARTESIAN_POINT('Ctrl Pts',(2.51660190465805,-1.,2.80427363984653));
#39355=CARTESIAN_POINT('Ctrl Pts',(2.51186983687818,-1.,2.79970585014168));
#39356=CARTESIAN_POINT('Ctrl Pts',(2.5081055597767,-1.,2.79596878057287));
#39357=CARTESIAN_POINT('Ctrl Pts',(2.50567182569081,-1.,2.79344192164147));
#39358=CARTESIAN_POINT('Ctrl Pts',(2.50455968395146,-1.,2.79217568804755));
#39359=CARTESIAN_POINT('Ctrl Pts',(2.50417932839313,-1.,2.79164172518905));
#39360=CARTESIAN_POINT('Ctrl Pts',(2.50410700351493,-1.,2.79145823440781));
#39361=CARTESIAN_POINT('Ctrl Pts',(2.50410331873176,-1.,2.79140942341258));
#39362=CARTESIAN_POINT('',(2.36531447826213,-1.,2.90994629141563));
#39363=CARTESIAN_POINT('Origin',(0.,-1.,0.));
#39364=CARTESIAN_POINT('',(2.52982887637028,-1.,3.35260583073571));
#39365=CARTESIAN_POINT('Ctrl Pts',(2.36531447826213,-1.,2.90994629141563));
#39366=CARTESIAN_POINT('Ctrl Pts',(2.3653621118858,-1.,2.90995756655559));
#39367=CARTESIAN_POINT('Ctrl Pts',(2.36553202948741,-1.,2.9100577052777));
#39368=CARTESIAN_POINT('Ctrl Pts',(2.36599991765853,-1.,2.91051690822262));
#39369=CARTESIAN_POINT('Ctrl Pts',(2.36707658451709,-1.,2.91181344022628));
#39370=CARTESIAN_POINT('Ctrl Pts',(2.36919161373074,-1.,2.91461249883016));
#39371=CARTESIAN_POINT('Ctrl Pts',(2.37229381109939,-1.,2.9189150379156));
#39372=CARTESIAN_POINT('Ctrl Pts',(2.37606510524271,-1.,2.92430340582912));
#39373=CARTESIAN_POINT('Ctrl Pts',(2.3802898958232,-1.,2.93049643640517));
#39374=CARTESIAN_POINT('Ctrl Pts',(2.38472771516476,-1.,2.93717903280599));
#39375=CARTESIAN_POINT('Ctrl Pts',(2.38914929090806,-1.,2.94404820669135));
#39376=CARTESIAN_POINT('Ctrl Pts',(2.39337207631613,-1.,2.95085857128372));
#39377=CARTESIAN_POINT('Ctrl Pts',(2.39730553974412,-1.,2.95748006482811));
#39378=CARTESIAN_POINT('Ctrl Pts',(2.40095565711535,-1.,2.96390432240181));
#39379=CARTESIAN_POINT('Ctrl Pts',(2.40438604734848,-1.,2.97019641312272));
#39380=CARTESIAN_POINT('Ctrl Pts',(2.40768975073691,-1.,2.97646002822395));
#39381=CARTESIAN_POINT('Ctrl Pts',(2.41095909342591,-1.,2.98280015815132));
#39382=CARTESIAN_POINT('Ctrl Pts',(2.4142506419963,-1.,2.98927983005851));
#39383=CARTESIAN_POINT('Ctrl Pts',(2.4175732450056,-1.,2.99590509293561));
#39384=CARTESIAN_POINT('Ctrl Pts',(2.42090763946812,-1.,3.00264868586038));
#39385=CARTESIAN_POINT('Ctrl Pts',(2.42421849439625,-1.,3.00946442616674));
#39386=CARTESIAN_POINT('Ctrl Pts',(2.4274685626416,-1.,3.01630420830494));
#39387=CARTESIAN_POINT('Ctrl Pts',(2.43063415586615,-1.,3.02313656035977));
#39388=CARTESIAN_POINT('Ctrl Pts',(2.43371241361462,-1.,3.02995534946946));
#39389=CARTESIAN_POINT('Ctrl Pts',(2.43671278042394,-1.,3.03676949672797));
#39390=CARTESIAN_POINT('Ctrl Pts',(2.43965194061849,-1.,3.04359685040545));
#39391=CARTESIAN_POINT('Ctrl Pts',(2.44254768923109,-1.,3.05045678021509));
#39392=CARTESIAN_POINT('Ctrl Pts',(2.44541251892568,-1.,3.05736242671521));
#39393=CARTESIAN_POINT('Ctrl Pts',(2.44824970516557,-1.,3.06431596421422));
#39394=CARTESIAN_POINT('Ctrl Pts',(2.45105688854432,-1.,3.0713129052131));
#39395=CARTESIAN_POINT('Ctrl Pts',(2.45382826787795,-1.,3.07834472886145));
#39396=CARTESIAN_POINT('Ctrl Pts',(2.45655725437037,-1.,3.08540206545313));
#39397=CARTESIAN_POINT('Ctrl Pts',(2.45923912563875,-1.,3.09247787931881));
#39398=CARTESIAN_POINT('Ctrl Pts',(2.4618730850188,-1.,3.09956993697048));
#39399=CARTESIAN_POINT('Ctrl Pts',(2.46446082979645,-1.,3.10667907901981));
#39400=CARTESIAN_POINT('Ctrl Pts',(2.46700558843507,-1.,3.11380805536124));
#39401=CARTESIAN_POINT('Ctrl Pts',(2.4695109894747,-1.,3.12096015766984));
#39402=CARTESIAN_POINT('Ctrl Pts',(2.47197997765868,-1.,3.12813790805948));
#39403=CARTESIAN_POINT('Ctrl Pts',(2.47441378371923,-1.,3.13534181229282));
#39404=CARTESIAN_POINT('Ctrl Pts',(2.47681245356095,-1.,3.14257099546531));
#39405=CARTESIAN_POINT('Ctrl Pts',(2.47917529057016,-1.,3.14982373241335));
#39406=CARTESIAN_POINT('Ctrl Pts',(2.48150133566568,-1.,3.15709802322735));
#39407=CARTESIAN_POINT('Ctrl Pts',(2.48378981792739,-1.,3.16439213290181));
#39408=CARTESIAN_POINT('Ctrl Pts',(2.48604065348619,-1.,3.17170518863357));
#39409=CARTESIAN_POINT('Ctrl Pts',(2.48825428288242,-1.,3.17903698136679));
#39410=CARTESIAN_POINT('Ctrl Pts',(2.49043146334095,-1.,3.18638771282315));
#39411=CARTESIAN_POINT('Ctrl Pts',(2.4925730723986,-1.,3.19375775555814));
#39412=CARTESIAN_POINT('Ctrl Pts',(2.49467992057726,-1.,3.20114742397549));
#39413=CARTESIAN_POINT('Ctrl Pts',(2.49675252647298,-1.,3.2085566984974));
#39414=CARTESIAN_POINT('Ctrl Pts',(2.49879114599293,-1.,3.21598526261157));
#39415=CARTESIAN_POINT('Ctrl Pts',(2.5007958720187,-1.,3.22343262620387));
#39416=CARTESIAN_POINT('Ctrl Pts',(2.50276671338074,-1.,3.23089822320596));
#39417=CARTESIAN_POINT('Ctrl Pts',(2.50470367580078,-1.,3.23838151080383));
#39418=CARTESIAN_POINT('Ctrl Pts',(2.50660685940645,-1.,3.24588208984042));
#39419=CARTESIAN_POINT('Ctrl Pts',(2.50847647070936,-1.,3.25339971461265));
#39420=CARTESIAN_POINT('Ctrl Pts',(2.51031277813697,-1.,3.26093423001716));
#39421=CARTESIAN_POINT('Ctrl Pts',(2.51211608411539,-1.,3.26848552888271));
#39422=CARTESIAN_POINT('Ctrl Pts',(2.51388669270329,-1.,3.27605350473048));
#39423=CARTESIAN_POINT('Ctrl Pts',(2.51562487464214,-1.,3.28363799702583));
#39424=CARTESIAN_POINT('Ctrl Pts',(2.51733085123316,-1.,3.2912387729863));
#39425=CARTESIAN_POINT('Ctrl Pts',(2.51900480700548,-1.,3.29885556387661));
#39426=CARTESIAN_POINT('Ctrl Pts',(2.52064689568167,-1.,3.30648808814986));
#39427=CARTESIAN_POINT('Ctrl Pts',(2.52225724871375,-1.,3.31413607874727));
#39428=CARTESIAN_POINT('Ctrl Pts',(2.52383598396878,-1.,3.32179931079521));
#39429=CARTESIAN_POINT('Ctrl Pts',(2.52538321165774,-1.,3.32947762189049));
#39430=CARTESIAN_POINT('Ctrl Pts',(2.52689902691551,-1.,3.33717090000955));
#39431=CARTESIAN_POINT('Ctrl Pts',(2.52808660916879,-1.,3.34333744117093));
#39432=CARTESIAN_POINT('Ctrl Pts',(2.5289632161143,-1.,3.34796903577628));
#39433=CARTESIAN_POINT('Ctrl Pts',(2.52954136549357,-1.,3.35105973714426));
#39434=CARTESIAN_POINT('Ctrl Pts',(2.52982887637028,-1.,3.35260583073571));
#39435=CARTESIAN_POINT('',(2.40675750623143,-1.,3.44202241512147));
#39436=CARTESIAN_POINT('',(2.52982887637028,-1.,3.35260583073571));
#39437=CARTESIAN_POINT('',(2.03660101169714,-1.,3.14877060440328));
#39438=CARTESIAN_POINT('Ctrl Pts',(2.40675750623143,-1.,3.44202241512147));
#39439=CARTESIAN_POINT('Ctrl Pts',(2.4053759295909,-1.,3.44127120683039));
#39440=CARTESIAN_POINT('Ctrl Pts',(2.40261515589405,-1.,3.43976627484234));
#39441=CARTESIAN_POINT('Ctrl Pts',(2.39848113410292,-1.,3.43750133064416));
#39442=CARTESIAN_POINT('Ctrl Pts',(2.39298338804493,-1.,3.4344663067854));
#39443=CARTESIAN_POINT('Ctrl Pts',(2.38613505843552,-1.,3.4306473271292));
#39444=CARTESIAN_POINT('Ctrl Pts',(2.37931067028926,-1.,3.42680309754399));
#39445=CARTESIAN_POINT('Ctrl Pts',(2.37251035954292,-1.,3.42293356216511));
#39446=CARTESIAN_POINT('Ctrl Pts',(2.36573431470642,-1.,3.41903866635852));
#39447=CARTESIAN_POINT('Ctrl Pts',(2.35898278606946,-1.,3.41511836751469));
#39448=CARTESIAN_POINT('Ctrl Pts',(2.35225606824109,-1.,3.41117262314119));
#39449=CARTESIAN_POINT('Ctrl Pts',(2.34555447649188,-1.,3.40720137404297));
#39450=CARTESIAN_POINT('Ctrl Pts',(2.33887832342782,-1.,3.40320452776743));
#39451=CARTESIAN_POINT('Ctrl Pts',(2.33222789882489,-1.,3.39918194577956));
#39452=CARTESIAN_POINT('Ctrl Pts',(2.3256034390248,-1.,3.39513342019756));
#39453=CARTESIAN_POINT('Ctrl Pts',(2.31900513925424,-1.,3.39105869474822));
#39454=CARTESIAN_POINT('Ctrl Pts',(2.31243319489367,-1.,3.38695751492462));
#39455=CARTESIAN_POINT('Ctrl Pts',(2.30588783640343,-1.,3.3828296733661));
#39456=CARTESIAN_POINT('Ctrl Pts',(2.29936936127624,-1.,3.37867504959433));
#39457=CARTESIAN_POINT('Ctrl Pts',(2.29287818007393,-1.,3.37449367172826));
#39458=CARTESIAN_POINT('Ctrl Pts',(2.28641481081137,-1.,3.37028570206488));
#39459=CARTESIAN_POINT('Ctrl Pts',(2.27997979458037,-1.,3.36605130713076));
#39460=CARTESIAN_POINT('Ctrl Pts',(2.2735736262093,-1.,3.36179055004409));
#39461=CARTESIAN_POINT('Ctrl Pts',(2.26719668579909,-1.,3.35750328523061));
#39462=CARTESIAN_POINT('Ctrl Pts',(2.26084915222449,-1.,3.35318902552626));
#39463=CARTESIAN_POINT('Ctrl Pts',(2.25453097693483,-1.,3.34884690292285));
#39464=CARTESIAN_POINT('Ctrl Pts',(2.24824207678256,-1.,3.34447596770723));
#39465=CARTESIAN_POINT('Ctrl Pts',(2.24198249391422,-1.,3.34007543738025));
#39466=CARTESIAN_POINT('Ctrl Pts',(2.23575256328812,-1.,3.33564495756482));
#39467=CARTESIAN_POINT('Ctrl Pts',(2.22955308907233,-1.,3.33118487773611));
#39468=CARTESIAN_POINT('Ctrl Pts',(2.22338548312772,-1.,3.3266964672289));
#39469=CARTESIAN_POINT('Ctrl Pts',(2.21725135110898,-1.,3.32218125618968));
#39470=CARTESIAN_POINT('Ctrl Pts',(2.21115211847875,-1.,3.31764044024235));
#39471=CARTESIAN_POINT('Ctrl Pts',(2.20508863150607,-1.,3.31307424608949));
#39472=CARTESIAN_POINT('Ctrl Pts',(2.19906078949922,-1.,3.30848134694595));
#39473=CARTESIAN_POINT('Ctrl Pts',(2.19306710376111,-1.,3.30385816281831));
#39474=CARTESIAN_POINT('Ctrl Pts',(2.18710556500327,-1.,3.29920022557639));
#39475=CARTESIAN_POINT('Ctrl Pts',(2.18117455557065,-1.,3.2945036150049));
#39476=CARTESIAN_POINT('Ctrl Pts',(2.17527380048423,-1.,3.28976645712568));
#39477=CARTESIAN_POINT('Ctrl Pts',(2.16940517773455,-1.,3.28499019979724));
#39478=CARTESIAN_POINT('Ctrl Pts',(2.16357391934425,-1.,3.280181508414));
#39479=CARTESIAN_POINT('Ctrl Pts',(2.15778690038347,-1.,3.27534954469187));
#39480=CARTESIAN_POINT('Ctrl Pts',(2.15205043199808,-1.,3.27050245897228));
#39481=CARTESIAN_POINT('Ctrl Pts',(2.1463680529566,-1.,3.26564388189759));
#39482=CARTESIAN_POINT('Ctrl Pts',(2.14073870754264,-1.,3.26077002641879));
#39483=CARTESIAN_POINT('Ctrl Pts',(2.13515375878803,-1.,3.25586495065054));
#39484=CARTESIAN_POINT('Ctrl Pts',(2.12960028396832,-1.,3.25090574494028));
#39485=CARTESIAN_POINT('Ctrl Pts',(2.12406646410962,-1.,3.24587102613376));
#39486=CARTESIAN_POINT('Ctrl Pts',(2.11854673326979,-1.,3.24074905517293));
#39487=CARTESIAN_POINT('Ctrl Pts',(2.11304604021773,-1.,3.23554444767099));
#39488=CARTESIAN_POINT('Ctrl Pts',(2.10758699642451,-1.,3.23028945793289));
#39489=CARTESIAN_POINT('Ctrl Pts',(2.10220384298492,-1.,3.22503437553434));
#39490=CARTESIAN_POINT('Ctrl Pts',(2.09692958434895,-1.,3.21982707347009));
#39491=CARTESIAN_POINT('Ctrl Pts',(2.09178419460443,-1.,3.21469429601654));
#39492=CARTESIAN_POINT('Ctrl Pts',(2.08676465517455,-1.,3.20962575845463));
#39493=CARTESIAN_POINT('Ctrl Pts',(2.08182850370878,-1.,3.2045481863073));
#39494=CARTESIAN_POINT('Ctrl Pts',(2.07690441870722,-1.,3.19934132836019));
#39495=CARTESIAN_POINT('Ctrl Pts',(2.07192253497857,-1.,3.19388465568252));
#39496=CARTESIAN_POINT('Ctrl Pts',(2.06684062744112,-1.,3.18809755562368));
#39497=CARTESIAN_POINT('Ctrl Pts',(2.06166849827101,-1.,3.18197692964614));
#39498=CARTESIAN_POINT('Ctrl Pts',(2.05650186773132,-1.,3.17564906975371));
#39499=CARTESIAN_POINT('Ctrl Pts',(2.05151770247233,-1.,3.16936341689527));
#39500=CARTESIAN_POINT('Ctrl Pts',(2.04693331247446,-1.,3.16343165058912));
#39501=CARTESIAN_POINT('Ctrl Pts',(2.04297406404027,-1.,3.15817983946367));
#39502=CARTESIAN_POINT('Ctrl Pts',(2.03984073791519,-1.,3.15389991674792));
#39503=CARTESIAN_POINT('Ctrl Pts',(2.03783225495961,-1.,3.15102344775328));
#39504=CARTESIAN_POINT('Ctrl Pts',(2.03693188810544,-1.,3.14959882629805));
#39505=CARTESIAN_POINT('Ctrl Pts',(2.03663974554932,-1.,3.1490119366901));
#39506=CARTESIAN_POINT('Ctrl Pts',(2.03659701539259,-1.,3.14881939088124));
#39507=CARTESIAN_POINT('Ctrl Pts',(2.03660101169714,-1.,3.14877060440328));
#39508=CARTESIAN_POINT('',(1.88097764062697,-1.,3.24413672884812));
#39509=CARTESIAN_POINT('Origin',(0.,-1.,0.));
#39510=CARTESIAN_POINT('',(1.97421938526992,-1.,3.70708211654725));
#39511=CARTESIAN_POINT('Ctrl Pts',(1.88097764062697,-1.,3.24413672884812));
#39512=CARTESIAN_POINT('Ctrl Pts',(1.8810229239812,-1.,3.24415531671284));
#39513=CARTESIAN_POINT('Ctrl Pts',(1.88117508446775,-1.,3.24428080353022));
#39514=CARTESIAN_POINT('Ctrl Pts',(1.88156537699203,-1.,3.24480754676064));
#39515=CARTESIAN_POINT('Ctrl Pts',(1.88242596600454,-1.,3.2462565441079));
#39516=CARTESIAN_POINT('Ctrl Pts',(1.88407708646357,-1.,3.24935200511918));
#39517=CARTESIAN_POINT('Ctrl Pts',(1.88646802523466,-1.,3.25408686339463));
#39518=CARTESIAN_POINT('Ctrl Pts',(1.88934996203698,-1.,3.25999885193947));
#39519=CARTESIAN_POINT('Ctrl Pts',(1.89255393500965,-1.,3.26677653888676));
#39520=CARTESIAN_POINT('Ctrl Pts',(1.89589172903793,-1.,3.27407108933139));
#39521=CARTESIAN_POINT('Ctrl Pts',(1.89918429230462,-1.,3.28154737912352));
#39522=CARTESIAN_POINT('Ctrl Pts',(1.90228971247527,-1.,3.2889344860029));
#39523=CARTESIAN_POINT('Ctrl Pts',(1.90513891864087,-1.,3.29608978722113));
#39524=CARTESIAN_POINT('Ctrl Pts',(1.90773912171341,-1.,3.30300595568195));
#39525=CARTESIAN_POINT('Ctrl Pts',(1.91014297830446,-1.,3.30975721158596));
#39526=CARTESIAN_POINT('Ctrl Pts',(1.91242616234442,-1.,3.31646052426364));
#39527=CARTESIAN_POINT('Ctrl Pts',(1.91466343916627,-1.,3.32323403454535));
#39528=CARTESIAN_POINT('Ctrl Pts',(1.91690081930331,-1.,3.33014884257873));
#39529=CARTESIAN_POINT('Ctrl Pts',(1.9191460961021,-1.,3.33721230710012));
#39530=CARTESIAN_POINT('Ctrl Pts',(1.92138450828404,-1.,3.34439448941961));
#39531=CARTESIAN_POINT('Ctrl Pts',(1.92358838440528,-1.,3.35164424847223));
#39532=CARTESIAN_POINT('Ctrl Pts',(1.92572846125756,-1.,3.35890824422965));
#39533=CARTESIAN_POINT('Ctrl Pts',(1.92778626543786,-1.,3.36615168657567));
#39534=CARTESIAN_POINT('Ctrl Pts',(1.92975993109877,-1.,3.37336807068043));
#39535=CARTESIAN_POINT('Ctrl Pts',(1.93165739093276,-1.,3.3805676852555));
#39536=CARTESIAN_POINT('Ctrl Pts',(1.93349233176788,-1.,3.38777076883256));
#39537=CARTESIAN_POINT('Ctrl Pts',(1.93527929945985,-1.,3.39499923640795));
#39538=CARTESIAN_POINT('Ctrl Pts',(1.93702857723098,-1.,3.40226802104109));
#39539=CARTESIAN_POINT('Ctrl Pts',(1.93874306008143,-1.,3.40957978266642));
#39540=CARTESIAN_POINT('Ctrl Pts',(1.94042111965246,-1.,3.41692971994096));
#39541=CARTESIAN_POINT('Ctrl Pts',(1.94205835913696,-1.,3.42430850941503));
#39542=CARTESIAN_POINT('Ctrl Pts',(1.94364973660284,-1.,3.43170586602434));
#39543=CARTESIAN_POINT('Ctrl Pts',(1.94519168842879,-1.,3.43911410197687));
#39544=CARTESIAN_POINT('Ctrl Pts',(1.94668377715329,-1.,3.44653088665681));
#39545=CARTESIAN_POINT('Ctrl Pts',(1.94812754766524,-1.,3.45395731584051));
#39546=CARTESIAN_POINT('Ctrl Pts',(1.94952575850197,-1.,3.46139661060962));
#39547=CARTESIAN_POINT('Ctrl Pts',(1.95088147859876,-1.,3.46885258974191));
#39548=CARTESIAN_POINT('Ctrl Pts',(1.95219722189876,-1.,3.47632820495921));
#39549=CARTESIAN_POINT('Ctrl Pts',(1.95347412486308,-1.,3.48382414832634));
#39550=CARTESIAN_POINT('Ctrl Pts',(1.95471236969643,-1.,3.49133956289133));
#39551=CARTESIAN_POINT('Ctrl Pts',(1.95591153823661,-1.,3.49887263575583));
#39552=CARTESIAN_POINT('Ctrl Pts',(1.95707099606511,-1.,3.50642124159909));
#39553=CARTESIAN_POINT('Ctrl Pts',(1.95819025316779,-1.,3.51398354617794));
#39554=CARTESIAN_POINT('Ctrl Pts',(1.95926936324461,-1.,3.52155867431486));
#39555=CARTESIAN_POINT('Ctrl Pts',(1.96030879411566,-1.,3.52914648844351));
#39556=CARTESIAN_POINT('Ctrl Pts',(1.96130926212689,-1.,3.53674730625813));
#39557=CARTESIAN_POINT('Ctrl Pts',(1.96227157573067,-1.,3.54436163300443));
#39558=CARTESIAN_POINT('Ctrl Pts',(1.96319648628644,-1.,3.55198990600886));
#39559=CARTESIAN_POINT('Ctrl Pts',(1.96408450906812,-1.,3.55963218706096));
#39560=CARTESIAN_POINT('Ctrl Pts',(1.96493594634567,-1.,3.56728820357791));
#39561=CARTESIAN_POINT('Ctrl Pts',(1.96575096652789,-1.,3.57495748600959));
#39562=CARTESIAN_POINT('Ctrl Pts',(1.96652966688911,-1.,3.58263947663829));
#39563=CARTESIAN_POINT('Ctrl Pts',(1.96727213799544,-1.,3.59033364022801));
#39564=CARTESIAN_POINT('Ctrl Pts',(1.96797854118369,-1.,3.59803959819938));
#39565=CARTESIAN_POINT('Ctrl Pts',(1.9686491188594,-1.,3.60575714017989));
#39566=CARTESIAN_POINT('Ctrl Pts',(1.96928416040877,-1.,3.61348615496704));
#39567=CARTESIAN_POINT('Ctrl Pts',(1.96988398129978,-1.,3.62122658401893));
#39568=CARTESIAN_POINT('Ctrl Pts',(1.97044889850463,-1.,3.62897836973293));
#39569=CARTESIAN_POINT('Ctrl Pts',(1.97097920454464,-1.,3.63674139590412));
#39570=CARTESIAN_POINT('Ctrl Pts',(1.97147515441164,-1.,3.64451546723514));
#39571=CARTESIAN_POINT('Ctrl Pts',(1.97193697240239,-1.,3.652300347166));
#39572=CARTESIAN_POINT('Ctrl Pts',(1.9723648543905,-1.,3.6600957816636));
#39573=CARTESIAN_POINT('Ctrl Pts',(1.97275897198678,-1.,3.66790152752075));
#39574=CARTESIAN_POINT('Ctrl Pts',(1.97311947678516,-1.,3.67571738107084));
#39575=CARTESIAN_POINT('Ctrl Pts',(1.97344650304519,-1.,3.68354319915092));
#39576=CARTESIAN_POINT('Ctrl Pts',(1.97374016225483,-1.,3.69137888599902));
#39577=CARTESIAN_POINT('Ctrl Pts',(1.97394846383216,-1.,3.6976552856004));
#39578=CARTESIAN_POINT('Ctrl Pts',(1.97408973726715,-1.,3.70236698912904));
#39579=CARTESIAN_POINT('Ctrl Pts',(1.97417727645308,-1.,3.70551008132332));
#39580=CARTESIAN_POINT('Ctrl Pts',(1.97421938526992,-1.,3.70708211654725));
#39581=CARTESIAN_POINT('',(1.8386753923786,-1.,3.77614523045147));
#39582=CARTESIAN_POINT('',(1.97421938526992,-1.,3.70708211654725));
#39583=CARTESIAN_POINT('',(1.5189508286633,-1.,3.42859860294306));
#39584=CARTESIAN_POINT('Ctrl Pts',(1.8386753923786,-1.,3.77614523045147));
#39585=CARTESIAN_POINT('Ctrl Pts',(1.83742834010626,-1.,3.77518714457833));
#39586=CARTESIAN_POINT('Ctrl Pts',(1.83493697934534,-1.,3.77326886064398));
#39587=CARTESIAN_POINT('Ctrl Pts',(1.83120816955645,-1.,3.77038509817999));
#39588=CARTESIAN_POINT('Ctrl Pts',(1.82625289220915,-1.,3.76652740353775));
#39589=CARTESIAN_POINT('Ctrl Pts',(1.82008629694091,-1.,3.76168412707948));
#39590=CARTESIAN_POINT('Ctrl Pts',(1.8139472983358,-1.,3.75681965683071));
#39591=CARTESIAN_POINT('Ctrl Pts',(1.80783603939617,-1.,3.75193395887977));
#39592=CARTESIAN_POINT('Ctrl Pts',(1.8017527148577,-1.,3.74702700875467));
#39593=CARTESIAN_POINT('Ctrl Pts',(1.79569757859422,-1.,3.74209880352445));
#39594=CARTESIAN_POINT('Ctrl Pts',(1.78967092823491,-1.,3.73714934730681));
#39595=CARTESIAN_POINT('Ctrl Pts',(1.78367308442901,-1.,3.7321786309547));
#39596=CARTESIAN_POINT('Ctrl Pts',(1.77770437039658,-1.,3.72718661205609));
#39597=CARTESIAN_POINT('Ctrl Pts',(1.77176509401761,-1.,3.72217319911254));
#39598=CARTESIAN_POINT('Ctrl Pts',(1.76585552124394,-1.,3.71713822377359));
#39599=CARTESIAN_POINT('Ctrl Pts',(1.75997588498865,-1.,3.71208146346136));
#39600=CARTESIAN_POINT('Ctrl Pts',(1.75412641804042,-1.,3.70700269736659));
#39601=CARTESIAN_POINT('Ctrl Pts',(1.74830738046057,-1.,3.7019017567335));
#39602=CARTESIAN_POINT('Ctrl Pts',(1.74251908492617,-1.,3.69677856910517));
#39603=CARTESIAN_POINT('Ctrl Pts',(1.73676193254557,-1.,3.69163322648036));
#39604=CARTESIAN_POINT('Ctrl Pts',(1.73103640956717,-1.,3.68646597019332));
#39605=CARTESIAN_POINT('Ctrl Pts',(1.72534302437056,-1.,3.68127704936579));
#39606=CARTESIAN_POINT('Ctrl Pts',(1.71968225581808,-1.,3.67606660374709));
#39607=CARTESIAN_POINT('Ctrl Pts',(1.71405450210383,-1.,3.67083454901611));
#39608=CARTESIAN_POINT('Ctrl Pts',(1.70846001610956,-1.,3.66558043198876));
#39609=CARTESIAN_POINT('Ctrl Pts',(1.70289888566873,-1.,3.66030338774847));
#39610=CARTESIAN_POINT('Ctrl Pts',(1.69737117722534,-1.,3.65500246526749));
#39611=CARTESIAN_POINT('Ctrl Pts',(1.69187705481689,-1.,3.64967689827371));
#39612=CARTESIAN_POINT('Ctrl Pts',(1.68641690471457,-1.,3.64432638915203));
#39613=CARTESIAN_POINT('Ctrl Pts',(1.68099146651586,-1.,3.63895140887462));
#39614=CARTESIAN_POINT('Ctrl Pts',(1.67560193613156,-1.,3.63355343201232));
#39615=CARTESIAN_POINT('Ctrl Pts',(1.67024966008044,-1.,3.62813422105271));
#39616=CARTESIAN_POINT('Ctrl Pts',(1.66493585923855,-1.,3.62269517989109));
#39617=CARTESIAN_POINT('Ctrl Pts',(1.65966133399186,-1.,3.61723666482456));
#39618=CARTESIAN_POINT('Ctrl Pts',(1.65442619244325,-1.,3.61175734965127));
#39619=CARTESIAN_POINT('Ctrl Pts',(1.64922952425832,-1.,3.60625346556992));
#39620=CARTESIAN_POINT('Ctrl Pts',(1.64407004385582,-1.,3.60072028513845));
#39621=CARTESIAN_POINT('Ctrl Pts',(1.63894676675352,-1.,3.59515368334893));
#39622=CARTESIAN_POINT('Ctrl Pts',(1.6338597145126,-1.,3.58955176627879));
#39623=CARTESIAN_POINT('Ctrl Pts',(1.62881051550745,-1.,3.58391625774343));
#39624=CARTESIAN_POINT('Ctrl Pts',(1.62380329464844,-1.,3.5782545595439));
#39625=CARTESIAN_POINT('Ctrl Pts',(1.61884340915404,-1.,3.57257679609806));
#39626=CARTESIAN_POINT('Ctrl Pts',(1.61393581747514,-1.,3.56689200468387));
#39627=CARTESIAN_POINT('Ctrl Pts',(1.60908344685457,-1.,3.5612043248298));
#39628=CARTESIAN_POINT('Ctrl Pts',(1.60428584699853,-1.,3.55550985096129));
#39629=CARTESIAN_POINT('Ctrl Pts',(1.59953698113457,-1.,3.54979148634454));
#39630=CARTESIAN_POINT('Ctrl Pts',(1.59482766949766,-1.,3.54402458182337));
#39631=CARTESIAN_POINT('Ctrl Pts',(1.59014958368739,-1.,3.53818616861077));
#39632=CARTESIAN_POINT('Ctrl Pts',(1.58549906268088,-1.,3.5322637814708));
#39633=CARTESIAN_POINT('Ctrl Pts',(1.58088027227848,-1.,3.52626275334881));
#39634=CARTESIAN_POINT('Ctrl Pts',(1.57631049988158,-1.,3.52021847865912));
#39635=CARTESIAN_POINT('Ctrl Pts',(1.57181569799743,-1.,3.51418598431665));
#39636=CARTESIAN_POINT('Ctrl Pts',(1.56742097575012,-1.,3.50821771695363));
#39637=CARTESIAN_POINT('Ctrl Pts',(1.56314187758675,-1.,3.50234321621578));
#39638=CARTESIAN_POINT('Ctrl Pts',(1.55897703097874,-1.,3.49655185179655));
#39639=CARTESIAN_POINT('Ctrl Pts',(1.55489595901116,-1.,3.4907646087742));
#39640=CARTESIAN_POINT('Ctrl Pts',(1.55084702970452,-1.,3.48485155928567));
#39641=CARTESIAN_POINT('Ctrl Pts',(1.54678009290276,-1.,3.47868272898751));
#39642=CARTESIAN_POINT('Ctrl Pts',(1.54266605398187,-1.,3.47217189224653));
#39643=CARTESIAN_POINT('Ctrl Pts',(1.53851507915502,-1.,3.46531752207153));
#39644=CARTESIAN_POINT('Ctrl Pts',(1.53440195378792,-1.,3.45825932955032));
#39645=CARTESIAN_POINT('Ctrl Pts',(1.53046244461635,-1.,3.45127136828305));
#39646=CARTESIAN_POINT('Ctrl Pts',(1.52686242875556,-1.,3.44469547526647));
#39647=CARTESIAN_POINT('Ctrl Pts',(1.5237734895035,-1.,3.4388889597401));
#39648=CARTESIAN_POINT('Ctrl Pts',(1.52134826724292,-1.,3.43417156977893));
#39649=CARTESIAN_POINT('Ctrl Pts',(1.5198144909338,-1.,3.43101631893414));
#39650=CARTESIAN_POINT('Ctrl Pts',(1.51914806898491,-1.,3.42946838852587));
#39651=CARTESIAN_POINT('Ctrl Pts',(1.5189513329503,-1.,3.42884302333841));
#39652=CARTESIAN_POINT('Ctrl Pts',(1.51893924967331,-1.,3.42864616361875));
#39653=CARTESIAN_POINT('Ctrl Pts',(1.5189508286633,-1.,3.42859860294306));
#39654=CARTESIAN_POINT('',(1.35032489087269,-1.,3.49844575334386));
#39655=CARTESIAN_POINT('Origin',(0.,-1.,0.));
#39656=CARTESIAN_POINT('',(1.36999806084572,-1.,3.97027773754922));
#39657=CARTESIAN_POINT('Ctrl Pts',(1.35032489087269,-1.,3.49844575334386));
#39658=CARTESIAN_POINT('Ctrl Pts',(1.35036670893102,-1.,3.49847119623841));
#39659=CARTESIAN_POINT('Ctrl Pts',(1.35049736560633,-1.,3.49861894124915));
#39660=CARTESIAN_POINT('Ctrl Pts',(1.35080045218652,-1.,3.49920025459856));
#39661=CARTESIAN_POINT('Ctrl Pts',(1.35142377279535,-1.,3.5007660381658));
#39662=CARTESIAN_POINT('Ctrl Pts',(1.3525703284343,-1.,3.50408168106113));
#39663=CARTESIAN_POINT('Ctrl Pts',(1.35419113576022,-1.,3.50913227060177));
#39664=CARTESIAN_POINT('Ctrl Pts',(1.35611275237288,-1.,3.51542230699919));
#39665=CARTESIAN_POINT('Ctrl Pts',(1.35821701528975,-1.,3.52261776117121));
#39666=CARTESIAN_POINT('Ctrl Pts',(1.36037259643827,-1.,3.53034464961849));
#39667=CARTESIAN_POINT('Ctrl Pts',(1.36245507339334,-1.,3.53824396425032));
#39668=CARTESIAN_POINT('Ctrl Pts',(1.36436666257567,-1.,3.54602591832893));
#39669=CARTESIAN_POINT('Ctrl Pts',(1.36606145456711,-1.,3.55353883995793));
#39670=CARTESIAN_POINT('Ctrl Pts',(1.36754771771174,-1.,3.56077662028492));
#39671=CARTESIAN_POINT('Ctrl Pts',(1.36886584973349,-1.,3.56782080304554));
#39672=CARTESIAN_POINT('Ctrl Pts',(1.37007229485646,-1.,3.57479875549453));
#39673=CARTESIAN_POINT('Ctrl Pts',(1.37122241663073,-1.,3.58183885982745));
#39674=CARTESIAN_POINT('Ctrl Pts',(1.37235053661,-1.,3.5890185384643));
#39675=CARTESIAN_POINT('Ctrl Pts',(1.37346320103184,-1.,3.59634627869117));
#39676=CARTESIAN_POINT('Ctrl Pts',(1.37455051379642,-1.,3.60379020124038));
#39677=CARTESIAN_POINT('Ctrl Pts',(1.37559314436641,-1.,3.61129546591082));
#39678=CARTESIAN_POINT('Ctrl Pts',(1.37657053403102,-1.,3.61880481160408));
#39679=CARTESIAN_POINT('Ctrl Pts',(1.37746987919868,-1.,3.62628098665112));
#39680=CARTESIAN_POINT('Ctrl Pts',(1.37829035457324,-1.,3.63371727442448));
#39681=CARTESIAN_POINT('Ctrl Pts',(1.37903818567347,-1.,3.64112507791112));
#39682=CARTESIAN_POINT('Ctrl Pts',(1.37972372481598,-1.,3.64852652756444));
#39683=CARTESIAN_POINT('Ctrl Pts',(1.38035791051215,-1.,3.65594554404396));
#39684=CARTESIAN_POINT('Ctrl Pts',(1.38094856333558,-1.,3.66339848520874));
#39685=CARTESIAN_POINT('Ctrl Pts',(1.38149812653876,-1.,3.67088843112282));
#39686=CARTESIAN_POINT('Ctrl Pts',(1.38200574290626,-1.,3.6784103848243));
#39687=CARTESIAN_POINT('Ctrl Pts',(1.38246852827185,-1.,3.68595444983844));
#39688=CARTESIAN_POINT('Ctrl Pts',(1.38288311171649,-1.,3.69350967899523));
#39689=CARTESIAN_POINT('Ctrl Pts',(1.38324717612862,-1.,3.70106792167894));
#39690=CARTESIAN_POINT('Ctrl Pts',(1.38356065402122,-1.,3.70862680753343));
#39691=CARTESIAN_POINT('Ctrl Pts',(1.38382489984585,-1.,3.7161876605181));
#39692=CARTESIAN_POINT('Ctrl Pts',(1.3840421342895,-1.,3.72375409358805));
#39693=CARTESIAN_POINT('Ctrl Pts',(1.38421479111531,-1.,3.73133035859283));
#39694=CARTESIAN_POINT('Ctrl Pts',(1.38434489156456,-1.,3.73891976418099));
#39695=CARTESIAN_POINT('Ctrl Pts',(1.38443344984389,-1.,3.7465231716786));
#39696=CARTESIAN_POINT('Ctrl Pts',(1.38448077997155,-1.,3.75413976318727));
#39697=CARTESIAN_POINT('Ctrl Pts',(1.38448675253343,-1.,3.76176768271347));
#39698=CARTESIAN_POINT('Ctrl Pts',(1.38445107339517,-1.,3.76940473185775));
#39699=CARTESIAN_POINT('Ctrl Pts',(1.38437354551435,-1.,3.77704902230441));
#39700=CARTESIAN_POINT('Ctrl Pts',(1.38425435883773,-1.,3.78469969805134));
#39701=CARTESIAN_POINT('Ctrl Pts',(1.38409399694588,-1.,3.79235669640907));
#39702=CARTESIAN_POINT('Ctrl Pts',(1.38389311766701,-1.,3.80002044322169));
#39703=CARTESIAN_POINT('Ctrl Pts',(1.38365244046226,-1.,3.80769156398429));
#39704=CARTESIAN_POINT('Ctrl Pts',(1.38337263902766,-1.,3.81537060817765));
#39705=CARTESIAN_POINT('Ctrl Pts',(1.38305421262724,-1.,3.82305771743715));
#39706=CARTESIAN_POINT('Ctrl Pts',(1.38269750245086,-1.,3.83075266982138));
#39707=CARTESIAN_POINT('Ctrl Pts',(1.38230274828774,-1.,3.83845502790609));
#39708=CARTESIAN_POINT('Ctrl Pts',(1.38187013346089,-1.,3.84616425605705));
#39709=CARTESIAN_POINT('Ctrl Pts',(1.38139983115075,-1.,3.85387983979557));
#39710=CARTESIAN_POINT('Ctrl Pts',(1.38089205993067,-1.,3.86160143044187));
#39711=CARTESIAN_POINT('Ctrl Pts',(1.38034709213129,-1.,3.86932885813403));
#39712=CARTESIAN_POINT('Ctrl Pts',(1.37976523097187,-1.,3.87706205830865));
#39713=CARTESIAN_POINT('Ctrl Pts',(1.37914679719446,-1.,3.88480102249461));
#39714=CARTESIAN_POINT('Ctrl Pts',(1.37849211287981,-1.,3.89254574338385));
#39715=CARTESIAN_POINT('Ctrl Pts',(1.3778014851263,-1.,3.90029615196255));
#39716=CARTESIAN_POINT('Ctrl Pts',(1.3770751963376,-1.,3.90805209522729));
#39717=CARTESIAN_POINT('Ctrl Pts',(1.37631350505516,-1.,3.91581337461825));
#39718=CARTESIAN_POINT('Ctrl Pts',(1.37551664448057,-1.,3.92357976987132));
#39719=CARTESIAN_POINT('Ctrl Pts',(1.37468482215784,-1.,3.93135106761941));
#39720=CARTESIAN_POINT('Ctrl Pts',(1.37381821967499,-1.,3.93912709041791));
#39721=CARTESIAN_POINT('Ctrl Pts',(1.37291699203423,-1.,3.94690771786926));
#39722=CARTESIAN_POINT('Ctrl Pts',(1.37198126433139,-1.,3.95469287283105));
#39723=CARTESIAN_POINT('Ctrl Pts',(1.37120515615663,-1.,3.96092458508407));
#39724=CARTESIAN_POINT('Ctrl Pts',(1.37060761746027,-1.,3.96560037975788));
#39725=CARTESIAN_POINT('Ctrl Pts',(1.37020239094758,-1.,3.9687184694173));
#39726=CARTESIAN_POINT('Ctrl Pts',(1.36999806084572,-1.,3.97027773754922));
#39727=CARTESIAN_POINT('',(1.22531898815164,-1.,4.01728681790024));
#39728=CARTESIAN_POINT('',(1.36999806084572,-1.,3.97027773754922));
#39729=CARTESIAN_POINT('',(0.963899035118985,-1.,3.62400312501199));
#39730=CARTESIAN_POINT('Ctrl Pts',(1.22531898815164,-1.,4.01728681790024));
#39731=CARTESIAN_POINT('Ctrl Pts',(1.22423716681317,-1.,4.01614544569895));
#39732=CARTESIAN_POINT('Ctrl Pts',(1.22207656455845,-1.,4.01386104433519));
#39733=CARTESIAN_POINT('Ctrl Pts',(1.21884478244403,-1.,4.01042947140789));
#39734=CARTESIAN_POINT('Ctrl Pts',(1.21455398918133,-1.,4.00584409522722));
#39735=CARTESIAN_POINT('Ctrl Pts',(1.20922097029551,-1.,4.00009577950721));
#39736=CARTESIAN_POINT('Ctrl Pts',(1.20391852375138,-1.,3.99433084799666));
#39737=CARTESIAN_POINT('Ctrl Pts',(1.19864679609566,-1.,3.98854928957189));
#39738=CARTESIAN_POINT('Ctrl Pts',(1.19340598349475,-1.,3.98275111052561));
#39739=CARTESIAN_POINT('Ctrl Pts',(1.18819633715539,-1.,3.97693634767754));
#39740=CARTESIAN_POINT('Ctrl Pts',(1.18301815039831,-1.,3.97110505165415));
#39741=CARTESIAN_POINT('Ctrl Pts',(1.17787174135592,-1.,3.96525726358159));
#39742=CARTESIAN_POINT('Ctrl Pts',(1.17275743590361,-1.,3.95939299213276));
#39743=CARTESIAN_POINT('Ctrl Pts',(1.16767555244438,-1.,3.95351219509876));
#39744=CARTESIAN_POINT('Ctrl Pts',(1.16262637999157,-1.,3.94761474780583));
#39745=CARTESIAN_POINT('Ctrl Pts',(1.15761018340956,-1.,3.94170046685203));
#39746=CARTESIAN_POINT('Ctrl Pts',(1.1526272271632,-1.,3.9357691705628));
#39747=CARTESIAN_POINT('Ctrl Pts',(1.14767779451123,-1.,3.92982073294257));
#39748=CARTESIAN_POINT('Ctrl Pts',(1.14276220561593,-1.,3.92385513133997));
#39749=CARTESIAN_POINT('Ctrl Pts',(1.13788084225554,-1.,3.91787251936827));
#39750=CARTESIAN_POINT('Ctrl Pts',(1.13303414693896,-1.,3.91187321145649));
#39751=CARTESIAN_POINT('Ctrl Pts',(1.12822258281553,-1.,3.90585753318737));
#39752=CARTESIAN_POINT('Ctrl Pts',(1.12344660099043,-1.,3.89982569750025));
#39753=CARTESIAN_POINT('Ctrl Pts',(1.11870660794603,-1.,3.89377768340344));
#39754=CARTESIAN_POINT('Ctrl Pts',(1.11400292434429,-1.,3.88771308285171));
#39755=CARTESIAN_POINT('Ctrl Pts',(1.10933577224008,-1.,3.88163105531724));
#39756=CARTESIAN_POINT('Ctrl Pts',(1.10470536603287,-1.,3.87553067187514));
#39757=CARTESIAN_POINT('Ctrl Pts',(1.10011198761195,-1.,3.86941120134849));
#39758=CARTESIAN_POINT('Ctrl Pts',(1.09555606505013,-1.,3.86327241021247));
#39759=CARTESIAN_POINT('Ctrl Pts',(1.09103825516294,-1.,3.85711487933931));
#39760=CARTESIAN_POINT('Ctrl Pts',(1.08655950846384,-1.,3.85094025222713));
#39761=CARTESIAN_POINT('Ctrl Pts',(1.08212087917991,-1.,3.8447504803063));
#39762=CARTESIAN_POINT('Ctrl Pts',(1.07772335353858,-1.,3.83854714117491));
#39763=CARTESIAN_POINT('Ctrl Pts',(1.07336766633459,-1.,3.83233071195144));
#39764=CARTESIAN_POINT('Ctrl Pts',(1.06905413180359,-1.,3.82609989967276));
#39765=CARTESIAN_POINT('Ctrl Pts',(1.0647824403893,-1.,3.81985083953012));
#39766=CARTESIAN_POINT('Ctrl Pts',(1.06055206187299,-1.,3.8135786611749));
#39767=CARTESIAN_POINT('Ctrl Pts',(1.05636266918644,-1.,3.80727913637791));
#39768=CARTESIAN_POINT('Ctrl Pts',(1.05221457990016,-1.,3.80095039790681));
#39769=CARTESIAN_POINT('Ctrl Pts',(1.04810913267639,-1.,3.79459440308786));
#39770=CARTESIAN_POINT('Ctrl Pts',(1.04404924374422,-1.,3.78821910787179));
#39771=CARTESIAN_POINT('Ctrl Pts',(1.04003862055798,-1.,3.7818353500817));
#39772=CARTESIAN_POINT('Ctrl Pts',(1.03608074678008,-1.,3.77545283140427));
#39773=CARTESIAN_POINT('Ctrl Pts',(1.03217786604919,-1.,3.76907609832516));
#39774=CARTESIAN_POINT('Ctrl Pts',(1.02833014458184,-1.,3.76270122291245));
#39775=CARTESIAN_POINT('Ctrl Pts',(1.02453429444668,-1.,3.75631037456224));
#39776=CARTESIAN_POINT('Ctrl Pts',(1.02078510487439,-1.,3.74987777155873));
#39777=CARTESIAN_POINT('Ctrl Pts',(1.01707794311088,-1.,3.74337942504993));
#39778=CARTESIAN_POINT('Ctrl Pts',(1.01341114319906,-1.,3.73680245055747));
#39779=CARTESIAN_POINT('Ctrl Pts',(1.00978798539491,-1.,3.73015276704407));
#39780=CARTESIAN_POINT('Ctrl Pts',(1.00622000735696,-1.,3.72346803750544));
#39781=CARTESIAN_POINT('Ctrl Pts',(1.00272423396802,-1.,3.71680667125047));
#39782=CARTESIAN_POINT('Ctrl Pts',(0.999317260756344,-1.,3.7102243971387));
#39783=CARTESIAN_POINT('Ctrl Pts',(0.996009819772431,-1.,3.70375282282107));
#39784=CARTESIAN_POINT('Ctrl Pts',(0.992802218332103,-1.,3.69738123415696));
#39785=CARTESIAN_POINT('Ctrl Pts',(0.989676715398858,-1.,3.69102682138955));
#39786=CARTESIAN_POINT('Ctrl Pts',(0.986602639864285,-1.,3.6845531792623));
#39787=CARTESIAN_POINT('Ctrl Pts',(0.983550791470864,-1.,3.67782408841876));
#39788=CARTESIAN_POINT('Ctrl Pts',(0.980505922458494,-1.,3.67074983340444));
#39789=CARTESIAN_POINT('Ctrl Pts',(0.977478312751416,-1.,3.66333049637403));
#39790=CARTESIAN_POINT('Ctrl Pts',(0.974519971354138,-1.,3.6557157673487));
#39791=CARTESIAN_POINT('Ctrl Pts',(0.971722122060277,-1.,3.64819756447072));
#39792=CARTESIAN_POINT('Ctrl Pts',(0.969195124674828,-1.,3.64113946505393));
#39793=CARTESIAN_POINT('Ctrl Pts',(0.967052554540877,-1.,3.6349212208096));
#39794=CARTESIAN_POINT('Ctrl Pts',(0.965395153165715,-1.,3.62988252139998));
#39795=CARTESIAN_POINT('Ctrl Pts',(0.964373850166081,-1.,3.62652618145252));
#39796=CARTESIAN_POINT('Ctrl Pts',(0.963957782642589,-1.,3.62489305727516));
#39797=CARTESIAN_POINT('Ctrl Pts',(0.963861297423578,-1.,3.62424461507455));
#39798=CARTESIAN_POINT('Ctrl Pts',(0.963880158556713,-1.,3.62404828878374));
#39799=CARTESIAN_POINT('Ctrl Pts',(0.963899035118985,-1.,3.62400312501199));
#39800=CARTESIAN_POINT('',(0.786422660833742,-1.,3.66661143271648));
#39801=CARTESIAN_POINT('Origin',(0.,-1.,0.));
#39802=CARTESIAN_POINT('',(0.732042837400619,-1.,4.13571194405636));
#39803=CARTESIAN_POINT('Ctrl Pts',(0.786422660833742,-1.,3.66661143271648));
#39804=CARTESIAN_POINT('Ctrl Pts',(0.786459983896781,-1.,3.66664310415236));
#39805=CARTESIAN_POINT('Ctrl Pts',(0.786565919559889,-1.,3.66680946938396));
#39806=CARTESIAN_POINT('Ctrl Pts',(0.786774337198499,-1.,3.66743103898844));
#39807=CARTESIAN_POINT('Ctrl Pts',(0.787145041181588,-1.,3.66907505398769));
#39808=CARTESIAN_POINT('Ctrl Pts',(0.787758799995426,-1.,3.672529236635));
#39809=CARTESIAN_POINT('Ctrl Pts',(0.788569566220662,-1.,3.67777119516438));
#39810=CARTESIAN_POINT('Ctrl Pts',(0.789483546065158,-1.,3.68428439784285));
#39811=CARTESIAN_POINT('Ctrl Pts',(0.790436284989579,-1.,3.69172044327754));
#39812=CARTESIAN_POINT('Ctrl Pts',(0.791356575696508,-1.,3.69968940808982));
#39813=CARTESIAN_POINT('Ctrl Pts',(0.792177688845967,-1.,3.70781724021879));
#39814=CARTESIAN_POINT('Ctrl Pts',(0.792848377370115,-1.,3.7158024239604));
#39815=CARTESIAN_POINT('Ctrl Pts',(0.79334702378387,-1.,3.7234879729357));
#39816=CARTESIAN_POINT('Ctrl Pts',(0.793682750269347,-1.,3.7308691469564));
#39817=CARTESIAN_POINT('Ctrl Pts',(0.79388270093679,-1.,3.73803280541576));
#39818=CARTESIAN_POINT('Ctrl Pts',(0.79398270045988,-1.,3.74511357728827));
#39819=CARTESIAN_POINT('Ctrl Pts',(0.79401734737144,-1.,3.75224692493895));
#39820=CARTESIAN_POINT('Ctrl Pts',(0.794008429135046,-1.,3.75951468666325));
#39821=CARTESIAN_POINT('Ctrl Pts',(0.793961083689141,-1.,3.76692626931184));
#39822=CARTESIAN_POINT('Ctrl Pts',(0.793870523787515,-1.,3.77444863801264));
#39823=CARTESIAN_POINT('Ctrl Pts',(0.793726235781339,-1.,3.78202460377617));
#39824=CARTESIAN_POINT('Ctrl Pts',(0.793516871680965,-1.,3.78959439439222));
#39825=CARTESIAN_POINT('Ctrl Pts',(0.7932356129732,-1.,3.79711921389862));
#39826=CARTESIAN_POINT('Ctrl Pts',(0.792882695234692,-1.,3.80459229925598));
#39827=CARTESIAN_POINT('Ctrl Pts',(0.792462483517568,-1.,3.81202588694726));
#39828=CARTESIAN_POINT('Ctrl Pts',(0.791981740718606,-1.,3.81944345442237));
#39829=CARTESIAN_POINT('Ctrl Pts',(0.791447528662381,-1.,3.82687033899799));
#39830=CARTESIAN_POINT('Ctrl Pts',(0.790865012705339,-1.,3.83432392054804));
#39831=CARTESIAN_POINT('Ctrl Pts',(0.790236124191289,-1.,3.84180762342476));
#39832=CARTESIAN_POINT('Ctrl Pts',(0.789560798155618,-1.,3.8493163780891));
#39833=CARTESIAN_POINT('Ctrl Pts',(0.788837734090688,-1.,3.85683995872536));
#39834=CARTESIAN_POINT('Ctrl Pts',(0.78806531509377,-1.,3.86436702561342));
#39835=CARTESIAN_POINT('Ctrl Pts',(0.78724252761798,-1.,3.87188916600905));
#39836=CARTESIAN_POINT('Ctrl Pts',(0.786369675812591,-1.,3.87940402818186));
#39837=CARTESIAN_POINT('Ctrl Pts',(0.785447890340723,-1.,3.88691313167399));
#39838=CARTESIAN_POINT('Ctrl Pts',(0.784478799358335,-1.,3.89442039235105));
#39839=CARTESIAN_POINT('Ctrl Pts',(0.783464141529082,-1.,3.90193039043971));
#39840=CARTESIAN_POINT('Ctrl Pts',(0.782405395622758,-1.,3.90944671004536));
#39841=CARTESIAN_POINT('Ctrl Pts',(0.781303428618343,-1.,3.9169703605466));
#39842=CARTESIAN_POINT('Ctrl Pts',(0.780158678615506,-1.,3.92450058323799));
#39843=CARTESIAN_POINT('Ctrl Pts',(0.778971308134786,-1.,3.93203552473153));
#39844=CARTESIAN_POINT('Ctrl Pts',(0.777741370568549,-1.,3.93957296768098));
#39845=CARTESIAN_POINT('Ctrl Pts',(0.776468966697959,-1.,3.94711101619471));
#39846=CARTESIAN_POINT('Ctrl Pts',(0.775154418039441,-1.,3.95464885452364));
#39847=CARTESIAN_POINT('Ctrl Pts',(0.773798212026682,-1.,3.96218649639876));
#39848=CARTESIAN_POINT('Ctrl Pts',(0.772400931772238,-1.,3.96972446532832));
#39849=CARTESIAN_POINT('Ctrl Pts',(0.770963190030503,-1.,3.97726349165507));
#39850=CARTESIAN_POINT('Ctrl Pts',(0.769485566245459,-1.,3.98480422348403));
#39851=CARTESIAN_POINT('Ctrl Pts',(0.767968531377707,-1.,3.99234687880892));
#39852=CARTESIAN_POINT('Ctrl Pts',(0.766412457135785,-1.,3.99989129179464));
#39853=CARTESIAN_POINT('Ctrl Pts',(0.764817648784946,-1.,4.00743706791366));
#39854=CARTESIAN_POINT('Ctrl Pts',(0.763184371182826,-1.,4.01498370680434));
#39855=CARTESIAN_POINT('Ctrl Pts',(0.761512875859941,-1.,4.02253072741347));
#39856=CARTESIAN_POINT('Ctrl Pts',(0.759803433244165,-1.,4.0300778195465));
#39857=CARTESIAN_POINT('Ctrl Pts',(0.758056338885553,-1.,4.03762485803468));
#39858=CARTESIAN_POINT('Ctrl Pts',(0.756271902370186,-1.,4.04517182654344));
#39859=CARTESIAN_POINT('Ctrl Pts',(0.754450441816411,-1.,4.05271876688106));
#39860=CARTESIAN_POINT('Ctrl Pts',(0.752592276482868,-1.,4.06026572221399));
#39861=CARTESIAN_POINT('Ctrl Pts',(0.750697720483175,-1.,4.06781267241886));
#39862=CARTESIAN_POINT('Ctrl Pts',(0.748767076679176,-1.,4.07535951055363));
#39863=CARTESIAN_POINT('Ctrl Pts',(0.746800631490821,-1.,4.08290608094789));
#39864=CARTESIAN_POINT('Ctrl Pts',(0.744798649705513,-1.,4.09045220253011));
#39865=CARTESIAN_POINT('Ctrl Pts',(0.742761369690017,-1.,4.09799769702712));
#39866=CARTESIAN_POINT('Ctrl Pts',(0.740688998555151,-1.,4.1055424175856));
#39867=CARTESIAN_POINT('Ctrl Pts',(0.738581708229118,-1.,4.11308626953795));
#39868=CARTESIAN_POINT('Ctrl Pts',(0.736439634335347,-1.,4.12062919626082));
#39869=CARTESIAN_POINT('Ctrl Pts',(0.734698226767512,-1.,4.12666277572794));
#39870=CARTESIAN_POINT('Ctrl Pts',(0.733376589325634,-1.,4.13118752796397));
#39871=CARTESIAN_POINT('Ctrl Pts',(0.732488575135925,-1.,4.13420383737278));
#39872=CARTESIAN_POINT('Ctrl Pts',(0.732042837400619,-1.,4.13571194405636));
#39873=CARTESIAN_POINT('',(0.581791163835814,-1.,4.15950947128175));
#39874=CARTESIAN_POINT('',(0.732042837400619,-1.,4.13571194405636));
#39875=CARTESIAN_POINT('',(0.385112848332549,-1.,3.73017266276632));
#39876=CARTESIAN_POINT('Ctrl Pts',(0.581791163835814,-1.,4.15950947128175));
#39877=CARTESIAN_POINT('Ctrl Pts',(0.580901211462913,-1.,4.15821291712391));
#39878=CARTESIAN_POINT('Ctrl Pts',(0.579124568912543,-1.,4.15561864787379));
#39879=CARTESIAN_POINT('Ctrl Pts',(0.576469391673916,-1.,4.1517237611974));
#39880=CARTESIAN_POINT('Ctrl Pts',(0.572948736066276,-1.,4.14652361065787));
#39881=CARTESIAN_POINT('Ctrl Pts',(0.568580610187115,-1.,4.14001179828669));
#39882=CARTESIAN_POINT('Ctrl Pts',(0.564245279535705,-1.,4.13348835726086));
#39883=CARTESIAN_POINT('Ctrl Pts',(0.559942890594628,-1.,4.12695329951859));
#39884=CARTESIAN_POINT('Ctrl Pts',(0.555673636130778,-1.,4.1204066619623));
#39885=CARTESIAN_POINT('Ctrl Pts',(0.551437758498246,-1.,4.11384852025578));
#39886=CARTESIAN_POINT('Ctrl Pts',(0.547235539486759,-1.,4.1072789702877));
#39887=CARTESIAN_POINT('Ctrl Pts',(0.543067286878457,-1.,4.10069810244473));
#39888=CARTESIAN_POINT('Ctrl Pts',(0.53893332117992,-1.,4.09410597627116));
#39889=CARTESIAN_POINT('Ctrl Pts',(0.534833963476999,-1.,4.08750259988693));
#39890=CARTESIAN_POINT('Ctrl Pts',(0.530769518728075,-1.,4.08088789536488));
#39891=CARTESIAN_POINT('Ctrl Pts',(0.526740277226999,-1.,4.07426172299496));
#39892=CARTESIAN_POINT('Ctrl Pts',(0.522746528602767,-1.,4.06762394471075));
#39893=CARTESIAN_POINT('Ctrl Pts',(0.518788572336809,-1.,4.06097448037934));
#39894=CARTESIAN_POINT('Ctrl Pts',(0.514866728193103,-1.,4.05431335771261));
#39895=CARTESIAN_POINT('Ctrl Pts',(0.510981349219173,-1.,4.04764078815591));
#39896=CARTESIAN_POINT('Ctrl Pts',(0.507132823288361,-1.,4.04095715149074));
#39897=CARTESIAN_POINT('Ctrl Pts',(0.503321556915513,-1.,4.0342628417439));
#39898=CARTESIAN_POINT('Ctrl Pts',(0.499547962340889,-1.,4.0275581398015));
#39899=CARTESIAN_POINT('Ctrl Pts',(0.495812444326222,-1.,4.02084308851813));
#39900=CARTESIAN_POINT('Ctrl Pts',(0.49211538341793,-1.,4.01411733503486));
#39901=CARTESIAN_POINT('Ctrl Pts',(0.48845713042453,-1.,4.0073800839092));
#39902=CARTESIAN_POINT('Ctrl Pts',(0.484838042421754,-1.,4.00063045119234));
#39903=CARTESIAN_POINT('Ctrl Pts',(0.481258512209637,-1.,3.99386775880655));
#39904=CARTESIAN_POINT('Ctrl Pts',(0.477718999122033,-1.,3.98709184306743));
#39905=CARTESIAN_POINT('Ctrl Pts',(0.474220061019542,-1.,3.9803033804443));
#39906=CARTESIAN_POINT('Ctrl Pts',(0.470762379613477,-1.,3.97350414289415));
#39907=CARTESIAN_POINT('Ctrl Pts',(0.467346690880671,-1.,3.96669622273946));
#39908=CARTESIAN_POINT('Ctrl Pts',(0.463973722115744,-1.,3.95988133243543));
#39909=CARTESIAN_POINT('Ctrl Pts',(0.460644124429119,-1.,3.95306005817363));
#39910=CARTESIAN_POINT('Ctrl Pts',(0.457358410451673,-1.,3.94623117206675));
#39911=CARTESIAN_POINT('Ctrl Pts',(0.454116879027575,-1.,3.93939080846298));
#39912=CARTESIAN_POINT('Ctrl Pts',(0.450919768356346,-1.,3.93253407403128));
#39913=CARTESIAN_POINT('Ctrl Pts',(0.447767416837296,-1.,3.92565674143424));
#39914=CARTESIAN_POINT('Ctrl Pts',(0.444660430230592,-1.,3.91875701610721));
#39915=CARTESIAN_POINT('Ctrl Pts',(0.441599824524047,-1.,3.91183704069146));
#39916=CARTESIAN_POINT('Ctrl Pts',(0.438587235458233,-1.,3.90490512938546));
#39917=CARTESIAN_POINT('Ctrl Pts',(0.435624629433505,-1.,3.8979725665544));
#39918=CARTESIAN_POINT('Ctrl Pts',(0.432713929544439,-1.,3.89104947940592));
#39919=CARTESIAN_POINT('Ctrl Pts',(0.429856640579733,-1.,3.88414070943334));
#39920=CARTESIAN_POINT('Ctrl Pts',(0.427053541173469,-1.,3.87724240306609));
#39921=CARTESIAN_POINT('Ctrl Pts',(0.424304173195142,-1.,3.87033643487882));
#39922=CARTESIAN_POINT('Ctrl Pts',(0.421607423177575,-1.,3.86339652542749));
#39923=CARTESIAN_POINT('Ctrl Pts',(0.418962468086809,-1.,3.85639825648031));
#39924=CARTESIAN_POINT('Ctrl Pts',(0.41636967805292,-1.,3.8493286415751));
#39925=CARTESIAN_POINT('Ctrl Pts',(0.413831367016726,-1.,3.84219403994742));
#39926=CARTESIAN_POINT('Ctrl Pts',(0.411353038798459,-1.,3.83503345578645));
#39927=CARTESIAN_POINT('Ctrl Pts',(0.408942371447376,-1.,3.82790724256397));
#39928=CARTESIAN_POINT('Ctrl Pts',(0.406607038258906,-1.,3.82087303913741));
#39929=CARTESIAN_POINT('Ctrl Pts',(0.404352694628236,-1.,3.81396374287762));
#39930=CARTESIAN_POINT('Ctrl Pts',(0.402181320148474,-1.,3.80716881962763));
#39931=CARTESIAN_POINT('Ctrl Pts',(0.400088346504726,-1.,3.80040370384659));
#39932=CARTESIAN_POINT('Ctrl Pts',(0.398064818684158,-1.,3.79352887163457));
#39933=CARTESIAN_POINT('Ctrl Pts',(0.396103205335028,-1.,3.78640521279479));
#39934=CARTESIAN_POINT('Ctrl Pts',(0.394202481011595,-1.,3.77894173114368));
#39935=CARTESIAN_POINT('Ctrl Pts',(0.392372786223346,-1.,3.77114011595892));
#39936=CARTESIAN_POINT('Ctrl Pts',(0.390642072979258,-1.,3.76315635032993));
#39937=CARTESIAN_POINT('Ctrl Pts',(0.38905477589825,-1.,3.75529302894757));
#39938=CARTESIAN_POINT('Ctrl Pts',(0.387663020050396,-1.,3.74792651696269));
#39939=CARTESIAN_POINT('Ctrl Pts',(0.386519576222035,-1.,3.74144965781088));
#39940=CARTESIAN_POINT('Ctrl Pts',(0.385670806454744,-1.,3.73621371845475));
#39941=CARTESIAN_POINT('Ctrl Pts',(0.385187124633964,-1.,3.73273893363318));
#39942=CARTESIAN_POINT('Ctrl Pts',(0.385031656499141,-1.,3.73106082862399));
#39943=CARTESIAN_POINT('Ctrl Pts',(0.385037797882046,-1.,3.73040527620929));
#39944=CARTESIAN_POINT('Ctrl Pts',(0.385087139001608,-1.,3.73021431755218));
#39945=CARTESIAN_POINT('Ctrl Pts',(0.385112848332549,-1.,3.73017266276632));
#39946=CARTESIAN_POINT('',(0.203156094897895,-1.,3.74449296982994));
#39947=CARTESIAN_POINT('Origin',(0.,-1.,0.));
#39948=CARTESIAN_POINT('',(0.0760622897878233,-1.,4.19931119685982));
#39949=CARTESIAN_POINT('Ctrl Pts',(0.203156094897895,-1.,3.74449296982994));
#39950=CARTESIAN_POINT('Ctrl Pts',(0.203188003947964,-1.,3.74453008995129));
#39951=CARTESIAN_POINT('Ctrl Pts',(0.203266610111263,-1.,3.74471097893961));
#39952=CARTESIAN_POINT('Ctrl Pts',(0.203375226874331,-1.,3.74535749969262));
#39953=CARTESIAN_POINT('Ctrl Pts',(0.203484186269314,-1.,3.74703926501843));
#39954=CARTESIAN_POINT('Ctrl Pts',(0.203550035479096,-1.,3.75054693397716));
#39955=CARTESIAN_POINT('Ctrl Pts',(0.203530796848403,-1.,3.75585118707924));
#39956=CARTESIAN_POINT('Ctrl Pts',(0.203414634707646,-1.,3.76242717937273));
#39957=CARTESIAN_POINT('Ctrl Pts',(0.203192390045337,-1.,3.76992071595267));
#39958=CARTESIAN_POINT('Ctrl Pts',(0.202854729699196,-1.,3.77793553476879));
#39959=CARTESIAN_POINT('Ctrl Pts',(0.202394260512192,-1.,3.78609175019317));
#39960=CARTESIAN_POINT('Ctrl Pts',(0.201807533800798,-1.,3.79408354187274));
#39961=CARTESIAN_POINT('Ctrl Pts',(0.201097756307251,-1.,3.80175247447171));
#39962=CARTESIAN_POINT('Ctrl Pts',(0.200274679433289,-1.,3.80909529318501));
#39963=CARTESIAN_POINT('Ctrl Pts',(0.199351525297396,-1.,3.81620203429702));
#39964=CARTESIAN_POINT('Ctrl Pts',(0.198342616900469,-1.,3.82321127348981));
#39965=CARTESIAN_POINT('Ctrl Pts',(0.197260935827375,-1.,3.83026221776488));
#39966=CARTESIAN_POINT('Ctrl Pts',(0.196115198971889,-1.,3.83743910616265));
#39967=CARTESIAN_POINT('Ctrl Pts',(0.194909009460254,-1.,3.84475203347052));
#39968=CARTESIAN_POINT('Ctrl Pts',(0.193642806777747,-1.,3.85216762264019));
#39969=CARTESIAN_POINT('Ctrl Pts',(0.192315153044979,-1.,3.85962774407652));
#39970=CARTESIAN_POINT('Ctrl Pts',(0.190924190418612,-1.,3.8670715862477));
#39971=CARTESIAN_POINT('Ctrl Pts',(0.189469253358254,-1.,3.87445976418377));
#39972=CARTESIAN_POINT('Ctrl Pts',(0.187951632512663,-1.,3.88178563496187));
#39973=CARTESIAN_POINT('Ctrl Pts',(0.186373724985263,-1.,3.88906196725817));
#39974=CARTESIAN_POINT('Ctrl Pts',(0.184738537728034,-1.,3.89631300742633));
#39975=CARTESIAN_POINT('Ctrl Pts',(0.183049081993193,-1.,3.90356488555138));
#39976=CARTESIAN_POINT('Ctrl Pts',(0.181307740731795,-1.,3.91083557557193));
#39977=CARTESIAN_POINT('Ctrl Pts',(0.179515885822894,-1.,3.91812876180948));
#39978=CARTESIAN_POINT('Ctrl Pts',(0.177674246152328,-1.,3.92543942697672));
#39979=CARTESIAN_POINT('Ctrl Pts',(0.175783136893872,-1.,3.93275726771049));
#39980=CARTESIAN_POINT('Ctrl Pts',(0.173842734974607,-1.,3.94007083096214));
#39981=CARTESIAN_POINT('Ctrl Pts',(0.171853355369232,-1.,3.94737164900861));
#39982=CARTESIAN_POINT('Ctrl Pts',(0.16981566637413,-1.,3.95465744665263));
#39983=CARTESIAN_POINT('Ctrl Pts',(0.167730547023312,-1.,3.96192990160296));
#39984=CARTESIAN_POINT('Ctrl Pts',(0.165598992851097,-1.,3.9691931362141));
#39985=CARTESIAN_POINT('Ctrl Pts',(0.163422004609998,-1.,3.97645194630944));
#39986=CARTESIAN_POINT('Ctrl Pts',(0.161200482186087,-1.,3.98371010319866));
#39987=CARTESIAN_POINT('Ctrl Pts',(0.158935123982796,-1.,3.99096873945862));
#39988=CARTESIAN_POINT('Ctrl Pts',(0.156626481393735,-1.,3.99822717425869));
#39989=CARTESIAN_POINT('Ctrl Pts',(0.154275004872309,-1.,4.00548360245297));
#39990=CARTESIAN_POINT('Ctrl Pts',(0.151881094022909,-1.,4.01273584234684));
#39991=CARTESIAN_POINT('Ctrl Pts',(0.149445144968707,-1.,4.01998203715588));
#39992=CARTESIAN_POINT('Ctrl Pts',(0.146967602878998,-1.,4.02722143147048));
#39993=CARTESIAN_POINT('Ctrl Pts',(0.144448947038352,-1.,4.03445411510403));
#39994=CARTESIAN_POINT('Ctrl Pts',(0.141889671485507,-1.,4.04168069633842));
#39995=CARTESIAN_POINT('Ctrl Pts',(0.139290267180059,-1.,4.04890199238056));
#39996=CARTESIAN_POINT('Ctrl Pts',(0.136651205046111,-1.,4.05611873400122));
#39997=CARTESIAN_POINT('Ctrl Pts',(0.133972916144225,-1.,4.06333121018476));
#39998=CARTESIAN_POINT('Ctrl Pts',(0.131255793548914,-1.,4.07053931528579));
#39999=CARTESIAN_POINT('Ctrl Pts',(0.128500200484813,-1.,4.07774270738809));
#40000=CARTESIAN_POINT('Ctrl Pts',(0.125706476822529,-1.,4.08494093372315));
#40001=CARTESIAN_POINT('Ctrl Pts',(0.122874946249119,-1.,4.09213355850836));
#40002=CARTESIAN_POINT('Ctrl Pts',(0.120005924388162,-1.,4.09932031767243));
#40003=CARTESIAN_POINT('Ctrl Pts',(0.117099722731704,-1.,4.10650113382187));
#40004=CARTESIAN_POINT('Ctrl Pts',(0.114156649609601,-1.,4.11367603925313));
#40005=CARTESIAN_POINT('Ctrl Pts',(0.111177012683377,-1.,4.12084512502444));
#40006=CARTESIAN_POINT('Ctrl Pts',(0.10816112052835,-1.,4.12800848371386));
#40007=CARTESIAN_POINT('Ctrl Pts',(0.105109286538864,-1.,4.13516614458396));
#40008=CARTESIAN_POINT('Ctrl Pts',(0.102021826577453,-1.,4.14231804938737));
#40009=CARTESIAN_POINT('Ctrl Pts',(0.0988990478899809,-1.,4.1494640891762));
#40010=CARTESIAN_POINT('Ctrl Pts',(0.0957412403297065,-1.,4.15660412653006));
#40011=CARTESIAN_POINT('Ctrl Pts',(0.0925486672167687,-1.,4.16373802265942));
#40012=CARTESIAN_POINT('Ctrl Pts',(0.0893215560850325,-1.,4.17086566491823));
#40013=CARTESIAN_POINT('Ctrl Pts',(0.0860600915552512,-1.,4.17798698669991));
#40014=CARTESIAN_POINT('Ctrl Pts',(0.0827644164389507,-1.,4.1851019532944));
#40015=CARTESIAN_POINT('Ctrl Pts',(0.08010058871176,-1.,4.19078883322483));
#40016=CARTESIAN_POINT('Ctrl Pts',(0.0780873956244399,-1.,4.19505112860624));
#40017=CARTESIAN_POINT('Ctrl Pts',(0.0767384596142192,-1.,4.19789138621624));
#40018=CARTESIAN_POINT('Ctrl Pts',(0.0760622897878233,-1.,4.19931119685982));
#40019=CARTESIAN_POINT('',(-0.0760622897878249,-1.,4.19931119685982));
#40020=CARTESIAN_POINT('',(0.0760622897878233,-1.,4.19931119685982));
#40021=CARTESIAN_POINT('',(-0.203156094896101,-1.,3.74449296983004));
#40022=CARTESIAN_POINT('Ctrl Pts',(-0.0760622897878249,-1.,4.19931119685982));
#40023=CARTESIAN_POINT('Ctrl Pts',(-0.0767384596141467,-1.,4.1978913862118));
#40024=CARTESIAN_POINT('Ctrl Pts',(-0.07808739562424,-1.,4.19505112859416));
#40025=CARTESIAN_POINT('Ctrl Pts',(-0.0801005887114322,-1.,4.19078883320504));
#40026=CARTESIAN_POINT('Ctrl Pts',(-0.0827644164385681,-1.,4.18510195327123));
#40027=CARTESIAN_POINT('Ctrl Pts',(-0.0860600915549399,-1.,4.17798698668094));
#40028=CARTESIAN_POINT('Ctrl Pts',(-0.0893215560848652,-1.,4.17086566490794));
#40029=CARTESIAN_POINT('Ctrl Pts',(-0.0925486672167534,-1.,4.16373802265839));
#40030=CARTESIAN_POINT('Ctrl Pts',(-0.0957412403298009,-1.,4.15660412653577));
#40031=CARTESIAN_POINT('Ctrl Pts',(-0.0988990478901228,-1.,4.14946408918485));
#40032=CARTESIAN_POINT('Ctrl Pts',(-0.102021826577584,-1.,4.14231804939538));
#40033=CARTESIAN_POINT('Ctrl Pts',(-0.105109286538945,-1.,4.13516614458895));
#40034=CARTESIAN_POINT('Ctrl Pts',(-0.10816112052837,-1.,4.12800848371504));
#40035=CARTESIAN_POINT('Ctrl Pts',(-0.111177012683347,-1.,4.1208451250225));
#40036=CARTESIAN_POINT('Ctrl Pts',(-0.114156649609546,-1.,4.11367603924961));
#40037=CARTESIAN_POINT('Ctrl Pts',(-0.117099722731648,-1.,4.10650113381833));
#40038=CARTESIAN_POINT('Ctrl Pts',(-0.120005924388124,-1.,4.09932031767002));
#40039=CARTESIAN_POINT('Ctrl Pts',(-0.122874946249107,-1.,4.09213355850756));
#40040=CARTESIAN_POINT('Ctrl Pts',(-0.12570647682254,-1.,4.08494093372377));
#40041=CARTESIAN_POINT('Ctrl Pts',(-0.128500200484838,-1.,4.07774270738954));
#40042=CARTESIAN_POINT('Ctrl Pts',(-0.131255793548941,-1.,4.0705393152874));
#40043=CARTESIAN_POINT('Ctrl Pts',(-0.133972916144245,-1.,4.06333121018596));
#40044=CARTESIAN_POINT('Ctrl Pts',(-0.136651205046119,-1.,4.05611873400172));
#40045=CARTESIAN_POINT('Ctrl Pts',(-0.139290267180057,-1.,4.04890199238036));
#40046=CARTESIAN_POINT('Ctrl Pts',(-0.1418896714855,-1.,4.04168069633781));
#40047=CARTESIAN_POINT('Ctrl Pts',(-0.144448947038345,-1.,4.03445411510333));
#40048=CARTESIAN_POINT('Ctrl Pts',(-0.146967602878994,-1.,4.02722143146994));
#40049=CARTESIAN_POINT('Ctrl Pts',(-0.149445144968707,-1.,4.01998203715564));
#40050=CARTESIAN_POINT('Ctrl Pts',(-0.151881094022911,-1.,4.01273584234689));
#40051=CARTESIAN_POINT('Ctrl Pts',(-0.154275004872311,-1.,4.00548360245319));
#40052=CARTESIAN_POINT('Ctrl Pts',(-0.156626481393734,-1.,3.99822717425893));
#40053=CARTESIAN_POINT('Ctrl Pts',(-0.158935123982793,-1.,3.99096873945878));
#40054=CARTESIAN_POINT('Ctrl Pts',(-0.161200482186085,-1.,3.98371010319872));
#40055=CARTESIAN_POINT('Ctrl Pts',(-0.163422004609999,-1.,3.97645194630943));
#40056=CARTESIAN_POINT('Ctrl Pts',(-0.165598992851102,-1.,3.96919313621407));
#40057=CARTESIAN_POINT('Ctrl Pts',(-0.16773054702332,-1.,3.96192990160296));
#40058=CARTESIAN_POINT('Ctrl Pts',(-0.169815666374139,-1.,3.95465744665268));
#40059=CARTESIAN_POINT('Ctrl Pts',(-0.17185335536924,-1.,3.94737164900868));
#40060=CARTESIAN_POINT('Ctrl Pts',(-0.17384273497461,-1.,3.94007083096217));
#40061=CARTESIAN_POINT('Ctrl Pts',(-0.175783136893868,-1.,3.93275726771042));
#40062=CARTESIAN_POINT('Ctrl Pts',(-0.177674246152318,-1.,3.92543942697655));
#40063=CARTESIAN_POINT('Ctrl Pts',(-0.179515885822882,-1.,3.91812876180926));
#40064=CARTESIAN_POINT('Ctrl Pts',(-0.181307740731786,-1.,3.91083557557175));
#40065=CARTESIAN_POINT('Ctrl Pts',(-0.183049081993191,-1.,3.90356488555132));
#40066=CARTESIAN_POINT('Ctrl Pts',(-0.184738537728043,-1.,3.89631300742646));
#40067=CARTESIAN_POINT('Ctrl Pts',(-0.186373724985281,-1.,3.88906196725848));
#40068=CARTESIAN_POINT('Ctrl Pts',(-0.187951632512685,-1.,3.88178563496228));
#40069=CARTESIAN_POINT('Ctrl Pts',(-0.189469253358273,-1.,3.87445976418412));
#40070=CARTESIAN_POINT('Ctrl Pts',(-0.19092419041862,-1.,3.86707158624783));
#40071=CARTESIAN_POINT('Ctrl Pts',(-0.192315153044971,-1.,3.85962774407633));
#40072=CARTESIAN_POINT('Ctrl Pts',(-0.193642806777723,-1.,3.85216762263966));
#40073=CARTESIAN_POINT('Ctrl Pts',(-0.194909009460221,-1.,3.84475203346977));
#40074=CARTESIAN_POINT('Ctrl Pts',(-0.196115198971859,-1.,3.83743910616195));
#40075=CARTESIAN_POINT('Ctrl Pts',(-0.197260935827362,-1.,3.83026221776456));
#40076=CARTESIAN_POINT('Ctrl Pts',(-0.198342616900487,-1.,3.82321127349016));
#40077=CARTESIAN_POINT('Ctrl Pts',(-0.199351525297447,-1.,3.81620203429815));
#40078=CARTESIAN_POINT('Ctrl Pts',(-0.200274679433365,-1.,3.80909529318669));
#40079=CARTESIAN_POINT('Ctrl Pts',(-0.201097756307326,-1.,3.80175247447337));
#40080=CARTESIAN_POINT('Ctrl Pts',(-0.201807533800837,-1.,3.7940835418736));
#40081=CARTESIAN_POINT('Ctrl Pts',(-0.20239426051216,-1.,3.78609175019242));
#40082=CARTESIAN_POINT('Ctrl Pts',(-0.202854729699081,-1.,3.77793553476614));
#40083=CARTESIAN_POINT('Ctrl Pts',(-0.203192390045165,-1.,3.7699207159487));
#40084=CARTESIAN_POINT('Ctrl Pts',(-0.203414634707479,-1.,3.76242717936885));
#40085=CARTESIAN_POINT('Ctrl Pts',(-0.203530796848322,-1.,3.75585118707734));
#40086=CARTESIAN_POINT('Ctrl Pts',(-0.203550035479166,-1.,3.75054693397875));
#40087=CARTESIAN_POINT('Ctrl Pts',(-0.203484186269415,-1.,3.74703926501752));
#40088=CARTESIAN_POINT('Ctrl Pts',(-0.203375226874122,-1.,3.74535749969115));
#40089=CARTESIAN_POINT('Ctrl Pts',(-0.203266610110531,-1.,3.74471097893845));
#40090=CARTESIAN_POINT('Ctrl Pts',(-0.203188003946657,-1.,3.74453008995092));
#40091=CARTESIAN_POINT('Ctrl Pts',(-0.203156094896101,-1.,3.74449296983004));
#40092=CARTESIAN_POINT('',(-0.385112848330762,-1.,3.73017266276651));
#40093=CARTESIAN_POINT('Origin',(0.,-1.,0.));
#40094=CARTESIAN_POINT('',(-0.581791163835815,-1.,4.15950947128175));
#40095=CARTESIAN_POINT('Ctrl Pts',(-0.385112848330762,-1.,3.73017266276651));
#40096=CARTESIAN_POINT('Ctrl Pts',(-0.385087139000375,-1.,3.73021431755274));
#40097=CARTESIAN_POINT('Ctrl Pts',(-0.385037797881504,-1.,3.73040527621055));
#40098=CARTESIAN_POINT('Ctrl Pts',(-0.385031656499164,-1.,3.73106082862548));
#40099=CARTESIAN_POINT('Ctrl Pts',(-0.385187124634206,-1.,3.73273893363406));
#40100=CARTESIAN_POINT('Ctrl Pts',(-0.385670806454566,-1.,3.73621371845318));
#40101=CARTESIAN_POINT('Ctrl Pts',(-0.386519576222251,-1.,3.74144965781276));
#40102=CARTESIAN_POINT('Ctrl Pts',(-0.387663020050836,-1.,3.74792651696654));
#40103=CARTESIAN_POINT('Ctrl Pts',(-0.389054775898702,-1.,3.75529302895152));
#40104=CARTESIAN_POINT('Ctrl Pts',(-0.39064207297956,-1.,3.76315635033257));
#40105=CARTESIAN_POINT('Ctrl Pts',(-0.392372786223433,-1.,3.77114011595967));
#40106=CARTESIAN_POINT('Ctrl Pts',(-0.394202481011499,-1.,3.77894173114283));
#40107=CARTESIAN_POINT('Ctrl Pts',(-0.396103205334841,-1.,3.78640521279313));
#40108=CARTESIAN_POINT('Ctrl Pts',(-0.39806481868397,-1.,3.7935288716329));
#40109=CARTESIAN_POINT('Ctrl Pts',(-0.4000883465046,-1.,3.80040370384546));
#40110=CARTESIAN_POINT('Ctrl Pts',(-0.402181320148436,-1.,3.80716881962728));
#40111=CARTESIAN_POINT('Ctrl Pts',(-0.404352694628273,-1.,3.81396374287793));
#40112=CARTESIAN_POINT('Ctrl Pts',(-0.406607038258985,-1.,3.8208730391381));
#40113=CARTESIAN_POINT('Ctrl Pts',(-0.40894237144746,-1.,3.82790724256471));
#40114=CARTESIAN_POINT('Ctrl Pts',(-0.411353038798519,-1.,3.83503345578698));
#40115=CARTESIAN_POINT('Ctrl Pts',(-0.413831367016748,-1.,3.84219403994762));
#40116=CARTESIAN_POINT('Ctrl Pts',(-0.416369678052907,-1.,3.84932864157497));
#40117=CARTESIAN_POINT('Ctrl Pts',(-0.418962468086773,-1.,3.85639825647996));
#40118=CARTESIAN_POINT('Ctrl Pts',(-0.421607423177534,-1.,3.86339652542709));
#40119=CARTESIAN_POINT('Ctrl Pts',(-0.424304173195111,-1.,3.87033643487851));
#40120=CARTESIAN_POINT('Ctrl Pts',(-0.427053541173457,-1.,3.87724240306597));
#40121=CARTESIAN_POINT('Ctrl Pts',(-0.429856640579741,-1.,3.88414070943341));
#40122=CARTESIAN_POINT('Ctrl Pts',(-0.432713929544458,-1.,3.89104947940611));
#40123=CARTESIAN_POINT('Ctrl Pts',(-0.435624629433528,-1.,3.89797256655462));
#40124=CARTESIAN_POINT('Ctrl Pts',(-0.43858723545825,-1.,3.90490512938563));
#40125=CARTESIAN_POINT('Ctrl Pts',(-0.441599824524054,-1.,3.91183704069153));
#40126=CARTESIAN_POINT('Ctrl Pts',(-0.444660430230591,-1.,3.91875701610719));
#40127=CARTESIAN_POINT('Ctrl Pts',(-0.447767416837293,-1.,3.92565674143416));
#40128=CARTESIAN_POINT('Ctrl Pts',(-0.450919768356348,-1.,3.93253407403123));
#40129=CARTESIAN_POINT('Ctrl Pts',(-0.454116879027584,-1.,3.93939080846298));
#40130=CARTESIAN_POINT('Ctrl Pts',(-0.457358410451683,-1.,3.94623117206678));
#40131=CARTESIAN_POINT('Ctrl Pts',(-0.460644124429121,-1.,3.95306005817364));
#40132=CARTESIAN_POINT('Ctrl Pts',(-0.463973722115733,-1.,3.95988133243538));
#40133=CARTESIAN_POINT('Ctrl Pts',(-0.467346690880643,-1.,3.9666962227393));
#40134=CARTESIAN_POINT('Ctrl Pts',(-0.470762379613439,-1.,3.97350414289392));
#40135=CARTESIAN_POINT('Ctrl Pts',(-0.47422006101951,-1.,3.98030338044409));
#40136=CARTESIAN_POINT('Ctrl Pts',(-0.477718999122027,-1.,3.98709184306738));
#40137=CARTESIAN_POINT('Ctrl Pts',(-0.481258512209675,-1.,3.99386775880679));
#40138=CARTESIAN_POINT('Ctrl Pts',(-0.484838042421835,-1.,4.00063045119288));
#40139=CARTESIAN_POINT('Ctrl Pts',(-0.488457130424633,-1.,4.0073800839099));
#40140=CARTESIAN_POINT('Ctrl Pts',(-0.492115383418018,-1.,4.01411733503546));
#40141=CARTESIAN_POINT('Ctrl Pts',(-0.495812444326251,-1.,4.02084308851832));
#40142=CARTESIAN_POINT('Ctrl Pts',(-0.499547962340821,-1.,4.02755813980101));
#40143=CARTESIAN_POINT('Ctrl Pts',(-0.503321556915346,-1.,4.03426284174272));
#40144=CARTESIAN_POINT('Ctrl Pts',(-0.507132823288136,-1.,4.04095715148915));
#40145=CARTESIAN_POINT('Ctrl Pts',(-0.51098134921897,-1.,4.04764078815447));
#40146=CARTESIAN_POINT('Ctrl Pts',(-0.514866728193017,-1.,4.05431335771199));
#40147=CARTESIAN_POINT('Ctrl Pts',(-0.518788572336924,-1.,4.06097448038013));
#40148=CARTESIAN_POINT('Ctrl Pts',(-0.522746528603107,-1.,4.06762394471314));
#40149=CARTESIAN_POINT('Ctrl Pts',(-0.526740277227498,-1.,4.07426172299847));
#40150=CARTESIAN_POINT('Ctrl Pts',(-0.530769518728571,-1.,4.08088789536836));
#40151=CARTESIAN_POINT('Ctrl Pts',(-0.534833963477273,-1.,4.08750259988885));
#40152=CARTESIAN_POINT('Ctrl Pts',(-0.538933321179756,-1.,4.09410597627));
#40153=CARTESIAN_POINT('Ctrl Pts',(-0.543067286877757,-1.,4.10069810243979));
#40154=CARTESIAN_POINT('Ctrl Pts',(-0.547235539485637,-1.,4.10727897027977));
#40155=CARTESIAN_POINT('Ctrl Pts',(-0.551437758497033,-1.,4.11384852024721));
#40156=CARTESIAN_POINT('Ctrl Pts',(-0.555673636129977,-1.,4.12040666195664));
#40157=CARTESIAN_POINT('Ctrl Pts',(-0.559942890594774,-1.,4.12695329951961));
#40158=CARTESIAN_POINT('Ctrl Pts',(-0.564245279537149,-1.,4.13348835727104));
#40159=CARTESIAN_POINT('Ctrl Pts',(-0.568580610189775,-1.,4.14001179830547));
#40160=CARTESIAN_POINT('Ctrl Pts',(-0.572948736069522,-1.,4.14652361068081));
#40161=CARTESIAN_POINT('Ctrl Pts',(-0.576469391676688,-1.,4.151723761217));
#40162=CARTESIAN_POINT('Ctrl Pts',(-0.579124568914235,-1.,4.15561864788576));
#40163=CARTESIAN_POINT('Ctrl Pts',(-0.580901211463535,-1.,4.1582129171283));
#40164=CARTESIAN_POINT('Ctrl Pts',(-0.581791163835815,-1.,4.15950947128175));
#40165=CARTESIAN_POINT('',(-0.73204283740062,-1.,4.13571194405636));
#40166=CARTESIAN_POINT('',(-0.581791163835815,-1.,4.15950947128175));
#40167=CARTESIAN_POINT('',(-0.786422660831985,-1.,3.66661143271685));
#40168=CARTESIAN_POINT('Ctrl Pts',(-0.73204283740062,-1.,4.13571194405636));
#40169=CARTESIAN_POINT('Ctrl Pts',(-0.73248857513516,-1.,4.1342038373684));
#40170=CARTESIAN_POINT('Ctrl Pts',(-0.733376589323546,-1.,4.13118752795207));
#40171=CARTESIAN_POINT('Ctrl Pts',(-0.734698226764092,-1.,4.12666277570844));
#40172=CARTESIAN_POINT('Ctrl Pts',(-0.736439634331345,-1.,4.120629196238));
#40173=CARTESIAN_POINT('Ctrl Pts',(-0.738581708225844,-1.,4.11308626951927));
#40174=CARTESIAN_POINT('Ctrl Pts',(-0.740688998553377,-1.,4.10554241757547));
#40175=CARTESIAN_POINT('Ctrl Pts',(-0.742761369689841,-1.,4.09799769702611));
#40176=CARTESIAN_POINT('Ctrl Pts',(-0.7447986497065,-1.,4.09045220253573));
#40177=CARTESIAN_POINT('Ctrl Pts',(-0.746800631492315,-1.,4.08290608095642));
#40178=CARTESIAN_POINT('Ctrl Pts',(-0.748767076680557,-1.,4.07535951056152));
#40179=CARTESIAN_POINT('Ctrl Pts',(-0.750697720484036,-1.,4.06781267242378));
#40180=CARTESIAN_POINT('Ctrl Pts',(-0.752592276483072,-1.,4.06026572221515));
#40181=CARTESIAN_POINT('Ctrl Pts',(-0.754450441816078,-1.,4.05271876687915));
#40182=CARTESIAN_POINT('Ctrl Pts',(-0.756271902369581,-1.,4.04517182653997));
#40183=CARTESIAN_POINT('Ctrl Pts',(-0.758056338884944,-1.,4.03762485803119));
#40184=CARTESIAN_POINT('Ctrl Pts',(-0.759803433243752,-1.,4.03007781954412));
#40185=CARTESIAN_POINT('Ctrl Pts',(-0.761512875859804,-1.,4.02253072741268));
#40186=CARTESIAN_POINT('Ctrl Pts',(-0.763184371182935,-1.,4.01498370680496));
#40187=CARTESIAN_POINT('Ctrl Pts',(-0.764817648785198,-1.,4.00743706791509));
#40188=CARTESIAN_POINT('Ctrl Pts',(-0.766412457136064,-1.,3.99989129179622));
#40189=CARTESIAN_POINT('Ctrl Pts',(-0.767968531377915,-1.,3.9923468788101));
#40190=CARTESIAN_POINT('Ctrl Pts',(-0.769485566245544,-1.,3.98480422348451));
#40191=CARTESIAN_POINT('Ctrl Pts',(-0.770963190030471,-1.,3.97726349165488));
#40192=CARTESIAN_POINT('Ctrl Pts',(-0.772400931772136,-1.,3.96972446532772));
#40193=CARTESIAN_POINT('Ctrl Pts',(-0.773798212026566,-1.,3.96218649639807));
#40194=CARTESIAN_POINT('Ctrl Pts',(-0.775154418039352,-1.,3.9546488545231));
#40195=CARTESIAN_POINT('Ctrl Pts',(-0.776468966697921,-1.,3.94711101619447));
#40196=CARTESIAN_POINT('Ctrl Pts',(-0.777741370568559,-1.,3.93957296768103));
#40197=CARTESIAN_POINT('Ctrl Pts',(-0.778971308134821,-1.,3.93203552473174));
#40198=CARTESIAN_POINT('Ctrl Pts',(-0.780158678615543,-1.,3.92450058323823));
#40199=CARTESIAN_POINT('Ctrl Pts',(-0.781303428618367,-1.,3.91697036054676));
#40200=CARTESIAN_POINT('Ctrl Pts',(-0.782405395622764,-1.,3.90944671004542));
#40201=CARTESIAN_POINT('Ctrl Pts',(-0.783464141529081,-1.,3.9019303904397));
#40202=CARTESIAN_POINT('Ctrl Pts',(-0.784478799358336,-1.,3.89442039235103));
#40203=CARTESIAN_POINT('Ctrl Pts',(-0.78544789034073,-1.,3.88691313167398));
#40204=CARTESIAN_POINT('Ctrl Pts',(-0.786369675812609,-1.,3.8794040281819));
#40205=CARTESIAN_POINT('Ctrl Pts',(-0.787242527617999,-1.,3.87188916600912));
#40206=CARTESIAN_POINT('Ctrl Pts',(-0.788065315093778,-1.,3.86436702561345));
#40207=CARTESIAN_POINT('Ctrl Pts',(-0.788837734090672,-1.,3.85683995872529));
#40208=CARTESIAN_POINT('Ctrl Pts',(-0.789560798155582,-1.,3.84931637808894));
#40209=CARTESIAN_POINT('Ctrl Pts',(-0.790236124191242,-1.,3.84180762342454));
#40210=CARTESIAN_POINT('Ctrl Pts',(-0.790865012705301,-1.,3.83432392054786));
#40211=CARTESIAN_POINT('Ctrl Pts',(-0.791447528662369,-1.,3.82687033899792));
#40212=CARTESIAN_POINT('Ctrl Pts',(-0.791981740718635,-1.,3.81944345442249));
#40213=CARTESIAN_POINT('Ctrl Pts',(-0.792462483517634,-1.,3.81202588694756));
#40214=CARTESIAN_POINT('Ctrl Pts',(-0.792882695234778,-1.,3.80459229925637));
#40215=CARTESIAN_POINT('Ctrl Pts',(-0.793235612973273,-1.,3.79711921389897));
#40216=CARTESIAN_POINT('Ctrl Pts',(-0.793516871680993,-1.,3.78959439439235));
#40217=CARTESIAN_POINT('Ctrl Pts',(-0.7937262357813,-1.,3.78202460377598));
#40218=CARTESIAN_POINT('Ctrl Pts',(-0.793870523787408,-1.,3.77444863801212));
#40219=CARTESIAN_POINT('Ctrl Pts',(-0.793961083688992,-1.,3.76692626931111));
#40220=CARTESIAN_POINT('Ctrl Pts',(-0.794008429134907,-1.,3.75951468666257));
#40221=CARTESIAN_POINT('Ctrl Pts',(-0.794017347371377,-1.,3.75224692493864));
#40222=CARTESIAN_POINT('Ctrl Pts',(-0.793982700459952,-1.,3.74511357728861));
#40223=CARTESIAN_POINT('Ctrl Pts',(-0.793882700937017,-1.,3.73803280541687));
#40224=CARTESIAN_POINT('Ctrl Pts',(-0.793682750269684,-1.,3.73086914695805));
#40225=CARTESIAN_POINT('Ctrl Pts',(-0.793347023784205,-1.,3.72348797293734));
#40226=CARTESIAN_POINT('Ctrl Pts',(-0.792848377370287,-1.,3.71580242396124));
#40227=CARTESIAN_POINT('Ctrl Pts',(-0.792177688845818,-1.,3.70781724021806));
#40228=CARTESIAN_POINT('Ctrl Pts',(-0.79135657569598,-1.,3.69968940808721));
#40229=CARTESIAN_POINT('Ctrl Pts',(-0.790436284988788,-1.,3.69172044327364));
#40230=CARTESIAN_POINT('Ctrl Pts',(-0.789483546064387,-1.,3.68428439783905));
#40231=CARTESIAN_POINT('Ctrl Pts',(-0.788569566220285,-1.,3.67777119516252));
#40232=CARTESIAN_POINT('Ctrl Pts',(-0.787758799995743,-1.,3.67252923663655));
#40233=CARTESIAN_POINT('Ctrl Pts',(-0.787145041181546,-1.,3.66907505398677));
#40234=CARTESIAN_POINT('Ctrl Pts',(-0.786774337198062,-1.,3.66743103898702));
#40235=CARTESIAN_POINT('Ctrl Pts',(-0.786565919558984,-1.,3.66680946938292));
#40236=CARTESIAN_POINT('Ctrl Pts',(-0.786459983895432,-1.,3.6666431041522));
#40237=CARTESIAN_POINT('Ctrl Pts',(-0.786422660831985,-1.,3.66661143271685));
#40238=CARTESIAN_POINT('',(-0.963899035117249,-1.,3.62400312501245));
#40239=CARTESIAN_POINT('Origin',(0.,-1.,0.));
#40240=CARTESIAN_POINT('',(-1.22531898815164,-1.,4.01728681790024));
#40241=CARTESIAN_POINT('Ctrl Pts',(-0.963899035117249,-1.,3.62400312501245));
#40242=CARTESIAN_POINT('Ctrl Pts',(-0.963880158555582,-1.,3.6240482887845));
#40243=CARTESIAN_POINT('Ctrl Pts',(-0.963861297423241,-1.,3.62424461507588));
#40244=CARTESIAN_POINT('Ctrl Pts',(-0.963957782642843,-1.,3.62489305727662));
#40245=CARTESIAN_POINT('Ctrl Pts',(-0.964373850166458,-1.,3.62652618145335));
#40246=CARTESIAN_POINT('Ctrl Pts',(-0.965395153165293,-1.,3.62988252139846));
#40247=CARTESIAN_POINT('Ctrl Pts',(-0.967052554541386,-1.,3.63492122081143));
#40248=CARTESIAN_POINT('Ctrl Pts',(-0.969195124675866,-1.,3.64113946505766));
#40249=CARTESIAN_POINT('Ctrl Pts',(-0.971722122061341,-1.,3.64819756447455));
#40250=CARTESIAN_POINT('Ctrl Pts',(-0.974519971354848,-1.,3.65571576735126));
#40251=CARTESIAN_POINT('Ctrl Pts',(-0.977478312751618,-1.,3.66333049637475));
#40252=CARTESIAN_POINT('Ctrl Pts',(-0.980505922458267,-1.,3.67074983340361));
#40253=CARTESIAN_POINT('Ctrl Pts',(-0.983550791470419,-1.,3.67782408841715));
#40254=CARTESIAN_POINT('Ctrl Pts',(-0.986602639863838,-1.,3.68455317926068));
#40255=CARTESIAN_POINT('Ctrl Pts',(-0.989676715398558,-1.,3.69102682138846));
#40256=CARTESIAN_POINT('Ctrl Pts',(-0.99280221833201,-1.,3.69738123415662));
#40257=CARTESIAN_POINT('Ctrl Pts',(-0.996009819772518,-1.,3.70375282282138));
#40258=CARTESIAN_POINT('Ctrl Pts',(-0.999317260756531,-1.,3.71022439713938));
#40259=CARTESIAN_POINT('Ctrl Pts',(-1.00272423396822,-1.,3.71680667125118));
#40260=CARTESIAN_POINT('Ctrl Pts',(-1.0062200073571,-1.,3.72346803750595));
#40261=CARTESIAN_POINT('Ctrl Pts',(-1.00978798539496,-1.,3.73015276704426));
#40262=CARTESIAN_POINT('Ctrl Pts',(-1.01341114319903,-1.,3.73680245055734));
#40263=CARTESIAN_POINT('Ctrl Pts',(-1.01707794311079,-1.,3.74337942504959));
#40264=CARTESIAN_POINT('Ctrl Pts',(-1.02078510487428,-1.,3.74987777155834));
#40265=CARTESIAN_POINT('Ctrl Pts',(-1.0245342944466,-1.,3.75631037456194));
#40266=CARTESIAN_POINT('Ctrl Pts',(-1.02833014458181,-1.,3.76270122291232));
#40267=CARTESIAN_POINT('Ctrl Pts',(-1.0321778660492,-1.,3.76907609832522));
#40268=CARTESIAN_POINT('Ctrl Pts',(-1.03608074678013,-1.,3.77545283140445));
#40269=CARTESIAN_POINT('Ctrl Pts',(-1.04003862055804,-1.,3.78183535008192));
#40270=CARTESIAN_POINT('Ctrl Pts',(-1.04404924374426,-1.,3.78821910787195));
#40271=CARTESIAN_POINT('Ctrl Pts',(-1.04810913267641,-1.,3.79459440308793));
#40272=CARTESIAN_POINT('Ctrl Pts',(-1.05221457990015,-1.,3.80095039790678));
#40273=CARTESIAN_POINT('Ctrl Pts',(-1.05636266918643,-1.,3.80727913637784));
#40274=CARTESIAN_POINT('Ctrl Pts',(-1.06055206187298,-1.,3.81357866117485));
#40275=CARTESIAN_POINT('Ctrl Pts',(-1.06478244038931,-1.,3.81985083953012));
#40276=CARTESIAN_POINT('Ctrl Pts',(-1.0690541318036,-1.,3.82609989967278));
#40277=CARTESIAN_POINT('Ctrl Pts',(-1.0733676663346,-1.,3.83233071195145));
#40278=CARTESIAN_POINT('Ctrl Pts',(-1.07772335353856,-1.,3.83854714117486));
#40279=CARTESIAN_POINT('Ctrl Pts',(-1.08212087917986,-1.,3.84475048030615));
#40280=CARTESIAN_POINT('Ctrl Pts',(-1.08655950846377,-1.,3.8509402522269));
#40281=CARTESIAN_POINT('Ctrl Pts',(-1.09103825516288,-1.,3.85711487933911));
#40282=CARTESIAN_POINT('Ctrl Pts',(-1.09555606505012,-1.,3.86327241021242));
#40283=CARTESIAN_POINT('Ctrl Pts',(-1.10011198761202,-1.,3.86941120134872));
#40284=CARTESIAN_POINT('Ctrl Pts',(-1.10470536603303,-1.,3.87553067187566));
#40285=CARTESIAN_POINT('Ctrl Pts',(-1.10933577224029,-1.,3.88163105531791));
#40286=CARTESIAN_POINT('Ctrl Pts',(-1.11400292434447,-1.,3.88771308285229));
#40287=CARTESIAN_POINT('Ctrl Pts',(-1.11870660794609,-1.,3.89377768340362));
#40288=CARTESIAN_POINT('Ctrl Pts',(-1.12344660099029,-1.,3.89982569749978));
#40289=CARTESIAN_POINT('Ctrl Pts',(-1.12822258281518,-1.,3.90585753318622));
#40290=CARTESIAN_POINT('Ctrl Pts',(-1.13303414693849,-1.,3.91187321145495));
#40291=CARTESIAN_POINT('Ctrl Pts',(-1.13788084225511,-1.,3.91787251936688));
#40292=CARTESIAN_POINT('Ctrl Pts',(-1.14276220561575,-1.,3.92385513133937));
#40293=CARTESIAN_POINT('Ctrl Pts',(-1.14767779451147,-1.,3.92982073294334));
#40294=CARTESIAN_POINT('Ctrl Pts',(-1.15262722716391,-1.,3.9357691705651));
#40295=CARTESIAN_POINT('Ctrl Pts',(-1.1576101834106,-1.,3.94170046685542));
#40296=CARTESIAN_POINT('Ctrl Pts',(-1.16262637999261,-1.,3.9476147478092));
#40297=CARTESIAN_POINT('Ctrl Pts',(-1.16767555244495,-1.,3.95351219510062));
#40298=CARTESIAN_POINT('Ctrl Pts',(-1.17275743590327,-1.,3.95939299213164));
#40299=CARTESIAN_POINT('Ctrl Pts',(-1.17787174135445,-1.,3.96525726357682));
#40300=CARTESIAN_POINT('Ctrl Pts',(-1.18301815039596,-1.,3.9711050516465));
#40301=CARTESIAN_POINT('Ctrl Pts',(-1.18819633715285,-1.,3.97693634766926));
#40302=CARTESIAN_POINT('Ctrl Pts',(-1.19340598349307,-1.,3.98275111052015));
#40303=CARTESIAN_POINT('Ctrl Pts',(-1.19864679609596,-1.,3.98854928957287));
#40304=CARTESIAN_POINT('Ctrl Pts',(-1.2039185237544,-1.,3.99433084800649));
#40305=CARTESIAN_POINT('Ctrl Pts',(-1.20922097030107,-1.,4.00009577952534));
#40306=CARTESIAN_POINT('Ctrl Pts',(-1.21455398918813,-1.,4.00584409524937));
#40307=CARTESIAN_POINT('Ctrl Pts',(-1.21884478244983,-1.,4.01042947142681));
#40308=CARTESIAN_POINT('Ctrl Pts',(-1.22207656456199,-1.,4.01386104434674));
#40309=CARTESIAN_POINT('Ctrl Pts',(-1.22423716681447,-1.,4.0161454457032));
#40310=CARTESIAN_POINT('Ctrl Pts',(-1.22531898815164,-1.,4.01728681790024));
#40311=CARTESIAN_POINT('',(-1.36999806084572,-1.,3.97027773754922));
#40312=CARTESIAN_POINT('',(-1.22531898815164,-1.,4.01728681790024));
#40313=CARTESIAN_POINT('',(-1.35032489087101,-1.,3.4984457533445));
#40314=CARTESIAN_POINT('Ctrl Pts',(-1.36999806084572,-1.,3.97027773754922));
#40315=CARTESIAN_POINT('Ctrl Pts',(-1.37020239094614,-1.,3.9687184694131));
#40316=CARTESIAN_POINT('Ctrl Pts',(-1.37060761745635,-1.,3.96560037974645));
#40317=CARTESIAN_POINT('Ctrl Pts',(-1.3712051561502,-1.,3.96092458506535));
#40318=CARTESIAN_POINT('Ctrl Pts',(-1.37198126432386,-1.,3.95469287280914));
#40319=CARTESIAN_POINT('Ctrl Pts',(-1.37291699202807,-1.,3.94690771785133));
#40320=CARTESIAN_POINT('Ctrl Pts',(-1.37381821967165,-1.,3.93912709040818));
#40321=CARTESIAN_POINT('Ctrl Pts',(-1.37468482215751,-1.,3.93135106761844));
#40322=CARTESIAN_POINT('Ctrl Pts',(-1.37551664448242,-1.,3.92357976987672));
#40323=CARTESIAN_POINT('Ctrl Pts',(-1.37631350505797,-1.,3.91581337462644));
#40324=CARTESIAN_POINT('Ctrl Pts',(-1.3770751963402,-1.,3.90805209523486));
#40325=CARTESIAN_POINT('Ctrl Pts',(-1.37780148512792,-1.,3.90029615196727));
#40326=CARTESIAN_POINT('Ctrl Pts',(-1.3784921128802,-1.,3.89254574338496));
#40327=CARTESIAN_POINT('Ctrl Pts',(-1.37914679719383,-1.,3.88480102249277));
#40328=CARTESIAN_POINT('Ctrl Pts',(-1.37976523097073,-1.,3.87706205830532));
#40329=CARTESIAN_POINT('Ctrl Pts',(-1.38034709213014,-1.,3.86932885813068));
#40330=CARTESIAN_POINT('Ctrl Pts',(-1.38089205992989,-1.,3.86160143043959));
#40331=CARTESIAN_POINT('Ctrl Pts',(-1.38139983115049,-1.,3.85387983979481));
#40332=CARTESIAN_POINT('Ctrl Pts',(-1.38187013346109,-1.,3.84616425605764));
#40333=CARTESIAN_POINT('Ctrl Pts',(-1.38230274828822,-1.,3.83845502790746));
#40334=CARTESIAN_POINT('Ctrl Pts',(-1.38269750245138,-1.,3.8307526698229));
#40335=CARTESIAN_POINT('Ctrl Pts',(-1.38305421262763,-1.,3.82305771743829));
#40336=CARTESIAN_POINT('Ctrl Pts',(-1.38337263902782,-1.,3.81537060817811));
#40337=CARTESIAN_POINT('Ctrl Pts',(-1.3836524404622,-1.,3.80769156398411));
#40338=CARTESIAN_POINT('Ctrl Pts',(-1.38389311766682,-1.,3.80002044322111));
#40339=CARTESIAN_POINT('Ctrl Pts',(-1.38409399694566,-1.,3.79235669640841));
#40340=CARTESIAN_POINT('Ctrl Pts',(-1.38425435883756,-1.,3.78469969805082));
#40341=CARTESIAN_POINT('Ctrl Pts',(-1.38437354551428,-1.,3.77704902230418));
#40342=CARTESIAN_POINT('Ctrl Pts',(-1.38445107339518,-1.,3.76940473185779));
#40343=CARTESIAN_POINT('Ctrl Pts',(-1.3844867525335,-1.,3.76176768271367));
#40344=CARTESIAN_POINT('Ctrl Pts',(-1.38448077997163,-1.,3.7541397631875));
#40345=CARTESIAN_POINT('Ctrl Pts',(-1.38443344984394,-1.,3.74652317167876));
#40346=CARTESIAN_POINT('Ctrl Pts',(-1.38434489156458,-1.,3.73891976418104));
#40347=CARTESIAN_POINT('Ctrl Pts',(-1.38421479111531,-1.,3.73133035859282));
#40348=CARTESIAN_POINT('Ctrl Pts',(-1.3840421342895,-1.,3.72375409358803));
#40349=CARTESIAN_POINT('Ctrl Pts',(-1.38382489984586,-1.,3.7161876605181));
#40350=CARTESIAN_POINT('Ctrl Pts',(-1.38356065402124,-1.,3.70862680753347));
#40351=CARTESIAN_POINT('Ctrl Pts',(-1.38324717612865,-1.,3.701067921679));
#40352=CARTESIAN_POINT('Ctrl Pts',(-1.38288311171651,-1.,3.69350967899526));
#40353=CARTESIAN_POINT('Ctrl Pts',(-1.38246852827182,-1.,3.68595444983837));
#40354=CARTESIAN_POINT('Ctrl Pts',(-1.3820057429062,-1.,3.67841038482414));
#40355=CARTESIAN_POINT('Ctrl Pts',(-1.38149812653868,-1.,3.67088843112262));
#40356=CARTESIAN_POINT('Ctrl Pts',(-1.38094856333552,-1.,3.66339848520857));
#40357=CARTESIAN_POINT('Ctrl Pts',(-1.38035791051213,-1.,3.6559455440439));
#40358=CARTESIAN_POINT('Ctrl Pts',(-1.37972372481603,-1.,3.64852652756456));
#40359=CARTESIAN_POINT('Ctrl Pts',(-1.37903818567359,-1.,3.64112507791141));
#40360=CARTESIAN_POINT('Ctrl Pts',(-1.37829035457339,-1.,3.63371727442486));
#40361=CARTESIAN_POINT('Ctrl Pts',(-1.37746987919881,-1.,3.62628098665145));
#40362=CARTESIAN_POINT('Ctrl Pts',(-1.37657053403107,-1.,3.6188048116042));
#40363=CARTESIAN_POINT('Ctrl Pts',(-1.37559314436634,-1.,3.61129546591064));
#40364=CARTESIAN_POINT('Ctrl Pts',(-1.37455051379623,-1.,3.60379020123988));
#40365=CARTESIAN_POINT('Ctrl Pts',(-1.37346320103157,-1.,3.59634627869048));
#40366=CARTESIAN_POINT('Ctrl Pts',(-1.37235053660976,-1.,3.58901853846365));
#40367=CARTESIAN_POINT('Ctrl Pts',(-1.37122241663062,-1.,3.58183885982715));
#40368=CARTESIAN_POINT('Ctrl Pts',(-1.37007229485659,-1.,3.57479875549486));
#40369=CARTESIAN_POINT('Ctrl Pts',(-1.36886584973389,-1.,3.5678208030466));
#40370=CARTESIAN_POINT('Ctrl Pts',(-1.36754771771233,-1.,3.56077662028649));
#40371=CARTESIAN_POINT('Ctrl Pts',(-1.3660614545677,-1.,3.55353883995949));
#40372=CARTESIAN_POINT('Ctrl Pts',(-1.36436666257598,-1.,3.54602591832973));
#40373=CARTESIAN_POINT('Ctrl Pts',(-1.36245507339307,-1.,3.53824396424961));
#40374=CARTESIAN_POINT('Ctrl Pts',(-1.36037259643734,-1.,3.530344649616));
#40375=CARTESIAN_POINT('Ctrl Pts',(-1.35821701528836,-1.,3.52261776116748));
#40376=CARTESIAN_POINT('Ctrl Pts',(-1.35611275237152,-1.,3.51542230699556));
#40377=CARTESIAN_POINT('Ctrl Pts',(-1.35419113575956,-1.,3.50913227059999));
#40378=CARTESIAN_POINT('Ctrl Pts',(-1.35257032843486,-1.,3.50408168106261));
#40379=CARTESIAN_POINT('Ctrl Pts',(-1.35142377279517,-1.,3.5007660381649));
#40380=CARTESIAN_POINT('Ctrl Pts',(-1.35080045218587,-1.,3.49920025459723));
#40381=CARTESIAN_POINT('Ctrl Pts',(-1.35049736560527,-1.,3.49861894124827));
#40382=CARTESIAN_POINT('Ctrl Pts',(-1.35036670892966,-1.,3.49847119623846));
#40383=CARTESIAN_POINT('Ctrl Pts',(-1.35032489087101,-1.,3.4984457533445));
#40384=CARTESIAN_POINT('',(-1.51895082866166,-1.,3.42859860294378));
#40385=CARTESIAN_POINT('Origin',(0.,-1.,0.));
#40386=CARTESIAN_POINT('',(-1.83867539237861,-1.,3.77614523045147));
#40387=CARTESIAN_POINT('Ctrl Pts',(-1.51895082866166,-1.,3.42859860294378));
#40388=CARTESIAN_POINT('Ctrl Pts',(-1.51893924967231,-1.,3.42864616361967));
#40389=CARTESIAN_POINT('Ctrl Pts',(-1.51895133295017,-1.,3.42884302333978));
#40390=CARTESIAN_POINT('Ctrl Pts',(-1.51914806898539,-1.,3.42946838852728));
#40391=CARTESIAN_POINT('Ctrl Pts',(-1.5198144909343,-1.,3.4310163189349));
#40392=CARTESIAN_POINT('Ctrl Pts',(-1.52134826724227,-1.,3.43417156977749));
#40393=CARTESIAN_POINT('Ctrl Pts',(-1.52377348950429,-1.,3.43888895974182));
#40394=CARTESIAN_POINT('Ctrl Pts',(-1.52686242875717,-1.,3.44469547527));
#40395=CARTESIAN_POINT('Ctrl Pts',(-1.530462444618,-1.,3.45127136828667));
#40396=CARTESIAN_POINT('Ctrl Pts',(-1.53440195378902,-1.,3.45825932955273));
#40397=CARTESIAN_POINT('Ctrl Pts',(-1.53851507915533,-1.,3.46531752207222));
#40398=CARTESIAN_POINT('Ctrl Pts',(-1.54266605398152,-1.,3.47217189224576));
#40399=CARTESIAN_POINT('Ctrl Pts',(-1.54678009290207,-1.,3.47868272898599));
#40400=CARTESIAN_POINT('Ctrl Pts',(-1.55084702970382,-1.,3.48485155928414));
#40401=CARTESIAN_POINT('Ctrl Pts',(-1.5548959590107,-1.,3.49076460877317));
#40402=CARTESIAN_POINT('Ctrl Pts',(-1.55897703097859,-1.,3.49655185179623));
#40403=CARTESIAN_POINT('Ctrl Pts',(-1.56314187758689,-1.,3.50234321621607));
#40404=CARTESIAN_POINT('Ctrl Pts',(-1.56742097575041,-1.,3.50821771695427));
#40405=CARTESIAN_POINT('Ctrl Pts',(-1.57181569799774,-1.,3.51418598431733));
#40406=CARTESIAN_POINT('Ctrl Pts',(-1.5763104998818,-1.,3.52021847865961));
#40407=CARTESIAN_POINT('Ctrl Pts',(-1.58088027227856,-1.,3.52626275334899));
#40408=CARTESIAN_POINT('Ctrl Pts',(-1.58549906268083,-1.,3.53226378147068));
#40409=CARTESIAN_POINT('Ctrl Pts',(-1.59014958368725,-1.,3.53818616861045));
#40410=CARTESIAN_POINT('Ctrl Pts',(-1.5948276694975,-1.,3.544024581823));
#40411=CARTESIAN_POINT('Ctrl Pts',(-1.59953698113444,-1.,3.54979148634426));
#40412=CARTESIAN_POINT('Ctrl Pts',(-1.60428584699848,-1.,3.55550985096117));
#40413=CARTESIAN_POINT('Ctrl Pts',(-1.60908344685459,-1.,3.56120432482986));
#40414=CARTESIAN_POINT('Ctrl Pts',(-1.61393581747522,-1.,3.56689200468404));
#40415=CARTESIAN_POINT('Ctrl Pts',(-1.61884340915412,-1.,3.57257679609826));
#40416=CARTESIAN_POINT('Ctrl Pts',(-1.62380329464851,-1.,3.57825455954405));
#40417=CARTESIAN_POINT('Ctrl Pts',(-1.62881051550748,-1.,3.5839162577435));
#40418=CARTESIAN_POINT('Ctrl Pts',(-1.63385971451259,-1.,3.58955176627876));
#40419=CARTESIAN_POINT('Ctrl Pts',(-1.63894676675349,-1.,3.59515368334887));
#40420=CARTESIAN_POINT('Ctrl Pts',(-1.6440700438558,-1.,3.6007202851384));
#40421=CARTESIAN_POINT('Ctrl Pts',(-1.64922952425833,-1.,3.60625346556992));
#40422=CARTESIAN_POINT('Ctrl Pts',(-1.65442619244327,-1.,3.61175734965129));
#40423=CARTESIAN_POINT('Ctrl Pts',(-1.65966133399186,-1.,3.61723666482457));
#40424=CARTESIAN_POINT('Ctrl Pts',(-1.66493585923853,-1.,3.62269517989104));
#40425=CARTESIAN_POINT('Ctrl Pts',(-1.67024966008037,-1.,3.62813422105257));
#40426=CARTESIAN_POINT('Ctrl Pts',(-1.67560193613145,-1.,3.63355343201211));
#40427=CARTESIAN_POINT('Ctrl Pts',(-1.68099146651577,-1.,3.63895140887443));
#40428=CARTESIAN_POINT('Ctrl Pts',(-1.68641690471455,-1.,3.64432638915199));
#40429=CARTESIAN_POINT('Ctrl Pts',(-1.691877054817,-1.,3.64967689827393));
#40430=CARTESIAN_POINT('Ctrl Pts',(-1.69737117722559,-1.,3.65500246526798));
#40431=CARTESIAN_POINT('Ctrl Pts',(-1.70289888566904,-1.,3.6603033877491));
#40432=CARTESIAN_POINT('Ctrl Pts',(-1.70846001610983,-1.,3.6655804319893));
#40433=CARTESIAN_POINT('Ctrl Pts',(-1.71405450210392,-1.,3.67083454901629));
#40434=CARTESIAN_POINT('Ctrl Pts',(-1.71968225581787,-1.,3.67606660374665));
#40435=CARTESIAN_POINT('Ctrl Pts',(-1.72534302437003,-1.,3.68127704936472));
#40436=CARTESIAN_POINT('Ctrl Pts',(-1.73103640956647,-1.,3.68646597019188));
#40437=CARTESIAN_POINT('Ctrl Pts',(-1.73676193254493,-1.,3.69163322647906));
#40438=CARTESIAN_POINT('Ctrl Pts',(-1.74251908492589,-1.,3.6967785691046));
#40439=CARTESIAN_POINT('Ctrl Pts',(-1.74830738046092,-1.,3.70190175673422));
#40440=CARTESIAN_POINT('Ctrl Pts',(-1.75412641804148,-1.,3.70700269736876));
#40441=CARTESIAN_POINT('Ctrl Pts',(-1.75997588499021,-1.,3.71208146346454));
#40442=CARTESIAN_POINT('Ctrl Pts',(-1.76585552124549,-1.,3.71713822377675));
#40443=CARTESIAN_POINT('Ctrl Pts',(-1.77176509401846,-1.,3.72217319911429));
#40444=CARTESIAN_POINT('Ctrl Pts',(-1.77770437039606,-1.,3.72718661205504));
#40445=CARTESIAN_POINT('Ctrl Pts',(-1.78367308442682,-1.,3.73217863095022));
#40446=CARTESIAN_POINT('Ctrl Pts',(-1.78967092823139,-1.,3.73714934729962));
#40447=CARTESIAN_POINT('Ctrl Pts',(-1.79569757859041,-1.,3.74209880351667));
#40448=CARTESIAN_POINT('Ctrl Pts',(-1.80175271485519,-1.,3.74702700874954));
#40449=CARTESIAN_POINT('Ctrl Pts',(-1.80783603939662,-1.,3.75193395888069));
#40450=CARTESIAN_POINT('Ctrl Pts',(-1.81394729834032,-1.,3.75681965683995));
#40451=CARTESIAN_POINT('Ctrl Pts',(-1.82008629694924,-1.,3.76168412709652));
#40452=CARTESIAN_POINT('Ctrl Pts',(-1.82625289221933,-1.,3.76652740355856));
#40453=CARTESIAN_POINT('Ctrl Pts',(-1.83120816956515,-1.,3.77038509819777));
#40454=CARTESIAN_POINT('Ctrl Pts',(-1.83493697935064,-1.,3.77326886065484));
#40455=CARTESIAN_POINT('Ctrl Pts',(-1.83742834010821,-1.,3.77518714458232));
#40456=CARTESIAN_POINT('Ctrl Pts',(-1.83867539237861,-1.,3.77614523045147));
#40457=CARTESIAN_POINT('',(-1.97421938526992,-1.,3.70708211654725));
#40458=CARTESIAN_POINT('',(-1.83867539237861,-1.,3.77614523045147));
#40459=CARTESIAN_POINT('',(-1.88097764062542,-1.,3.24413672884902));
#40460=CARTESIAN_POINT('Ctrl Pts',(-1.97421938526992,-1.,3.70708211654725));
#40461=CARTESIAN_POINT('Ctrl Pts',(-1.974177276451,-1.,3.7055100813194));
#40462=CARTESIAN_POINT('Ctrl Pts',(-1.97408973726149,-1.,3.70236698911837));
#40463=CARTESIAN_POINT('Ctrl Pts',(-1.97394846382289,-1.,3.69765528558292));
#40464=CARTESIAN_POINT('Ctrl Pts',(-1.97374016224397,-1.,3.69137888597855));
#40465=CARTESIAN_POINT('Ctrl Pts',(-1.97344650303631,-1.,3.68354319913416));
#40466=CARTESIAN_POINT('Ctrl Pts',(-1.97311947678035,-1.,3.67571738106175));
#40467=CARTESIAN_POINT('Ctrl Pts',(-1.9727589719863,-1.,3.66790152751984));
#40468=CARTESIAN_POINT('Ctrl Pts',(-1.97236485439317,-1.,3.66009578166865));
#40469=CARTESIAN_POINT('Ctrl Pts',(-1.97193697240645,-1.,3.65230034717364));
#40470=CARTESIAN_POINT('Ctrl Pts',(-1.97147515441539,-1.,3.64451546724221));
#40471=CARTESIAN_POINT('Ctrl Pts',(-1.97097920454698,-1.,3.63674139590853));
#40472=CARTESIAN_POINT('Ctrl Pts',(-1.97044889850518,-1.,3.62897836973397));
#40473=CARTESIAN_POINT('Ctrl Pts',(-1.96988398129888,-1.,3.62122658401722));
#40474=CARTESIAN_POINT('Ctrl Pts',(-1.96928416040712,-1.,3.61348615496393));
#40475=CARTESIAN_POINT('Ctrl Pts',(-1.96864911885775,-1.,3.60575714017676));
#40476=CARTESIAN_POINT('Ctrl Pts',(-1.96797854118257,-1.,3.59803959819725));
#40477=CARTESIAN_POINT('Ctrl Pts',(-1.96727213799507,-1.,3.5903336402273));
#40478=CARTESIAN_POINT('Ctrl Pts',(-1.9665296668894,-1.,3.58263947663884));
#40479=CARTESIAN_POINT('Ctrl Pts',(-1.96575096652857,-1.,3.57495748601088));
#40480=CARTESIAN_POINT('Ctrl Pts',(-1.96493594634643,-1.,3.56728820357933));
#40481=CARTESIAN_POINT('Ctrl Pts',(-1.96408450906868,-1.,3.55963218706201));
#40482=CARTESIAN_POINT('Ctrl Pts',(-1.96319648628667,-1.,3.55198990600929));
#40483=CARTESIAN_POINT('Ctrl Pts',(-1.96227157573058,-1.,3.54436163300425));
#40484=CARTESIAN_POINT('Ctrl Pts',(-1.96130926212661,-1.,3.53674730625759));
#40485=CARTESIAN_POINT('Ctrl Pts',(-1.96030879411534,-1.,3.52914648844289));
#40486=CARTESIAN_POINT('Ctrl Pts',(-1.95926936324436,-1.,3.52155867431438));
#40487=CARTESIAN_POINT('Ctrl Pts',(-1.95819025316768,-1.,3.51398354617772));
#40488=CARTESIAN_POINT('Ctrl Pts',(-1.95707099606514,-1.,3.50642124159913));
#40489=CARTESIAN_POINT('Ctrl Pts',(-1.9559115382367,-1.,3.49887263575602));
#40490=CARTESIAN_POINT('Ctrl Pts',(-1.95471236969653,-1.,3.49133956289154));
#40491=CARTESIAN_POINT('Ctrl Pts',(-1.95347412486316,-1.,3.48382414832648));
#40492=CARTESIAN_POINT('Ctrl Pts',(-1.95219722189878,-1.,3.47632820495926));
#40493=CARTESIAN_POINT('Ctrl Pts',(-1.95088147859876,-1.,3.4688525897419));
#40494=CARTESIAN_POINT('Ctrl Pts',(-1.94952575850196,-1.,3.46139661060959));
#40495=CARTESIAN_POINT('Ctrl Pts',(-1.94812754766524,-1.,3.45395731584051));
#40496=CARTESIAN_POINT('Ctrl Pts',(-1.94668377715332,-1.,3.44653088665685));
#40497=CARTESIAN_POINT('Ctrl Pts',(-1.94519168842883,-1.,3.43911410197693));
#40498=CARTESIAN_POINT('Ctrl Pts',(-1.94364973660285,-1.,3.43170586602436));
#40499=CARTESIAN_POINT('Ctrl Pts',(-1.94205835913692,-1.,3.42430850941497));
#40500=CARTESIAN_POINT('Ctrl Pts',(-1.94042111965237,-1.,3.41692971994082));
#40501=CARTESIAN_POINT('Ctrl Pts',(-1.93874306008132,-1.,3.40957978266622));
#40502=CARTESIAN_POINT('Ctrl Pts',(-1.93702857723089,-1.,3.40226802104093));
#40503=CARTESIAN_POINT('Ctrl Pts',(-1.93527929945982,-1.,3.39499923640789));
#40504=CARTESIAN_POINT('Ctrl Pts',(-1.93349233176794,-1.,3.38777076883267));
#40505=CARTESIAN_POINT('Ctrl Pts',(-1.93165739093292,-1.,3.38056768525577));
#40506=CARTESIAN_POINT('Ctrl Pts',(-1.92975993109897,-1.,3.37336807068078));
#40507=CARTESIAN_POINT('Ctrl Pts',(-1.92778626543803,-1.,3.36615168657597));
#40508=CARTESIAN_POINT('Ctrl Pts',(-1.92572846125763,-1.,3.35890824422976));
#40509=CARTESIAN_POINT('Ctrl Pts',(-1.92358838440518,-1.,3.35164424847206));
#40510=CARTESIAN_POINT('Ctrl Pts',(-1.92138450828378,-1.,3.34439448941915));
#40511=CARTESIAN_POINT('Ctrl Pts',(-1.91914609610173,-1.,3.33721230709948));
#40512=CARTESIAN_POINT('Ctrl Pts',(-1.91690081930297,-1.,3.33014884257812));
#40513=CARTESIAN_POINT('Ctrl Pts',(-1.91466343916612,-1.,3.32323403454507));
#40514=CARTESIAN_POINT('Ctrl Pts',(-1.91242616234459,-1.,3.31646052426395));
#40515=CARTESIAN_POINT('Ctrl Pts',(-1.91014297830502,-1.,3.30975721158694));
#40516=CARTESIAN_POINT('Ctrl Pts',(-1.90773912171424,-1.,3.30300595568341));
#40517=CARTESIAN_POINT('Ctrl Pts',(-1.9051389186417,-1.,3.29608978722258));
#40518=CARTESIAN_POINT('Ctrl Pts',(-1.9022897124757,-1.,3.28893448600364));
#40519=CARTESIAN_POINT('Ctrl Pts',(-1.89918429230425,-1.,3.28154737912287));
#40520=CARTESIAN_POINT('Ctrl Pts',(-1.89589172903662,-1.,3.27407108932908));
#40521=CARTESIAN_POINT('Ctrl Pts',(-1.89255393500769,-1.,3.2667765388833));
#40522=CARTESIAN_POINT('Ctrl Pts',(-1.88934996203508,-1.,3.2599988519361));
#40523=CARTESIAN_POINT('Ctrl Pts',(-1.88646802523372,-1.,3.25408686339298));
#40524=CARTESIAN_POINT('Ctrl Pts',(-1.88407708646435,-1.,3.24935200512055));
#40525=CARTESIAN_POINT('Ctrl Pts',(-1.88242596600422,-1.,3.24625654410705));
#40526=CARTESIAN_POINT('Ctrl Pts',(-1.88156537699118,-1.,3.24480754675942));
#40527=CARTESIAN_POINT('Ctrl Pts',(-1.88117508446657,-1.,3.24428080352952));
#40528=CARTESIAN_POINT('Ctrl Pts',(-1.88102292397987,-1.,3.2441553167131));
#40529=CARTESIAN_POINT('Ctrl Pts',(-1.88097764062542,-1.,3.24413672884902));
#40530=CARTESIAN_POINT('',(-2.03660101169564,-1.,3.14877060440425));
#40531=CARTESIAN_POINT('Origin',(0.,-1.,0.));
#40532=CARTESIAN_POINT('',(-2.40675750623143,-1.,3.44202241512147));
#40533=CARTESIAN_POINT('Ctrl Pts',(-2.03660101169564,-1.,3.14877060440425));
#40534=CARTESIAN_POINT('Ctrl Pts',(-2.03659701539175,-1.,3.1488193908823));
#40535=CARTESIAN_POINT('Ctrl Pts',(-2.03663974554941,-1.,3.14901193669147));
#40536=CARTESIAN_POINT('Ctrl Pts',(-2.03693188810614,-1.,3.14959882629936));
#40537=CARTESIAN_POINT('Ctrl Pts',(-2.03783225496023,-1.,3.15102344775396));
#40538=CARTESIAN_POINT('Ctrl Pts',(-2.03984073791432,-1.,3.1538999167466));
#40539=CARTESIAN_POINT('Ctrl Pts',(-2.04297406404132,-1.,3.15817983946525));
#40540=CARTESIAN_POINT('Ctrl Pts',(-2.0469333124766,-1.,3.16343165059235));
#40541=CARTESIAN_POINT('Ctrl Pts',(-2.05151770247452,-1.,3.16936341689859));
#40542=CARTESIAN_POINT('Ctrl Pts',(-2.05650186773279,-1.,3.17564906975592));
#40543=CARTESIAN_POINT('Ctrl Pts',(-2.06166849827143,-1.,3.18197692964677));
#40544=CARTESIAN_POINT('Ctrl Pts',(-2.06684062744065,-1.,3.18809755562297));
#40545=CARTESIAN_POINT('Ctrl Pts',(-2.07192253497765,-1.,3.19388465568113));
#40546=CARTESIAN_POINT('Ctrl Pts',(-2.0769044187063,-1.,3.19934132835879));
#40547=CARTESIAN_POINT('Ctrl Pts',(-2.08182850370816,-1.,3.20454818630635));
#40548=CARTESIAN_POINT('Ctrl Pts',(-2.08676465517435,-1.,3.20962575845433));
#40549=CARTESIAN_POINT('Ctrl Pts',(-2.0917841946046,-1.,3.2146942960168));
#40550=CARTESIAN_POINT('Ctrl Pts',(-2.09692958434933,-1.,3.21982707347067));
#40551=CARTESIAN_POINT('Ctrl Pts',(-2.10220384298533,-1.,3.22503437553496));
#40552=CARTESIAN_POINT('Ctrl Pts',(-2.1075869964248,-1.,3.23028945793334));
#40553=CARTESIAN_POINT('Ctrl Pts',(-2.11304604021784,-1.,3.23554444767115));
#40554=CARTESIAN_POINT('Ctrl Pts',(-2.11854673326972,-1.,3.24074905517282));
#40555=CARTESIAN_POINT('Ctrl Pts',(-2.12406646410943,-1.,3.24587102613347));
#40556=CARTESIAN_POINT('Ctrl Pts',(-2.1296002839681,-1.,3.25090574493994));
#40557=CARTESIAN_POINT('Ctrl Pts',(-2.13515375878786,-1.,3.25586495065027));
#40558=CARTESIAN_POINT('Ctrl Pts',(-2.14073870754257,-1.,3.26077002641868));
#40559=CARTESIAN_POINT('Ctrl Pts',(-2.14636805295663,-1.,3.26564388189764));
#40560=CARTESIAN_POINT('Ctrl Pts',(-2.15205043199818,-1.,3.27050245897244));
#40561=CARTESIAN_POINT('Ctrl Pts',(-2.15778690038359,-1.,3.27534954469206));
#40562=CARTESIAN_POINT('Ctrl Pts',(-2.16357391934434,-1.,3.28018150841414));
#40563=CARTESIAN_POINT('Ctrl Pts',(-2.16940517773459,-1.,3.2849901997973));
#40564=CARTESIAN_POINT('Ctrl Pts',(-2.17527380048422,-1.,3.28976645712566));
#40565=CARTESIAN_POINT('Ctrl Pts',(-2.18117455557062,-1.,3.29450361500484));
#40566=CARTESIAN_POINT('Ctrl Pts',(-2.18710556500325,-1.,3.29920022557635));
#40567=CARTESIAN_POINT('Ctrl Pts',(-2.19306710376112,-1.,3.30385816281831));
#40568=CARTESIAN_POINT('Ctrl Pts',(-2.19906078949924,-1.,3.30848134694596));
#40569=CARTESIAN_POINT('Ctrl Pts',(-2.20508863150608,-1.,3.3130742460895));
#40570=CARTESIAN_POINT('Ctrl Pts',(-2.21115211847872,-1.,3.31764044024231));
#40571=CARTESIAN_POINT('Ctrl Pts',(-2.21725135110889,-1.,3.32218125618955));
#40572=CARTESIAN_POINT('Ctrl Pts',(-2.22338548312758,-1.,3.32669646722871));
#40573=CARTESIAN_POINT('Ctrl Pts',(-2.22955308907221,-1.,3.33118487773593));
#40574=CARTESIAN_POINT('Ctrl Pts',(-2.2357525632881,-1.,3.33564495756478));
#40575=CARTESIAN_POINT('Ctrl Pts',(-2.24198249391437,-1.,3.34007543738044));
#40576=CARTESIAN_POINT('Ctrl Pts',(-2.24824207678288,-1.,3.34447596770768));
#40577=CARTESIAN_POINT('Ctrl Pts',(-2.25453097693524,-1.,3.34884690292342));
#40578=CARTESIAN_POINT('Ctrl Pts',(-2.26084915222484,-1.,3.35318902552676));
#40579=CARTESIAN_POINT('Ctrl Pts',(-2.26719668579921,-1.,3.35750328523077));
#40580=CARTESIAN_POINT('Ctrl Pts',(-2.27357362620902,-1.,3.36179055004369));
#40581=CARTESIAN_POINT('Ctrl Pts',(-2.27997979457968,-1.,3.36605130712978));
#40582=CARTESIAN_POINT('Ctrl Pts',(-2.28641481081045,-1.,3.37028570206357));
#40583=CARTESIAN_POINT('Ctrl Pts',(-2.2928781800731,-1.,3.37449367172707));
#40584=CARTESIAN_POINT('Ctrl Pts',(-2.29936936127588,-1.,3.37867504959382));
#40585=CARTESIAN_POINT('Ctrl Pts',(-2.30588783640389,-1.,3.38282967336676));
#40586=CARTESIAN_POINT('Ctrl Pts',(-2.31243319489505,-1.,3.38695751492659));
#40587=CARTESIAN_POINT('Ctrl Pts',(-2.31900513925627,-1.,3.39105869475112));
#40588=CARTESIAN_POINT('Ctrl Pts',(-2.32560343902683,-1.,3.39513342020045));
#40589=CARTESIAN_POINT('Ctrl Pts',(-2.33222789882601,-1.,3.39918194578115));
#40590=CARTESIAN_POINT('Ctrl Pts',(-2.33887832342715,-1.,3.40320452776646));
#40591=CARTESIAN_POINT('Ctrl Pts',(-2.34555447648901,-1.,3.40720137403888));
#40592=CARTESIAN_POINT('Ctrl Pts',(-2.35225606823649,-1.,3.41117262313464));
#40593=CARTESIAN_POINT('Ctrl Pts',(-2.35898278606449,-1.,3.4151183675076));
#40594=CARTESIAN_POINT('Ctrl Pts',(-2.36573431470314,-1.,3.41903866635384));
#40595=CARTESIAN_POINT('Ctrl Pts',(-2.37251035954351,-1.,3.42293356216595));
#40596=CARTESIAN_POINT('Ctrl Pts',(-2.37931067029517,-1.,3.42680309755241));
#40597=CARTESIAN_POINT('Ctrl Pts',(-2.38613505844641,-1.,3.43064732714472));
#40598=CARTESIAN_POINT('Ctrl Pts',(-2.39298338805823,-1.,3.43446630680436));
#40599=CARTESIAN_POINT('Ctrl Pts',(-2.39848113411429,-1.,3.43750133066036));
#40600=CARTESIAN_POINT('Ctrl Pts',(-2.40261515590099,-1.,3.43976627485223));
#40601=CARTESIAN_POINT('Ctrl Pts',(-2.40537592959345,-1.,3.44127120683402));
#40602=CARTESIAN_POINT('Ctrl Pts',(-2.40675750623143,-1.,3.44202241512147));
#40603=CARTESIAN_POINT('',(-2.52982887637028,-1.,3.35260583073571));
#40604=CARTESIAN_POINT('',(-2.40675750623143,-1.,3.44202241512147));
#40605=CARTESIAN_POINT('',(-2.36531447826073,-1.,2.90994629141676));
#40606=CARTESIAN_POINT('Ctrl Pts',(-2.52982887637028,-1.,3.35260583073571));
#40607=CARTESIAN_POINT('Ctrl Pts',(-2.5295413654909,-1.,3.35105973714071));
#40608=CARTESIAN_POINT('Ctrl Pts',(-2.52896321610703,-1.,3.34796903576663));
#40609=CARTESIAN_POINT('Ctrl Pts',(-2.52808660915689,-1.,3.34333744115511));
#40610=CARTESIAN_POINT('Ctrl Pts',(-2.52689902690158,-1.,3.33717089999103));
#40611=CARTESIAN_POINT('Ctrl Pts',(-2.52538321164634,-1.,3.32947762187533));
#40612=CARTESIAN_POINT('Ctrl Pts',(-2.5238359839626,-1.,3.32179931078699));
#40613=CARTESIAN_POINT('Ctrl Pts',(-2.52225724871313,-1.,3.31413607874645));
#40614=CARTESIAN_POINT('Ctrl Pts',(-2.52064689568511,-1.,3.30648808815442));
#40615=CARTESIAN_POINT('Ctrl Pts',(-2.51900480701069,-1.,3.29885556388352));
#40616=CARTESIAN_POINT('Ctrl Pts',(-2.51733085123797,-1.,3.2912387729927));
#40617=CARTESIAN_POINT('Ctrl Pts',(-2.51562487464514,-1.,3.28363799702982));
#40618=CARTESIAN_POINT('Ctrl Pts',(-2.513886692704,-1.,3.27605350473142));
#40619=CARTESIAN_POINT('Ctrl Pts',(-2.51211608411423,-1.,3.26848552888115));
#40620=CARTESIAN_POINT('Ctrl Pts',(-2.51031277813486,-1.,3.26093423001434));
#40621=CARTESIAN_POINT('Ctrl Pts',(-2.50847647070723,-1.,3.25339971460982));
#40622=CARTESIAN_POINT('Ctrl Pts',(-2.506606859405,-1.,3.24588208983849));
#40623=CARTESIAN_POINT('Ctrl Pts',(-2.5047036758003,-1.,3.23838151080319));
#40624=CARTESIAN_POINT('Ctrl Pts',(-2.50276671338111,-1.,3.23089822320646));
#40625=CARTESIAN_POINT('Ctrl Pts',(-2.50079587201957,-1.,3.22343262620503));
#40626=CARTESIAN_POINT('Ctrl Pts',(-2.4987911459939,-1.,3.21598526261286));
#40627=CARTESIAN_POINT('Ctrl Pts',(-2.4967525264737,-1.,3.20855669849836));
#40628=CARTESIAN_POINT('Ctrl Pts',(-2.49467992057755,-1.,3.20114742397588));
#40629=CARTESIAN_POINT('Ctrl Pts',(-2.49257307239848,-1.,3.19375775555798));
#40630=CARTESIAN_POINT('Ctrl Pts',(-2.49043146334059,-1.,3.18638771282266));
#40631=CARTESIAN_POINT('Ctrl Pts',(-2.48825428288201,-1.,3.17903698136622));
#40632=CARTESIAN_POINT('Ctrl Pts',(-2.48604065348587,-1.,3.17170518863313));
#40633=CARTESIAN_POINT('Ctrl Pts',(-2.48378981792725,-1.,3.16439213290161));
#40634=CARTESIAN_POINT('Ctrl Pts',(-2.48150133566571,-1.,3.15709802322739));
#40635=CARTESIAN_POINT('Ctrl Pts',(-2.47917529057029,-1.,3.14982373241352));
#40636=CARTESIAN_POINT('Ctrl Pts',(-2.47681245356109,-1.,3.1425709954655));
#40637=CARTESIAN_POINT('Ctrl Pts',(-2.47441378371932,-1.,3.13534181229295));
#40638=CARTESIAN_POINT('Ctrl Pts',(-2.47197997765871,-1.,3.12813790805952));
#40639=CARTESIAN_POINT('Ctrl Pts',(-2.46951098947469,-1.,3.12096015766983));
#40640=CARTESIAN_POINT('Ctrl Pts',(-2.46700558843506,-1.,3.11380805536122));
#40641=CARTESIAN_POINT('Ctrl Pts',(-2.46446082979646,-1.,3.1066790790198));
#40642=CARTESIAN_POINT('Ctrl Pts',(-2.46187308501884,-1.,3.09956993697052));
#40643=CARTESIAN_POINT('Ctrl Pts',(-2.4592391256388,-1.,3.09247787931887));
#40644=CARTESIAN_POINT('Ctrl Pts',(-2.45655725437039,-1.,3.08540206545315));
#40645=CARTESIAN_POINT('Ctrl Pts',(-2.4538282678779,-1.,3.07834472886139));
#40646=CARTESIAN_POINT('Ctrl Pts',(-2.45105688854422,-1.,3.07131290521297));
#40647=CARTESIAN_POINT('Ctrl Pts',(-2.44824970516544,-1.,3.06431596421405));
#40648=CARTESIAN_POINT('Ctrl Pts',(-2.44541251892556,-1.,3.05736242671506));
#40649=CARTESIAN_POINT('Ctrl Pts',(-2.44254768923105,-1.,3.05045678021504));
#40650=CARTESIAN_POINT('Ctrl Pts',(-2.43965194061857,-1.,3.04359685040555));
#40651=CARTESIAN_POINT('Ctrl Pts',(-2.43671278042414,-1.,3.03676949672821));
#40652=CARTESIAN_POINT('Ctrl Pts',(-2.43371241361488,-1.,3.02995534946978));
#40653=CARTESIAN_POINT('Ctrl Pts',(-2.43063415586637,-1.,3.02313656036004));
#40654=CARTESIAN_POINT('Ctrl Pts',(-2.42746856264168,-1.,3.01630420830504));
#40655=CARTESIAN_POINT('Ctrl Pts',(-2.42421849439613,-1.,3.00946442616658));
#40656=CARTESIAN_POINT('Ctrl Pts',(-2.42090763946779,-1.,3.00264868585996));
#40657=CARTESIAN_POINT('Ctrl Pts',(-2.41757324500514,-1.,2.99590509293503));
#40658=CARTESIAN_POINT('Ctrl Pts',(-2.41425064199586,-1.,2.98927983005796));
#40659=CARTESIAN_POINT('Ctrl Pts',(-2.41095909342571,-1.,2.98280015815107));
#40660=CARTESIAN_POINT('Ctrl Pts',(-2.40768975073713,-1.,2.97646002822422));
#40661=CARTESIAN_POINT('Ctrl Pts',(-2.40438604734919,-1.,2.9701964131236));
#40662=CARTESIAN_POINT('Ctrl Pts',(-2.4009556571164,-1.,2.96390432240312));
#40663=CARTESIAN_POINT('Ctrl Pts',(-2.39730553974517,-1.,2.95748006482942));
#40664=CARTESIAN_POINT('Ctrl Pts',(-2.39337207631667,-1.,2.95085857128439));
#40665=CARTESIAN_POINT('Ctrl Pts',(-2.38914929090759,-1.,2.94404820669076));
#40666=CARTESIAN_POINT('Ctrl Pts',(-2.38472771516311,-1.,2.93717903280391));
#40667=CARTESIAN_POINT('Ctrl Pts',(-2.38028989582073,-1.,2.93049643640206));
#40668=CARTESIAN_POINT('Ctrl Pts',(-2.3760651052403,-1.,2.92430340582608));
#40669=CARTESIAN_POINT('Ctrl Pts',(-2.37229381109821,-1.,2.91891503791411));
#40670=CARTESIAN_POINT('Ctrl Pts',(-2.36919161373173,-1.,2.9146124988314));
#40671=CARTESIAN_POINT('Ctrl Pts',(-2.36707658451664,-1.,2.91181344022549));
#40672=CARTESIAN_POINT('Ctrl Pts',(-2.36599991765749,-1.,2.91051690822156));
#40673=CARTESIAN_POINT('Ctrl Pts',(-2.36553202948613,-1.,2.91005770527719));
#40674=CARTESIAN_POINT('Ctrl Pts',(-2.36536211188453,-1.,2.90995756655606));
#40675=CARTESIAN_POINT('Ctrl Pts',(-2.36531447826074,-1.,2.90994629141676));
#40676=CARTESIAN_POINT('',(-2.50410331873042,-1.,2.79140942341378));
#40677=CARTESIAN_POINT('Origin',(0.,-1.,0.));
#40678=CARTESIAN_POINT('',(-2.91557726271063,-1.,3.02314558451372));
#40679=CARTESIAN_POINT('Ctrl Pts',(-2.50410331873042,-1.,2.79140942341378));
#40680=CARTESIAN_POINT('Ctrl Pts',(-2.50410700351426,-1.,2.79145823440899));
#40681=CARTESIAN_POINT('Ctrl Pts',(-2.50417932839343,-1.,2.79164172519039));
#40682=CARTESIAN_POINT('Ctrl Pts',(-2.50455968395235,-1.,2.79217568804874));
#40683=CARTESIAN_POINT('Ctrl Pts',(-2.50567182569153,-1.,2.79344192164204));
#40684=CARTESIAN_POINT('Ctrl Pts',(-2.50810555977564,-1.,2.7959687805717));
#40685=CARTESIAN_POINT('Ctrl Pts',(-2.51186983687947,-1.,2.79970585014308));
#40686=CARTESIAN_POINT('Ctrl Pts',(-2.51660190466067,-1.,2.80427363984939));
#40687=CARTESIAN_POINT('Ctrl Pts',(-2.52205778589922,-1.,2.80941521967234));
#40688=CARTESIAN_POINT('Ctrl Pts',(-2.52796388055457,-1.,2.8148437904867));
#40689=CARTESIAN_POINT('Ctrl Pts',(-2.53405679667463,-1.,2.82028550483744));
#40690=CARTESIAN_POINT('Ctrl Pts',(-2.54012272520141,-1.,2.82552167649157));
#40691=CARTESIAN_POINT('Ctrl Pts',(-2.54604736792542,-1.,2.83044254225794));
#40692=CARTESIAN_POINT('Ctrl Pts',(-2.55182152806964,-1.,2.83505269592412));
#40693=CARTESIAN_POINT('Ctrl Pts',(-2.55749952145165,-1.,2.83942515220699));
#40694=CARTESIAN_POINT('Ctrl Pts',(-2.56316920798489,-1.,2.84366802680211));
#40695=CARTESIAN_POINT('Ctrl Pts',(-2.56891984251743,-1.,2.84788893329091));
#40696=CARTESIAN_POINT('Ctrl Pts',(-2.57480482727128,-1.,2.85215360144483));
#40697=CARTESIAN_POINT('Ctrl Pts',(-2.58082875254407,-1.,2.85647171715147));
#40698=CARTESIAN_POINT('Ctrl Pts',(-2.5869677064356,-1.,2.86081999003668));
#40699=CARTESIAN_POINT('Ctrl Pts',(-2.59318160184921,-1.,2.86515629953528));
#40700=CARTESIAN_POINT('Ctrl Pts',(-2.59942875223202,-1.,2.86943633170712));
#40701=CARTESIAN_POINT('Ctrl Pts',(-2.6056817788128,-1.,2.87363176656475));
#40702=CARTESIAN_POINT('Ctrl Pts',(-2.61193507170928,-1.,2.87773881947885));
#40703=CARTESIAN_POINT('Ctrl Pts',(-2.61819596473087,-1.,2.88176821427502));
#40704=CARTESIAN_POINT('Ctrl Pts',(-2.62447947640253,-1.,2.88573922195049));
#40705=CARTESIAN_POINT('Ctrl Pts',(-2.63080195420771,-1.,2.88967244854243));
#40706=CARTESIAN_POINT('Ctrl Pts',(-2.63717442263944,-1.,2.89358228854557));
#40707=CARTESIAN_POINT('Ctrl Pts',(-2.64359851684146,-1.,2.89747231723361));
#40708=CARTESIAN_POINT('Ctrl Pts',(-2.65007017365576,-1.,2.90133950224879));
#40709=CARTESIAN_POINT('Ctrl Pts',(-2.65658188464287,-1.,2.90517678087467));
#40710=CARTESIAN_POINT('Ctrl Pts',(-2.66312542616809,-1.,2.90897617968921));
#40711=CARTESIAN_POINT('Ctrl Pts',(-2.66969458792627,-1.,2.91273193382876));
#40712=CARTESIAN_POINT('Ctrl Pts',(-2.67628728855309,-1.,2.91644290704281));
#40713=CARTESIAN_POINT('Ctrl Pts',(-2.68290409279689,-1.,2.92011090722152));
#40714=CARTESIAN_POINT('Ctrl Pts',(-2.68954721165342,-1.,2.92373955325876));
#40715=CARTESIAN_POINT('Ctrl Pts',(-2.69621932864302,-1.,2.92733294395268));
#40716=CARTESIAN_POINT('Ctrl Pts',(-2.70292247416881,-1.,2.93089438233746));
#40717=CARTESIAN_POINT('Ctrl Pts',(-2.70965695523776,-1.,2.93442516311168));
#40718=CARTESIAN_POINT('Ctrl Pts',(-2.71642190053575,-1.,2.93792519474955));
#40719=CARTESIAN_POINT('Ctrl Pts',(-2.72321571511322,-1.,2.94139351933882));
#40720=CARTESIAN_POINT('Ctrl Pts',(-2.73003657371613,-1.,2.94482887675139));
#40721=CARTESIAN_POINT('Ctrl Pts',(-2.73688288329825,-1.,2.94823023414381));
#40722=CARTESIAN_POINT('Ctrl Pts',(-2.7437537949221,-1.,2.95159737214305));
#40723=CARTESIAN_POINT('Ctrl Pts',(-2.75064903318996,-1.,2.95493069316211));
#40724=CARTESIAN_POINT('Ctrl Pts',(-2.75756867888393,-1.,2.9582309766594));
#40725=CARTESIAN_POINT('Ctrl Pts',(-2.76451296269571,-1.,2.96149914764832));
#40726=CARTESIAN_POINT('Ctrl Pts',(-2.77148206836464,-1.,2.96473605585548));
#40727=CARTESIAN_POINT('Ctrl Pts',(-2.77847589542767,-1.,2.9679422104295));
#40728=CARTESIAN_POINT('Ctrl Pts',(-2.78549409123657,-1.,2.97111781461349));
#40729=CARTESIAN_POINT('Ctrl Pts',(-2.79253615718147,-1.,2.97426288347475));
#40730=CARTESIAN_POINT('Ctrl Pts',(-2.79960153278186,-1.,2.97737733718242));
#40731=CARTESIAN_POINT('Ctrl Pts',(-2.80668968101162,-1.,2.98046109647299));
#40732=CARTESIAN_POINT('Ctrl Pts',(-2.81380019196454,-1.,2.9835141977994));
#40733=CARTESIAN_POINT('Ctrl Pts',(-2.82093279065704,-1.,2.98653680669434));
#40734=CARTESIAN_POINT('Ctrl Pts',(-2.82808728190402,-1.,2.98952916401699));
#40735=CARTESIAN_POINT('Ctrl Pts',(-2.83526351254383,-1.,2.99249155170479));
#40736=CARTESIAN_POINT('Ctrl Pts',(-2.84246132984334,-1.,2.995424253416));
#40737=CARTESIAN_POINT('Ctrl Pts',(-2.84968053289104,-1.,2.99832751144566));
#40738=CARTESIAN_POINT('Ctrl Pts',(-2.85692085715129,-1.,3.0012015079552));
#40739=CARTESIAN_POINT('Ctrl Pts',(-2.86418200833065,-1.,3.00404638316245));
#40740=CARTESIAN_POINT('Ctrl Pts',(-2.87146368430104,-1.,3.00686224485374));
#40741=CARTESIAN_POINT('Ctrl Pts',(-2.87876560072799,-1.,3.0096491810855));
#40742=CARTESIAN_POINT('Ctrl Pts',(-2.88608751706796,-1.,3.01240727309568));
#40743=CARTESIAN_POINT('Ctrl Pts',(-2.8934292556764,-1.,3.01513660433291));
#40744=CARTESIAN_POINT('Ctrl Pts',(-2.90079069102661,-1.,3.01783725123646));
#40745=CARTESIAN_POINT('Ctrl Pts',(-2.90669553303902,-1.,3.01997487194926));
#40746=CARTESIAN_POINT('Ctrl Pts',(-2.91113297349052,-1.,3.02156522743299));
#40747=CARTESIAN_POINT('Ctrl Pts',(-2.91409518070707,-1.,3.02261975104912));
#40748=CARTESIAN_POINT('Ctrl Pts',(-2.91557726271063,-1.,3.02314558451372));
#40749=CARTESIAN_POINT('',(-3.02314558451372,-1.,2.91557726271063));
#40750=CARTESIAN_POINT('',(-2.91557726271063,-1.,3.02314558451372));
#40751=CARTESIAN_POINT('',(-2.79140942341258,-1.,2.50410331873176));
#40752=CARTESIAN_POINT('Ctrl Pts',(-3.02314558451372,-1.,2.91557726271063));
#40753=CARTESIAN_POINT('Ctrl Pts',(-3.02261975104593,-1.,2.91409518070399));
#40754=CARTESIAN_POINT('Ctrl Pts',(-3.02156522742431,-1.,2.91113297348212));
#40755=CARTESIAN_POINT('Ctrl Pts',(-3.01997487193503,-1.,2.90669553302526));
#40756=CARTESIAN_POINT('Ctrl Pts',(-3.01783725121981,-1.,2.9007906910105));
#40757=CARTESIAN_POINT('Ctrl Pts',(-3.01513660431928,-1.,2.89342925566321));
#40758=CARTESIAN_POINT('Ctrl Pts',(-3.01240727308829,-1.,2.8860875170608));
#40759=CARTESIAN_POINT('Ctrl Pts',(-3.00964918108476,-1.,2.87876560072727));
#40760=CARTESIAN_POINT('Ctrl Pts',(-3.00686224485784,-1.,2.87146368430502));
#40761=CARTESIAN_POINT('Ctrl Pts',(-3.00404638316867,-1.,2.86418200833667));
#40762=CARTESIAN_POINT('Ctrl Pts',(-3.00120150796095,-1.,2.85692085715686));
#40763=CARTESIAN_POINT('Ctrl Pts',(-2.99832751144925,-1.,2.84968053289451));
#40764=CARTESIAN_POINT('Ctrl Pts',(-2.99542425341685,-1.,2.84246132984415));
#40765=CARTESIAN_POINT('Ctrl Pts',(-2.9924915517034,-1.,2.83526351254248));
#40766=CARTESIAN_POINT('Ctrl Pts',(-2.98952916401446,-1.,2.82808728190157));
#40767=CARTESIAN_POINT('Ctrl Pts',(-2.9865368066918,-1.,2.82093279065457));
#40768=CARTESIAN_POINT('Ctrl Pts',(-2.98351419779767,-1.,2.81380019196286));
#40769=CARTESIAN_POINT('Ctrl Pts',(-2.98046109647241,-1.,2.80668968101106));
#40770=CARTESIAN_POINT('Ctrl Pts',(-2.97737733718287,-1.,2.7996015327823));
#40771=CARTESIAN_POINT('Ctrl Pts',(-2.9742628834758,-1.,2.79253615718248));
#40772=CARTESIAN_POINT('Ctrl Pts',(-2.97111781461465,-1.,2.78549409123769));
#40773=CARTESIAN_POINT('Ctrl Pts',(-2.96794221043036,-1.,2.7784758954285));
#40774=CARTESIAN_POINT('Ctrl Pts',(-2.96473605585583,-1.,2.77148206836498));
#40775=CARTESIAN_POINT('Ctrl Pts',(-2.96149914764818,-1.,2.76451296269557));
#40776=CARTESIAN_POINT('Ctrl Pts',(-2.95823097665896,-1.,2.7575686788835));
#40777=CARTESIAN_POINT('Ctrl Pts',(-2.95493069316161,-1.,2.75064903318947));
#40778=CARTESIAN_POINT('Ctrl Pts',(-2.95159737214266,-1.,2.74375379492172));
#40779=CARTESIAN_POINT('Ctrl Pts',(-2.94823023414364,-1.,2.73688288329808));
#40780=CARTESIAN_POINT('Ctrl Pts',(-2.94482887675143,-1.,2.73003657371617));
#40781=CARTESIAN_POINT('Ctrl Pts',(-2.94139351933897,-1.,2.72321571511337));
#40782=CARTESIAN_POINT('Ctrl Pts',(-2.93792519474972,-1.,2.71642190053592));
#40783=CARTESIAN_POINT('Ctrl Pts',(-2.93442516311179,-1.,2.70965695523787));
#40784=CARTESIAN_POINT('Ctrl Pts',(-2.9308943823375,-1.,2.70292247416885));
#40785=CARTESIAN_POINT('Ctrl Pts',(-2.92733294395267,-1.,2.69621932864301));
#40786=CARTESIAN_POINT('Ctrl Pts',(-2.92373955325875,-1.,2.68954721165339));
#40787=CARTESIAN_POINT('Ctrl Pts',(-2.92011090722152,-1.,2.68290409279688));
#40788=CARTESIAN_POINT('Ctrl Pts',(-2.91644290704285,-1.,2.67628728855312));
#40789=CARTESIAN_POINT('Ctrl Pts',(-2.91273193382882,-1.,2.66969458792631));
#40790=CARTESIAN_POINT('Ctrl Pts',(-2.90897617968923,-1.,2.6631254261681));
#40791=CARTESIAN_POINT('Ctrl Pts',(-2.90517678087461,-1.,2.65658188464282));
#40792=CARTESIAN_POINT('Ctrl Pts',(-2.90133950224867,-1.,2.65007017365564));
#40793=CARTESIAN_POINT('Ctrl Pts',(-2.89747231723345,-1.,2.64359851684131));
#40794=CARTESIAN_POINT('Ctrl Pts',(-2.89358228854544,-1.,2.63717442263932));
#40795=CARTESIAN_POINT('Ctrl Pts',(-2.88967244854239,-1.,2.63080195420767));
#40796=CARTESIAN_POINT('Ctrl Pts',(-2.88573922195059,-1.,2.62447947640262));
#40797=CARTESIAN_POINT('Ctrl Pts',(-2.88176821427525,-1.,2.61819596473108));
#40798=CARTESIAN_POINT('Ctrl Pts',(-2.87773881947916,-1.,2.61193507170955));
#40799=CARTESIAN_POINT('Ctrl Pts',(-2.87363176656501,-1.,2.60568177881303));
#40800=CARTESIAN_POINT('Ctrl Pts',(-2.86943633170722,-1.,2.5994287522321));
#40801=CARTESIAN_POINT('Ctrl Pts',(-2.86515629953513,-1.,2.59318160184908));
#40802=CARTESIAN_POINT('Ctrl Pts',(-2.86081999003629,-1.,2.58696770643524));
#40803=CARTESIAN_POINT('Ctrl Pts',(-2.85647171715092,-1.,2.58082875254357));
#40804=CARTESIAN_POINT('Ctrl Pts',(-2.85215360144431,-1.,2.57480482727081));
#40805=CARTESIAN_POINT('Ctrl Pts',(-2.84788893329067,-1.,2.56891984251721));
#40806=CARTESIAN_POINT('Ctrl Pts',(-2.84366802680237,-1.,2.56316920798513));
#40807=CARTESIAN_POINT('Ctrl Pts',(-2.83942515220782,-1.,2.55749952145241));
#40808=CARTESIAN_POINT('Ctrl Pts',(-2.83505269592536,-1.,2.55182152807077));
#40809=CARTESIAN_POINT('Ctrl Pts',(-2.83044254225917,-1.,2.54604736792655));
#40810=CARTESIAN_POINT('Ctrl Pts',(-2.8255216764922,-1.,2.54012272520199));
#40811=CARTESIAN_POINT('Ctrl Pts',(-2.82028550483689,-1.,2.53405679667412));
#40812=CARTESIAN_POINT('Ctrl Pts',(-2.81484379048475,-1.,2.52796388055278));
#40813=CARTESIAN_POINT('Ctrl Pts',(-2.80941521966941,-1.,2.52205778589653));
#40814=CARTESIAN_POINT('Ctrl Pts',(-2.80427363984653,-1.,2.51660190465805));
#40815=CARTESIAN_POINT('Ctrl Pts',(-2.79970585014168,-1.,2.51186983687818));
#40816=CARTESIAN_POINT('Ctrl Pts',(-2.79596878057287,-1.,2.50810555977671));
#40817=CARTESIAN_POINT('Ctrl Pts',(-2.79344192164147,-1.,2.50567182569081));
#40818=CARTESIAN_POINT('Ctrl Pts',(-2.79217568804755,-1.,2.50455968395146));
#40819=CARTESIAN_POINT('Ctrl Pts',(-2.79164172518905,-1.,2.50417932839313));
#40820=CARTESIAN_POINT('Ctrl Pts',(-2.79145823440781,-1.,2.50410700351493));
#40821=CARTESIAN_POINT('Ctrl Pts',(-2.79140942341258,-1.,2.50410331873176));
#40822=CARTESIAN_POINT('',(-2.90994629141562,-1.,2.36531447826213));
#40823=CARTESIAN_POINT('Origin',(0.,-1.,0.));
#40824=CARTESIAN_POINT('',(-3.35260583073571,-1.,2.52982887637028));
#40825=CARTESIAN_POINT('Ctrl Pts',(-2.90994629141562,-1.,2.36531447826213));
#40826=CARTESIAN_POINT('Ctrl Pts',(-2.90995756655558,-1.,2.3653621118858));
#40827=CARTESIAN_POINT('Ctrl Pts',(-2.9100577052777,-1.,2.36553202948741));
#40828=CARTESIAN_POINT('Ctrl Pts',(-2.91051690822262,-1.,2.36599991765853));
#40829=CARTESIAN_POINT('Ctrl Pts',(-2.91181344022628,-1.,2.36707658451709));
#40830=CARTESIAN_POINT('Ctrl Pts',(-2.91461249883016,-1.,2.36919161373074));
#40831=CARTESIAN_POINT('Ctrl Pts',(-2.9189150379156,-1.,2.37229381109939));
#40832=CARTESIAN_POINT('Ctrl Pts',(-2.92430340582912,-1.,2.37606510524271));
#40833=CARTESIAN_POINT('Ctrl Pts',(-2.93049643640517,-1.,2.3802898958232));
#40834=CARTESIAN_POINT('Ctrl Pts',(-2.93717903280599,-1.,2.38472771516476));
#40835=CARTESIAN_POINT('Ctrl Pts',(-2.94404820669135,-1.,2.38914929090806));
#40836=CARTESIAN_POINT('Ctrl Pts',(-2.95085857128372,-1.,2.39337207631613));
#40837=CARTESIAN_POINT('Ctrl Pts',(-2.95748006482811,-1.,2.39730553974412));
#40838=CARTESIAN_POINT('Ctrl Pts',(-2.96390432240181,-1.,2.40095565711535));
#40839=CARTESIAN_POINT('Ctrl Pts',(-2.97019641312272,-1.,2.40438604734848));
#40840=CARTESIAN_POINT('Ctrl Pts',(-2.97646002822395,-1.,2.40768975073691));
#40841=CARTESIAN_POINT('Ctrl Pts',(-2.98280015815132,-1.,2.41095909342591));
#40842=CARTESIAN_POINT('Ctrl Pts',(-2.98927983005851,-1.,2.4142506419963));
#40843=CARTESIAN_POINT('Ctrl Pts',(-2.99590509293561,-1.,2.4175732450056));
#40844=CARTESIAN_POINT('Ctrl Pts',(-3.00264868586038,-1.,2.42090763946812));
#40845=CARTESIAN_POINT('Ctrl Pts',(-3.00946442616674,-1.,2.42421849439625));
#40846=CARTESIAN_POINT('Ctrl Pts',(-3.01630420830494,-1.,2.4274685626416));
#40847=CARTESIAN_POINT('Ctrl Pts',(-3.02313656035977,-1.,2.43063415586615));
#40848=CARTESIAN_POINT('Ctrl Pts',(-3.02995534946946,-1.,2.43371241361462));
#40849=CARTESIAN_POINT('Ctrl Pts',(-3.03676949672797,-1.,2.43671278042394));
#40850=CARTESIAN_POINT('Ctrl Pts',(-3.04359685040545,-1.,2.43965194061849));
#40851=CARTESIAN_POINT('Ctrl Pts',(-3.05045678021509,-1.,2.44254768923109));
#40852=CARTESIAN_POINT('Ctrl Pts',(-3.05736242671521,-1.,2.44541251892568));
#40853=CARTESIAN_POINT('Ctrl Pts',(-3.06431596421422,-1.,2.44824970516558));
#40854=CARTESIAN_POINT('Ctrl Pts',(-3.0713129052131,-1.,2.45105688854432));
#40855=CARTESIAN_POINT('Ctrl Pts',(-3.07834472886145,-1.,2.45382826787795));
#40856=CARTESIAN_POINT('Ctrl Pts',(-3.08540206545313,-1.,2.45655725437037));
#40857=CARTESIAN_POINT('Ctrl Pts',(-3.09247787931881,-1.,2.45923912563875));
#40858=CARTESIAN_POINT('Ctrl Pts',(-3.09956993697048,-1.,2.4618730850188));
#40859=CARTESIAN_POINT('Ctrl Pts',(-3.10667907901981,-1.,2.46446082979645));
#40860=CARTESIAN_POINT('Ctrl Pts',(-3.11380805536124,-1.,2.46700558843507));
#40861=CARTESIAN_POINT('Ctrl Pts',(-3.12096015766984,-1.,2.4695109894747));
#40862=CARTESIAN_POINT('Ctrl Pts',(-3.12813790805948,-1.,2.47197997765868));
#40863=CARTESIAN_POINT('Ctrl Pts',(-3.13534181229282,-1.,2.47441378371923));
#40864=CARTESIAN_POINT('Ctrl Pts',(-3.14257099546531,-1.,2.47681245356095));
#40865=CARTESIAN_POINT('Ctrl Pts',(-3.14982373241335,-1.,2.47917529057016));
#40866=CARTESIAN_POINT('Ctrl Pts',(-3.15709802322735,-1.,2.48150133566568));
#40867=CARTESIAN_POINT('Ctrl Pts',(-3.16439213290181,-1.,2.48378981792739));
#40868=CARTESIAN_POINT('Ctrl Pts',(-3.17170518863357,-1.,2.48604065348619));
#40869=CARTESIAN_POINT('Ctrl Pts',(-3.17903698136679,-1.,2.48825428288243));
#40870=CARTESIAN_POINT('Ctrl Pts',(-3.18638771282315,-1.,2.49043146334095));
#40871=CARTESIAN_POINT('Ctrl Pts',(-3.19375775555814,-1.,2.4925730723986));
#40872=CARTESIAN_POINT('Ctrl Pts',(-3.20114742397549,-1.,2.49467992057726));
#40873=CARTESIAN_POINT('Ctrl Pts',(-3.2085566984974,-1.,2.49675252647298));
#40874=CARTESIAN_POINT('Ctrl Pts',(-3.21598526261157,-1.,2.49879114599293));
#40875=CARTESIAN_POINT('Ctrl Pts',(-3.22343262620387,-1.,2.5007958720187));
#40876=CARTESIAN_POINT('Ctrl Pts',(-3.23089822320596,-1.,2.50276671338074));
#40877=CARTESIAN_POINT('Ctrl Pts',(-3.23838151080383,-1.,2.50470367580078));
#40878=CARTESIAN_POINT('Ctrl Pts',(-3.24588208984042,-1.,2.50660685940645));
#40879=CARTESIAN_POINT('Ctrl Pts',(-3.25339971461265,-1.,2.50847647070936));
#40880=CARTESIAN_POINT('Ctrl Pts',(-3.26093423001716,-1.,2.51031277813697));
#40881=CARTESIAN_POINT('Ctrl Pts',(-3.26848552888271,-1.,2.51211608411539));
#40882=CARTESIAN_POINT('Ctrl Pts',(-3.27605350473048,-1.,2.51388669270329));
#40883=CARTESIAN_POINT('Ctrl Pts',(-3.28363799702583,-1.,2.51562487464215));
#40884=CARTESIAN_POINT('Ctrl Pts',(-3.2912387729863,-1.,2.51733085123316));
#40885=CARTESIAN_POINT('Ctrl Pts',(-3.29885556387661,-1.,2.51900480700548));
#40886=CARTESIAN_POINT('Ctrl Pts',(-3.30648808814986,-1.,2.52064689568167));
#40887=CARTESIAN_POINT('Ctrl Pts',(-3.31413607874727,-1.,2.52225724871375));
#40888=CARTESIAN_POINT('Ctrl Pts',(-3.32179931079521,-1.,2.52383598396878));
#40889=CARTESIAN_POINT('Ctrl Pts',(-3.32947762189049,-1.,2.52538321165774));
#40890=CARTESIAN_POINT('Ctrl Pts',(-3.33717090000955,-1.,2.52689902691551));
#40891=CARTESIAN_POINT('Ctrl Pts',(-3.34333744117093,-1.,2.52808660916879));
#40892=CARTESIAN_POINT('Ctrl Pts',(-3.34796903577628,-1.,2.5289632161143));
#40893=CARTESIAN_POINT('Ctrl Pts',(-3.35105973714426,-1.,2.52954136549357));
#40894=CARTESIAN_POINT('Ctrl Pts',(-3.35260583073571,-1.,2.52982887637028));
#40895=CARTESIAN_POINT('',(-3.44202241512147,-1.,2.40675750623143));
#40896=CARTESIAN_POINT('',(-3.35260583073571,-1.,2.52982887637028));
#40897=CARTESIAN_POINT('',(-3.14877060440327,-1.,2.03660101169715));
#40898=CARTESIAN_POINT('Ctrl Pts',(-3.44202241512147,-1.,2.40675750623143));
#40899=CARTESIAN_POINT('Ctrl Pts',(-3.44127120683039,-1.,2.4053759295909));
#40900=CARTESIAN_POINT('Ctrl Pts',(-3.43976627484234,-1.,2.40261515589405));
#40901=CARTESIAN_POINT('Ctrl Pts',(-3.43750133064416,-1.,2.39848113410292));
#40902=CARTESIAN_POINT('Ctrl Pts',(-3.4344663067854,-1.,2.39298338804493));
#40903=CARTESIAN_POINT('Ctrl Pts',(-3.4306473271292,-1.,2.38613505843552));
#40904=CARTESIAN_POINT('Ctrl Pts',(-3.42680309754399,-1.,2.37931067028926));
#40905=CARTESIAN_POINT('Ctrl Pts',(-3.42293356216511,-1.,2.37251035954292));
#40906=CARTESIAN_POINT('Ctrl Pts',(-3.41903866635852,-1.,2.36573431470642));
#40907=CARTESIAN_POINT('Ctrl Pts',(-3.41511836751469,-1.,2.35898278606946));
#40908=CARTESIAN_POINT('Ctrl Pts',(-3.41117262314119,-1.,2.35225606824109));
#40909=CARTESIAN_POINT('Ctrl Pts',(-3.40720137404297,-1.,2.34555447649188));
#40910=CARTESIAN_POINT('Ctrl Pts',(-3.40320452776743,-1.,2.33887832342782));
#40911=CARTESIAN_POINT('Ctrl Pts',(-3.39918194577956,-1.,2.33222789882489));
#40912=CARTESIAN_POINT('Ctrl Pts',(-3.39513342019756,-1.,2.3256034390248));
#40913=CARTESIAN_POINT('Ctrl Pts',(-3.39105869474822,-1.,2.31900513925424));
#40914=CARTESIAN_POINT('Ctrl Pts',(-3.38695751492462,-1.,2.31243319489367));
#40915=CARTESIAN_POINT('Ctrl Pts',(-3.3828296733661,-1.,2.30588783640343));
#40916=CARTESIAN_POINT('Ctrl Pts',(-3.37867504959433,-1.,2.29936936127624));
#40917=CARTESIAN_POINT('Ctrl Pts',(-3.37449367172826,-1.,2.29287818007393));
#40918=CARTESIAN_POINT('Ctrl Pts',(-3.37028570206488,-1.,2.28641481081137));
#40919=CARTESIAN_POINT('Ctrl Pts',(-3.36605130713076,-1.,2.27997979458037));
#40920=CARTESIAN_POINT('Ctrl Pts',(-3.36179055004409,-1.,2.2735736262093));
#40921=CARTESIAN_POINT('Ctrl Pts',(-3.35750328523061,-1.,2.2671966857991));
#40922=CARTESIAN_POINT('Ctrl Pts',(-3.35318902552626,-1.,2.26084915222449));
#40923=CARTESIAN_POINT('Ctrl Pts',(-3.34884690292285,-1.,2.25453097693483));
#40924=CARTESIAN_POINT('Ctrl Pts',(-3.34447596770723,-1.,2.24824207678256));
#40925=CARTESIAN_POINT('Ctrl Pts',(-3.34007543738025,-1.,2.24198249391422));
#40926=CARTESIAN_POINT('Ctrl Pts',(-3.33564495756482,-1.,2.23575256328812));
#40927=CARTESIAN_POINT('Ctrl Pts',(-3.33118487773611,-1.,2.22955308907233));
#40928=CARTESIAN_POINT('Ctrl Pts',(-3.3266964672289,-1.,2.22338548312772));
#40929=CARTESIAN_POINT('Ctrl Pts',(-3.32218125618968,-1.,2.21725135110898));
#40930=CARTESIAN_POINT('Ctrl Pts',(-3.31764044024235,-1.,2.21115211847875));
#40931=CARTESIAN_POINT('Ctrl Pts',(-3.31307424608949,-1.,2.20508863150607));
#40932=CARTESIAN_POINT('Ctrl Pts',(-3.30848134694595,-1.,2.19906078949923));
#40933=CARTESIAN_POINT('Ctrl Pts',(-3.30385816281831,-1.,2.19306710376111));
#40934=CARTESIAN_POINT('Ctrl Pts',(-3.29920022557639,-1.,2.18710556500327));
#40935=CARTESIAN_POINT('Ctrl Pts',(-3.2945036150049,-1.,2.18117455557065));
#40936=CARTESIAN_POINT('Ctrl Pts',(-3.28976645712568,-1.,2.17527380048423));
#40937=CARTESIAN_POINT('Ctrl Pts',(-3.28499019979724,-1.,2.16940517773455));
#40938=CARTESIAN_POINT('Ctrl Pts',(-3.280181508414,-1.,2.16357391934425));
#40939=CARTESIAN_POINT('Ctrl Pts',(-3.27534954469187,-1.,2.15778690038347));
#40940=CARTESIAN_POINT('Ctrl Pts',(-3.27050245897228,-1.,2.15205043199808));
#40941=CARTESIAN_POINT('Ctrl Pts',(-3.26564388189759,-1.,2.1463680529566));
#40942=CARTESIAN_POINT('Ctrl Pts',(-3.26077002641879,-1.,2.14073870754264));
#40943=CARTESIAN_POINT('Ctrl Pts',(-3.25586495065054,-1.,2.13515375878803));
#40944=CARTESIAN_POINT('Ctrl Pts',(-3.25090574494028,-1.,2.12960028396832));
#40945=CARTESIAN_POINT('Ctrl Pts',(-3.24587102613376,-1.,2.12406646410962));
#40946=CARTESIAN_POINT('Ctrl Pts',(-3.24074905517293,-1.,2.11854673326979));
#40947=CARTESIAN_POINT('Ctrl Pts',(-3.23554444767099,-1.,2.11304604021773));
#40948=CARTESIAN_POINT('Ctrl Pts',(-3.23028945793289,-1.,2.10758699642451));
#40949=CARTESIAN_POINT('Ctrl Pts',(-3.22503437553434,-1.,2.10220384298492));
#40950=CARTESIAN_POINT('Ctrl Pts',(-3.21982707347009,-1.,2.09692958434895));
#40951=CARTESIAN_POINT('Ctrl Pts',(-3.21469429601654,-1.,2.09178419460443));
#40952=CARTESIAN_POINT('Ctrl Pts',(-3.20962575845463,-1.,2.08676465517455));
#40953=CARTESIAN_POINT('Ctrl Pts',(-3.2045481863073,-1.,2.08182850370878));
#40954=CARTESIAN_POINT('Ctrl Pts',(-3.19934132836019,-1.,2.07690441870722));
#40955=CARTESIAN_POINT('Ctrl Pts',(-3.19388465568252,-1.,2.07192253497857));
#40956=CARTESIAN_POINT('Ctrl Pts',(-3.18809755562368,-1.,2.06684062744112));
#40957=CARTESIAN_POINT('Ctrl Pts',(-3.18197692964614,-1.,2.06166849827101));
#40958=CARTESIAN_POINT('Ctrl Pts',(-3.17564906975371,-1.,2.05650186773132));
#40959=CARTESIAN_POINT('Ctrl Pts',(-3.16936341689527,-1.,2.05151770247233));
#40960=CARTESIAN_POINT('Ctrl Pts',(-3.16343165058912,-1.,2.04693331247446));
#40961=CARTESIAN_POINT('Ctrl Pts',(-3.15817983946367,-1.,2.04297406404027));
#40962=CARTESIAN_POINT('Ctrl Pts',(-3.15389991674792,-1.,2.03984073791519));
#40963=CARTESIAN_POINT('Ctrl Pts',(-3.15102344775328,-1.,2.03783225495961));
#40964=CARTESIAN_POINT('Ctrl Pts',(-3.14959882629805,-1.,2.03693188810544));
#40965=CARTESIAN_POINT('Ctrl Pts',(-3.1490119366901,-1.,2.03663974554932));
#40966=CARTESIAN_POINT('Ctrl Pts',(-3.14881939088124,-1.,2.03659701539259));
#40967=CARTESIAN_POINT('Ctrl Pts',(-3.14877060440328,-1.,2.03660101169715));
#40968=CARTESIAN_POINT('',(-3.24413672884812,-1.,1.88097764062697));
#40969=CARTESIAN_POINT('Origin',(0.,-1.,0.));
#40970=CARTESIAN_POINT('',(-3.70708211654725,-1.,1.97421938526992));
#40971=CARTESIAN_POINT('Ctrl Pts',(-3.24413672884812,-1.,1.88097764062697));
#40972=CARTESIAN_POINT('Ctrl Pts',(-3.24415531671284,-1.,1.8810229239812));
#40973=CARTESIAN_POINT('Ctrl Pts',(-3.24428080353022,-1.,1.88117508446775));
#40974=CARTESIAN_POINT('Ctrl Pts',(-3.24480754676064,-1.,1.88156537699203));
#40975=CARTESIAN_POINT('Ctrl Pts',(-3.2462565441079,-1.,1.88242596600454));
#40976=CARTESIAN_POINT('Ctrl Pts',(-3.24935200511918,-1.,1.88407708646357));
#40977=CARTESIAN_POINT('Ctrl Pts',(-3.25408686339463,-1.,1.88646802523466));
#40978=CARTESIAN_POINT('Ctrl Pts',(-3.25999885193947,-1.,1.88934996203698));
#40979=CARTESIAN_POINT('Ctrl Pts',(-3.26677653888676,-1.,1.89255393500965));
#40980=CARTESIAN_POINT('Ctrl Pts',(-3.27407108933139,-1.,1.89589172903793));
#40981=CARTESIAN_POINT('Ctrl Pts',(-3.28154737912352,-1.,1.89918429230462));
#40982=CARTESIAN_POINT('Ctrl Pts',(-3.2889344860029,-1.,1.90228971247527));
#40983=CARTESIAN_POINT('Ctrl Pts',(-3.29608978722113,-1.,1.90513891864087));
#40984=CARTESIAN_POINT('Ctrl Pts',(-3.30300595568195,-1.,1.90773912171341));
#40985=CARTESIAN_POINT('Ctrl Pts',(-3.30975721158596,-1.,1.91014297830446));
#40986=CARTESIAN_POINT('Ctrl Pts',(-3.31646052426364,-1.,1.91242616234442));
#40987=CARTESIAN_POINT('Ctrl Pts',(-3.32323403454535,-1.,1.91466343916628));
#40988=CARTESIAN_POINT('Ctrl Pts',(-3.33014884257873,-1.,1.91690081930331));
#40989=CARTESIAN_POINT('Ctrl Pts',(-3.33721230710012,-1.,1.9191460961021));
#40990=CARTESIAN_POINT('Ctrl Pts',(-3.34439448941961,-1.,1.92138450828404));
#40991=CARTESIAN_POINT('Ctrl Pts',(-3.35164424847223,-1.,1.92358838440528));
#40992=CARTESIAN_POINT('Ctrl Pts',(-3.35890824422965,-1.,1.92572846125756));
#40993=CARTESIAN_POINT('Ctrl Pts',(-3.36615168657567,-1.,1.92778626543786));
#40994=CARTESIAN_POINT('Ctrl Pts',(-3.37336807068043,-1.,1.92975993109877));
#40995=CARTESIAN_POINT('Ctrl Pts',(-3.3805676852555,-1.,1.93165739093276));
#40996=CARTESIAN_POINT('Ctrl Pts',(-3.38777076883256,-1.,1.93349233176788));
#40997=CARTESIAN_POINT('Ctrl Pts',(-3.39499923640795,-1.,1.93527929945985));
#40998=CARTESIAN_POINT('Ctrl Pts',(-3.40226802104109,-1.,1.93702857723098));
#40999=CARTESIAN_POINT('Ctrl Pts',(-3.40957978266642,-1.,1.93874306008143));
#41000=CARTESIAN_POINT('Ctrl Pts',(-3.41692971994096,-1.,1.94042111965246));
#41001=CARTESIAN_POINT('Ctrl Pts',(-3.42430850941503,-1.,1.94205835913696));
#41002=CARTESIAN_POINT('Ctrl Pts',(-3.43170586602434,-1.,1.94364973660284));
#41003=CARTESIAN_POINT('Ctrl Pts',(-3.43911410197687,-1.,1.94519168842879));
#41004=CARTESIAN_POINT('Ctrl Pts',(-3.44653088665681,-1.,1.94668377715329));
#41005=CARTESIAN_POINT('Ctrl Pts',(-3.45395731584051,-1.,1.94812754766524));
#41006=CARTESIAN_POINT('Ctrl Pts',(-3.46139661060962,-1.,1.94952575850197));
#41007=CARTESIAN_POINT('Ctrl Pts',(-3.46885258974191,-1.,1.95088147859876));
#41008=CARTESIAN_POINT('Ctrl Pts',(-3.47632820495921,-1.,1.95219722189876));
#41009=CARTESIAN_POINT('Ctrl Pts',(-3.48382414832634,-1.,1.95347412486308));
#41010=CARTESIAN_POINT('Ctrl Pts',(-3.49133956289133,-1.,1.95471236969643));
#41011=CARTESIAN_POINT('Ctrl Pts',(-3.49887263575583,-1.,1.95591153823661));
#41012=CARTESIAN_POINT('Ctrl Pts',(-3.50642124159909,-1.,1.95707099606511));
#41013=CARTESIAN_POINT('Ctrl Pts',(-3.51398354617794,-1.,1.95819025316779));
#41014=CARTESIAN_POINT('Ctrl Pts',(-3.52155867431486,-1.,1.95926936324461));
#41015=CARTESIAN_POINT('Ctrl Pts',(-3.52914648844351,-1.,1.96030879411566));
#41016=CARTESIAN_POINT('Ctrl Pts',(-3.53674730625813,-1.,1.96130926212689));
#41017=CARTESIAN_POINT('Ctrl Pts',(-3.54436163300443,-1.,1.96227157573067));
#41018=CARTESIAN_POINT('Ctrl Pts',(-3.55198990600886,-1.,1.96319648628644));
#41019=CARTESIAN_POINT('Ctrl Pts',(-3.55963218706096,-1.,1.96408450906812));
#41020=CARTESIAN_POINT('Ctrl Pts',(-3.56728820357791,-1.,1.96493594634567));
#41021=CARTESIAN_POINT('Ctrl Pts',(-3.57495748600959,-1.,1.96575096652789));
#41022=CARTESIAN_POINT('Ctrl Pts',(-3.58263947663829,-1.,1.96652966688911));
#41023=CARTESIAN_POINT('Ctrl Pts',(-3.59033364022801,-1.,1.96727213799544));
#41024=CARTESIAN_POINT('Ctrl Pts',(-3.59803959819938,-1.,1.96797854118369));
#41025=CARTESIAN_POINT('Ctrl Pts',(-3.60575714017989,-1.,1.9686491188594));
#41026=CARTESIAN_POINT('Ctrl Pts',(-3.61348615496704,-1.,1.96928416040877));
#41027=CARTESIAN_POINT('Ctrl Pts',(-3.62122658401893,-1.,1.96988398129978));
#41028=CARTESIAN_POINT('Ctrl Pts',(-3.62897836973293,-1.,1.97044889850463));
#41029=CARTESIAN_POINT('Ctrl Pts',(-3.63674139590412,-1.,1.97097920454464));
#41030=CARTESIAN_POINT('Ctrl Pts',(-3.64451546723514,-1.,1.97147515441164));
#41031=CARTESIAN_POINT('Ctrl Pts',(-3.652300347166,-1.,1.9719369724024));
#41032=CARTESIAN_POINT('Ctrl Pts',(-3.6600957816636,-1.,1.9723648543905));
#41033=CARTESIAN_POINT('Ctrl Pts',(-3.66790152752075,-1.,1.97275897198678));
#41034=CARTESIAN_POINT('Ctrl Pts',(-3.67571738107084,-1.,1.97311947678516));
#41035=CARTESIAN_POINT('Ctrl Pts',(-3.68354319915092,-1.,1.97344650304519));
#41036=CARTESIAN_POINT('Ctrl Pts',(-3.69137888599902,-1.,1.97374016225483));
#41037=CARTESIAN_POINT('Ctrl Pts',(-3.6976552856004,-1.,1.97394846383216));
#41038=CARTESIAN_POINT('Ctrl Pts',(-3.70236698912904,-1.,1.97408973726715));
#41039=CARTESIAN_POINT('Ctrl Pts',(-3.70551008132332,-1.,1.97417727645308));
#41040=CARTESIAN_POINT('Ctrl Pts',(-3.70708211654725,-1.,1.97421938526992));
#41041=CARTESIAN_POINT('',(-3.77614523045147,-1.,1.8386753923786));
#41042=CARTESIAN_POINT('',(-3.70708211654725,-1.,1.97421938526992));
#41043=CARTESIAN_POINT('',(-3.42859860294306,-1.,1.5189508286633));
#41044=CARTESIAN_POINT('Ctrl Pts',(-3.77614523045147,-1.,1.8386753923786));
#41045=CARTESIAN_POINT('Ctrl Pts',(-3.77518714457833,-1.,1.83742834010626));
#41046=CARTESIAN_POINT('Ctrl Pts',(-3.77326886064398,-1.,1.83493697934534));
#41047=CARTESIAN_POINT('Ctrl Pts',(-3.77038509817999,-1.,1.83120816955645));
#41048=CARTESIAN_POINT('Ctrl Pts',(-3.76652740353775,-1.,1.82625289220915));
#41049=CARTESIAN_POINT('Ctrl Pts',(-3.76168412707948,-1.,1.82008629694091));
#41050=CARTESIAN_POINT('Ctrl Pts',(-3.75681965683071,-1.,1.8139472983358));
#41051=CARTESIAN_POINT('Ctrl Pts',(-3.75193395887977,-1.,1.80783603939617));
#41052=CARTESIAN_POINT('Ctrl Pts',(-3.74702700875467,-1.,1.8017527148577));
#41053=CARTESIAN_POINT('Ctrl Pts',(-3.74209880352445,-1.,1.79569757859422));
#41054=CARTESIAN_POINT('Ctrl Pts',(-3.73714934730681,-1.,1.78967092823491));
#41055=CARTESIAN_POINT('Ctrl Pts',(-3.7321786309547,-1.,1.78367308442901));
#41056=CARTESIAN_POINT('Ctrl Pts',(-3.72718661205609,-1.,1.77770437039658));
#41057=CARTESIAN_POINT('Ctrl Pts',(-3.72217319911254,-1.,1.77176509401761));
#41058=CARTESIAN_POINT('Ctrl Pts',(-3.71713822377359,-1.,1.76585552124394));
#41059=CARTESIAN_POINT('Ctrl Pts',(-3.71208146346136,-1.,1.75997588498865));
#41060=CARTESIAN_POINT('Ctrl Pts',(-3.70700269736659,-1.,1.75412641804042));
#41061=CARTESIAN_POINT('Ctrl Pts',(-3.7019017567335,-1.,1.74830738046057));
#41062=CARTESIAN_POINT('Ctrl Pts',(-3.69677856910517,-1.,1.74251908492617));
#41063=CARTESIAN_POINT('Ctrl Pts',(-3.69163322648036,-1.,1.73676193254557));
#41064=CARTESIAN_POINT('Ctrl Pts',(-3.68646597019332,-1.,1.73103640956717));
#41065=CARTESIAN_POINT('Ctrl Pts',(-3.68127704936579,-1.,1.72534302437056));
#41066=CARTESIAN_POINT('Ctrl Pts',(-3.67606660374709,-1.,1.71968225581808));
#41067=CARTESIAN_POINT('Ctrl Pts',(-3.67083454901611,-1.,1.71405450210383));
#41068=CARTESIAN_POINT('Ctrl Pts',(-3.66558043198876,-1.,1.70846001610956));
#41069=CARTESIAN_POINT('Ctrl Pts',(-3.66030338774847,-1.,1.70289888566873));
#41070=CARTESIAN_POINT('Ctrl Pts',(-3.65500246526749,-1.,1.69737117722534));
#41071=CARTESIAN_POINT('Ctrl Pts',(-3.64967689827371,-1.,1.69187705481689));
#41072=CARTESIAN_POINT('Ctrl Pts',(-3.64432638915203,-1.,1.68641690471457));
#41073=CARTESIAN_POINT('Ctrl Pts',(-3.63895140887462,-1.,1.68099146651586));
#41074=CARTESIAN_POINT('Ctrl Pts',(-3.63355343201232,-1.,1.67560193613156));
#41075=CARTESIAN_POINT('Ctrl Pts',(-3.62813422105271,-1.,1.67024966008045));
#41076=CARTESIAN_POINT('Ctrl Pts',(-3.62269517989109,-1.,1.66493585923855));
#41077=CARTESIAN_POINT('Ctrl Pts',(-3.61723666482456,-1.,1.65966133399186));
#41078=CARTESIAN_POINT('Ctrl Pts',(-3.61175734965127,-1.,1.65442619244325));
#41079=CARTESIAN_POINT('Ctrl Pts',(-3.60625346556992,-1.,1.64922952425832));
#41080=CARTESIAN_POINT('Ctrl Pts',(-3.60072028513845,-1.,1.64407004385582));
#41081=CARTESIAN_POINT('Ctrl Pts',(-3.59515368334893,-1.,1.63894676675352));
#41082=CARTESIAN_POINT('Ctrl Pts',(-3.58955176627879,-1.,1.6338597145126));
#41083=CARTESIAN_POINT('Ctrl Pts',(-3.58391625774343,-1.,1.62881051550745));
#41084=CARTESIAN_POINT('Ctrl Pts',(-3.5782545595439,-1.,1.62380329464844));
#41085=CARTESIAN_POINT('Ctrl Pts',(-3.57257679609806,-1.,1.61884340915404));
#41086=CARTESIAN_POINT('Ctrl Pts',(-3.56689200468387,-1.,1.61393581747514));
#41087=CARTESIAN_POINT('Ctrl Pts',(-3.5612043248298,-1.,1.60908344685457));
#41088=CARTESIAN_POINT('Ctrl Pts',(-3.55550985096129,-1.,1.60428584699853));
#41089=CARTESIAN_POINT('Ctrl Pts',(-3.54979148634454,-1.,1.59953698113457));
#41090=CARTESIAN_POINT('Ctrl Pts',(-3.54402458182337,-1.,1.59482766949766));
#41091=CARTESIAN_POINT('Ctrl Pts',(-3.53818616861077,-1.,1.59014958368739));
#41092=CARTESIAN_POINT('Ctrl Pts',(-3.5322637814708,-1.,1.58549906268088));
#41093=CARTESIAN_POINT('Ctrl Pts',(-3.52626275334881,-1.,1.58088027227848));
#41094=CARTESIAN_POINT('Ctrl Pts',(-3.52021847865912,-1.,1.57631049988158));
#41095=CARTESIAN_POINT('Ctrl Pts',(-3.51418598431665,-1.,1.57181569799743));
#41096=CARTESIAN_POINT('Ctrl Pts',(-3.50821771695363,-1.,1.56742097575012));
#41097=CARTESIAN_POINT('Ctrl Pts',(-3.50234321621578,-1.,1.56314187758675));
#41098=CARTESIAN_POINT('Ctrl Pts',(-3.49655185179655,-1.,1.55897703097874));
#41099=CARTESIAN_POINT('Ctrl Pts',(-3.4907646087742,-1.,1.55489595901116));
#41100=CARTESIAN_POINT('Ctrl Pts',(-3.48485155928567,-1.,1.55084702970452));
#41101=CARTESIAN_POINT('Ctrl Pts',(-3.47868272898751,-1.,1.54678009290276));
#41102=CARTESIAN_POINT('Ctrl Pts',(-3.47217189224653,-1.,1.54266605398187));
#41103=CARTESIAN_POINT('Ctrl Pts',(-3.46531752207153,-1.,1.53851507915502));
#41104=CARTESIAN_POINT('Ctrl Pts',(-3.45825932955032,-1.,1.53440195378792));
#41105=CARTESIAN_POINT('Ctrl Pts',(-3.45127136828305,-1.,1.53046244461635));
#41106=CARTESIAN_POINT('Ctrl Pts',(-3.44469547526647,-1.,1.52686242875556));
#41107=CARTESIAN_POINT('Ctrl Pts',(-3.4388889597401,-1.,1.5237734895035));
#41108=CARTESIAN_POINT('Ctrl Pts',(-3.43417156977893,-1.,1.52134826724292));
#41109=CARTESIAN_POINT('Ctrl Pts',(-3.43101631893414,-1.,1.5198144909338));
#41110=CARTESIAN_POINT('Ctrl Pts',(-3.42946838852587,-1.,1.51914806898491));
#41111=CARTESIAN_POINT('Ctrl Pts',(-3.42884302333841,-1.,1.5189513329503));
#41112=CARTESIAN_POINT('Ctrl Pts',(-3.42864616361875,-1.,1.51893924967331));
#41113=CARTESIAN_POINT('Ctrl Pts',(-3.42859860294306,-1.,1.5189508286633));
#41114=CARTESIAN_POINT('',(-3.49844575334386,-1.,1.35032489087269));
#41115=CARTESIAN_POINT('Origin',(0.,-1.,0.));
#41116=CARTESIAN_POINT('',(-3.97027773754922,-1.,1.36999806084572));
#41117=CARTESIAN_POINT('Ctrl Pts',(-3.49844575334386,-1.,1.35032489087269));
#41118=CARTESIAN_POINT('Ctrl Pts',(-3.49847119623841,-1.,1.35036670893102));
#41119=CARTESIAN_POINT('Ctrl Pts',(-3.49861894124915,-1.,1.35049736560633));
#41120=CARTESIAN_POINT('Ctrl Pts',(-3.49920025459856,-1.,1.35080045218652));
#41121=CARTESIAN_POINT('Ctrl Pts',(-3.5007660381658,-1.,1.35142377279535));
#41122=CARTESIAN_POINT('Ctrl Pts',(-3.50408168106113,-1.,1.3525703284343));
#41123=CARTESIAN_POINT('Ctrl Pts',(-3.50913227060177,-1.,1.35419113576022));
#41124=CARTESIAN_POINT('Ctrl Pts',(-3.51542230699919,-1.,1.35611275237288));
#41125=CARTESIAN_POINT('Ctrl Pts',(-3.52261776117121,-1.,1.35821701528975));
#41126=CARTESIAN_POINT('Ctrl Pts',(-3.53034464961849,-1.,1.36037259643827));
#41127=CARTESIAN_POINT('Ctrl Pts',(-3.53824396425032,-1.,1.36245507339334));
#41128=CARTESIAN_POINT('Ctrl Pts',(-3.54602591832893,-1.,1.36436666257567));
#41129=CARTESIAN_POINT('Ctrl Pts',(-3.55353883995793,-1.,1.36606145456711));
#41130=CARTESIAN_POINT('Ctrl Pts',(-3.56077662028492,-1.,1.36754771771174));
#41131=CARTESIAN_POINT('Ctrl Pts',(-3.56782080304554,-1.,1.36886584973349));
#41132=CARTESIAN_POINT('Ctrl Pts',(-3.57479875549453,-1.,1.37007229485646));
#41133=CARTESIAN_POINT('Ctrl Pts',(-3.58183885982745,-1.,1.37122241663073));
#41134=CARTESIAN_POINT('Ctrl Pts',(-3.5890185384643,-1.,1.37235053661));
#41135=CARTESIAN_POINT('Ctrl Pts',(-3.59634627869117,-1.,1.37346320103184));
#41136=CARTESIAN_POINT('Ctrl Pts',(-3.60379020124038,-1.,1.37455051379642));
#41137=CARTESIAN_POINT('Ctrl Pts',(-3.61129546591082,-1.,1.37559314436641));
#41138=CARTESIAN_POINT('Ctrl Pts',(-3.61880481160408,-1.,1.37657053403102));
#41139=CARTESIAN_POINT('Ctrl Pts',(-3.62628098665112,-1.,1.37746987919868));
#41140=CARTESIAN_POINT('Ctrl Pts',(-3.63371727442448,-1.,1.37829035457324));
#41141=CARTESIAN_POINT('Ctrl Pts',(-3.64112507791112,-1.,1.37903818567347));
#41142=CARTESIAN_POINT('Ctrl Pts',(-3.64852652756444,-1.,1.37972372481598));
#41143=CARTESIAN_POINT('Ctrl Pts',(-3.65594554404396,-1.,1.38035791051215));
#41144=CARTESIAN_POINT('Ctrl Pts',(-3.66339848520874,-1.,1.38094856333558));
#41145=CARTESIAN_POINT('Ctrl Pts',(-3.67088843112282,-1.,1.38149812653876));
#41146=CARTESIAN_POINT('Ctrl Pts',(-3.6784103848243,-1.,1.38200574290626));
#41147=CARTESIAN_POINT('Ctrl Pts',(-3.68595444983844,-1.,1.38246852827185));
#41148=CARTESIAN_POINT('Ctrl Pts',(-3.69350967899523,-1.,1.38288311171649));
#41149=CARTESIAN_POINT('Ctrl Pts',(-3.70106792167894,-1.,1.38324717612862));
#41150=CARTESIAN_POINT('Ctrl Pts',(-3.70862680753343,-1.,1.38356065402122));
#41151=CARTESIAN_POINT('Ctrl Pts',(-3.7161876605181,-1.,1.38382489984585));
#41152=CARTESIAN_POINT('Ctrl Pts',(-3.72375409358805,-1.,1.3840421342895));
#41153=CARTESIAN_POINT('Ctrl Pts',(-3.73133035859283,-1.,1.38421479111531));
#41154=CARTESIAN_POINT('Ctrl Pts',(-3.73891976418099,-1.,1.38434489156456));
#41155=CARTESIAN_POINT('Ctrl Pts',(-3.7465231716786,-1.,1.38443344984389));
#41156=CARTESIAN_POINT('Ctrl Pts',(-3.75413976318727,-1.,1.38448077997155));
#41157=CARTESIAN_POINT('Ctrl Pts',(-3.76176768271347,-1.,1.38448675253343));
#41158=CARTESIAN_POINT('Ctrl Pts',(-3.76940473185775,-1.,1.38445107339517));
#41159=CARTESIAN_POINT('Ctrl Pts',(-3.77704902230441,-1.,1.38437354551435));
#41160=CARTESIAN_POINT('Ctrl Pts',(-3.78469969805134,-1.,1.38425435883773));
#41161=CARTESIAN_POINT('Ctrl Pts',(-3.79235669640907,-1.,1.38409399694588));
#41162=CARTESIAN_POINT('Ctrl Pts',(-3.80002044322169,-1.,1.38389311766701));
#41163=CARTESIAN_POINT('Ctrl Pts',(-3.80769156398429,-1.,1.38365244046226));
#41164=CARTESIAN_POINT('Ctrl Pts',(-3.81537060817765,-1.,1.38337263902766));
#41165=CARTESIAN_POINT('Ctrl Pts',(-3.82305771743715,-1.,1.38305421262724));
#41166=CARTESIAN_POINT('Ctrl Pts',(-3.83075266982138,-1.,1.38269750245086));
#41167=CARTESIAN_POINT('Ctrl Pts',(-3.83845502790609,-1.,1.38230274828774));
#41168=CARTESIAN_POINT('Ctrl Pts',(-3.84616425605705,-1.,1.38187013346089));
#41169=CARTESIAN_POINT('Ctrl Pts',(-3.85387983979557,-1.,1.38139983115075));
#41170=CARTESIAN_POINT('Ctrl Pts',(-3.86160143044187,-1.,1.38089205993067));
#41171=CARTESIAN_POINT('Ctrl Pts',(-3.86932885813403,-1.,1.38034709213129));
#41172=CARTESIAN_POINT('Ctrl Pts',(-3.87706205830865,-1.,1.37976523097187));
#41173=CARTESIAN_POINT('Ctrl Pts',(-3.88480102249461,-1.,1.37914679719446));
#41174=CARTESIAN_POINT('Ctrl Pts',(-3.89254574338385,-1.,1.37849211287981));
#41175=CARTESIAN_POINT('Ctrl Pts',(-3.90029615196255,-1.,1.3778014851263));
#41176=CARTESIAN_POINT('Ctrl Pts',(-3.90805209522729,-1.,1.3770751963376));
#41177=CARTESIAN_POINT('Ctrl Pts',(-3.91581337461825,-1.,1.37631350505516));
#41178=CARTESIAN_POINT('Ctrl Pts',(-3.92357976987132,-1.,1.37551664448057));
#41179=CARTESIAN_POINT('Ctrl Pts',(-3.93135106761941,-1.,1.37468482215784));
#41180=CARTESIAN_POINT('Ctrl Pts',(-3.93912709041791,-1.,1.37381821967499));
#41181=CARTESIAN_POINT('Ctrl Pts',(-3.94690771786926,-1.,1.37291699203423));
#41182=CARTESIAN_POINT('Ctrl Pts',(-3.95469287283105,-1.,1.37198126433139));
#41183=CARTESIAN_POINT('Ctrl Pts',(-3.96092458508407,-1.,1.37120515615663));
#41184=CARTESIAN_POINT('Ctrl Pts',(-3.96560037975788,-1.,1.37060761746027));
#41185=CARTESIAN_POINT('Ctrl Pts',(-3.9687184694173,-1.,1.37020239094758));
#41186=CARTESIAN_POINT('Ctrl Pts',(-3.97027773754922,-1.,1.36999806084572));
#41187=CARTESIAN_POINT('',(-4.01728681790024,-1.,1.22531898815164));
#41188=CARTESIAN_POINT('',(-3.97027773754922,-1.,1.36999806084572));
#41189=CARTESIAN_POINT('',(-3.62400312501199,-1.,0.963899035118985));
#41190=CARTESIAN_POINT('Ctrl Pts',(-4.01728681790024,-1.,1.22531898815164));
#41191=CARTESIAN_POINT('Ctrl Pts',(-4.01614544569895,-1.,1.22423716681317));
#41192=CARTESIAN_POINT('Ctrl Pts',(-4.01386104433519,-1.,1.22207656455845));
#41193=CARTESIAN_POINT('Ctrl Pts',(-4.01042947140789,-1.,1.21884478244403));
#41194=CARTESIAN_POINT('Ctrl Pts',(-4.00584409522722,-1.,1.21455398918133));
#41195=CARTESIAN_POINT('Ctrl Pts',(-4.00009577950721,-1.,1.20922097029551));
#41196=CARTESIAN_POINT('Ctrl Pts',(-3.99433084799666,-1.,1.20391852375139));
#41197=CARTESIAN_POINT('Ctrl Pts',(-3.98854928957189,-1.,1.19864679609566));
#41198=CARTESIAN_POINT('Ctrl Pts',(-3.98275111052561,-1.,1.19340598349475));
#41199=CARTESIAN_POINT('Ctrl Pts',(-3.97693634767754,-1.,1.18819633715539));
#41200=CARTESIAN_POINT('Ctrl Pts',(-3.97110505165415,-1.,1.18301815039831));
#41201=CARTESIAN_POINT('Ctrl Pts',(-3.96525726358159,-1.,1.17787174135592));
#41202=CARTESIAN_POINT('Ctrl Pts',(-3.95939299213276,-1.,1.17275743590361));
#41203=CARTESIAN_POINT('Ctrl Pts',(-3.95351219509876,-1.,1.16767555244438));
#41204=CARTESIAN_POINT('Ctrl Pts',(-3.94761474780583,-1.,1.16262637999157));
#41205=CARTESIAN_POINT('Ctrl Pts',(-3.94170046685203,-1.,1.15761018340956));
#41206=CARTESIAN_POINT('Ctrl Pts',(-3.9357691705628,-1.,1.1526272271632));
#41207=CARTESIAN_POINT('Ctrl Pts',(-3.92982073294257,-1.,1.14767779451123));
#41208=CARTESIAN_POINT('Ctrl Pts',(-3.92385513133997,-1.,1.14276220561593));
#41209=CARTESIAN_POINT('Ctrl Pts',(-3.91787251936827,-1.,1.13788084225554));
#41210=CARTESIAN_POINT('Ctrl Pts',(-3.91187321145649,-1.,1.13303414693896));
#41211=CARTESIAN_POINT('Ctrl Pts',(-3.90585753318737,-1.,1.12822258281553));
#41212=CARTESIAN_POINT('Ctrl Pts',(-3.89982569750025,-1.,1.12344660099043));
#41213=CARTESIAN_POINT('Ctrl Pts',(-3.89377768340344,-1.,1.11870660794603));
#41214=CARTESIAN_POINT('Ctrl Pts',(-3.88771308285171,-1.,1.11400292434429));
#41215=CARTESIAN_POINT('Ctrl Pts',(-3.88163105531724,-1.,1.10933577224008));
#41216=CARTESIAN_POINT('Ctrl Pts',(-3.87553067187514,-1.,1.10470536603287));
#41217=CARTESIAN_POINT('Ctrl Pts',(-3.86941120134849,-1.,1.10011198761195));
#41218=CARTESIAN_POINT('Ctrl Pts',(-3.86327241021247,-1.,1.09555606505013));
#41219=CARTESIAN_POINT('Ctrl Pts',(-3.85711487933931,-1.,1.09103825516294));
#41220=CARTESIAN_POINT('Ctrl Pts',(-3.85094025222713,-1.,1.08655950846384));
#41221=CARTESIAN_POINT('Ctrl Pts',(-3.8447504803063,-1.,1.08212087917991));
#41222=CARTESIAN_POINT('Ctrl Pts',(-3.83854714117491,-1.,1.07772335353858));
#41223=CARTESIAN_POINT('Ctrl Pts',(-3.83233071195144,-1.,1.07336766633459));
#41224=CARTESIAN_POINT('Ctrl Pts',(-3.82609989967276,-1.,1.06905413180359));
#41225=CARTESIAN_POINT('Ctrl Pts',(-3.81985083953012,-1.,1.0647824403893));
#41226=CARTESIAN_POINT('Ctrl Pts',(-3.8135786611749,-1.,1.06055206187299));
#41227=CARTESIAN_POINT('Ctrl Pts',(-3.80727913637791,-1.,1.05636266918644));
#41228=CARTESIAN_POINT('Ctrl Pts',(-3.80095039790681,-1.,1.05221457990016));
#41229=CARTESIAN_POINT('Ctrl Pts',(-3.79459440308786,-1.,1.04810913267639));
#41230=CARTESIAN_POINT('Ctrl Pts',(-3.78821910787179,-1.,1.04404924374422));
#41231=CARTESIAN_POINT('Ctrl Pts',(-3.7818353500817,-1.,1.04003862055798));
#41232=CARTESIAN_POINT('Ctrl Pts',(-3.77545283140427,-1.,1.03608074678008));
#41233=CARTESIAN_POINT('Ctrl Pts',(-3.76907609832516,-1.,1.03217786604919));
#41234=CARTESIAN_POINT('Ctrl Pts',(-3.76270122291245,-1.,1.02833014458184));
#41235=CARTESIAN_POINT('Ctrl Pts',(-3.75631037456224,-1.,1.02453429444668));
#41236=CARTESIAN_POINT('Ctrl Pts',(-3.74987777155873,-1.,1.02078510487439));
#41237=CARTESIAN_POINT('Ctrl Pts',(-3.74337942504993,-1.,1.01707794311088));
#41238=CARTESIAN_POINT('Ctrl Pts',(-3.73680245055747,-1.,1.01341114319906));
#41239=CARTESIAN_POINT('Ctrl Pts',(-3.73015276704407,-1.,1.00978798539491));
#41240=CARTESIAN_POINT('Ctrl Pts',(-3.72346803750544,-1.,1.00622000735696));
#41241=CARTESIAN_POINT('Ctrl Pts',(-3.71680667125047,-1.,1.00272423396802));
#41242=CARTESIAN_POINT('Ctrl Pts',(-3.7102243971387,-1.,0.999317260756344));
#41243=CARTESIAN_POINT('Ctrl Pts',(-3.70375282282107,-1.,0.996009819772431));
#41244=CARTESIAN_POINT('Ctrl Pts',(-3.69738123415696,-1.,0.992802218332103));
#41245=CARTESIAN_POINT('Ctrl Pts',(-3.69102682138955,-1.,0.989676715398858));
#41246=CARTESIAN_POINT('Ctrl Pts',(-3.6845531792623,-1.,0.986602639864285));
#41247=CARTESIAN_POINT('Ctrl Pts',(-3.67782408841876,-1.,0.983550791470864));
#41248=CARTESIAN_POINT('Ctrl Pts',(-3.67074983340444,-1.,0.980505922458494));
#41249=CARTESIAN_POINT('Ctrl Pts',(-3.66333049637403,-1.,0.977478312751416));
#41250=CARTESIAN_POINT('Ctrl Pts',(-3.6557157673487,-1.,0.974519971354138));
#41251=CARTESIAN_POINT('Ctrl Pts',(-3.64819756447072,-1.,0.971722122060277));
#41252=CARTESIAN_POINT('Ctrl Pts',(-3.64113946505393,-1.,0.969195124674829));
#41253=CARTESIAN_POINT('Ctrl Pts',(-3.6349212208096,-1.,0.967052554540877));
#41254=CARTESIAN_POINT('Ctrl Pts',(-3.62988252139998,-1.,0.965395153165716));
#41255=CARTESIAN_POINT('Ctrl Pts',(-3.62652618145252,-1.,0.964373850166081));
#41256=CARTESIAN_POINT('Ctrl Pts',(-3.62489305727516,-1.,0.963957782642589));
#41257=CARTESIAN_POINT('Ctrl Pts',(-3.62424461507455,-1.,0.963861297423579));
#41258=CARTESIAN_POINT('Ctrl Pts',(-3.62404828878375,-1.,0.963880158556713));
#41259=CARTESIAN_POINT('Ctrl Pts',(-3.62400312501199,-1.,0.963899035118985));
#41260=CARTESIAN_POINT('',(-3.66661143271648,-1.,0.786422660833743));
#41261=CARTESIAN_POINT('Origin',(0.,-1.,0.));
#41262=CARTESIAN_POINT('',(-4.13571194405636,-1.,0.732042837400619));
#41263=CARTESIAN_POINT('Ctrl Pts',(-3.66661143271648,-1.,0.786422660833743));
#41264=CARTESIAN_POINT('Ctrl Pts',(-3.66664310415236,-1.,0.786459983896781));
#41265=CARTESIAN_POINT('Ctrl Pts',(-3.66680946938396,-1.,0.78656591955989));
#41266=CARTESIAN_POINT('Ctrl Pts',(-3.66743103898844,-1.,0.786774337198499));
#41267=CARTESIAN_POINT('Ctrl Pts',(-3.66907505398769,-1.,0.787145041181588));
#41268=CARTESIAN_POINT('Ctrl Pts',(-3.672529236635,-1.,0.787758799995426));
#41269=CARTESIAN_POINT('Ctrl Pts',(-3.67777119516438,-1.,0.788569566220662));
#41270=CARTESIAN_POINT('Ctrl Pts',(-3.68428439784285,-1.,0.789483546065158));
#41271=CARTESIAN_POINT('Ctrl Pts',(-3.69172044327754,-1.,0.79043628498958));
#41272=CARTESIAN_POINT('Ctrl Pts',(-3.69968940808982,-1.,0.791356575696509));
#41273=CARTESIAN_POINT('Ctrl Pts',(-3.70781724021879,-1.,0.792177688845967));
#41274=CARTESIAN_POINT('Ctrl Pts',(-3.7158024239604,-1.,0.792848377370115));
#41275=CARTESIAN_POINT('Ctrl Pts',(-3.7234879729357,-1.,0.79334702378387));
#41276=CARTESIAN_POINT('Ctrl Pts',(-3.7308691469564,-1.,0.793682750269347));
#41277=CARTESIAN_POINT('Ctrl Pts',(-3.73803280541576,-1.,0.79388270093679));
#41278=CARTESIAN_POINT('Ctrl Pts',(-3.74511357728827,-1.,0.79398270045988));
#41279=CARTESIAN_POINT('Ctrl Pts',(-3.75224692493895,-1.,0.79401734737144));
#41280=CARTESIAN_POINT('Ctrl Pts',(-3.75951468666325,-1.,0.794008429135047));
#41281=CARTESIAN_POINT('Ctrl Pts',(-3.76692626931184,-1.,0.793961083689141));
#41282=CARTESIAN_POINT('Ctrl Pts',(-3.77444863801264,-1.,0.793870523787515));
#41283=CARTESIAN_POINT('Ctrl Pts',(-3.78202460377617,-1.,0.793726235781339));
#41284=CARTESIAN_POINT('Ctrl Pts',(-3.78959439439222,-1.,0.793516871680966));
#41285=CARTESIAN_POINT('Ctrl Pts',(-3.79711921389862,-1.,0.7932356129732));
#41286=CARTESIAN_POINT('Ctrl Pts',(-3.80459229925598,-1.,0.792882695234693));
#41287=CARTESIAN_POINT('Ctrl Pts',(-3.81202588694726,-1.,0.792462483517568));
#41288=CARTESIAN_POINT('Ctrl Pts',(-3.81944345442237,-1.,0.791981740718606));
#41289=CARTESIAN_POINT('Ctrl Pts',(-3.82687033899799,-1.,0.791447528662381));
#41290=CARTESIAN_POINT('Ctrl Pts',(-3.83432392054804,-1.,0.79086501270534));
#41291=CARTESIAN_POINT('Ctrl Pts',(-3.84180762342476,-1.,0.790236124191289));
#41292=CARTESIAN_POINT('Ctrl Pts',(-3.8493163780891,-1.,0.789560798155618));
#41293=CARTESIAN_POINT('Ctrl Pts',(-3.85683995872536,-1.,0.788837734090688));
#41294=CARTESIAN_POINT('Ctrl Pts',(-3.86436702561342,-1.,0.788065315093771));
#41295=CARTESIAN_POINT('Ctrl Pts',(-3.87188916600905,-1.,0.78724252761798));
#41296=CARTESIAN_POINT('Ctrl Pts',(-3.87940402818186,-1.,0.786369675812592));
#41297=CARTESIAN_POINT('Ctrl Pts',(-3.88691313167399,-1.,0.785447890340723));
#41298=CARTESIAN_POINT('Ctrl Pts',(-3.89442039235105,-1.,0.784478799358335));
#41299=CARTESIAN_POINT('Ctrl Pts',(-3.90193039043971,-1.,0.783464141529082));
#41300=CARTESIAN_POINT('Ctrl Pts',(-3.90944671004536,-1.,0.782405395622758));
#41301=CARTESIAN_POINT('Ctrl Pts',(-3.9169703605466,-1.,0.781303428618343));
#41302=CARTESIAN_POINT('Ctrl Pts',(-3.92450058323799,-1.,0.780158678615506));
#41303=CARTESIAN_POINT('Ctrl Pts',(-3.93203552473153,-1.,0.778971308134786));
#41304=CARTESIAN_POINT('Ctrl Pts',(-3.93957296768098,-1.,0.777741370568549));
#41305=CARTESIAN_POINT('Ctrl Pts',(-3.94711101619471,-1.,0.77646896669796));
#41306=CARTESIAN_POINT('Ctrl Pts',(-3.95464885452364,-1.,0.775154418039441));
#41307=CARTESIAN_POINT('Ctrl Pts',(-3.96218649639876,-1.,0.773798212026682));
#41308=CARTESIAN_POINT('Ctrl Pts',(-3.96972446532832,-1.,0.772400931772238));
#41309=CARTESIAN_POINT('Ctrl Pts',(-3.97726349165507,-1.,0.770963190030503));
#41310=CARTESIAN_POINT('Ctrl Pts',(-3.98480422348403,-1.,0.769485566245459));
#41311=CARTESIAN_POINT('Ctrl Pts',(-3.99234687880892,-1.,0.767968531377708));
#41312=CARTESIAN_POINT('Ctrl Pts',(-3.99989129179464,-1.,0.766412457135785));
#41313=CARTESIAN_POINT('Ctrl Pts',(-4.00743706791366,-1.,0.764817648784946));
#41314=CARTESIAN_POINT('Ctrl Pts',(-4.01498370680434,-1.,0.763184371182826));
#41315=CARTESIAN_POINT('Ctrl Pts',(-4.02253072741347,-1.,0.761512875859941));
#41316=CARTESIAN_POINT('Ctrl Pts',(-4.0300778195465,-1.,0.759803433244166));
#41317=CARTESIAN_POINT('Ctrl Pts',(-4.03762485803468,-1.,0.758056338885553));
#41318=CARTESIAN_POINT('Ctrl Pts',(-4.04517182654344,-1.,0.756271902370186));
#41319=CARTESIAN_POINT('Ctrl Pts',(-4.05271876688106,-1.,0.754450441816411));
#41320=CARTESIAN_POINT('Ctrl Pts',(-4.06026572221399,-1.,0.752592276482869));
#41321=CARTESIAN_POINT('Ctrl Pts',(-4.06781267241886,-1.,0.750697720483175));
#41322=CARTESIAN_POINT('Ctrl Pts',(-4.07535951055363,-1.,0.748767076679177));
#41323=CARTESIAN_POINT('Ctrl Pts',(-4.08290608094789,-1.,0.746800631490821));
#41324=CARTESIAN_POINT('Ctrl Pts',(-4.09045220253011,-1.,0.744798649705514));
#41325=CARTESIAN_POINT('Ctrl Pts',(-4.09799769702712,-1.,0.742761369690017));
#41326=CARTESIAN_POINT('Ctrl Pts',(-4.1055424175856,-1.,0.740688998555151));
#41327=CARTESIAN_POINT('Ctrl Pts',(-4.11308626953795,-1.,0.738581708229118));
#41328=CARTESIAN_POINT('Ctrl Pts',(-4.12062919626082,-1.,0.736439634335347));
#41329=CARTESIAN_POINT('Ctrl Pts',(-4.12666277572794,-1.,0.734698226767512));
#41330=CARTESIAN_POINT('Ctrl Pts',(-4.13118752796397,-1.,0.733376589325634));
#41331=CARTESIAN_POINT('Ctrl Pts',(-4.13420383737278,-1.,0.732488575135926));
#41332=CARTESIAN_POINT('Ctrl Pts',(-4.13571194405636,-1.,0.732042837400619));
#41333=CARTESIAN_POINT('',(-4.15950947128175,-1.,0.581791163835814));
#41334=CARTESIAN_POINT('',(-4.13571194405636,-1.,0.732042837400619));
#41335=CARTESIAN_POINT('',(-3.73017266276632,-1.,0.385112848332549));
#41336=CARTESIAN_POINT('Ctrl Pts',(-4.15950947128175,-1.,0.581791163835814));
#41337=CARTESIAN_POINT('Ctrl Pts',(-4.15821291712391,-1.,0.580901211462913));
#41338=CARTESIAN_POINT('Ctrl Pts',(-4.15561864787379,-1.,0.579124568912543));
#41339=CARTESIAN_POINT('Ctrl Pts',(-4.1517237611974,-1.,0.576469391673916));
#41340=CARTESIAN_POINT('Ctrl Pts',(-4.14652361065787,-1.,0.572948736066276));
#41341=CARTESIAN_POINT('Ctrl Pts',(-4.14001179828669,-1.,0.568580610187116));
#41342=CARTESIAN_POINT('Ctrl Pts',(-4.13348835726086,-1.,0.564245279535705));
#41343=CARTESIAN_POINT('Ctrl Pts',(-4.12695329951859,-1.,0.559942890594628));
#41344=CARTESIAN_POINT('Ctrl Pts',(-4.1204066619623,-1.,0.555673636130778));
#41345=CARTESIAN_POINT('Ctrl Pts',(-4.11384852025578,-1.,0.551437758498246));
#41346=CARTESIAN_POINT('Ctrl Pts',(-4.1072789702877,-1.,0.547235539486759));
#41347=CARTESIAN_POINT('Ctrl Pts',(-4.10069810244473,-1.,0.543067286878457));
#41348=CARTESIAN_POINT('Ctrl Pts',(-4.09410597627116,-1.,0.53893332117992));
#41349=CARTESIAN_POINT('Ctrl Pts',(-4.08750259988693,-1.,0.534833963476999));
#41350=CARTESIAN_POINT('Ctrl Pts',(-4.08088789536488,-1.,0.530769518728075));
#41351=CARTESIAN_POINT('Ctrl Pts',(-4.07426172299496,-1.,0.526740277226999));
#41352=CARTESIAN_POINT('Ctrl Pts',(-4.06762394471075,-1.,0.522746528602767));
#41353=CARTESIAN_POINT('Ctrl Pts',(-4.06097448037934,-1.,0.518788572336809));
#41354=CARTESIAN_POINT('Ctrl Pts',(-4.05431335771261,-1.,0.514866728193104));
#41355=CARTESIAN_POINT('Ctrl Pts',(-4.04764078815591,-1.,0.510981349219173));
#41356=CARTESIAN_POINT('Ctrl Pts',(-4.04095715149074,-1.,0.507132823288361));
#41357=CARTESIAN_POINT('Ctrl Pts',(-4.0342628417439,-1.,0.503321556915513));
#41358=CARTESIAN_POINT('Ctrl Pts',(-4.0275581398015,-1.,0.499547962340889));
#41359=CARTESIAN_POINT('Ctrl Pts',(-4.02084308851813,-1.,0.495812444326223));
#41360=CARTESIAN_POINT('Ctrl Pts',(-4.01411733503486,-1.,0.49211538341793));
#41361=CARTESIAN_POINT('Ctrl Pts',(-4.0073800839092,-1.,0.48845713042453));
#41362=CARTESIAN_POINT('Ctrl Pts',(-4.00063045119234,-1.,0.484838042421754));
#41363=CARTESIAN_POINT('Ctrl Pts',(-3.99386775880655,-1.,0.481258512209638));
#41364=CARTESIAN_POINT('Ctrl Pts',(-3.98709184306743,-1.,0.477718999122033));
#41365=CARTESIAN_POINT('Ctrl Pts',(-3.9803033804443,-1.,0.474220061019542));
#41366=CARTESIAN_POINT('Ctrl Pts',(-3.97350414289415,-1.,0.470762379613477));
#41367=CARTESIAN_POINT('Ctrl Pts',(-3.96669622273946,-1.,0.467346690880671));
#41368=CARTESIAN_POINT('Ctrl Pts',(-3.95988133243543,-1.,0.463973722115744));
#41369=CARTESIAN_POINT('Ctrl Pts',(-3.95306005817363,-1.,0.460644124429119));
#41370=CARTESIAN_POINT('Ctrl Pts',(-3.94623117206675,-1.,0.457358410451674));
#41371=CARTESIAN_POINT('Ctrl Pts',(-3.93939080846298,-1.,0.454116879027576));
#41372=CARTESIAN_POINT('Ctrl Pts',(-3.93253407403128,-1.,0.450919768356347));
#41373=CARTESIAN_POINT('Ctrl Pts',(-3.92565674143424,-1.,0.447767416837296));
#41374=CARTESIAN_POINT('Ctrl Pts',(-3.91875701610721,-1.,0.444660430230592));
#41375=CARTESIAN_POINT('Ctrl Pts',(-3.91183704069146,-1.,0.441599824524047));
#41376=CARTESIAN_POINT('Ctrl Pts',(-3.90490512938546,-1.,0.438587235458233));
#41377=CARTESIAN_POINT('Ctrl Pts',(-3.8979725665544,-1.,0.435624629433505));
#41378=CARTESIAN_POINT('Ctrl Pts',(-3.89104947940592,-1.,0.432713929544439));
#41379=CARTESIAN_POINT('Ctrl Pts',(-3.88414070943334,-1.,0.429856640579733));
#41380=CARTESIAN_POINT('Ctrl Pts',(-3.87724240306609,-1.,0.427053541173469));
#41381=CARTESIAN_POINT('Ctrl Pts',(-3.87033643487882,-1.,0.424304173195142));
#41382=CARTESIAN_POINT('Ctrl Pts',(-3.86339652542749,-1.,0.421607423177575));
#41383=CARTESIAN_POINT('Ctrl Pts',(-3.85639825648031,-1.,0.418962468086809));
#41384=CARTESIAN_POINT('Ctrl Pts',(-3.8493286415751,-1.,0.41636967805292));
#41385=CARTESIAN_POINT('Ctrl Pts',(-3.84219403994742,-1.,0.413831367016726));
#41386=CARTESIAN_POINT('Ctrl Pts',(-3.83503345578645,-1.,0.411353038798459));
#41387=CARTESIAN_POINT('Ctrl Pts',(-3.82790724256397,-1.,0.408942371447377));
#41388=CARTESIAN_POINT('Ctrl Pts',(-3.82087303913741,-1.,0.406607038258906));
#41389=CARTESIAN_POINT('Ctrl Pts',(-3.81396374287762,-1.,0.404352694628236));
#41390=CARTESIAN_POINT('Ctrl Pts',(-3.80716881962763,-1.,0.402181320148474));
#41391=CARTESIAN_POINT('Ctrl Pts',(-3.80040370384659,-1.,0.400088346504726));
#41392=CARTESIAN_POINT('Ctrl Pts',(-3.79352887163457,-1.,0.398064818684158));
#41393=CARTESIAN_POINT('Ctrl Pts',(-3.78640521279479,-1.,0.396103205335028));
#41394=CARTESIAN_POINT('Ctrl Pts',(-3.77894173114368,-1.,0.394202481011595));
#41395=CARTESIAN_POINT('Ctrl Pts',(-3.77114011595892,-1.,0.392372786223346));
#41396=CARTESIAN_POINT('Ctrl Pts',(-3.76315635032993,-1.,0.390642072979259));
#41397=CARTESIAN_POINT('Ctrl Pts',(-3.75529302894757,-1.,0.389054775898251));
#41398=CARTESIAN_POINT('Ctrl Pts',(-3.74792651696269,-1.,0.387663020050396));
#41399=CARTESIAN_POINT('Ctrl Pts',(-3.74144965781088,-1.,0.386519576222035));
#41400=CARTESIAN_POINT('Ctrl Pts',(-3.73621371845475,-1.,0.385670806454744));
#41401=CARTESIAN_POINT('Ctrl Pts',(-3.73273893363318,-1.,0.385187124633964));
#41402=CARTESIAN_POINT('Ctrl Pts',(-3.73106082862399,-1.,0.385031656499141));
#41403=CARTESIAN_POINT('Ctrl Pts',(-3.73040527620929,-1.,0.385037797882046));
#41404=CARTESIAN_POINT('Ctrl Pts',(-3.73021431755218,-1.,0.385087139001609));
#41405=CARTESIAN_POINT('Ctrl Pts',(-3.73017266276632,-1.,0.385112848332549));
#41406=CARTESIAN_POINT('',(-3.74449296982994,-1.,0.203156094897895));
#41407=CARTESIAN_POINT('Origin',(0.,-1.,0.));
#41408=CARTESIAN_POINT('',(-4.19931119685982,-1.,0.0760622897878236));
#41409=CARTESIAN_POINT('Ctrl Pts',(-3.74449296982994,-1.,0.203156094897895));
#41410=CARTESIAN_POINT('Ctrl Pts',(-3.74453008995129,-1.,0.203188003947965));
#41411=CARTESIAN_POINT('Ctrl Pts',(-3.74471097893961,-1.,0.203266610111264));
#41412=CARTESIAN_POINT('Ctrl Pts',(-3.74535749969262,-1.,0.203375226874331));
#41413=CARTESIAN_POINT('Ctrl Pts',(-3.74703926501843,-1.,0.203484186269314));
#41414=CARTESIAN_POINT('Ctrl Pts',(-3.75054693397716,-1.,0.203550035479097));
#41415=CARTESIAN_POINT('Ctrl Pts',(-3.75585118707924,-1.,0.203530796848403));
#41416=CARTESIAN_POINT('Ctrl Pts',(-3.76242717937273,-1.,0.203414634707646));
#41417=CARTESIAN_POINT('Ctrl Pts',(-3.76992071595267,-1.,0.203192390045337));
#41418=CARTESIAN_POINT('Ctrl Pts',(-3.77793553476879,-1.,0.202854729699196));
#41419=CARTESIAN_POINT('Ctrl Pts',(-3.78609175019317,-1.,0.202394260512193));
#41420=CARTESIAN_POINT('Ctrl Pts',(-3.79408354187274,-1.,0.201807533800799));
#41421=CARTESIAN_POINT('Ctrl Pts',(-3.80175247447171,-1.,0.201097756307252));
#41422=CARTESIAN_POINT('Ctrl Pts',(-3.80909529318501,-1.,0.20027467943329));
#41423=CARTESIAN_POINT('Ctrl Pts',(-3.81620203429702,-1.,0.199351525297396));
#41424=CARTESIAN_POINT('Ctrl Pts',(-3.82321127348981,-1.,0.19834261690047));
#41425=CARTESIAN_POINT('Ctrl Pts',(-3.83026221776488,-1.,0.197260935827375));
#41426=CARTESIAN_POINT('Ctrl Pts',(-3.83743910616265,-1.,0.196115198971889));
#41427=CARTESIAN_POINT('Ctrl Pts',(-3.84475203347052,-1.,0.194909009460254));
#41428=CARTESIAN_POINT('Ctrl Pts',(-3.85216762264019,-1.,0.193642806777747));
#41429=CARTESIAN_POINT('Ctrl Pts',(-3.85962774407652,-1.,0.192315153044979));
#41430=CARTESIAN_POINT('Ctrl Pts',(-3.8670715862477,-1.,0.190924190418613));
#41431=CARTESIAN_POINT('Ctrl Pts',(-3.87445976418377,-1.,0.189469253358254));
#41432=CARTESIAN_POINT('Ctrl Pts',(-3.88178563496187,-1.,0.187951632512663));
#41433=CARTESIAN_POINT('Ctrl Pts',(-3.88906196725817,-1.,0.186373724985263));
#41434=CARTESIAN_POINT('Ctrl Pts',(-3.89631300742633,-1.,0.184738537728035));
#41435=CARTESIAN_POINT('Ctrl Pts',(-3.90356488555138,-1.,0.183049081993193));
#41436=CARTESIAN_POINT('Ctrl Pts',(-3.91083557557193,-1.,0.181307740731796));
#41437=CARTESIAN_POINT('Ctrl Pts',(-3.91812876180948,-1.,0.179515885822894));
#41438=CARTESIAN_POINT('Ctrl Pts',(-3.92543942697672,-1.,0.177674246152328));
#41439=CARTESIAN_POINT('Ctrl Pts',(-3.93275726771049,-1.,0.175783136893872));
#41440=CARTESIAN_POINT('Ctrl Pts',(-3.94007083096214,-1.,0.173842734974607));
#41441=CARTESIAN_POINT('Ctrl Pts',(-3.94737164900861,-1.,0.171853355369233));
#41442=CARTESIAN_POINT('Ctrl Pts',(-3.95465744665263,-1.,0.16981566637413));
#41443=CARTESIAN_POINT('Ctrl Pts',(-3.96192990160296,-1.,0.167730547023312));
#41444=CARTESIAN_POINT('Ctrl Pts',(-3.9691931362141,-1.,0.165598992851097));
#41445=CARTESIAN_POINT('Ctrl Pts',(-3.97645194630944,-1.,0.163422004609999));
#41446=CARTESIAN_POINT('Ctrl Pts',(-3.98371010319866,-1.,0.161200482186087));
#41447=CARTESIAN_POINT('Ctrl Pts',(-3.99096873945862,-1.,0.158935123982796));
#41448=CARTESIAN_POINT('Ctrl Pts',(-3.99822717425869,-1.,0.156626481393735));
#41449=CARTESIAN_POINT('Ctrl Pts',(-4.00548360245297,-1.,0.15427500487231));
#41450=CARTESIAN_POINT('Ctrl Pts',(-4.01273584234684,-1.,0.151881094022909));
#41451=CARTESIAN_POINT('Ctrl Pts',(-4.01998203715588,-1.,0.149445144968707));
#41452=CARTESIAN_POINT('Ctrl Pts',(-4.02722143147048,-1.,0.146967602878998));
#41453=CARTESIAN_POINT('Ctrl Pts',(-4.03445411510403,-1.,0.144448947038352));
#41454=CARTESIAN_POINT('Ctrl Pts',(-4.04168069633842,-1.,0.141889671485508));
#41455=CARTESIAN_POINT('Ctrl Pts',(-4.04890199238056,-1.,0.139290267180059));
#41456=CARTESIAN_POINT('Ctrl Pts',(-4.05611873400122,-1.,0.136651205046111));
#41457=CARTESIAN_POINT('Ctrl Pts',(-4.06333121018476,-1.,0.133972916144225));
#41458=CARTESIAN_POINT('Ctrl Pts',(-4.07053931528579,-1.,0.131255793548914));
#41459=CARTESIAN_POINT('Ctrl Pts',(-4.07774270738809,-1.,0.128500200484814));
#41460=CARTESIAN_POINT('Ctrl Pts',(-4.08494093372315,-1.,0.125706476822529));
#41461=CARTESIAN_POINT('Ctrl Pts',(-4.09213355850836,-1.,0.122874946249119));
#41462=CARTESIAN_POINT('Ctrl Pts',(-4.09932031767243,-1.,0.120005924388162));
#41463=CARTESIAN_POINT('Ctrl Pts',(-4.10650113382187,-1.,0.117099722731704));
#41464=CARTESIAN_POINT('Ctrl Pts',(-4.11367603925313,-1.,0.114156649609601));
#41465=CARTESIAN_POINT('Ctrl Pts',(-4.12084512502444,-1.,0.111177012683377));
#41466=CARTESIAN_POINT('Ctrl Pts',(-4.12800848371386,-1.,0.10816112052835));
#41467=CARTESIAN_POINT('Ctrl Pts',(-4.13516614458396,-1.,0.105109286538864));
#41468=CARTESIAN_POINT('Ctrl Pts',(-4.14231804938737,-1.,0.102021826577454));
#41469=CARTESIAN_POINT('Ctrl Pts',(-4.1494640891762,-1.,0.0988990478899811));
#41470=CARTESIAN_POINT('Ctrl Pts',(-4.15660412653006,-1.,0.0957412403297067));
#41471=CARTESIAN_POINT('Ctrl Pts',(-4.16373802265942,-1.,0.092548667216769));
#41472=CARTESIAN_POINT('Ctrl Pts',(-4.17086566491823,-1.,0.0893215560850327));
#41473=CARTESIAN_POINT('Ctrl Pts',(-4.17798698669991,-1.,0.0860600915552515));
#41474=CARTESIAN_POINT('Ctrl Pts',(-4.1851019532944,-1.,0.082764416438951));
#41475=CARTESIAN_POINT('Ctrl Pts',(-4.19078883322483,-1.,0.0801005887117603));
#41476=CARTESIAN_POINT('Ctrl Pts',(-4.19505112860624,-1.,0.0780873956244402));
#41477=CARTESIAN_POINT('Ctrl Pts',(-4.19789138621624,-1.,0.0767384596142195));
#41478=CARTESIAN_POINT('Ctrl Pts',(-4.19931119685982,-1.,0.0760622897878236));
#41479=CARTESIAN_POINT('',(-4.19931119685982,-1.,-0.0760622897878246));
#41480=CARTESIAN_POINT('',(-4.19931119685982,-1.,0.0760622897878236));
#41481=CARTESIAN_POINT('',(-3.74449296983004,-1.,-0.203156094896101));
#41482=CARTESIAN_POINT('Ctrl Pts',(-4.19931119685982,-1.,-0.0760622897878246));
#41483=CARTESIAN_POINT('Ctrl Pts',(-4.1978913862118,-1.,-0.0767384596141464));
#41484=CARTESIAN_POINT('Ctrl Pts',(-4.19505112859416,-1.,-0.0780873956242397));
#41485=CARTESIAN_POINT('Ctrl Pts',(-4.19078883320504,-1.,-0.080100588711432));
#41486=CARTESIAN_POINT('Ctrl Pts',(-4.18510195327123,-1.,-0.0827644164385679));
#41487=CARTESIAN_POINT('Ctrl Pts',(-4.17798698668094,-1.,-0.0860600915549397));
#41488=CARTESIAN_POINT('Ctrl Pts',(-4.17086566490794,-1.,-0.0893215560848649));
#41489=CARTESIAN_POINT('Ctrl Pts',(-4.16373802265839,-1.,-0.0925486672167531));
#41490=CARTESIAN_POINT('Ctrl Pts',(-4.15660412653577,-1.,-0.0957412403298007));
#41491=CARTESIAN_POINT('Ctrl Pts',(-4.14946408918485,-1.,-0.0988990478901226));
#41492=CARTESIAN_POINT('Ctrl Pts',(-4.14231804939538,-1.,-0.102021826577584));
#41493=CARTESIAN_POINT('Ctrl Pts',(-4.13516614458895,-1.,-0.105109286538945));
#41494=CARTESIAN_POINT('Ctrl Pts',(-4.12800848371504,-1.,-0.108161120528369));
#41495=CARTESIAN_POINT('Ctrl Pts',(-4.1208451250225,-1.,-0.111177012683347));
#41496=CARTESIAN_POINT('Ctrl Pts',(-4.11367603924961,-1.,-0.114156649609546));
#41497=CARTESIAN_POINT('Ctrl Pts',(-4.10650113381833,-1.,-0.117099722731648));
#41498=CARTESIAN_POINT('Ctrl Pts',(-4.09932031767002,-1.,-0.120005924388124));
#41499=CARTESIAN_POINT('Ctrl Pts',(-4.09213355850756,-1.,-0.122874946249107));
#41500=CARTESIAN_POINT('Ctrl Pts',(-4.08494093372377,-1.,-0.12570647682254));
#41501=CARTESIAN_POINT('Ctrl Pts',(-4.07774270738954,-1.,-0.128500200484838));
#41502=CARTESIAN_POINT('Ctrl Pts',(-4.0705393152874,-1.,-0.13125579354894));
#41503=CARTESIAN_POINT('Ctrl Pts',(-4.06333121018596,-1.,-0.133972916144245));
#41504=CARTESIAN_POINT('Ctrl Pts',(-4.05611873400172,-1.,-0.136651205046119));
#41505=CARTESIAN_POINT('Ctrl Pts',(-4.04890199238036,-1.,-0.139290267180057));
#41506=CARTESIAN_POINT('Ctrl Pts',(-4.04168069633781,-1.,-0.1418896714855));
#41507=CARTESIAN_POINT('Ctrl Pts',(-4.03445411510333,-1.,-0.144448947038345));
#41508=CARTESIAN_POINT('Ctrl Pts',(-4.02722143146994,-1.,-0.146967602878994));
#41509=CARTESIAN_POINT('Ctrl Pts',(-4.01998203715564,-1.,-0.149445144968707));
#41510=CARTESIAN_POINT('Ctrl Pts',(-4.01273584234689,-1.,-0.151881094022911));
#41511=CARTESIAN_POINT('Ctrl Pts',(-4.00548360245319,-1.,-0.154275004872311));
#41512=CARTESIAN_POINT('Ctrl Pts',(-3.99822717425893,-1.,-0.156626481393734));
#41513=CARTESIAN_POINT('Ctrl Pts',(-3.99096873945878,-1.,-0.158935123982793));
#41514=CARTESIAN_POINT('Ctrl Pts',(-3.98371010319872,-1.,-0.161200482186085));
#41515=CARTESIAN_POINT('Ctrl Pts',(-3.97645194630943,-1.,-0.163422004609999));
#41516=CARTESIAN_POINT('Ctrl Pts',(-3.96919313621407,-1.,-0.165598992851102));
#41517=CARTESIAN_POINT('Ctrl Pts',(-3.96192990160296,-1.,-0.167730547023319));
#41518=CARTESIAN_POINT('Ctrl Pts',(-3.95465744665268,-1.,-0.169815666374139));
#41519=CARTESIAN_POINT('Ctrl Pts',(-3.94737164900868,-1.,-0.17185335536924));
#41520=CARTESIAN_POINT('Ctrl Pts',(-3.94007083096217,-1.,-0.17384273497461));
#41521=CARTESIAN_POINT('Ctrl Pts',(-3.93275726771042,-1.,-0.175783136893868));
#41522=CARTESIAN_POINT('Ctrl Pts',(-3.92543942697655,-1.,-0.177674246152317));
#41523=CARTESIAN_POINT('Ctrl Pts',(-3.91812876180926,-1.,-0.179515885822882));
#41524=CARTESIAN_POINT('Ctrl Pts',(-3.91083557557175,-1.,-0.181307740731786));
#41525=CARTESIAN_POINT('Ctrl Pts',(-3.90356488555132,-1.,-0.183049081993191));
#41526=CARTESIAN_POINT('Ctrl Pts',(-3.89631300742646,-1.,-0.184738537728043));
#41527=CARTESIAN_POINT('Ctrl Pts',(-3.88906196725848,-1.,-0.18637372498528));
#41528=CARTESIAN_POINT('Ctrl Pts',(-3.88178563496228,-1.,-0.187951632512685));
#41529=CARTESIAN_POINT('Ctrl Pts',(-3.87445976418412,-1.,-0.189469253358272));
#41530=CARTESIAN_POINT('Ctrl Pts',(-3.86707158624783,-1.,-0.19092419041862));
#41531=CARTESIAN_POINT('Ctrl Pts',(-3.85962774407633,-1.,-0.192315153044971));
#41532=CARTESIAN_POINT('Ctrl Pts',(-3.85216762263966,-1.,-0.193642806777723));
#41533=CARTESIAN_POINT('Ctrl Pts',(-3.84475203346977,-1.,-0.194909009460221));
#41534=CARTESIAN_POINT('Ctrl Pts',(-3.83743910616195,-1.,-0.196115198971859));
#41535=CARTESIAN_POINT('Ctrl Pts',(-3.83026221776456,-1.,-0.197260935827361));
#41536=CARTESIAN_POINT('Ctrl Pts',(-3.82321127349016,-1.,-0.198342616900486));
#41537=CARTESIAN_POINT('Ctrl Pts',(-3.81620203429815,-1.,-0.199351525297447));
#41538=CARTESIAN_POINT('Ctrl Pts',(-3.80909529318669,-1.,-0.200274679433364));
#41539=CARTESIAN_POINT('Ctrl Pts',(-3.80175247447337,-1.,-0.201097756307326));
#41540=CARTESIAN_POINT('Ctrl Pts',(-3.7940835418736,-1.,-0.201807533800837));
#41541=CARTESIAN_POINT('Ctrl Pts',(-3.78609175019242,-1.,-0.20239426051216));
#41542=CARTESIAN_POINT('Ctrl Pts',(-3.77793553476614,-1.,-0.202854729699081));
#41543=CARTESIAN_POINT('Ctrl Pts',(-3.7699207159487,-1.,-0.203192390045164));
#41544=CARTESIAN_POINT('Ctrl Pts',(-3.76242717936885,-1.,-0.203414634707478));
#41545=CARTESIAN_POINT('Ctrl Pts',(-3.75585118707734,-1.,-0.203530796848322));
#41546=CARTESIAN_POINT('Ctrl Pts',(-3.75054693397875,-1.,-0.203550035479166));
#41547=CARTESIAN_POINT('Ctrl Pts',(-3.74703926501752,-1.,-0.203484186269415));
#41548=CARTESIAN_POINT('Ctrl Pts',(-3.74535749969115,-1.,-0.203375226874121));
#41549=CARTESIAN_POINT('Ctrl Pts',(-3.74471097893845,-1.,-0.203266610110531));
#41550=CARTESIAN_POINT('Ctrl Pts',(-3.74453008995092,-1.,-0.203188003946657));
#41551=CARTESIAN_POINT('Ctrl Pts',(-3.74449296983004,-1.,-0.203156094896101));
#41552=CARTESIAN_POINT('',(-3.73017266276651,-1.,-0.385112848330762));
#41553=CARTESIAN_POINT('Origin',(0.,-1.,0.));
#41554=CARTESIAN_POINT('',(-4.15950947128175,-1.,-0.581791163835815));
#41555=CARTESIAN_POINT('Ctrl Pts',(-3.73017266276651,-1.,-0.385112848330762));
#41556=CARTESIAN_POINT('Ctrl Pts',(-3.73021431755274,-1.,-0.385087139000374));
#41557=CARTESIAN_POINT('Ctrl Pts',(-3.73040527621055,-1.,-0.385037797881504));
#41558=CARTESIAN_POINT('Ctrl Pts',(-3.73106082862548,-1.,-0.385031656499164));
#41559=CARTESIAN_POINT('Ctrl Pts',(-3.73273893363406,-1.,-0.385187124634206));
#41560=CARTESIAN_POINT('Ctrl Pts',(-3.73621371845318,-1.,-0.385670806454566));
#41561=CARTESIAN_POINT('Ctrl Pts',(-3.74144965781276,-1.,-0.386519576222251));
#41562=CARTESIAN_POINT('Ctrl Pts',(-3.74792651696654,-1.,-0.387663020050836));
#41563=CARTESIAN_POINT('Ctrl Pts',(-3.75529302895152,-1.,-0.389054775898702));
#41564=CARTESIAN_POINT('Ctrl Pts',(-3.76315635033257,-1.,-0.39064207297956));
#41565=CARTESIAN_POINT('Ctrl Pts',(-3.77114011595967,-1.,-0.392372786223432));
#41566=CARTESIAN_POINT('Ctrl Pts',(-3.77894173114283,-1.,-0.394202481011499));
#41567=CARTESIAN_POINT('Ctrl Pts',(-3.78640521279313,-1.,-0.396103205334841));
#41568=CARTESIAN_POINT('Ctrl Pts',(-3.7935288716329,-1.,-0.398064818683969));
#41569=CARTESIAN_POINT('Ctrl Pts',(-3.80040370384546,-1.,-0.4000883465046));
#41570=CARTESIAN_POINT('Ctrl Pts',(-3.80716881962728,-1.,-0.402181320148436));
#41571=CARTESIAN_POINT('Ctrl Pts',(-3.81396374287793,-1.,-0.404352694628273));
#41572=CARTESIAN_POINT('Ctrl Pts',(-3.8208730391381,-1.,-0.406607038258985));
#41573=CARTESIAN_POINT('Ctrl Pts',(-3.82790724256471,-1.,-0.40894237144746));
#41574=CARTESIAN_POINT('Ctrl Pts',(-3.83503345578698,-1.,-0.411353038798518));
#41575=CARTESIAN_POINT('Ctrl Pts',(-3.84219403994762,-1.,-0.413831367016748));
#41576=CARTESIAN_POINT('Ctrl Pts',(-3.84932864157497,-1.,-0.416369678052907));
#41577=CARTESIAN_POINT('Ctrl Pts',(-3.85639825647996,-1.,-0.418962468086773));
#41578=CARTESIAN_POINT('Ctrl Pts',(-3.86339652542709,-1.,-0.421607423177534));
#41579=CARTESIAN_POINT('Ctrl Pts',(-3.87033643487851,-1.,-0.424304173195111));
#41580=CARTESIAN_POINT('Ctrl Pts',(-3.87724240306597,-1.,-0.427053541173457));
#41581=CARTESIAN_POINT('Ctrl Pts',(-3.88414070943341,-1.,-0.429856640579741));
#41582=CARTESIAN_POINT('Ctrl Pts',(-3.89104947940611,-1.,-0.432713929544458));
#41583=CARTESIAN_POINT('Ctrl Pts',(-3.89797256655462,-1.,-0.435624629433527));
#41584=CARTESIAN_POINT('Ctrl Pts',(-3.90490512938563,-1.,-0.438587235458249));
#41585=CARTESIAN_POINT('Ctrl Pts',(-3.91183704069153,-1.,-0.441599824524054));
#41586=CARTESIAN_POINT('Ctrl Pts',(-3.91875701610719,-1.,-0.444660430230591));
#41587=CARTESIAN_POINT('Ctrl Pts',(-3.92565674143416,-1.,-0.447767416837292));
#41588=CARTESIAN_POINT('Ctrl Pts',(-3.93253407403123,-1.,-0.450919768356348));
#41589=CARTESIAN_POINT('Ctrl Pts',(-3.93939080846298,-1.,-0.454116879027584));
#41590=CARTESIAN_POINT('Ctrl Pts',(-3.94623117206678,-1.,-0.457358410451683));
#41591=CARTESIAN_POINT('Ctrl Pts',(-3.95306005817364,-1.,-0.460644124429121));
#41592=CARTESIAN_POINT('Ctrl Pts',(-3.95988133243538,-1.,-0.463973722115733));
#41593=CARTESIAN_POINT('Ctrl Pts',(-3.9666962227393,-1.,-0.467346690880643));
#41594=CARTESIAN_POINT('Ctrl Pts',(-3.97350414289392,-1.,-0.470762379613439));
#41595=CARTESIAN_POINT('Ctrl Pts',(-3.98030338044409,-1.,-0.47422006101951));
#41596=CARTESIAN_POINT('Ctrl Pts',(-3.98709184306738,-1.,-0.477718999122027));
#41597=CARTESIAN_POINT('Ctrl Pts',(-3.99386775880679,-1.,-0.481258512209675));
#41598=CARTESIAN_POINT('Ctrl Pts',(-4.00063045119288,-1.,-0.484838042421835));
#41599=CARTESIAN_POINT('Ctrl Pts',(-4.0073800839099,-1.,-0.488457130424633));
#41600=CARTESIAN_POINT('Ctrl Pts',(-4.01411733503546,-1.,-0.492115383418018));
#41601=CARTESIAN_POINT('Ctrl Pts',(-4.02084308851832,-1.,-0.495812444326251));
#41602=CARTESIAN_POINT('Ctrl Pts',(-4.02755813980101,-1.,-0.499547962340821));
#41603=CARTESIAN_POINT('Ctrl Pts',(-4.03426284174272,-1.,-0.503321556915346));
#41604=CARTESIAN_POINT('Ctrl Pts',(-4.04095715148915,-1.,-0.507132823288136));
#41605=CARTESIAN_POINT('Ctrl Pts',(-4.04764078815447,-1.,-0.51098134921897));
#41606=CARTESIAN_POINT('Ctrl Pts',(-4.05431335771199,-1.,-0.514866728193017));
#41607=CARTESIAN_POINT('Ctrl Pts',(-4.06097448038013,-1.,-0.518788572336923));
#41608=CARTESIAN_POINT('Ctrl Pts',(-4.06762394471314,-1.,-0.522746528603107));
#41609=CARTESIAN_POINT('Ctrl Pts',(-4.07426172299847,-1.,-0.526740277227498));
#41610=CARTESIAN_POINT('Ctrl Pts',(-4.08088789536836,-1.,-0.530769518728571));
#41611=CARTESIAN_POINT('Ctrl Pts',(-4.08750259988885,-1.,-0.534833963477273));
#41612=CARTESIAN_POINT('Ctrl Pts',(-4.09410597627,-1.,-0.538933321179756));
#41613=CARTESIAN_POINT('Ctrl Pts',(-4.10069810243979,-1.,-0.543067286877757));
#41614=CARTESIAN_POINT('Ctrl Pts',(-4.10727897027977,-1.,-0.547235539485637));
#41615=CARTESIAN_POINT('Ctrl Pts',(-4.11384852024721,-1.,-0.551437758497032));
#41616=CARTESIAN_POINT('Ctrl Pts',(-4.12040666195664,-1.,-0.555673636129977));
#41617=CARTESIAN_POINT('Ctrl Pts',(-4.12695329951961,-1.,-0.559942890594773));
#41618=CARTESIAN_POINT('Ctrl Pts',(-4.13348835727104,-1.,-0.564245279537148));
#41619=CARTESIAN_POINT('Ctrl Pts',(-4.14001179830547,-1.,-0.568580610189774));
#41620=CARTESIAN_POINT('Ctrl Pts',(-4.14652361068081,-1.,-0.572948736069522));
#41621=CARTESIAN_POINT('Ctrl Pts',(-4.151723761217,-1.,-0.576469391676688));
#41622=CARTESIAN_POINT('Ctrl Pts',(-4.15561864788576,-1.,-0.579124568914235));
#41623=CARTESIAN_POINT('Ctrl Pts',(-4.1582129171283,-1.,-0.580901211463535));
#41624=CARTESIAN_POINT('Ctrl Pts',(-4.15950947128175,-1.,-0.581791163835815));
#41625=CARTESIAN_POINT('',(-4.13571194405636,-1.,-0.73204283740062));
#41626=CARTESIAN_POINT('',(-4.15950947128175,-1.,-0.581791163835815));
#41627=CARTESIAN_POINT('',(-3.66661143271685,-1.,-0.786422660831985));
#41628=CARTESIAN_POINT('Ctrl Pts',(-4.13571194405636,-1.,-0.73204283740062));
#41629=CARTESIAN_POINT('Ctrl Pts',(-4.1342038373684,-1.,-0.732488575135159));
#41630=CARTESIAN_POINT('Ctrl Pts',(-4.13118752795207,-1.,-0.733376589323546));
#41631=CARTESIAN_POINT('Ctrl Pts',(-4.12666277570844,-1.,-0.734698226764092));
#41632=CARTESIAN_POINT('Ctrl Pts',(-4.120629196238,-1.,-0.736439634331345));
#41633=CARTESIAN_POINT('Ctrl Pts',(-4.11308626951927,-1.,-0.738581708225844));
#41634=CARTESIAN_POINT('Ctrl Pts',(-4.10554241757547,-1.,-0.740688998553377));
#41635=CARTESIAN_POINT('Ctrl Pts',(-4.09799769702611,-1.,-0.742761369689841));
#41636=CARTESIAN_POINT('Ctrl Pts',(-4.09045220253573,-1.,-0.7447986497065));
#41637=CARTESIAN_POINT('Ctrl Pts',(-4.08290608095642,-1.,-0.746800631492315));
#41638=CARTESIAN_POINT('Ctrl Pts',(-4.07535951056152,-1.,-0.748767076680557));
#41639=CARTESIAN_POINT('Ctrl Pts',(-4.06781267242378,-1.,-0.750697720484036));
#41640=CARTESIAN_POINT('Ctrl Pts',(-4.06026572221515,-1.,-0.752592276483072));
#41641=CARTESIAN_POINT('Ctrl Pts',(-4.05271876687915,-1.,-0.754450441816078));
#41642=CARTESIAN_POINT('Ctrl Pts',(-4.04517182653997,-1.,-0.756271902369581));
#41643=CARTESIAN_POINT('Ctrl Pts',(-4.03762485803119,-1.,-0.758056338884944));
#41644=CARTESIAN_POINT('Ctrl Pts',(-4.03007781954412,-1.,-0.759803433243752));
#41645=CARTESIAN_POINT('Ctrl Pts',(-4.02253072741268,-1.,-0.761512875859804));
#41646=CARTESIAN_POINT('Ctrl Pts',(-4.01498370680496,-1.,-0.763184371182935));
#41647=CARTESIAN_POINT('Ctrl Pts',(-4.00743706791509,-1.,-0.764817648785197));
#41648=CARTESIAN_POINT('Ctrl Pts',(-3.99989129179622,-1.,-0.766412457136064));
#41649=CARTESIAN_POINT('Ctrl Pts',(-3.9923468788101,-1.,-0.767968531377915));
#41650=CARTESIAN_POINT('Ctrl Pts',(-3.98480422348451,-1.,-0.769485566245544));
#41651=CARTESIAN_POINT('Ctrl Pts',(-3.97726349165488,-1.,-0.770963190030471));
#41652=CARTESIAN_POINT('Ctrl Pts',(-3.96972446532772,-1.,-0.772400931772136));
#41653=CARTESIAN_POINT('Ctrl Pts',(-3.96218649639807,-1.,-0.773798212026565));
#41654=CARTESIAN_POINT('Ctrl Pts',(-3.9546488545231,-1.,-0.775154418039351));
#41655=CARTESIAN_POINT('Ctrl Pts',(-3.94711101619447,-1.,-0.776468966697921));
#41656=CARTESIAN_POINT('Ctrl Pts',(-3.93957296768103,-1.,-0.777741370568558));
#41657=CARTESIAN_POINT('Ctrl Pts',(-3.93203552473174,-1.,-0.778971308134821));
#41658=CARTESIAN_POINT('Ctrl Pts',(-3.92450058323823,-1.,-0.780158678615542));
#41659=CARTESIAN_POINT('Ctrl Pts',(-3.91697036054676,-1.,-0.781303428618366));
#41660=CARTESIAN_POINT('Ctrl Pts',(-3.90944671004542,-1.,-0.782405395622764));
#41661=CARTESIAN_POINT('Ctrl Pts',(-3.9019303904397,-1.,-0.783464141529081));
#41662=CARTESIAN_POINT('Ctrl Pts',(-3.89442039235103,-1.,-0.784478799358336));
#41663=CARTESIAN_POINT('Ctrl Pts',(-3.88691313167398,-1.,-0.78544789034073));
#41664=CARTESIAN_POINT('Ctrl Pts',(-3.8794040281819,-1.,-0.786369675812608));
#41665=CARTESIAN_POINT('Ctrl Pts',(-3.87188916600912,-1.,-0.787242527617999));
#41666=CARTESIAN_POINT('Ctrl Pts',(-3.86436702561345,-1.,-0.788065315093777));
#41667=CARTESIAN_POINT('Ctrl Pts',(-3.85683995872529,-1.,-0.788837734090672));
#41668=CARTESIAN_POINT('Ctrl Pts',(-3.84931637808894,-1.,-0.789560798155582));
#41669=CARTESIAN_POINT('Ctrl Pts',(-3.84180762342454,-1.,-0.790236124191242));
#41670=CARTESIAN_POINT('Ctrl Pts',(-3.83432392054786,-1.,-0.790865012705301));
#41671=CARTESIAN_POINT('Ctrl Pts',(-3.82687033899792,-1.,-0.791447528662369));
#41672=CARTESIAN_POINT('Ctrl Pts',(-3.81944345442249,-1.,-0.791981740718635));
#41673=CARTESIAN_POINT('Ctrl Pts',(-3.81202588694756,-1.,-0.792462483517634));
#41674=CARTESIAN_POINT('Ctrl Pts',(-3.80459229925637,-1.,-0.792882695234778));
#41675=CARTESIAN_POINT('Ctrl Pts',(-3.79711921389897,-1.,-0.793235612973273));
#41676=CARTESIAN_POINT('Ctrl Pts',(-3.78959439439235,-1.,-0.793516871680993));
#41677=CARTESIAN_POINT('Ctrl Pts',(-3.78202460377598,-1.,-0.7937262357813));
#41678=CARTESIAN_POINT('Ctrl Pts',(-3.77444863801212,-1.,-0.793870523787408));
#41679=CARTESIAN_POINT('Ctrl Pts',(-3.76692626931111,-1.,-0.793961083688991));
#41680=CARTESIAN_POINT('Ctrl Pts',(-3.75951468666257,-1.,-0.794008429134907));
#41681=CARTESIAN_POINT('Ctrl Pts',(-3.75224692493864,-1.,-0.794017347371377));
#41682=CARTESIAN_POINT('Ctrl Pts',(-3.74511357728861,-1.,-0.793982700459952));
#41683=CARTESIAN_POINT('Ctrl Pts',(-3.73803280541687,-1.,-0.793882700937017));
#41684=CARTESIAN_POINT('Ctrl Pts',(-3.73086914695805,-1.,-0.793682750269684));
#41685=CARTESIAN_POINT('Ctrl Pts',(-3.72348797293734,-1.,-0.793347023784205));
#41686=CARTESIAN_POINT('Ctrl Pts',(-3.71580242396124,-1.,-0.792848377370287));
#41687=CARTESIAN_POINT('Ctrl Pts',(-3.70781724021806,-1.,-0.792177688845818));
#41688=CARTESIAN_POINT('Ctrl Pts',(-3.69968940808721,-1.,-0.79135657569598));
#41689=CARTESIAN_POINT('Ctrl Pts',(-3.69172044327364,-1.,-0.790436284988787));
#41690=CARTESIAN_POINT('Ctrl Pts',(-3.68428439783905,-1.,-0.789483546064387));
#41691=CARTESIAN_POINT('Ctrl Pts',(-3.67777119516252,-1.,-0.788569566220285));
#41692=CARTESIAN_POINT('Ctrl Pts',(-3.67252923663655,-1.,-0.787758799995742));
#41693=CARTESIAN_POINT('Ctrl Pts',(-3.66907505398677,-1.,-0.787145041181545));
#41694=CARTESIAN_POINT('Ctrl Pts',(-3.66743103898702,-1.,-0.786774337198062));
#41695=CARTESIAN_POINT('Ctrl Pts',(-3.66680946938292,-1.,-0.786565919558984));
#41696=CARTESIAN_POINT('Ctrl Pts',(-3.6666431041522,-1.,-0.786459983895432));
#41697=CARTESIAN_POINT('Ctrl Pts',(-3.66661143271685,-1.,-0.786422660831985));
#41698=CARTESIAN_POINT('',(-3.62400312501245,-1.,-0.963899035117249));
#41699=CARTESIAN_POINT('Origin',(0.,-1.,0.));
#41700=CARTESIAN_POINT('',(-4.01728681790024,-1.,-1.22531898815164));
#41701=CARTESIAN_POINT('Ctrl Pts',(-3.62400312501245,-1.,-0.963899035117249));
#41702=CARTESIAN_POINT('Ctrl Pts',(-3.6240482887845,-1.,-0.963880158555582));
#41703=CARTESIAN_POINT('Ctrl Pts',(-3.62424461507588,-1.,-0.963861297423241));
#41704=CARTESIAN_POINT('Ctrl Pts',(-3.62489305727662,-1.,-0.963957782642843));
#41705=CARTESIAN_POINT('Ctrl Pts',(-3.62652618145335,-1.,-0.964373850166457));
#41706=CARTESIAN_POINT('Ctrl Pts',(-3.62988252139846,-1.,-0.965395153165293));
#41707=CARTESIAN_POINT('Ctrl Pts',(-3.63492122081143,-1.,-0.967052554541385));
#41708=CARTESIAN_POINT('Ctrl Pts',(-3.64113946505766,-1.,-0.969195124675865));
#41709=CARTESIAN_POINT('Ctrl Pts',(-3.64819756447455,-1.,-0.971722122061341));
#41710=CARTESIAN_POINT('Ctrl Pts',(-3.65571576735126,-1.,-0.974519971354848));
#41711=CARTESIAN_POINT('Ctrl Pts',(-3.66333049637475,-1.,-0.977478312751618));
#41712=CARTESIAN_POINT('Ctrl Pts',(-3.67074983340361,-1.,-0.980505922458267));
#41713=CARTESIAN_POINT('Ctrl Pts',(-3.67782408841715,-1.,-0.983550791470419));
#41714=CARTESIAN_POINT('Ctrl Pts',(-3.68455317926068,-1.,-0.986602639863837));
#41715=CARTESIAN_POINT('Ctrl Pts',(-3.69102682138846,-1.,-0.989676715398558));
#41716=CARTESIAN_POINT('Ctrl Pts',(-3.69738123415662,-1.,-0.99280221833201));
#41717=CARTESIAN_POINT('Ctrl Pts',(-3.70375282282138,-1.,-0.996009819772518));
#41718=CARTESIAN_POINT('Ctrl Pts',(-3.71022439713938,-1.,-0.99931726075653));
#41719=CARTESIAN_POINT('Ctrl Pts',(-3.71680667125118,-1.,-1.00272423396822));
#41720=CARTESIAN_POINT('Ctrl Pts',(-3.72346803750595,-1.,-1.0062200073571));
#41721=CARTESIAN_POINT('Ctrl Pts',(-3.73015276704426,-1.,-1.00978798539496));
#41722=CARTESIAN_POINT('Ctrl Pts',(-3.73680245055734,-1.,-1.01341114319903));
#41723=CARTESIAN_POINT('Ctrl Pts',(-3.74337942504959,-1.,-1.01707794311079));
#41724=CARTESIAN_POINT('Ctrl Pts',(-3.74987777155834,-1.,-1.02078510487428));
#41725=CARTESIAN_POINT('Ctrl Pts',(-3.75631037456194,-1.,-1.0245342944466));
#41726=CARTESIAN_POINT('Ctrl Pts',(-3.76270122291232,-1.,-1.02833014458181));
#41727=CARTESIAN_POINT('Ctrl Pts',(-3.76907609832522,-1.,-1.0321778660492));
#41728=CARTESIAN_POINT('Ctrl Pts',(-3.77545283140445,-1.,-1.03608074678013));
#41729=CARTESIAN_POINT('Ctrl Pts',(-3.78183535008192,-1.,-1.04003862055804));
#41730=CARTESIAN_POINT('Ctrl Pts',(-3.78821910787195,-1.,-1.04404924374426));
#41731=CARTESIAN_POINT('Ctrl Pts',(-3.79459440308793,-1.,-1.04810913267641));
#41732=CARTESIAN_POINT('Ctrl Pts',(-3.80095039790678,-1.,-1.05221457990015));
#41733=CARTESIAN_POINT('Ctrl Pts',(-3.80727913637784,-1.,-1.05636266918643));
#41734=CARTESIAN_POINT('Ctrl Pts',(-3.81357866117485,-1.,-1.06055206187298));
#41735=CARTESIAN_POINT('Ctrl Pts',(-3.81985083953012,-1.,-1.06478244038931));
#41736=CARTESIAN_POINT('Ctrl Pts',(-3.82609989967278,-1.,-1.0690541318036));
#41737=CARTESIAN_POINT('Ctrl Pts',(-3.83233071195145,-1.,-1.0733676663346));
#41738=CARTESIAN_POINT('Ctrl Pts',(-3.83854714117486,-1.,-1.07772335353856));
#41739=CARTESIAN_POINT('Ctrl Pts',(-3.84475048030615,-1.,-1.08212087917986));
#41740=CARTESIAN_POINT('Ctrl Pts',(-3.8509402522269,-1.,-1.08655950846377));
#41741=CARTESIAN_POINT('Ctrl Pts',(-3.85711487933911,-1.,-1.09103825516288));
#41742=CARTESIAN_POINT('Ctrl Pts',(-3.86327241021242,-1.,-1.09555606505012));
#41743=CARTESIAN_POINT('Ctrl Pts',(-3.86941120134872,-1.,-1.10011198761202));
#41744=CARTESIAN_POINT('Ctrl Pts',(-3.87553067187566,-1.,-1.10470536603303));
#41745=CARTESIAN_POINT('Ctrl Pts',(-3.88163105531791,-1.,-1.10933577224029));
#41746=CARTESIAN_POINT('Ctrl Pts',(-3.88771308285229,-1.,-1.11400292434447));
#41747=CARTESIAN_POINT('Ctrl Pts',(-3.89377768340362,-1.,-1.11870660794609));
#41748=CARTESIAN_POINT('Ctrl Pts',(-3.89982569749978,-1.,-1.12344660099029));
#41749=CARTESIAN_POINT('Ctrl Pts',(-3.90585753318622,-1.,-1.12822258281518));
#41750=CARTESIAN_POINT('Ctrl Pts',(-3.91187321145495,-1.,-1.13303414693849));
#41751=CARTESIAN_POINT('Ctrl Pts',(-3.91787251936688,-1.,-1.13788084225511));
#41752=CARTESIAN_POINT('Ctrl Pts',(-3.92385513133937,-1.,-1.14276220561575));
#41753=CARTESIAN_POINT('Ctrl Pts',(-3.92982073294334,-1.,-1.14767779451147));
#41754=CARTESIAN_POINT('Ctrl Pts',(-3.9357691705651,-1.,-1.1526272271639));
#41755=CARTESIAN_POINT('Ctrl Pts',(-3.94170046685542,-1.,-1.1576101834106));
#41756=CARTESIAN_POINT('Ctrl Pts',(-3.9476147478092,-1.,-1.16262637999261));
#41757=CARTESIAN_POINT('Ctrl Pts',(-3.95351219510062,-1.,-1.16767555244495));
#41758=CARTESIAN_POINT('Ctrl Pts',(-3.95939299213164,-1.,-1.17275743590327));
#41759=CARTESIAN_POINT('Ctrl Pts',(-3.96525726357682,-1.,-1.17787174135445));
#41760=CARTESIAN_POINT('Ctrl Pts',(-3.9711050516465,-1.,-1.18301815039596));
#41761=CARTESIAN_POINT('Ctrl Pts',(-3.97693634766926,-1.,-1.18819633715285));
#41762=CARTESIAN_POINT('Ctrl Pts',(-3.98275111052015,-1.,-1.19340598349307));
#41763=CARTESIAN_POINT('Ctrl Pts',(-3.98854928957287,-1.,-1.19864679609596));
#41764=CARTESIAN_POINT('Ctrl Pts',(-3.99433084800649,-1.,-1.2039185237544));
#41765=CARTESIAN_POINT('Ctrl Pts',(-4.00009577952534,-1.,-1.20922097030107));
#41766=CARTESIAN_POINT('Ctrl Pts',(-4.00584409524937,-1.,-1.21455398918813));
#41767=CARTESIAN_POINT('Ctrl Pts',(-4.01042947142681,-1.,-1.21884478244983));
#41768=CARTESIAN_POINT('Ctrl Pts',(-4.01386104434674,-1.,-1.22207656456199));
#41769=CARTESIAN_POINT('Ctrl Pts',(-4.0161454457032,-1.,-1.22423716681447));
#41770=CARTESIAN_POINT('Ctrl Pts',(-4.01728681790024,-1.,-1.22531898815164));
#41771=CARTESIAN_POINT('',(-3.97027773754922,-1.,-1.36999806084572));
#41772=CARTESIAN_POINT('',(-4.01728681790024,-1.,-1.22531898815164));
#41773=CARTESIAN_POINT('',(-3.4984457533445,-1.,-1.35032489087101));
#41774=CARTESIAN_POINT('Ctrl Pts',(-3.97027773754922,-1.,-1.36999806084572));
#41775=CARTESIAN_POINT('Ctrl Pts',(-3.9687184694131,-1.,-1.37020239094614));
#41776=CARTESIAN_POINT('Ctrl Pts',(-3.96560037974645,-1.,-1.37060761745635));
#41777=CARTESIAN_POINT('Ctrl Pts',(-3.96092458506535,-1.,-1.3712051561502));
#41778=CARTESIAN_POINT('Ctrl Pts',(-3.95469287280914,-1.,-1.37198126432386));
#41779=CARTESIAN_POINT('Ctrl Pts',(-3.94690771785133,-1.,-1.37291699202807));
#41780=CARTESIAN_POINT('Ctrl Pts',(-3.93912709040818,-1.,-1.37381821967165));
#41781=CARTESIAN_POINT('Ctrl Pts',(-3.93135106761844,-1.,-1.37468482215751));
#41782=CARTESIAN_POINT('Ctrl Pts',(-3.92357976987672,-1.,-1.37551664448242));
#41783=CARTESIAN_POINT('Ctrl Pts',(-3.91581337462644,-1.,-1.37631350505797));
#41784=CARTESIAN_POINT('Ctrl Pts',(-3.90805209523486,-1.,-1.3770751963402));
#41785=CARTESIAN_POINT('Ctrl Pts',(-3.90029615196727,-1.,-1.37780148512792));
#41786=CARTESIAN_POINT('Ctrl Pts',(-3.89254574338496,-1.,-1.3784921128802));
#41787=CARTESIAN_POINT('Ctrl Pts',(-3.88480102249277,-1.,-1.37914679719383));
#41788=CARTESIAN_POINT('Ctrl Pts',(-3.87706205830532,-1.,-1.37976523097073));
#41789=CARTESIAN_POINT('Ctrl Pts',(-3.86932885813068,-1.,-1.38034709213014));
#41790=CARTESIAN_POINT('Ctrl Pts',(-3.86160143043959,-1.,-1.38089205992989));
#41791=CARTESIAN_POINT('Ctrl Pts',(-3.85387983979481,-1.,-1.38139983115049));
#41792=CARTESIAN_POINT('Ctrl Pts',(-3.84616425605764,-1.,-1.38187013346109));
#41793=CARTESIAN_POINT('Ctrl Pts',(-3.83845502790746,-1.,-1.38230274828821));
#41794=CARTESIAN_POINT('Ctrl Pts',(-3.8307526698229,-1.,-1.38269750245138));
#41795=CARTESIAN_POINT('Ctrl Pts',(-3.82305771743829,-1.,-1.38305421262763));
#41796=CARTESIAN_POINT('Ctrl Pts',(-3.81537060817811,-1.,-1.38337263902782));
#41797=CARTESIAN_POINT('Ctrl Pts',(-3.80769156398411,-1.,-1.3836524404622));
#41798=CARTESIAN_POINT('Ctrl Pts',(-3.80002044322111,-1.,-1.38389311766682));
#41799=CARTESIAN_POINT('Ctrl Pts',(-3.79235669640841,-1.,-1.38409399694566));
#41800=CARTESIAN_POINT('Ctrl Pts',(-3.78469969805082,-1.,-1.38425435883756));
#41801=CARTESIAN_POINT('Ctrl Pts',(-3.77704902230418,-1.,-1.38437354551428));
#41802=CARTESIAN_POINT('Ctrl Pts',(-3.76940473185779,-1.,-1.38445107339518));
#41803=CARTESIAN_POINT('Ctrl Pts',(-3.76176768271367,-1.,-1.3844867525335));
#41804=CARTESIAN_POINT('Ctrl Pts',(-3.7541397631875,-1.,-1.38448077997163));
#41805=CARTESIAN_POINT('Ctrl Pts',(-3.74652317167876,-1.,-1.38443344984394));
#41806=CARTESIAN_POINT('Ctrl Pts',(-3.73891976418104,-1.,-1.38434489156458));
#41807=CARTESIAN_POINT('Ctrl Pts',(-3.73133035859282,-1.,-1.38421479111531));
#41808=CARTESIAN_POINT('Ctrl Pts',(-3.72375409358803,-1.,-1.3840421342895));
#41809=CARTESIAN_POINT('Ctrl Pts',(-3.7161876605181,-1.,-1.38382489984586));
#41810=CARTESIAN_POINT('Ctrl Pts',(-3.70862680753347,-1.,-1.38356065402124));
#41811=CARTESIAN_POINT('Ctrl Pts',(-3.701067921679,-1.,-1.38324717612865));
#41812=CARTESIAN_POINT('Ctrl Pts',(-3.69350967899526,-1.,-1.3828831117165));
#41813=CARTESIAN_POINT('Ctrl Pts',(-3.68595444983837,-1.,-1.38246852827182));
#41814=CARTESIAN_POINT('Ctrl Pts',(-3.67841038482414,-1.,-1.3820057429062));
#41815=CARTESIAN_POINT('Ctrl Pts',(-3.67088843112262,-1.,-1.38149812653868));
#41816=CARTESIAN_POINT('Ctrl Pts',(-3.66339848520857,-1.,-1.38094856333552));
#41817=CARTESIAN_POINT('Ctrl Pts',(-3.6559455440439,-1.,-1.38035791051212));
#41818=CARTESIAN_POINT('Ctrl Pts',(-3.64852652756456,-1.,-1.37972372481603));
#41819=CARTESIAN_POINT('Ctrl Pts',(-3.64112507791141,-1.,-1.37903818567359));
#41820=CARTESIAN_POINT('Ctrl Pts',(-3.63371727442486,-1.,-1.37829035457339));
#41821=CARTESIAN_POINT('Ctrl Pts',(-3.62628098665145,-1.,-1.37746987919881));
#41822=CARTESIAN_POINT('Ctrl Pts',(-3.6188048116042,-1.,-1.37657053403107));
#41823=CARTESIAN_POINT('Ctrl Pts',(-3.61129546591064,-1.,-1.37559314436634));
#41824=CARTESIAN_POINT('Ctrl Pts',(-3.60379020123988,-1.,-1.37455051379623));
#41825=CARTESIAN_POINT('Ctrl Pts',(-3.59634627869048,-1.,-1.37346320103157));
#41826=CARTESIAN_POINT('Ctrl Pts',(-3.58901853846365,-1.,-1.37235053660976));
#41827=CARTESIAN_POINT('Ctrl Pts',(-3.58183885982715,-1.,-1.37122241663062));
#41828=CARTESIAN_POINT('Ctrl Pts',(-3.57479875549486,-1.,-1.37007229485659));
#41829=CARTESIAN_POINT('Ctrl Pts',(-3.5678208030466,-1.,-1.36886584973389));
#41830=CARTESIAN_POINT('Ctrl Pts',(-3.56077662028649,-1.,-1.36754771771233));
#41831=CARTESIAN_POINT('Ctrl Pts',(-3.55353883995949,-1.,-1.3660614545677));
#41832=CARTESIAN_POINT('Ctrl Pts',(-3.54602591832973,-1.,-1.36436666257597));
#41833=CARTESIAN_POINT('Ctrl Pts',(-3.53824396424961,-1.,-1.36245507339307));
#41834=CARTESIAN_POINT('Ctrl Pts',(-3.530344649616,-1.,-1.36037259643734));
#41835=CARTESIAN_POINT('Ctrl Pts',(-3.52261776116748,-1.,-1.35821701528836));
#41836=CARTESIAN_POINT('Ctrl Pts',(-3.51542230699556,-1.,-1.35611275237152));
#41837=CARTESIAN_POINT('Ctrl Pts',(-3.50913227059999,-1.,-1.35419113575956));
#41838=CARTESIAN_POINT('Ctrl Pts',(-3.50408168106261,-1.,-1.35257032843486));
#41839=CARTESIAN_POINT('Ctrl Pts',(-3.5007660381649,-1.,-1.35142377279517));
#41840=CARTESIAN_POINT('Ctrl Pts',(-3.49920025459723,-1.,-1.35080045218587));
#41841=CARTESIAN_POINT('Ctrl Pts',(-3.49861894124827,-1.,-1.35049736560527));
#41842=CARTESIAN_POINT('Ctrl Pts',(-3.49847119623846,-1.,-1.35036670892966));
#41843=CARTESIAN_POINT('Ctrl Pts',(-3.4984457533445,-1.,-1.35032489087101));
#41844=CARTESIAN_POINT('',(-3.42859860294378,-1.,-1.51895082866166));
#41845=CARTESIAN_POINT('Origin',(0.,-1.,0.));
#41846=CARTESIAN_POINT('',(-3.77614523045147,-1.,-1.83867539237861));
#41847=CARTESIAN_POINT('Ctrl Pts',(-3.42859860294378,-1.,-1.51895082866166));
#41848=CARTESIAN_POINT('Ctrl Pts',(-3.42864616361967,-1.,-1.51893924967231));
#41849=CARTESIAN_POINT('Ctrl Pts',(-3.42884302333978,-1.,-1.51895133295017));
#41850=CARTESIAN_POINT('Ctrl Pts',(-3.42946838852728,-1.,-1.51914806898539));
#41851=CARTESIAN_POINT('Ctrl Pts',(-3.43101631893491,-1.,-1.5198144909343));
#41852=CARTESIAN_POINT('Ctrl Pts',(-3.43417156977749,-1.,-1.52134826724227));
#41853=CARTESIAN_POINT('Ctrl Pts',(-3.43888895974182,-1.,-1.52377348950429));
#41854=CARTESIAN_POINT('Ctrl Pts',(-3.44469547527,-1.,-1.52686242875717));
#41855=CARTESIAN_POINT('Ctrl Pts',(-3.45127136828667,-1.,-1.530462444618));
#41856=CARTESIAN_POINT('Ctrl Pts',(-3.45825932955273,-1.,-1.53440195378902));
#41857=CARTESIAN_POINT('Ctrl Pts',(-3.46531752207222,-1.,-1.53851507915533));
#41858=CARTESIAN_POINT('Ctrl Pts',(-3.47217189224576,-1.,-1.54266605398152));
#41859=CARTESIAN_POINT('Ctrl Pts',(-3.47868272898599,-1.,-1.54678009290206));
#41860=CARTESIAN_POINT('Ctrl Pts',(-3.48485155928414,-1.,-1.55084702970382));
#41861=CARTESIAN_POINT('Ctrl Pts',(-3.49076460877317,-1.,-1.5548959590107));
#41862=CARTESIAN_POINT('Ctrl Pts',(-3.49655185179623,-1.,-1.55897703097859));
#41863=CARTESIAN_POINT('Ctrl Pts',(-3.50234321621607,-1.,-1.56314187758689));
#41864=CARTESIAN_POINT('Ctrl Pts',(-3.50821771695427,-1.,-1.56742097575041));
#41865=CARTESIAN_POINT('Ctrl Pts',(-3.51418598431733,-1.,-1.57181569799774));
#41866=CARTESIAN_POINT('Ctrl Pts',(-3.52021847865961,-1.,-1.5763104998818));
#41867=CARTESIAN_POINT('Ctrl Pts',(-3.52626275334899,-1.,-1.58088027227856));
#41868=CARTESIAN_POINT('Ctrl Pts',(-3.53226378147068,-1.,-1.58549906268083));
#41869=CARTESIAN_POINT('Ctrl Pts',(-3.53818616861045,-1.,-1.59014958368725));
#41870=CARTESIAN_POINT('Ctrl Pts',(-3.544024581823,-1.,-1.5948276694975));
#41871=CARTESIAN_POINT('Ctrl Pts',(-3.54979148634426,-1.,-1.59953698113444));
#41872=CARTESIAN_POINT('Ctrl Pts',(-3.55550985096117,-1.,-1.60428584699848));
#41873=CARTESIAN_POINT('Ctrl Pts',(-3.56120432482986,-1.,-1.60908344685459));
#41874=CARTESIAN_POINT('Ctrl Pts',(-3.56689200468404,-1.,-1.61393581747522));
#41875=CARTESIAN_POINT('Ctrl Pts',(-3.57257679609826,-1.,-1.61884340915412));
#41876=CARTESIAN_POINT('Ctrl Pts',(-3.57825455954405,-1.,-1.62380329464851));
#41877=CARTESIAN_POINT('Ctrl Pts',(-3.5839162577435,-1.,-1.62881051550748));
#41878=CARTESIAN_POINT('Ctrl Pts',(-3.58955176627876,-1.,-1.63385971451259));
#41879=CARTESIAN_POINT('Ctrl Pts',(-3.59515368334887,-1.,-1.63894676675349));
#41880=CARTESIAN_POINT('Ctrl Pts',(-3.6007202851384,-1.,-1.6440700438558));
#41881=CARTESIAN_POINT('Ctrl Pts',(-3.60625346556992,-1.,-1.64922952425833));
#41882=CARTESIAN_POINT('Ctrl Pts',(-3.61175734965129,-1.,-1.65442619244327));
#41883=CARTESIAN_POINT('Ctrl Pts',(-3.61723666482457,-1.,-1.65966133399186));
#41884=CARTESIAN_POINT('Ctrl Pts',(-3.62269517989104,-1.,-1.66493585923853));
#41885=CARTESIAN_POINT('Ctrl Pts',(-3.62813422105257,-1.,-1.67024966008037));
#41886=CARTESIAN_POINT('Ctrl Pts',(-3.63355343201211,-1.,-1.67560193613145));
#41887=CARTESIAN_POINT('Ctrl Pts',(-3.63895140887443,-1.,-1.68099146651577));
#41888=CARTESIAN_POINT('Ctrl Pts',(-3.64432638915199,-1.,-1.68641690471455));
#41889=CARTESIAN_POINT('Ctrl Pts',(-3.64967689827393,-1.,-1.691877054817));
#41890=CARTESIAN_POINT('Ctrl Pts',(-3.65500246526798,-1.,-1.69737117722558));
#41891=CARTESIAN_POINT('Ctrl Pts',(-3.6603033877491,-1.,-1.70289888566904));
#41892=CARTESIAN_POINT('Ctrl Pts',(-3.6655804319893,-1.,-1.70846001610983));
#41893=CARTESIAN_POINT('Ctrl Pts',(-3.67083454901629,-1.,-1.71405450210392));
#41894=CARTESIAN_POINT('Ctrl Pts',(-3.67606660374665,-1.,-1.71968225581787));
#41895=CARTESIAN_POINT('Ctrl Pts',(-3.68127704936472,-1.,-1.72534302437003));
#41896=CARTESIAN_POINT('Ctrl Pts',(-3.68646597019188,-1.,-1.73103640956647));
#41897=CARTESIAN_POINT('Ctrl Pts',(-3.69163322647906,-1.,-1.73676193254493));
#41898=CARTESIAN_POINT('Ctrl Pts',(-3.6967785691046,-1.,-1.74251908492589));
#41899=CARTESIAN_POINT('Ctrl Pts',(-3.70190175673422,-1.,-1.74830738046092));
#41900=CARTESIAN_POINT('Ctrl Pts',(-3.70700269736876,-1.,-1.75412641804148));
#41901=CARTESIAN_POINT('Ctrl Pts',(-3.71208146346454,-1.,-1.75997588499021));
#41902=CARTESIAN_POINT('Ctrl Pts',(-3.71713822377675,-1.,-1.76585552124549));
#41903=CARTESIAN_POINT('Ctrl Pts',(-3.72217319911429,-1.,-1.77176509401846));
#41904=CARTESIAN_POINT('Ctrl Pts',(-3.72718661205504,-1.,-1.77770437039606));
#41905=CARTESIAN_POINT('Ctrl Pts',(-3.73217863095022,-1.,-1.78367308442682));
#41906=CARTESIAN_POINT('Ctrl Pts',(-3.73714934729962,-1.,-1.78967092823139));
#41907=CARTESIAN_POINT('Ctrl Pts',(-3.74209880351667,-1.,-1.79569757859041));
#41908=CARTESIAN_POINT('Ctrl Pts',(-3.74702700874954,-1.,-1.80175271485519));
#41909=CARTESIAN_POINT('Ctrl Pts',(-3.75193395888069,-1.,-1.80783603939662));
#41910=CARTESIAN_POINT('Ctrl Pts',(-3.75681965683995,-1.,-1.81394729834032));
#41911=CARTESIAN_POINT('Ctrl Pts',(-3.76168412709652,-1.,-1.82008629694924));
#41912=CARTESIAN_POINT('Ctrl Pts',(-3.76652740355856,-1.,-1.82625289221933));
#41913=CARTESIAN_POINT('Ctrl Pts',(-3.77038509819777,-1.,-1.83120816956515));
#41914=CARTESIAN_POINT('Ctrl Pts',(-3.77326886065484,-1.,-1.83493697935064));
#41915=CARTESIAN_POINT('Ctrl Pts',(-3.77518714458232,-1.,-1.83742834010821));
#41916=CARTESIAN_POINT('Ctrl Pts',(-3.77614523045147,-1.,-1.83867539237861));
#41917=CARTESIAN_POINT('',(-3.70708211654725,-1.,-1.97421938526992));
#41918=CARTESIAN_POINT('',(-3.77614523045147,-1.,-1.83867539237861));
#41919=CARTESIAN_POINT('',(-3.24413672884902,-1.,-1.88097764062542));
#41920=CARTESIAN_POINT('Ctrl Pts',(-3.70708211654725,-1.,-1.97421938526992));
#41921=CARTESIAN_POINT('Ctrl Pts',(-3.7055100813194,-1.,-1.974177276451));
#41922=CARTESIAN_POINT('Ctrl Pts',(-3.70236698911837,-1.,-1.97408973726149));
#41923=CARTESIAN_POINT('Ctrl Pts',(-3.69765528558292,-1.,-1.97394846382288));
#41924=CARTESIAN_POINT('Ctrl Pts',(-3.69137888597855,-1.,-1.97374016224397));
#41925=CARTESIAN_POINT('Ctrl Pts',(-3.68354319913416,-1.,-1.9734465030363));
#41926=CARTESIAN_POINT('Ctrl Pts',(-3.67571738106175,-1.,-1.97311947678035));
#41927=CARTESIAN_POINT('Ctrl Pts',(-3.66790152751984,-1.,-1.9727589719863));
#41928=CARTESIAN_POINT('Ctrl Pts',(-3.66009578166865,-1.,-1.97236485439317));
#41929=CARTESIAN_POINT('Ctrl Pts',(-3.65230034717364,-1.,-1.97193697240645));
#41930=CARTESIAN_POINT('Ctrl Pts',(-3.64451546724221,-1.,-1.97147515441539));
#41931=CARTESIAN_POINT('Ctrl Pts',(-3.63674139590853,-1.,-1.97097920454698));
#41932=CARTESIAN_POINT('Ctrl Pts',(-3.62897836973397,-1.,-1.97044889850518));
#41933=CARTESIAN_POINT('Ctrl Pts',(-3.62122658401722,-1.,-1.96988398129888));
#41934=CARTESIAN_POINT('Ctrl Pts',(-3.61348615496393,-1.,-1.96928416040712));
#41935=CARTESIAN_POINT('Ctrl Pts',(-3.60575714017676,-1.,-1.96864911885775));
#41936=CARTESIAN_POINT('Ctrl Pts',(-3.59803959819725,-1.,-1.96797854118257));
#41937=CARTESIAN_POINT('Ctrl Pts',(-3.5903336402273,-1.,-1.96727213799507));
#41938=CARTESIAN_POINT('Ctrl Pts',(-3.58263947663884,-1.,-1.9665296668894));
#41939=CARTESIAN_POINT('Ctrl Pts',(-3.57495748601088,-1.,-1.96575096652857));
#41940=CARTESIAN_POINT('Ctrl Pts',(-3.56728820357933,-1.,-1.96493594634643));
#41941=CARTESIAN_POINT('Ctrl Pts',(-3.55963218706201,-1.,-1.96408450906868));
#41942=CARTESIAN_POINT('Ctrl Pts',(-3.55198990600929,-1.,-1.96319648628667));
#41943=CARTESIAN_POINT('Ctrl Pts',(-3.54436163300425,-1.,-1.96227157573058));
#41944=CARTESIAN_POINT('Ctrl Pts',(-3.53674730625759,-1.,-1.96130926212661));
#41945=CARTESIAN_POINT('Ctrl Pts',(-3.52914648844289,-1.,-1.96030879411534));
#41946=CARTESIAN_POINT('Ctrl Pts',(-3.52155867431438,-1.,-1.95926936324436));
#41947=CARTESIAN_POINT('Ctrl Pts',(-3.51398354617772,-1.,-1.95819025316768));
#41948=CARTESIAN_POINT('Ctrl Pts',(-3.50642124159913,-1.,-1.95707099606513));
#41949=CARTESIAN_POINT('Ctrl Pts',(-3.49887263575602,-1.,-1.9559115382367));
#41950=CARTESIAN_POINT('Ctrl Pts',(-3.49133956289154,-1.,-1.95471236969653));
#41951=CARTESIAN_POINT('Ctrl Pts',(-3.48382414832648,-1.,-1.95347412486316));
#41952=CARTESIAN_POINT('Ctrl Pts',(-3.47632820495926,-1.,-1.95219722189878));
#41953=CARTESIAN_POINT('Ctrl Pts',(-3.4688525897419,-1.,-1.95088147859876));
#41954=CARTESIAN_POINT('Ctrl Pts',(-3.46139661060959,-1.,-1.94952575850196));
#41955=CARTESIAN_POINT('Ctrl Pts',(-3.45395731584051,-1.,-1.94812754766524));
#41956=CARTESIAN_POINT('Ctrl Pts',(-3.44653088665685,-1.,-1.94668377715332));
#41957=CARTESIAN_POINT('Ctrl Pts',(-3.43911410197693,-1.,-1.94519168842883));
#41958=CARTESIAN_POINT('Ctrl Pts',(-3.43170586602436,-1.,-1.94364973660285));
#41959=CARTESIAN_POINT('Ctrl Pts',(-3.42430850941497,-1.,-1.94205835913692));
#41960=CARTESIAN_POINT('Ctrl Pts',(-3.41692971994082,-1.,-1.94042111965237));
#41961=CARTESIAN_POINT('Ctrl Pts',(-3.40957978266622,-1.,-1.93874306008132));
#41962=CARTESIAN_POINT('Ctrl Pts',(-3.40226802104093,-1.,-1.93702857723089));
#41963=CARTESIAN_POINT('Ctrl Pts',(-3.39499923640789,-1.,-1.93527929945982));
#41964=CARTESIAN_POINT('Ctrl Pts',(-3.38777076883267,-1.,-1.93349233176794));
#41965=CARTESIAN_POINT('Ctrl Pts',(-3.38056768525577,-1.,-1.93165739093292));
#41966=CARTESIAN_POINT('Ctrl Pts',(-3.37336807068078,-1.,-1.92975993109897));
#41967=CARTESIAN_POINT('Ctrl Pts',(-3.36615168657597,-1.,-1.92778626543803));
#41968=CARTESIAN_POINT('Ctrl Pts',(-3.35890824422976,-1.,-1.92572846125763));
#41969=CARTESIAN_POINT('Ctrl Pts',(-3.35164424847206,-1.,-1.92358838440518));
#41970=CARTESIAN_POINT('Ctrl Pts',(-3.34439448941915,-1.,-1.92138450828378));
#41971=CARTESIAN_POINT('Ctrl Pts',(-3.33721230709948,-1.,-1.91914609610173));
#41972=CARTESIAN_POINT('Ctrl Pts',(-3.33014884257812,-1.,-1.91690081930297));
#41973=CARTESIAN_POINT('Ctrl Pts',(-3.32323403454507,-1.,-1.91466343916612));
#41974=CARTESIAN_POINT('Ctrl Pts',(-3.31646052426395,-1.,-1.91242616234459));
#41975=CARTESIAN_POINT('Ctrl Pts',(-3.30975721158694,-1.,-1.91014297830502));
#41976=CARTESIAN_POINT('Ctrl Pts',(-3.30300595568341,-1.,-1.90773912171424));
#41977=CARTESIAN_POINT('Ctrl Pts',(-3.29608978722258,-1.,-1.9051389186417));
#41978=CARTESIAN_POINT('Ctrl Pts',(-3.28893448600364,-1.,-1.9022897124757));
#41979=CARTESIAN_POINT('Ctrl Pts',(-3.28154737912287,-1.,-1.89918429230424));
#41980=CARTESIAN_POINT('Ctrl Pts',(-3.27407108932908,-1.,-1.89589172903662));
#41981=CARTESIAN_POINT('Ctrl Pts',(-3.2667765388833,-1.,-1.89255393500769));
#41982=CARTESIAN_POINT('Ctrl Pts',(-3.2599988519361,-1.,-1.88934996203508));
#41983=CARTESIAN_POINT('Ctrl Pts',(-3.25408686339298,-1.,-1.88646802523372));
#41984=CARTESIAN_POINT('Ctrl Pts',(-3.24935200512055,-1.,-1.88407708646435));
#41985=CARTESIAN_POINT('Ctrl Pts',(-3.24625654410705,-1.,-1.88242596600422));
#41986=CARTESIAN_POINT('Ctrl Pts',(-3.24480754675942,-1.,-1.88156537699118));
#41987=CARTESIAN_POINT('Ctrl Pts',(-3.24428080352952,-1.,-1.88117508446657));
#41988=CARTESIAN_POINT('Ctrl Pts',(-3.24415531671311,-1.,-1.88102292397987));
#41989=CARTESIAN_POINT('Ctrl Pts',(-3.24413672884902,-1.,-1.88097764062542));
#41990=CARTESIAN_POINT('',(-3.14877060440425,-1.,-2.03660101169564));
#41991=CARTESIAN_POINT('Origin',(0.,-1.,0.));
#41992=CARTESIAN_POINT('',(-3.44202241512147,-1.,-2.40675750623143));
#41993=CARTESIAN_POINT('Ctrl Pts',(-3.14877060440425,-1.,-2.03660101169564));
#41994=CARTESIAN_POINT('Ctrl Pts',(-3.1488193908823,-1.,-2.03659701539175));
#41995=CARTESIAN_POINT('Ctrl Pts',(-3.14901193669147,-1.,-2.03663974554941));
#41996=CARTESIAN_POINT('Ctrl Pts',(-3.14959882629936,-1.,-2.03693188810614));
#41997=CARTESIAN_POINT('Ctrl Pts',(-3.15102344775396,-1.,-2.03783225496023));
#41998=CARTESIAN_POINT('Ctrl Pts',(-3.1538999167466,-1.,-2.03984073791432));
#41999=CARTESIAN_POINT('Ctrl Pts',(-3.15817983946525,-1.,-2.04297406404132));
#42000=CARTESIAN_POINT('Ctrl Pts',(-3.16343165059235,-1.,-2.0469333124766));
#42001=CARTESIAN_POINT('Ctrl Pts',(-3.16936341689859,-1.,-2.05151770247452));
#42002=CARTESIAN_POINT('Ctrl Pts',(-3.17564906975592,-1.,-2.05650186773279));
#42003=CARTESIAN_POINT('Ctrl Pts',(-3.18197692964677,-1.,-2.06166849827143));
#42004=CARTESIAN_POINT('Ctrl Pts',(-3.18809755562297,-1.,-2.06684062744065));
#42005=CARTESIAN_POINT('Ctrl Pts',(-3.19388465568113,-1.,-2.07192253497765));
#42006=CARTESIAN_POINT('Ctrl Pts',(-3.19934132835879,-1.,-2.0769044187063));
#42007=CARTESIAN_POINT('Ctrl Pts',(-3.20454818630635,-1.,-2.08182850370816));
#42008=CARTESIAN_POINT('Ctrl Pts',(-3.20962575845433,-1.,-2.08676465517435));
#42009=CARTESIAN_POINT('Ctrl Pts',(-3.2146942960168,-1.,-2.0917841946046));
#42010=CARTESIAN_POINT('Ctrl Pts',(-3.21982707347067,-1.,-2.09692958434933));
#42011=CARTESIAN_POINT('Ctrl Pts',(-3.22503437553496,-1.,-2.10220384298533));
#42012=CARTESIAN_POINT('Ctrl Pts',(-3.23028945793334,-1.,-2.1075869964248));
#42013=CARTESIAN_POINT('Ctrl Pts',(-3.23554444767115,-1.,-2.11304604021784));
#42014=CARTESIAN_POINT('Ctrl Pts',(-3.24074905517282,-1.,-2.11854673326972));
#42015=CARTESIAN_POINT('Ctrl Pts',(-3.24587102613347,-1.,-2.12406646410943));
#42016=CARTESIAN_POINT('Ctrl Pts',(-3.25090574493994,-1.,-2.1296002839681));
#42017=CARTESIAN_POINT('Ctrl Pts',(-3.25586495065027,-1.,-2.13515375878786));
#42018=CARTESIAN_POINT('Ctrl Pts',(-3.26077002641868,-1.,-2.14073870754257));
#42019=CARTESIAN_POINT('Ctrl Pts',(-3.26564388189764,-1.,-2.14636805295663));
#42020=CARTESIAN_POINT('Ctrl Pts',(-3.27050245897244,-1.,-2.15205043199818));
#42021=CARTESIAN_POINT('Ctrl Pts',(-3.27534954469206,-1.,-2.15778690038359));
#42022=CARTESIAN_POINT('Ctrl Pts',(-3.28018150841414,-1.,-2.16357391934434));
#42023=CARTESIAN_POINT('Ctrl Pts',(-3.2849901997973,-1.,-2.16940517773459));
#42024=CARTESIAN_POINT('Ctrl Pts',(-3.28976645712566,-1.,-2.17527380048422));
#42025=CARTESIAN_POINT('Ctrl Pts',(-3.29450361500484,-1.,-2.18117455557062));
#42026=CARTESIAN_POINT('Ctrl Pts',(-3.29920022557635,-1.,-2.18710556500325));
#42027=CARTESIAN_POINT('Ctrl Pts',(-3.30385816281831,-1.,-2.19306710376112));
#42028=CARTESIAN_POINT('Ctrl Pts',(-3.30848134694596,-1.,-2.19906078949924));
#42029=CARTESIAN_POINT('Ctrl Pts',(-3.3130742460895,-1.,-2.20508863150608));
#42030=CARTESIAN_POINT('Ctrl Pts',(-3.31764044024231,-1.,-2.21115211847872));
#42031=CARTESIAN_POINT('Ctrl Pts',(-3.32218125618955,-1.,-2.21725135110889));
#42032=CARTESIAN_POINT('Ctrl Pts',(-3.32669646722871,-1.,-2.22338548312758));
#42033=CARTESIAN_POINT('Ctrl Pts',(-3.33118487773593,-1.,-2.22955308907221));
#42034=CARTESIAN_POINT('Ctrl Pts',(-3.33564495756478,-1.,-2.2357525632881));
#42035=CARTESIAN_POINT('Ctrl Pts',(-3.34007543738044,-1.,-2.24198249391437));
#42036=CARTESIAN_POINT('Ctrl Pts',(-3.34447596770768,-1.,-2.24824207678288));
#42037=CARTESIAN_POINT('Ctrl Pts',(-3.34884690292342,-1.,-2.25453097693524));
#42038=CARTESIAN_POINT('Ctrl Pts',(-3.35318902552676,-1.,-2.26084915222484));
#42039=CARTESIAN_POINT('Ctrl Pts',(-3.35750328523077,-1.,-2.26719668579921));
#42040=CARTESIAN_POINT('Ctrl Pts',(-3.36179055004369,-1.,-2.27357362620902));
#42041=CARTESIAN_POINT('Ctrl Pts',(-3.36605130712978,-1.,-2.27997979457968));
#42042=CARTESIAN_POINT('Ctrl Pts',(-3.37028570206357,-1.,-2.28641481081045));
#42043=CARTESIAN_POINT('Ctrl Pts',(-3.37449367172707,-1.,-2.2928781800731));
#42044=CARTESIAN_POINT('Ctrl Pts',(-3.37867504959382,-1.,-2.29936936127588));
#42045=CARTESIAN_POINT('Ctrl Pts',(-3.38282967336676,-1.,-2.30588783640389));
#42046=CARTESIAN_POINT('Ctrl Pts',(-3.38695751492659,-1.,-2.31243319489505));
#42047=CARTESIAN_POINT('Ctrl Pts',(-3.39105869475112,-1.,-2.31900513925627));
#42048=CARTESIAN_POINT('Ctrl Pts',(-3.39513342020045,-1.,-2.32560343902683));
#42049=CARTESIAN_POINT('Ctrl Pts',(-3.39918194578115,-1.,-2.33222789882601));
#42050=CARTESIAN_POINT('Ctrl Pts',(-3.40320452776646,-1.,-2.33887832342715));
#42051=CARTESIAN_POINT('Ctrl Pts',(-3.40720137403888,-1.,-2.34555447648901));
#42052=CARTESIAN_POINT('Ctrl Pts',(-3.41117262313464,-1.,-2.35225606823649));
#42053=CARTESIAN_POINT('Ctrl Pts',(-3.4151183675076,-1.,-2.35898278606449));
#42054=CARTESIAN_POINT('Ctrl Pts',(-3.41903866635384,-1.,-2.36573431470314));
#42055=CARTESIAN_POINT('Ctrl Pts',(-3.42293356216595,-1.,-2.37251035954351));
#42056=CARTESIAN_POINT('Ctrl Pts',(-3.42680309755241,-1.,-2.37931067029517));
#42057=CARTESIAN_POINT('Ctrl Pts',(-3.43064732714472,-1.,-2.38613505844641));
#42058=CARTESIAN_POINT('Ctrl Pts',(-3.43446630680436,-1.,-2.39298338805823));
#42059=CARTESIAN_POINT('Ctrl Pts',(-3.43750133066036,-1.,-2.39848113411429));
#42060=CARTESIAN_POINT('Ctrl Pts',(-3.43976627485223,-1.,-2.40261515590099));
#42061=CARTESIAN_POINT('Ctrl Pts',(-3.44127120683402,-1.,-2.40537592959345));
#42062=CARTESIAN_POINT('Ctrl Pts',(-3.44202241512147,-1.,-2.40675750623143));
#42063=CARTESIAN_POINT('',(-3.35260583073571,-1.,-2.52982887637028));
#42064=CARTESIAN_POINT('',(-3.44202241512147,-1.,-2.40675750623143));
#42065=CARTESIAN_POINT('',(-2.90994629141676,-1.,-2.36531447826073));
#42066=CARTESIAN_POINT('Ctrl Pts',(-3.35260583073571,-1.,-2.52982887637028));
#42067=CARTESIAN_POINT('Ctrl Pts',(-3.35105973714071,-1.,-2.5295413654909));
#42068=CARTESIAN_POINT('Ctrl Pts',(-3.34796903576663,-1.,-2.52896321610703));
#42069=CARTESIAN_POINT('Ctrl Pts',(-3.34333744115511,-1.,-2.52808660915689));
#42070=CARTESIAN_POINT('Ctrl Pts',(-3.33717089999103,-1.,-2.52689902690158));
#42071=CARTESIAN_POINT('Ctrl Pts',(-3.32947762187533,-1.,-2.52538321164634));
#42072=CARTESIAN_POINT('Ctrl Pts',(-3.32179931078699,-1.,-2.5238359839626));
#42073=CARTESIAN_POINT('Ctrl Pts',(-3.31413607874645,-1.,-2.52225724871313));
#42074=CARTESIAN_POINT('Ctrl Pts',(-3.30648808815442,-1.,-2.52064689568511));
#42075=CARTESIAN_POINT('Ctrl Pts',(-3.29885556388352,-1.,-2.51900480701069));
#42076=CARTESIAN_POINT('Ctrl Pts',(-3.2912387729927,-1.,-2.51733085123797));
#42077=CARTESIAN_POINT('Ctrl Pts',(-3.28363799702982,-1.,-2.51562487464514));
#42078=CARTESIAN_POINT('Ctrl Pts',(-3.27605350473142,-1.,-2.513886692704));
#42079=CARTESIAN_POINT('Ctrl Pts',(-3.26848552888115,-1.,-2.51211608411423));
#42080=CARTESIAN_POINT('Ctrl Pts',(-3.26093423001434,-1.,-2.51031277813486));
#42081=CARTESIAN_POINT('Ctrl Pts',(-3.25339971460982,-1.,-2.50847647070723));
#42082=CARTESIAN_POINT('Ctrl Pts',(-3.24588208983849,-1.,-2.506606859405));
#42083=CARTESIAN_POINT('Ctrl Pts',(-3.23838151080319,-1.,-2.5047036758003));
#42084=CARTESIAN_POINT('Ctrl Pts',(-3.23089822320646,-1.,-2.50276671338111));
#42085=CARTESIAN_POINT('Ctrl Pts',(-3.22343262620503,-1.,-2.50079587201957));
#42086=CARTESIAN_POINT('Ctrl Pts',(-3.21598526261286,-1.,-2.4987911459939));
#42087=CARTESIAN_POINT('Ctrl Pts',(-3.20855669849836,-1.,-2.4967525264737));
#42088=CARTESIAN_POINT('Ctrl Pts',(-3.20114742397588,-1.,-2.49467992057755));
#42089=CARTESIAN_POINT('Ctrl Pts',(-3.19375775555798,-1.,-2.49257307239848));
#42090=CARTESIAN_POINT('Ctrl Pts',(-3.18638771282266,-1.,-2.49043146334059));
#42091=CARTESIAN_POINT('Ctrl Pts',(-3.17903698136622,-1.,-2.48825428288201));
#42092=CARTESIAN_POINT('Ctrl Pts',(-3.17170518863313,-1.,-2.48604065348587));
#42093=CARTESIAN_POINT('Ctrl Pts',(-3.16439213290161,-1.,-2.48378981792725));
#42094=CARTESIAN_POINT('Ctrl Pts',(-3.15709802322739,-1.,-2.48150133566571));
#42095=CARTESIAN_POINT('Ctrl Pts',(-3.14982373241352,-1.,-2.47917529057029));
#42096=CARTESIAN_POINT('Ctrl Pts',(-3.1425709954655,-1.,-2.47681245356109));
#42097=CARTESIAN_POINT('Ctrl Pts',(-3.13534181229295,-1.,-2.47441378371932));
#42098=CARTESIAN_POINT('Ctrl Pts',(-3.12813790805952,-1.,-2.47197997765871));
#42099=CARTESIAN_POINT('Ctrl Pts',(-3.12096015766983,-1.,-2.46951098947469));
#42100=CARTESIAN_POINT('Ctrl Pts',(-3.11380805536122,-1.,-2.46700558843506));
#42101=CARTESIAN_POINT('Ctrl Pts',(-3.1066790790198,-1.,-2.46446082979646));
#42102=CARTESIAN_POINT('Ctrl Pts',(-3.09956993697052,-1.,-2.46187308501884));
#42103=CARTESIAN_POINT('Ctrl Pts',(-3.09247787931887,-1.,-2.4592391256388));
#42104=CARTESIAN_POINT('Ctrl Pts',(-3.08540206545315,-1.,-2.45655725437039));
#42105=CARTESIAN_POINT('Ctrl Pts',(-3.07834472886139,-1.,-2.4538282678779));
#42106=CARTESIAN_POINT('Ctrl Pts',(-3.07131290521297,-1.,-2.45105688854422));
#42107=CARTESIAN_POINT('Ctrl Pts',(-3.06431596421405,-1.,-2.44824970516544));
#42108=CARTESIAN_POINT('Ctrl Pts',(-3.05736242671506,-1.,-2.44541251892556));
#42109=CARTESIAN_POINT('Ctrl Pts',(-3.05045678021504,-1.,-2.44254768923105));
#42110=CARTESIAN_POINT('Ctrl Pts',(-3.04359685040555,-1.,-2.43965194061857));
#42111=CARTESIAN_POINT('Ctrl Pts',(-3.03676949672821,-1.,-2.43671278042414));
#42112=CARTESIAN_POINT('Ctrl Pts',(-3.02995534946978,-1.,-2.43371241361488));
#42113=CARTESIAN_POINT('Ctrl Pts',(-3.02313656036004,-1.,-2.43063415586637));
#42114=CARTESIAN_POINT('Ctrl Pts',(-3.01630420830504,-1.,-2.42746856264168));
#42115=CARTESIAN_POINT('Ctrl Pts',(-3.00946442616658,-1.,-2.42421849439613));
#42116=CARTESIAN_POINT('Ctrl Pts',(-3.00264868585996,-1.,-2.42090763946779));
#42117=CARTESIAN_POINT('Ctrl Pts',(-2.99590509293503,-1.,-2.41757324500514));
#42118=CARTESIAN_POINT('Ctrl Pts',(-2.98927983005796,-1.,-2.41425064199586));
#42119=CARTESIAN_POINT('Ctrl Pts',(-2.98280015815107,-1.,-2.41095909342571));
#42120=CARTESIAN_POINT('Ctrl Pts',(-2.97646002822422,-1.,-2.40768975073713));
#42121=CARTESIAN_POINT('Ctrl Pts',(-2.9701964131236,-1.,-2.40438604734919));
#42122=CARTESIAN_POINT('Ctrl Pts',(-2.96390432240312,-1.,-2.4009556571164));
#42123=CARTESIAN_POINT('Ctrl Pts',(-2.95748006482942,-1.,-2.39730553974517));
#42124=CARTESIAN_POINT('Ctrl Pts',(-2.95085857128439,-1.,-2.39337207631667));
#42125=CARTESIAN_POINT('Ctrl Pts',(-2.94404820669076,-1.,-2.38914929090759));
#42126=CARTESIAN_POINT('Ctrl Pts',(-2.93717903280391,-1.,-2.38472771516311));
#42127=CARTESIAN_POINT('Ctrl Pts',(-2.93049643640206,-1.,-2.38028989582073));
#42128=CARTESIAN_POINT('Ctrl Pts',(-2.92430340582608,-1.,-2.3760651052403));
#42129=CARTESIAN_POINT('Ctrl Pts',(-2.91891503791411,-1.,-2.37229381109821));
#42130=CARTESIAN_POINT('Ctrl Pts',(-2.9146124988314,-1.,-2.36919161373173));
#42131=CARTESIAN_POINT('Ctrl Pts',(-2.91181344022549,-1.,-2.36707658451664));
#42132=CARTESIAN_POINT('Ctrl Pts',(-2.91051690822156,-1.,-2.36599991765749));
#42133=CARTESIAN_POINT('Ctrl Pts',(-2.91005770527719,-1.,-2.36553202948613));
#42134=CARTESIAN_POINT('Ctrl Pts',(-2.90995756655606,-1.,-2.36536211188453));
#42135=CARTESIAN_POINT('Ctrl Pts',(-2.90994629141676,-1.,-2.36531447826074));
#42136=CARTESIAN_POINT('',(-2.79140942341378,-1.,-2.50410331873042));
#42137=CARTESIAN_POINT('Origin',(0.,-1.,0.));
#42138=CARTESIAN_POINT('',(-3.02314558451372,-1.,-2.91557726271063));
#42139=CARTESIAN_POINT('Ctrl Pts',(-2.79140942341378,-1.,-2.50410331873042));
#42140=CARTESIAN_POINT('Ctrl Pts',(-2.79145823440899,-1.,-2.50410700351426));
#42141=CARTESIAN_POINT('Ctrl Pts',(-2.79164172519039,-1.,-2.50417932839343));
#42142=CARTESIAN_POINT('Ctrl Pts',(-2.79217568804874,-1.,-2.50455968395235));
#42143=CARTESIAN_POINT('Ctrl Pts',(-2.79344192164204,-1.,-2.50567182569153));
#42144=CARTESIAN_POINT('Ctrl Pts',(-2.7959687805717,-1.,-2.50810555977564));
#42145=CARTESIAN_POINT('Ctrl Pts',(-2.79970585014308,-1.,-2.51186983687947));
#42146=CARTESIAN_POINT('Ctrl Pts',(-2.80427363984939,-1.,-2.51660190466067));
#42147=CARTESIAN_POINT('Ctrl Pts',(-2.80941521967234,-1.,-2.52205778589922));
#42148=CARTESIAN_POINT('Ctrl Pts',(-2.8148437904867,-1.,-2.52796388055457));
#42149=CARTESIAN_POINT('Ctrl Pts',(-2.82028550483744,-1.,-2.53405679667463));
#42150=CARTESIAN_POINT('Ctrl Pts',(-2.82552167649157,-1.,-2.54012272520141));
#42151=CARTESIAN_POINT('Ctrl Pts',(-2.83044254225794,-1.,-2.54604736792542));
#42152=CARTESIAN_POINT('Ctrl Pts',(-2.83505269592412,-1.,-2.55182152806964));
#42153=CARTESIAN_POINT('Ctrl Pts',(-2.83942515220699,-1.,-2.55749952145165));
#42154=CARTESIAN_POINT('Ctrl Pts',(-2.84366802680211,-1.,-2.56316920798489));
#42155=CARTESIAN_POINT('Ctrl Pts',(-2.84788893329091,-1.,-2.56891984251743));
#42156=CARTESIAN_POINT('Ctrl Pts',(-2.85215360144483,-1.,-2.57480482727128));
#42157=CARTESIAN_POINT('Ctrl Pts',(-2.85647171715147,-1.,-2.58082875254407));
#42158=CARTESIAN_POINT('Ctrl Pts',(-2.86081999003668,-1.,-2.5869677064356));
#42159=CARTESIAN_POINT('Ctrl Pts',(-2.86515629953528,-1.,-2.59318160184921));
#42160=CARTESIAN_POINT('Ctrl Pts',(-2.86943633170712,-1.,-2.59942875223202));
#42161=CARTESIAN_POINT('Ctrl Pts',(-2.87363176656475,-1.,-2.6056817788128));
#42162=CARTESIAN_POINT('Ctrl Pts',(-2.87773881947885,-1.,-2.61193507170928));
#42163=CARTESIAN_POINT('Ctrl Pts',(-2.88176821427502,-1.,-2.61819596473087));
#42164=CARTESIAN_POINT('Ctrl Pts',(-2.88573922195049,-1.,-2.62447947640253));
#42165=CARTESIAN_POINT('Ctrl Pts',(-2.88967244854243,-1.,-2.63080195420771));
#42166=CARTESIAN_POINT('Ctrl Pts',(-2.89358228854557,-1.,-2.63717442263944));
#42167=CARTESIAN_POINT('Ctrl Pts',(-2.89747231723361,-1.,-2.64359851684146));
#42168=CARTESIAN_POINT('Ctrl Pts',(-2.90133950224879,-1.,-2.65007017365576));
#42169=CARTESIAN_POINT('Ctrl Pts',(-2.90517678087467,-1.,-2.65658188464287));
#42170=CARTESIAN_POINT('Ctrl Pts',(-2.90897617968921,-1.,-2.66312542616808));
#42171=CARTESIAN_POINT('Ctrl Pts',(-2.91273193382876,-1.,-2.66969458792627));
#42172=CARTESIAN_POINT('Ctrl Pts',(-2.91644290704281,-1.,-2.67628728855309));
#42173=CARTESIAN_POINT('Ctrl Pts',(-2.92011090722152,-1.,-2.68290409279689));
#42174=CARTESIAN_POINT('Ctrl Pts',(-2.92373955325876,-1.,-2.68954721165342));
#42175=CARTESIAN_POINT('Ctrl Pts',(-2.92733294395268,-1.,-2.69621932864302));
#42176=CARTESIAN_POINT('Ctrl Pts',(-2.93089438233746,-1.,-2.70292247416881));
#42177=CARTESIAN_POINT('Ctrl Pts',(-2.93442516311168,-1.,-2.70965695523776));
#42178=CARTESIAN_POINT('Ctrl Pts',(-2.93792519474955,-1.,-2.71642190053575));
#42179=CARTESIAN_POINT('Ctrl Pts',(-2.94139351933882,-1.,-2.72321571511322));
#42180=CARTESIAN_POINT('Ctrl Pts',(-2.94482887675139,-1.,-2.73003657371613));
#42181=CARTESIAN_POINT('Ctrl Pts',(-2.94823023414381,-1.,-2.73688288329825));
#42182=CARTESIAN_POINT('Ctrl Pts',(-2.95159737214305,-1.,-2.7437537949221));
#42183=CARTESIAN_POINT('Ctrl Pts',(-2.95493069316211,-1.,-2.75064903318996));
#42184=CARTESIAN_POINT('Ctrl Pts',(-2.9582309766594,-1.,-2.75756867888393));
#42185=CARTESIAN_POINT('Ctrl Pts',(-2.96149914764832,-1.,-2.76451296269571));
#42186=CARTESIAN_POINT('Ctrl Pts',(-2.96473605585548,-1.,-2.77148206836464));
#42187=CARTESIAN_POINT('Ctrl Pts',(-2.9679422104295,-1.,-2.77847589542767));
#42188=CARTESIAN_POINT('Ctrl Pts',(-2.97111781461349,-1.,-2.78549409123657));
#42189=CARTESIAN_POINT('Ctrl Pts',(-2.97426288347475,-1.,-2.79253615718147));
#42190=CARTESIAN_POINT('Ctrl Pts',(-2.97737733718242,-1.,-2.79960153278186));
#42191=CARTESIAN_POINT('Ctrl Pts',(-2.98046109647299,-1.,-2.80668968101162));
#42192=CARTESIAN_POINT('Ctrl Pts',(-2.9835141977994,-1.,-2.81380019196454));
#42193=CARTESIAN_POINT('Ctrl Pts',(-2.98653680669434,-1.,-2.82093279065704));
#42194=CARTESIAN_POINT('Ctrl Pts',(-2.98952916401699,-1.,-2.82808728190402));
#42195=CARTESIAN_POINT('Ctrl Pts',(-2.99249155170479,-1.,-2.83526351254383));
#42196=CARTESIAN_POINT('Ctrl Pts',(-2.995424253416,-1.,-2.84246132984334));
#42197=CARTESIAN_POINT('Ctrl Pts',(-2.99832751144566,-1.,-2.84968053289104));
#42198=CARTESIAN_POINT('Ctrl Pts',(-3.0012015079552,-1.,-2.85692085715129));
#42199=CARTESIAN_POINT('Ctrl Pts',(-3.00404638316245,-1.,-2.86418200833065));
#42200=CARTESIAN_POINT('Ctrl Pts',(-3.00686224485374,-1.,-2.87146368430104));
#42201=CARTESIAN_POINT('Ctrl Pts',(-3.0096491810855,-1.,-2.87876560072799));
#42202=CARTESIAN_POINT('Ctrl Pts',(-3.01240727309568,-1.,-2.88608751706796));
#42203=CARTESIAN_POINT('Ctrl Pts',(-3.01513660433291,-1.,-2.8934292556764));
#42204=CARTESIAN_POINT('Ctrl Pts',(-3.01783725123646,-1.,-2.90079069102661));
#42205=CARTESIAN_POINT('Ctrl Pts',(-3.01997487194926,-1.,-2.90669553303902));
#42206=CARTESIAN_POINT('Ctrl Pts',(-3.02156522743299,-1.,-2.91113297349052));
#42207=CARTESIAN_POINT('Ctrl Pts',(-3.02261975104912,-1.,-2.91409518070707));
#42208=CARTESIAN_POINT('Ctrl Pts',(-3.02314558451372,-1.,-2.91557726271063));
#42209=CARTESIAN_POINT('',(-2.91557726271063,-1.,-3.02314558451372));
#42210=CARTESIAN_POINT('',(-3.02314558451372,-1.,-2.91557726271063));
#42211=CARTESIAN_POINT('',(-2.50410331873176,-1.,-2.79140942341258));
#42212=CARTESIAN_POINT('Ctrl Pts',(-2.91557726271063,-1.,-3.02314558451372));
#42213=CARTESIAN_POINT('Ctrl Pts',(-2.91409518070399,-1.,-3.02261975104593));
#42214=CARTESIAN_POINT('Ctrl Pts',(-2.91113297348212,-1.,-3.02156522742431));
#42215=CARTESIAN_POINT('Ctrl Pts',(-2.90669553302526,-1.,-3.01997487193503));
#42216=CARTESIAN_POINT('Ctrl Pts',(-2.9007906910105,-1.,-3.01783725121981));
#42217=CARTESIAN_POINT('Ctrl Pts',(-2.89342925566321,-1.,-3.01513660431928));
#42218=CARTESIAN_POINT('Ctrl Pts',(-2.8860875170608,-1.,-3.01240727308829));
#42219=CARTESIAN_POINT('Ctrl Pts',(-2.87876560072727,-1.,-3.00964918108476));
#42220=CARTESIAN_POINT('Ctrl Pts',(-2.87146368430502,-1.,-3.00686224485784));
#42221=CARTESIAN_POINT('Ctrl Pts',(-2.86418200833667,-1.,-3.00404638316867));
#42222=CARTESIAN_POINT('Ctrl Pts',(-2.85692085715686,-1.,-3.00120150796095));
#42223=CARTESIAN_POINT('Ctrl Pts',(-2.84968053289451,-1.,-2.99832751144925));
#42224=CARTESIAN_POINT('Ctrl Pts',(-2.84246132984415,-1.,-2.99542425341685));
#42225=CARTESIAN_POINT('Ctrl Pts',(-2.83526351254248,-1.,-2.99249155170339));
#42226=CARTESIAN_POINT('Ctrl Pts',(-2.82808728190157,-1.,-2.98952916401446));
#42227=CARTESIAN_POINT('Ctrl Pts',(-2.82093279065457,-1.,-2.9865368066918));
#42228=CARTESIAN_POINT('Ctrl Pts',(-2.81380019196286,-1.,-2.98351419779767));
#42229=CARTESIAN_POINT('Ctrl Pts',(-2.80668968101106,-1.,-2.98046109647241));
#42230=CARTESIAN_POINT('Ctrl Pts',(-2.7996015327823,-1.,-2.97737733718287));
#42231=CARTESIAN_POINT('Ctrl Pts',(-2.79253615718248,-1.,-2.9742628834758));
#42232=CARTESIAN_POINT('Ctrl Pts',(-2.78549409123769,-1.,-2.97111781461465));
#42233=CARTESIAN_POINT('Ctrl Pts',(-2.7784758954285,-1.,-2.96794221043036));
#42234=CARTESIAN_POINT('Ctrl Pts',(-2.77148206836498,-1.,-2.96473605585583));
#42235=CARTESIAN_POINT('Ctrl Pts',(-2.76451296269557,-1.,-2.96149914764818));
#42236=CARTESIAN_POINT('Ctrl Pts',(-2.7575686788835,-1.,-2.95823097665896));
#42237=CARTESIAN_POINT('Ctrl Pts',(-2.75064903318947,-1.,-2.95493069316161));
#42238=CARTESIAN_POINT('Ctrl Pts',(-2.74375379492172,-1.,-2.95159737214266));
#42239=CARTESIAN_POINT('Ctrl Pts',(-2.73688288329808,-1.,-2.94823023414364));
#42240=CARTESIAN_POINT('Ctrl Pts',(-2.73003657371617,-1.,-2.94482887675143));
#42241=CARTESIAN_POINT('Ctrl Pts',(-2.72321571511337,-1.,-2.94139351933897));
#42242=CARTESIAN_POINT('Ctrl Pts',(-2.71642190053592,-1.,-2.93792519474972));
#42243=CARTESIAN_POINT('Ctrl Pts',(-2.70965695523787,-1.,-2.93442516311179));
#42244=CARTESIAN_POINT('Ctrl Pts',(-2.70292247416885,-1.,-2.93089438233749));
#42245=CARTESIAN_POINT('Ctrl Pts',(-2.69621932864301,-1.,-2.92733294395267));
#42246=CARTESIAN_POINT('Ctrl Pts',(-2.68954721165339,-1.,-2.92373955325875));
#42247=CARTESIAN_POINT('Ctrl Pts',(-2.68290409279688,-1.,-2.92011090722152));
#42248=CARTESIAN_POINT('Ctrl Pts',(-2.67628728855312,-1.,-2.91644290704285));
#42249=CARTESIAN_POINT('Ctrl Pts',(-2.66969458792631,-1.,-2.91273193382882));
#42250=CARTESIAN_POINT('Ctrl Pts',(-2.6631254261681,-1.,-2.90897617968923));
#42251=CARTESIAN_POINT('Ctrl Pts',(-2.65658188464282,-1.,-2.90517678087461));
#42252=CARTESIAN_POINT('Ctrl Pts',(-2.65007017365564,-1.,-2.90133950224867));
#42253=CARTESIAN_POINT('Ctrl Pts',(-2.64359851684131,-1.,-2.89747231723345));
#42254=CARTESIAN_POINT('Ctrl Pts',(-2.63717442263932,-1.,-2.89358228854544));
#42255=CARTESIAN_POINT('Ctrl Pts',(-2.63080195420767,-1.,-2.88967244854239));
#42256=CARTESIAN_POINT('Ctrl Pts',(-2.62447947640262,-1.,-2.88573922195059));
#42257=CARTESIAN_POINT('Ctrl Pts',(-2.61819596473108,-1.,-2.88176821427525));
#42258=CARTESIAN_POINT('Ctrl Pts',(-2.61193507170955,-1.,-2.87773881947915));
#42259=CARTESIAN_POINT('Ctrl Pts',(-2.60568177881303,-1.,-2.87363176656501));
#42260=CARTESIAN_POINT('Ctrl Pts',(-2.5994287522321,-1.,-2.86943633170722));
#42261=CARTESIAN_POINT('Ctrl Pts',(-2.59318160184908,-1.,-2.86515629953513));
#42262=CARTESIAN_POINT('Ctrl Pts',(-2.58696770643524,-1.,-2.86081999003629));
#42263=CARTESIAN_POINT('Ctrl Pts',(-2.58082875254357,-1.,-2.85647171715092));
#42264=CARTESIAN_POINT('Ctrl Pts',(-2.57480482727081,-1.,-2.85215360144431));
#42265=CARTESIAN_POINT('Ctrl Pts',(-2.56891984251721,-1.,-2.84788893329067));
#42266=CARTESIAN_POINT('Ctrl Pts',(-2.56316920798513,-1.,-2.84366802680237));
#42267=CARTESIAN_POINT('Ctrl Pts',(-2.55749952145241,-1.,-2.83942515220782));
#42268=CARTESIAN_POINT('Ctrl Pts',(-2.55182152807077,-1.,-2.83505269592536));
#42269=CARTESIAN_POINT('Ctrl Pts',(-2.54604736792655,-1.,-2.83044254225917));
#42270=CARTESIAN_POINT('Ctrl Pts',(-2.54012272520199,-1.,-2.8255216764922));
#42271=CARTESIAN_POINT('Ctrl Pts',(-2.53405679667412,-1.,-2.82028550483689));
#42272=CARTESIAN_POINT('Ctrl Pts',(-2.52796388055278,-1.,-2.81484379048475));
#42273=CARTESIAN_POINT('Ctrl Pts',(-2.52205778589653,-1.,-2.80941521966941));
#42274=CARTESIAN_POINT('Ctrl Pts',(-2.51660190465805,-1.,-2.80427363984653));
#42275=CARTESIAN_POINT('Ctrl Pts',(-2.51186983687818,-1.,-2.79970585014168));
#42276=CARTESIAN_POINT('Ctrl Pts',(-2.50810555977671,-1.,-2.79596878057287));
#42277=CARTESIAN_POINT('Ctrl Pts',(-2.50567182569081,-1.,-2.79344192164147));
#42278=CARTESIAN_POINT('Ctrl Pts',(-2.50455968395146,-1.,-2.79217568804755));
#42279=CARTESIAN_POINT('Ctrl Pts',(-2.50417932839313,-1.,-2.79164172518905));
#42280=CARTESIAN_POINT('Ctrl Pts',(-2.50410700351493,-1.,-2.79145823440781));
#42281=CARTESIAN_POINT('Ctrl Pts',(-2.50410331873176,-1.,-2.79140942341258));
#42282=CARTESIAN_POINT('',(-2.36531447826213,-1.,-2.90994629141562));
#42283=CARTESIAN_POINT('Origin',(0.,-1.,0.));
#42284=CARTESIAN_POINT('',(-2.52982887637028,-1.,-3.35260583073571));
#42285=CARTESIAN_POINT('Ctrl Pts',(-2.36531447826213,-1.,-2.90994629141562));
#42286=CARTESIAN_POINT('Ctrl Pts',(-2.3653621118858,-1.,-2.90995756655558));
#42287=CARTESIAN_POINT('Ctrl Pts',(-2.36553202948741,-1.,-2.9100577052777));
#42288=CARTESIAN_POINT('Ctrl Pts',(-2.36599991765853,-1.,-2.91051690822262));
#42289=CARTESIAN_POINT('Ctrl Pts',(-2.36707658451709,-1.,-2.91181344022628));
#42290=CARTESIAN_POINT('Ctrl Pts',(-2.36919161373074,-1.,-2.91461249883016));
#42291=CARTESIAN_POINT('Ctrl Pts',(-2.37229381109939,-1.,-2.9189150379156));
#42292=CARTESIAN_POINT('Ctrl Pts',(-2.37606510524271,-1.,-2.92430340582912));
#42293=CARTESIAN_POINT('Ctrl Pts',(-2.3802898958232,-1.,-2.93049643640517));
#42294=CARTESIAN_POINT('Ctrl Pts',(-2.38472771516476,-1.,-2.93717903280599));
#42295=CARTESIAN_POINT('Ctrl Pts',(-2.38914929090806,-1.,-2.94404820669135));
#42296=CARTESIAN_POINT('Ctrl Pts',(-2.39337207631613,-1.,-2.95085857128372));
#42297=CARTESIAN_POINT('Ctrl Pts',(-2.39730553974412,-1.,-2.95748006482811));
#42298=CARTESIAN_POINT('Ctrl Pts',(-2.40095565711535,-1.,-2.96390432240181));
#42299=CARTESIAN_POINT('Ctrl Pts',(-2.40438604734848,-1.,-2.97019641312272));
#42300=CARTESIAN_POINT('Ctrl Pts',(-2.40768975073691,-1.,-2.97646002822395));
#42301=CARTESIAN_POINT('Ctrl Pts',(-2.41095909342591,-1.,-2.98280015815132));
#42302=CARTESIAN_POINT('Ctrl Pts',(-2.4142506419963,-1.,-2.98927983005851));
#42303=CARTESIAN_POINT('Ctrl Pts',(-2.4175732450056,-1.,-2.99590509293561));
#42304=CARTESIAN_POINT('Ctrl Pts',(-2.42090763946812,-1.,-3.00264868586038));
#42305=CARTESIAN_POINT('Ctrl Pts',(-2.42421849439625,-1.,-3.00946442616674));
#42306=CARTESIAN_POINT('Ctrl Pts',(-2.4274685626416,-1.,-3.01630420830494));
#42307=CARTESIAN_POINT('Ctrl Pts',(-2.43063415586615,-1.,-3.02313656035977));
#42308=CARTESIAN_POINT('Ctrl Pts',(-2.43371241361462,-1.,-3.02995534946946));
#42309=CARTESIAN_POINT('Ctrl Pts',(-2.43671278042394,-1.,-3.03676949672797));
#42310=CARTESIAN_POINT('Ctrl Pts',(-2.43965194061849,-1.,-3.04359685040545));
#42311=CARTESIAN_POINT('Ctrl Pts',(-2.44254768923109,-1.,-3.05045678021509));
#42312=CARTESIAN_POINT('Ctrl Pts',(-2.44541251892568,-1.,-3.05736242671521));
#42313=CARTESIAN_POINT('Ctrl Pts',(-2.44824970516558,-1.,-3.06431596421422));
#42314=CARTESIAN_POINT('Ctrl Pts',(-2.45105688854432,-1.,-3.0713129052131));
#42315=CARTESIAN_POINT('Ctrl Pts',(-2.45382826787795,-1.,-3.07834472886145));
#42316=CARTESIAN_POINT('Ctrl Pts',(-2.45655725437037,-1.,-3.08540206545313));
#42317=CARTESIAN_POINT('Ctrl Pts',(-2.45923912563875,-1.,-3.09247787931881));
#42318=CARTESIAN_POINT('Ctrl Pts',(-2.4618730850188,-1.,-3.09956993697048));
#42319=CARTESIAN_POINT('Ctrl Pts',(-2.46446082979645,-1.,-3.10667907901981));
#42320=CARTESIAN_POINT('Ctrl Pts',(-2.46700558843507,-1.,-3.11380805536124));
#42321=CARTESIAN_POINT('Ctrl Pts',(-2.4695109894747,-1.,-3.12096015766984));
#42322=CARTESIAN_POINT('Ctrl Pts',(-2.47197997765868,-1.,-3.12813790805948));
#42323=CARTESIAN_POINT('Ctrl Pts',(-2.47441378371923,-1.,-3.13534181229282));
#42324=CARTESIAN_POINT('Ctrl Pts',(-2.47681245356095,-1.,-3.14257099546531));
#42325=CARTESIAN_POINT('Ctrl Pts',(-2.47917529057016,-1.,-3.14982373241335));
#42326=CARTESIAN_POINT('Ctrl Pts',(-2.48150133566568,-1.,-3.15709802322735));
#42327=CARTESIAN_POINT('Ctrl Pts',(-2.48378981792739,-1.,-3.16439213290181));
#42328=CARTESIAN_POINT('Ctrl Pts',(-2.48604065348619,-1.,-3.17170518863357));
#42329=CARTESIAN_POINT('Ctrl Pts',(-2.48825428288243,-1.,-3.17903698136679));
#42330=CARTESIAN_POINT('Ctrl Pts',(-2.49043146334095,-1.,-3.18638771282315));
#42331=CARTESIAN_POINT('Ctrl Pts',(-2.4925730723986,-1.,-3.19375775555814));
#42332=CARTESIAN_POINT('Ctrl Pts',(-2.49467992057726,-1.,-3.20114742397549));
#42333=CARTESIAN_POINT('Ctrl Pts',(-2.49675252647298,-1.,-3.2085566984974));
#42334=CARTESIAN_POINT('Ctrl Pts',(-2.49879114599293,-1.,-3.21598526261157));
#42335=CARTESIAN_POINT('Ctrl Pts',(-2.5007958720187,-1.,-3.22343262620387));
#42336=CARTESIAN_POINT('Ctrl Pts',(-2.50276671338074,-1.,-3.23089822320596));
#42337=CARTESIAN_POINT('Ctrl Pts',(-2.50470367580078,-1.,-3.23838151080383));
#42338=CARTESIAN_POINT('Ctrl Pts',(-2.50660685940645,-1.,-3.24588208984042));
#42339=CARTESIAN_POINT('Ctrl Pts',(-2.50847647070936,-1.,-3.25339971461265));
#42340=CARTESIAN_POINT('Ctrl Pts',(-2.51031277813697,-1.,-3.26093423001716));
#42341=CARTESIAN_POINT('Ctrl Pts',(-2.51211608411539,-1.,-3.26848552888271));
#42342=CARTESIAN_POINT('Ctrl Pts',(-2.51388669270329,-1.,-3.27605350473048));
#42343=CARTESIAN_POINT('Ctrl Pts',(-2.51562487464215,-1.,-3.28363799702583));
#42344=CARTESIAN_POINT('Ctrl Pts',(-2.51733085123316,-1.,-3.2912387729863));
#42345=CARTESIAN_POINT('Ctrl Pts',(-2.51900480700548,-1.,-3.29885556387661));
#42346=CARTESIAN_POINT('Ctrl Pts',(-2.52064689568167,-1.,-3.30648808814986));
#42347=CARTESIAN_POINT('Ctrl Pts',(-2.52225724871375,-1.,-3.31413607874727));
#42348=CARTESIAN_POINT('Ctrl Pts',(-2.52383598396878,-1.,-3.32179931079521));
#42349=CARTESIAN_POINT('Ctrl Pts',(-2.52538321165774,-1.,-3.32947762189049));
#42350=CARTESIAN_POINT('Ctrl Pts',(-2.52689902691551,-1.,-3.33717090000955));
#42351=CARTESIAN_POINT('Ctrl Pts',(-2.52808660916879,-1.,-3.34333744117093));
#42352=CARTESIAN_POINT('Ctrl Pts',(-2.5289632161143,-1.,-3.34796903577628));
#42353=CARTESIAN_POINT('Ctrl Pts',(-2.52954136549357,-1.,-3.35105973714426));
#42354=CARTESIAN_POINT('Ctrl Pts',(-2.52982887637028,-1.,-3.35260583073571));
#42355=CARTESIAN_POINT('',(-2.40675750623143,-1.,-3.44202241512147));
#42356=CARTESIAN_POINT('',(-2.52982887637028,-1.,-3.35260583073571));
#42357=CARTESIAN_POINT('',(-2.03660101169715,-1.,-3.14877060440327));
#42358=CARTESIAN_POINT('Ctrl Pts',(-2.40675750623143,-1.,-3.44202241512147));
#42359=CARTESIAN_POINT('Ctrl Pts',(-2.4053759295909,-1.,-3.44127120683039));
#42360=CARTESIAN_POINT('Ctrl Pts',(-2.40261515589405,-1.,-3.43976627484234));
#42361=CARTESIAN_POINT('Ctrl Pts',(-2.39848113410292,-1.,-3.43750133064416));
#42362=CARTESIAN_POINT('Ctrl Pts',(-2.39298338804493,-1.,-3.4344663067854));
#42363=CARTESIAN_POINT('Ctrl Pts',(-2.38613505843552,-1.,-3.4306473271292));
#42364=CARTESIAN_POINT('Ctrl Pts',(-2.37931067028926,-1.,-3.42680309754399));
#42365=CARTESIAN_POINT('Ctrl Pts',(-2.37251035954292,-1.,-3.42293356216511));
#42366=CARTESIAN_POINT('Ctrl Pts',(-2.36573431470642,-1.,-3.41903866635852));
#42367=CARTESIAN_POINT('Ctrl Pts',(-2.35898278606946,-1.,-3.41511836751469));
#42368=CARTESIAN_POINT('Ctrl Pts',(-2.35225606824109,-1.,-3.41117262314119));
#42369=CARTESIAN_POINT('Ctrl Pts',(-2.34555447649188,-1.,-3.40720137404297));
#42370=CARTESIAN_POINT('Ctrl Pts',(-2.33887832342782,-1.,-3.40320452776743));
#42371=CARTESIAN_POINT('Ctrl Pts',(-2.33222789882489,-1.,-3.39918194577956));
#42372=CARTESIAN_POINT('Ctrl Pts',(-2.3256034390248,-1.,-3.39513342019756));
#42373=CARTESIAN_POINT('Ctrl Pts',(-2.31900513925424,-1.,-3.39105869474822));
#42374=CARTESIAN_POINT('Ctrl Pts',(-2.31243319489367,-1.,-3.38695751492462));
#42375=CARTESIAN_POINT('Ctrl Pts',(-2.30588783640343,-1.,-3.3828296733661));
#42376=CARTESIAN_POINT('Ctrl Pts',(-2.29936936127624,-1.,-3.37867504959433));
#42377=CARTESIAN_POINT('Ctrl Pts',(-2.29287818007393,-1.,-3.37449367172826));
#42378=CARTESIAN_POINT('Ctrl Pts',(-2.28641481081137,-1.,-3.37028570206488));
#42379=CARTESIAN_POINT('Ctrl Pts',(-2.27997979458037,-1.,-3.36605130713076));
#42380=CARTESIAN_POINT('Ctrl Pts',(-2.2735736262093,-1.,-3.36179055004409));
#42381=CARTESIAN_POINT('Ctrl Pts',(-2.2671966857991,-1.,-3.35750328523061));
#42382=CARTESIAN_POINT('Ctrl Pts',(-2.26084915222449,-1.,-3.35318902552626));
#42383=CARTESIAN_POINT('Ctrl Pts',(-2.25453097693483,-1.,-3.34884690292285));
#42384=CARTESIAN_POINT('Ctrl Pts',(-2.24824207678256,-1.,-3.34447596770723));
#42385=CARTESIAN_POINT('Ctrl Pts',(-2.24198249391422,-1.,-3.34007543738025));
#42386=CARTESIAN_POINT('Ctrl Pts',(-2.23575256328812,-1.,-3.33564495756482));
#42387=CARTESIAN_POINT('Ctrl Pts',(-2.22955308907233,-1.,-3.33118487773611));
#42388=CARTESIAN_POINT('Ctrl Pts',(-2.22338548312772,-1.,-3.3266964672289));
#42389=CARTESIAN_POINT('Ctrl Pts',(-2.21725135110898,-1.,-3.32218125618968));
#42390=CARTESIAN_POINT('Ctrl Pts',(-2.21115211847875,-1.,-3.31764044024235));
#42391=CARTESIAN_POINT('Ctrl Pts',(-2.20508863150607,-1.,-3.31307424608949));
#42392=CARTESIAN_POINT('Ctrl Pts',(-2.19906078949923,-1.,-3.30848134694595));
#42393=CARTESIAN_POINT('Ctrl Pts',(-2.19306710376111,-1.,-3.30385816281831));
#42394=CARTESIAN_POINT('Ctrl Pts',(-2.18710556500327,-1.,-3.29920022557639));
#42395=CARTESIAN_POINT('Ctrl Pts',(-2.18117455557065,-1.,-3.2945036150049));
#42396=CARTESIAN_POINT('Ctrl Pts',(-2.17527380048423,-1.,-3.28976645712568));
#42397=CARTESIAN_POINT('Ctrl Pts',(-2.16940517773455,-1.,-3.28499019979724));
#42398=CARTESIAN_POINT('Ctrl Pts',(-2.16357391934425,-1.,-3.280181508414));
#42399=CARTESIAN_POINT('Ctrl Pts',(-2.15778690038347,-1.,-3.27534954469187));
#42400=CARTESIAN_POINT('Ctrl Pts',(-2.15205043199808,-1.,-3.27050245897228));
#42401=CARTESIAN_POINT('Ctrl Pts',(-2.1463680529566,-1.,-3.26564388189759));
#42402=CARTESIAN_POINT('Ctrl Pts',(-2.14073870754264,-1.,-3.26077002641879));
#42403=CARTESIAN_POINT('Ctrl Pts',(-2.13515375878803,-1.,-3.25586495065054));
#42404=CARTESIAN_POINT('Ctrl Pts',(-2.12960028396832,-1.,-3.25090574494028));
#42405=CARTESIAN_POINT('Ctrl Pts',(-2.12406646410962,-1.,-3.24587102613376));
#42406=CARTESIAN_POINT('Ctrl Pts',(-2.11854673326979,-1.,-3.24074905517293));
#42407=CARTESIAN_POINT('Ctrl Pts',(-2.11304604021773,-1.,-3.23554444767099));
#42408=CARTESIAN_POINT('Ctrl Pts',(-2.10758699642451,-1.,-3.23028945793289));
#42409=CARTESIAN_POINT('Ctrl Pts',(-2.10220384298492,-1.,-3.22503437553434));
#42410=CARTESIAN_POINT('Ctrl Pts',(-2.09692958434895,-1.,-3.21982707347009));
#42411=CARTESIAN_POINT('Ctrl Pts',(-2.09178419460443,-1.,-3.21469429601654));
#42412=CARTESIAN_POINT('Ctrl Pts',(-2.08676465517455,-1.,-3.20962575845463));
#42413=CARTESIAN_POINT('Ctrl Pts',(-2.08182850370878,-1.,-3.2045481863073));
#42414=CARTESIAN_POINT('Ctrl Pts',(-2.07690441870722,-1.,-3.19934132836019));
#42415=CARTESIAN_POINT('Ctrl Pts',(-2.07192253497857,-1.,-3.19388465568252));
#42416=CARTESIAN_POINT('Ctrl Pts',(-2.06684062744112,-1.,-3.18809755562368));
#42417=CARTESIAN_POINT('Ctrl Pts',(-2.06166849827101,-1.,-3.18197692964614));
#42418=CARTESIAN_POINT('Ctrl Pts',(-2.05650186773132,-1.,-3.17564906975371));
#42419=CARTESIAN_POINT('Ctrl Pts',(-2.05151770247233,-1.,-3.16936341689527));
#42420=CARTESIAN_POINT('Ctrl Pts',(-2.04693331247446,-1.,-3.16343165058912));
#42421=CARTESIAN_POINT('Ctrl Pts',(-2.04297406404027,-1.,-3.15817983946367));
#42422=CARTESIAN_POINT('Ctrl Pts',(-2.03984073791519,-1.,-3.15389991674792));
#42423=CARTESIAN_POINT('Ctrl Pts',(-2.03783225495961,-1.,-3.15102344775328));
#42424=CARTESIAN_POINT('Ctrl Pts',(-2.03693188810544,-1.,-3.14959882629805));
#42425=CARTESIAN_POINT('Ctrl Pts',(-2.03663974554932,-1.,-3.1490119366901));
#42426=CARTESIAN_POINT('Ctrl Pts',(-2.03659701539259,-1.,-3.14881939088124));
#42427=CARTESIAN_POINT('Ctrl Pts',(-2.03660101169715,-1.,-3.14877060440328));
#42428=CARTESIAN_POINT('',(-1.88097764062697,-1.,-3.24413672884812));
#42429=CARTESIAN_POINT('Origin',(0.,-1.,0.));
#42430=CARTESIAN_POINT('',(-1.97421938526992,-1.,-3.70708211654725));
#42431=CARTESIAN_POINT('Ctrl Pts',(-1.88097764062697,-1.,-3.24413672884812));
#42432=CARTESIAN_POINT('Ctrl Pts',(-1.8810229239812,-1.,-3.24415531671284));
#42433=CARTESIAN_POINT('Ctrl Pts',(-1.88117508446775,-1.,-3.24428080353022));
#42434=CARTESIAN_POINT('Ctrl Pts',(-1.88156537699203,-1.,-3.24480754676064));
#42435=CARTESIAN_POINT('Ctrl Pts',(-1.88242596600454,-1.,-3.2462565441079));
#42436=CARTESIAN_POINT('Ctrl Pts',(-1.88407708646357,-1.,-3.24935200511918));
#42437=CARTESIAN_POINT('Ctrl Pts',(-1.88646802523466,-1.,-3.25408686339463));
#42438=CARTESIAN_POINT('Ctrl Pts',(-1.88934996203698,-1.,-3.25999885193947));
#42439=CARTESIAN_POINT('Ctrl Pts',(-1.89255393500965,-1.,-3.26677653888676));
#42440=CARTESIAN_POINT('Ctrl Pts',(-1.89589172903793,-1.,-3.27407108933139));
#42441=CARTESIAN_POINT('Ctrl Pts',(-1.89918429230462,-1.,-3.28154737912352));
#42442=CARTESIAN_POINT('Ctrl Pts',(-1.90228971247527,-1.,-3.2889344860029));
#42443=CARTESIAN_POINT('Ctrl Pts',(-1.90513891864087,-1.,-3.29608978722113));
#42444=CARTESIAN_POINT('Ctrl Pts',(-1.90773912171341,-1.,-3.30300595568195));
#42445=CARTESIAN_POINT('Ctrl Pts',(-1.91014297830446,-1.,-3.30975721158596));
#42446=CARTESIAN_POINT('Ctrl Pts',(-1.91242616234442,-1.,-3.31646052426364));
#42447=CARTESIAN_POINT('Ctrl Pts',(-1.91466343916628,-1.,-3.32323403454535));
#42448=CARTESIAN_POINT('Ctrl Pts',(-1.91690081930331,-1.,-3.33014884257873));
#42449=CARTESIAN_POINT('Ctrl Pts',(-1.9191460961021,-1.,-3.33721230710012));
#42450=CARTESIAN_POINT('Ctrl Pts',(-1.92138450828404,-1.,-3.34439448941961));
#42451=CARTESIAN_POINT('Ctrl Pts',(-1.92358838440528,-1.,-3.35164424847223));
#42452=CARTESIAN_POINT('Ctrl Pts',(-1.92572846125756,-1.,-3.35890824422965));
#42453=CARTESIAN_POINT('Ctrl Pts',(-1.92778626543786,-1.,-3.36615168657567));
#42454=CARTESIAN_POINT('Ctrl Pts',(-1.92975993109877,-1.,-3.37336807068043));
#42455=CARTESIAN_POINT('Ctrl Pts',(-1.93165739093276,-1.,-3.3805676852555));
#42456=CARTESIAN_POINT('Ctrl Pts',(-1.93349233176788,-1.,-3.38777076883256));
#42457=CARTESIAN_POINT('Ctrl Pts',(-1.93527929945985,-1.,-3.39499923640795));
#42458=CARTESIAN_POINT('Ctrl Pts',(-1.93702857723098,-1.,-3.40226802104109));
#42459=CARTESIAN_POINT('Ctrl Pts',(-1.93874306008143,-1.,-3.40957978266642));
#42460=CARTESIAN_POINT('Ctrl Pts',(-1.94042111965246,-1.,-3.41692971994096));
#42461=CARTESIAN_POINT('Ctrl Pts',(-1.94205835913696,-1.,-3.42430850941503));
#42462=CARTESIAN_POINT('Ctrl Pts',(-1.94364973660284,-1.,-3.43170586602434));
#42463=CARTESIAN_POINT('Ctrl Pts',(-1.94519168842879,-1.,-3.43911410197687));
#42464=CARTESIAN_POINT('Ctrl Pts',(-1.94668377715329,-1.,-3.44653088665681));
#42465=CARTESIAN_POINT('Ctrl Pts',(-1.94812754766524,-1.,-3.45395731584051));
#42466=CARTESIAN_POINT('Ctrl Pts',(-1.94952575850197,-1.,-3.46139661060962));
#42467=CARTESIAN_POINT('Ctrl Pts',(-1.95088147859877,-1.,-3.46885258974191));
#42468=CARTESIAN_POINT('Ctrl Pts',(-1.95219722189876,-1.,-3.47632820495921));
#42469=CARTESIAN_POINT('Ctrl Pts',(-1.95347412486309,-1.,-3.48382414832634));
#42470=CARTESIAN_POINT('Ctrl Pts',(-1.95471236969643,-1.,-3.49133956289133));
#42471=CARTESIAN_POINT('Ctrl Pts',(-1.95591153823661,-1.,-3.49887263575583));
#42472=CARTESIAN_POINT('Ctrl Pts',(-1.95707099606511,-1.,-3.50642124159909));
#42473=CARTESIAN_POINT('Ctrl Pts',(-1.95819025316779,-1.,-3.51398354617794));
#42474=CARTESIAN_POINT('Ctrl Pts',(-1.95926936324461,-1.,-3.52155867431486));
#42475=CARTESIAN_POINT('Ctrl Pts',(-1.96030879411566,-1.,-3.52914648844351));
#42476=CARTESIAN_POINT('Ctrl Pts',(-1.96130926212689,-1.,-3.53674730625813));
#42477=CARTESIAN_POINT('Ctrl Pts',(-1.96227157573067,-1.,-3.54436163300443));
#42478=CARTESIAN_POINT('Ctrl Pts',(-1.96319648628644,-1.,-3.55198990600886));
#42479=CARTESIAN_POINT('Ctrl Pts',(-1.96408450906812,-1.,-3.55963218706096));
#42480=CARTESIAN_POINT('Ctrl Pts',(-1.96493594634567,-1.,-3.56728820357791));
#42481=CARTESIAN_POINT('Ctrl Pts',(-1.96575096652789,-1.,-3.57495748600959));
#42482=CARTESIAN_POINT('Ctrl Pts',(-1.96652966688911,-1.,-3.58263947663829));
#42483=CARTESIAN_POINT('Ctrl Pts',(-1.96727213799544,-1.,-3.59033364022801));
#42484=CARTESIAN_POINT('Ctrl Pts',(-1.96797854118369,-1.,-3.59803959819938));
#42485=CARTESIAN_POINT('Ctrl Pts',(-1.9686491188594,-1.,-3.60575714017989));
#42486=CARTESIAN_POINT('Ctrl Pts',(-1.96928416040877,-1.,-3.61348615496704));
#42487=CARTESIAN_POINT('Ctrl Pts',(-1.96988398129978,-1.,-3.62122658401893));
#42488=CARTESIAN_POINT('Ctrl Pts',(-1.97044889850463,-1.,-3.62897836973293));
#42489=CARTESIAN_POINT('Ctrl Pts',(-1.97097920454464,-1.,-3.63674139590412));
#42490=CARTESIAN_POINT('Ctrl Pts',(-1.97147515441164,-1.,-3.64451546723514));
#42491=CARTESIAN_POINT('Ctrl Pts',(-1.9719369724024,-1.,-3.652300347166));
#42492=CARTESIAN_POINT('Ctrl Pts',(-1.9723648543905,-1.,-3.6600957816636));
#42493=CARTESIAN_POINT('Ctrl Pts',(-1.97275897198678,-1.,-3.66790152752075));
#42494=CARTESIAN_POINT('Ctrl Pts',(-1.97311947678517,-1.,-3.67571738107084));
#42495=CARTESIAN_POINT('Ctrl Pts',(-1.97344650304519,-1.,-3.68354319915092));
#42496=CARTESIAN_POINT('Ctrl Pts',(-1.97374016225483,-1.,-3.69137888599902));
#42497=CARTESIAN_POINT('Ctrl Pts',(-1.97394846383216,-1.,-3.6976552856004));
#42498=CARTESIAN_POINT('Ctrl Pts',(-1.97408973726715,-1.,-3.70236698912904));
#42499=CARTESIAN_POINT('Ctrl Pts',(-1.97417727645308,-1.,-3.70551008132332));
#42500=CARTESIAN_POINT('Ctrl Pts',(-1.97421938526992,-1.,-3.70708211654725));
#42501=CARTESIAN_POINT('',(-1.83867539237861,-1.,-3.77614523045147));
#42502=CARTESIAN_POINT('',(-1.97421938526992,-1.,-3.70708211654725));
#42503=CARTESIAN_POINT('',(-1.5189508286633,-1.,-3.42859860294306));
#42504=CARTESIAN_POINT('Ctrl Pts',(-1.83867539237861,-1.,-3.77614523045147));
#42505=CARTESIAN_POINT('Ctrl Pts',(-1.83742834010626,-1.,-3.77518714457833));
#42506=CARTESIAN_POINT('Ctrl Pts',(-1.83493697934534,-1.,-3.77326886064398));
#42507=CARTESIAN_POINT('Ctrl Pts',(-1.83120816955645,-1.,-3.77038509817999));
#42508=CARTESIAN_POINT('Ctrl Pts',(-1.82625289220915,-1.,-3.76652740353775));
#42509=CARTESIAN_POINT('Ctrl Pts',(-1.82008629694091,-1.,-3.76168412707948));
#42510=CARTESIAN_POINT('Ctrl Pts',(-1.8139472983358,-1.,-3.75681965683071));
#42511=CARTESIAN_POINT('Ctrl Pts',(-1.80783603939617,-1.,-3.75193395887977));
#42512=CARTESIAN_POINT('Ctrl Pts',(-1.8017527148577,-1.,-3.74702700875467));
#42513=CARTESIAN_POINT('Ctrl Pts',(-1.79569757859422,-1.,-3.74209880352445));
#42514=CARTESIAN_POINT('Ctrl Pts',(-1.78967092823491,-1.,-3.73714934730681));
#42515=CARTESIAN_POINT('Ctrl Pts',(-1.78367308442901,-1.,-3.7321786309547));
#42516=CARTESIAN_POINT('Ctrl Pts',(-1.77770437039658,-1.,-3.72718661205609));
#42517=CARTESIAN_POINT('Ctrl Pts',(-1.77176509401761,-1.,-3.72217319911254));
#42518=CARTESIAN_POINT('Ctrl Pts',(-1.76585552124394,-1.,-3.71713822377359));
#42519=CARTESIAN_POINT('Ctrl Pts',(-1.75997588498865,-1.,-3.71208146346136));
#42520=CARTESIAN_POINT('Ctrl Pts',(-1.75412641804042,-1.,-3.70700269736659));
#42521=CARTESIAN_POINT('Ctrl Pts',(-1.74830738046057,-1.,-3.7019017567335));
#42522=CARTESIAN_POINT('Ctrl Pts',(-1.74251908492617,-1.,-3.69677856910517));
#42523=CARTESIAN_POINT('Ctrl Pts',(-1.73676193254557,-1.,-3.69163322648036));
#42524=CARTESIAN_POINT('Ctrl Pts',(-1.73103640956717,-1.,-3.68646597019332));
#42525=CARTESIAN_POINT('Ctrl Pts',(-1.72534302437056,-1.,-3.68127704936579));
#42526=CARTESIAN_POINT('Ctrl Pts',(-1.71968225581808,-1.,-3.67606660374709));
#42527=CARTESIAN_POINT('Ctrl Pts',(-1.71405450210384,-1.,-3.67083454901611));
#42528=CARTESIAN_POINT('Ctrl Pts',(-1.70846001610956,-1.,-3.66558043198876));
#42529=CARTESIAN_POINT('Ctrl Pts',(-1.70289888566873,-1.,-3.66030338774847));
#42530=CARTESIAN_POINT('Ctrl Pts',(-1.69737117722534,-1.,-3.65500246526749));
#42531=CARTESIAN_POINT('Ctrl Pts',(-1.69187705481689,-1.,-3.64967689827371));
#42532=CARTESIAN_POINT('Ctrl Pts',(-1.68641690471457,-1.,-3.64432638915203));
#42533=CARTESIAN_POINT('Ctrl Pts',(-1.68099146651586,-1.,-3.63895140887462));
#42534=CARTESIAN_POINT('Ctrl Pts',(-1.67560193613156,-1.,-3.63355343201232));
#42535=CARTESIAN_POINT('Ctrl Pts',(-1.67024966008045,-1.,-3.62813422105271));
#42536=CARTESIAN_POINT('Ctrl Pts',(-1.66493585923855,-1.,-3.62269517989109));
#42537=CARTESIAN_POINT('Ctrl Pts',(-1.65966133399186,-1.,-3.61723666482456));
#42538=CARTESIAN_POINT('Ctrl Pts',(-1.65442619244325,-1.,-3.61175734965127));
#42539=CARTESIAN_POINT('Ctrl Pts',(-1.64922952425832,-1.,-3.60625346556992));
#42540=CARTESIAN_POINT('Ctrl Pts',(-1.64407004385582,-1.,-3.60072028513845));
#42541=CARTESIAN_POINT('Ctrl Pts',(-1.63894676675352,-1.,-3.59515368334893));
#42542=CARTESIAN_POINT('Ctrl Pts',(-1.6338597145126,-1.,-3.58955176627879));
#42543=CARTESIAN_POINT('Ctrl Pts',(-1.62881051550745,-1.,-3.58391625774343));
#42544=CARTESIAN_POINT('Ctrl Pts',(-1.62380329464844,-1.,-3.5782545595439));
#42545=CARTESIAN_POINT('Ctrl Pts',(-1.61884340915404,-1.,-3.57257679609806));
#42546=CARTESIAN_POINT('Ctrl Pts',(-1.61393581747514,-1.,-3.56689200468387));
#42547=CARTESIAN_POINT('Ctrl Pts',(-1.60908344685457,-1.,-3.5612043248298));
#42548=CARTESIAN_POINT('Ctrl Pts',(-1.60428584699853,-1.,-3.55550985096129));
#42549=CARTESIAN_POINT('Ctrl Pts',(-1.59953698113457,-1.,-3.54979148634454));
#42550=CARTESIAN_POINT('Ctrl Pts',(-1.59482766949766,-1.,-3.54402458182337));
#42551=CARTESIAN_POINT('Ctrl Pts',(-1.59014958368739,-1.,-3.53818616861077));
#42552=CARTESIAN_POINT('Ctrl Pts',(-1.58549906268088,-1.,-3.5322637814708));
#42553=CARTESIAN_POINT('Ctrl Pts',(-1.58088027227848,-1.,-3.52626275334881));
#42554=CARTESIAN_POINT('Ctrl Pts',(-1.57631049988158,-1.,-3.52021847865912));
#42555=CARTESIAN_POINT('Ctrl Pts',(-1.57181569799743,-1.,-3.51418598431665));
#42556=CARTESIAN_POINT('Ctrl Pts',(-1.56742097575012,-1.,-3.50821771695363));
#42557=CARTESIAN_POINT('Ctrl Pts',(-1.56314187758675,-1.,-3.50234321621578));
#42558=CARTESIAN_POINT('Ctrl Pts',(-1.55897703097874,-1.,-3.49655185179655));
#42559=CARTESIAN_POINT('Ctrl Pts',(-1.55489595901116,-1.,-3.4907646087742));
#42560=CARTESIAN_POINT('Ctrl Pts',(-1.55084702970452,-1.,-3.48485155928567));
#42561=CARTESIAN_POINT('Ctrl Pts',(-1.54678009290276,-1.,-3.47868272898751));
#42562=CARTESIAN_POINT('Ctrl Pts',(-1.54266605398187,-1.,-3.47217189224653));
#42563=CARTESIAN_POINT('Ctrl Pts',(-1.53851507915502,-1.,-3.46531752207153));
#42564=CARTESIAN_POINT('Ctrl Pts',(-1.53440195378792,-1.,-3.45825932955032));
#42565=CARTESIAN_POINT('Ctrl Pts',(-1.53046244461635,-1.,-3.45127136828305));
#42566=CARTESIAN_POINT('Ctrl Pts',(-1.52686242875556,-1.,-3.44469547526647));
#42567=CARTESIAN_POINT('Ctrl Pts',(-1.5237734895035,-1.,-3.4388889597401));
#42568=CARTESIAN_POINT('Ctrl Pts',(-1.52134826724293,-1.,-3.43417156977893));
#42569=CARTESIAN_POINT('Ctrl Pts',(-1.5198144909338,-1.,-3.43101631893414));
#42570=CARTESIAN_POINT('Ctrl Pts',(-1.51914806898491,-1.,-3.42946838852587));
#42571=CARTESIAN_POINT('Ctrl Pts',(-1.5189513329503,-1.,-3.42884302333841));
#42572=CARTESIAN_POINT('Ctrl Pts',(-1.51893924967331,-1.,-3.42864616361875));
#42573=CARTESIAN_POINT('Ctrl Pts',(-1.5189508286633,-1.,-3.42859860294306));
#42574=CARTESIAN_POINT('',(-1.35032489087269,-1.,-3.49844575334386));
#42575=CARTESIAN_POINT('Origin',(0.,-1.,0.));
#42576=CARTESIAN_POINT('',(-1.36999806084572,-1.,-3.97027773754922));
#42577=CARTESIAN_POINT('Ctrl Pts',(-1.35032489087269,-1.,-3.49844575334386));
#42578=CARTESIAN_POINT('Ctrl Pts',(-1.35036670893102,-1.,-3.49847119623841));
#42579=CARTESIAN_POINT('Ctrl Pts',(-1.35049736560633,-1.,-3.49861894124915));
#42580=CARTESIAN_POINT('Ctrl Pts',(-1.35080045218652,-1.,-3.49920025459856));
#42581=CARTESIAN_POINT('Ctrl Pts',(-1.35142377279535,-1.,-3.5007660381658));
#42582=CARTESIAN_POINT('Ctrl Pts',(-1.3525703284343,-1.,-3.50408168106113));
#42583=CARTESIAN_POINT('Ctrl Pts',(-1.35419113576022,-1.,-3.50913227060177));
#42584=CARTESIAN_POINT('Ctrl Pts',(-1.35611275237288,-1.,-3.51542230699919));
#42585=CARTESIAN_POINT('Ctrl Pts',(-1.35821701528975,-1.,-3.52261776117121));
#42586=CARTESIAN_POINT('Ctrl Pts',(-1.36037259643827,-1.,-3.53034464961849));
#42587=CARTESIAN_POINT('Ctrl Pts',(-1.36245507339334,-1.,-3.53824396425032));
#42588=CARTESIAN_POINT('Ctrl Pts',(-1.36436666257567,-1.,-3.54602591832893));
#42589=CARTESIAN_POINT('Ctrl Pts',(-1.36606145456711,-1.,-3.55353883995793));
#42590=CARTESIAN_POINT('Ctrl Pts',(-1.36754771771174,-1.,-3.56077662028492));
#42591=CARTESIAN_POINT('Ctrl Pts',(-1.36886584973349,-1.,-3.56782080304554));
#42592=CARTESIAN_POINT('Ctrl Pts',(-1.37007229485646,-1.,-3.57479875549453));
#42593=CARTESIAN_POINT('Ctrl Pts',(-1.37122241663073,-1.,-3.58183885982745));
#42594=CARTESIAN_POINT('Ctrl Pts',(-1.37235053661,-1.,-3.5890185384643));
#42595=CARTESIAN_POINT('Ctrl Pts',(-1.37346320103184,-1.,-3.59634627869117));
#42596=CARTESIAN_POINT('Ctrl Pts',(-1.37455051379642,-1.,-3.60379020124038));
#42597=CARTESIAN_POINT('Ctrl Pts',(-1.37559314436641,-1.,-3.61129546591082));
#42598=CARTESIAN_POINT('Ctrl Pts',(-1.37657053403102,-1.,-3.61880481160408));
#42599=CARTESIAN_POINT('Ctrl Pts',(-1.37746987919868,-1.,-3.62628098665112));
#42600=CARTESIAN_POINT('Ctrl Pts',(-1.37829035457324,-1.,-3.63371727442448));
#42601=CARTESIAN_POINT('Ctrl Pts',(-1.37903818567347,-1.,-3.64112507791112));
#42602=CARTESIAN_POINT('Ctrl Pts',(-1.37972372481598,-1.,-3.64852652756444));
#42603=CARTESIAN_POINT('Ctrl Pts',(-1.38035791051215,-1.,-3.65594554404396));
#42604=CARTESIAN_POINT('Ctrl Pts',(-1.38094856333558,-1.,-3.66339848520874));
#42605=CARTESIAN_POINT('Ctrl Pts',(-1.38149812653876,-1.,-3.67088843112282));
#42606=CARTESIAN_POINT('Ctrl Pts',(-1.38200574290626,-1.,-3.6784103848243));
#42607=CARTESIAN_POINT('Ctrl Pts',(-1.38246852827185,-1.,-3.68595444983844));
#42608=CARTESIAN_POINT('Ctrl Pts',(-1.38288311171649,-1.,-3.69350967899523));
#42609=CARTESIAN_POINT('Ctrl Pts',(-1.38324717612862,-1.,-3.70106792167894));
#42610=CARTESIAN_POINT('Ctrl Pts',(-1.38356065402122,-1.,-3.70862680753343));
#42611=CARTESIAN_POINT('Ctrl Pts',(-1.38382489984585,-1.,-3.7161876605181));
#42612=CARTESIAN_POINT('Ctrl Pts',(-1.3840421342895,-1.,-3.72375409358805));
#42613=CARTESIAN_POINT('Ctrl Pts',(-1.38421479111531,-1.,-3.73133035859283));
#42614=CARTESIAN_POINT('Ctrl Pts',(-1.38434489156456,-1.,-3.73891976418099));
#42615=CARTESIAN_POINT('Ctrl Pts',(-1.38443344984389,-1.,-3.7465231716786));
#42616=CARTESIAN_POINT('Ctrl Pts',(-1.38448077997155,-1.,-3.75413976318727));
#42617=CARTESIAN_POINT('Ctrl Pts',(-1.38448675253343,-1.,-3.76176768271347));
#42618=CARTESIAN_POINT('Ctrl Pts',(-1.38445107339517,-1.,-3.76940473185775));
#42619=CARTESIAN_POINT('Ctrl Pts',(-1.38437354551435,-1.,-3.77704902230441));
#42620=CARTESIAN_POINT('Ctrl Pts',(-1.38425435883773,-1.,-3.78469969805134));
#42621=CARTESIAN_POINT('Ctrl Pts',(-1.38409399694589,-1.,-3.79235669640907));
#42622=CARTESIAN_POINT('Ctrl Pts',(-1.38389311766701,-1.,-3.80002044322169));
#42623=CARTESIAN_POINT('Ctrl Pts',(-1.38365244046226,-1.,-3.80769156398429));
#42624=CARTESIAN_POINT('Ctrl Pts',(-1.38337263902766,-1.,-3.81537060817765));
#42625=CARTESIAN_POINT('Ctrl Pts',(-1.38305421262724,-1.,-3.82305771743715));
#42626=CARTESIAN_POINT('Ctrl Pts',(-1.38269750245086,-1.,-3.83075266982138));
#42627=CARTESIAN_POINT('Ctrl Pts',(-1.38230274828774,-1.,-3.83845502790609));
#42628=CARTESIAN_POINT('Ctrl Pts',(-1.38187013346089,-1.,-3.84616425605705));
#42629=CARTESIAN_POINT('Ctrl Pts',(-1.38139983115075,-1.,-3.85387983979557));
#42630=CARTESIAN_POINT('Ctrl Pts',(-1.38089205993067,-1.,-3.86160143044187));
#42631=CARTESIAN_POINT('Ctrl Pts',(-1.38034709213129,-1.,-3.86932885813403));
#42632=CARTESIAN_POINT('Ctrl Pts',(-1.37976523097187,-1.,-3.87706205830865));
#42633=CARTESIAN_POINT('Ctrl Pts',(-1.37914679719446,-1.,-3.88480102249461));
#42634=CARTESIAN_POINT('Ctrl Pts',(-1.37849211287981,-1.,-3.89254574338385));
#42635=CARTESIAN_POINT('Ctrl Pts',(-1.3778014851263,-1.,-3.90029615196255));
#42636=CARTESIAN_POINT('Ctrl Pts',(-1.3770751963376,-1.,-3.90805209522729));
#42637=CARTESIAN_POINT('Ctrl Pts',(-1.37631350505516,-1.,-3.91581337461825));
#42638=CARTESIAN_POINT('Ctrl Pts',(-1.37551664448057,-1.,-3.92357976987132));
#42639=CARTESIAN_POINT('Ctrl Pts',(-1.37468482215784,-1.,-3.93135106761941));
#42640=CARTESIAN_POINT('Ctrl Pts',(-1.37381821967499,-1.,-3.93912709041791));
#42641=CARTESIAN_POINT('Ctrl Pts',(-1.37291699203423,-1.,-3.94690771786926));
#42642=CARTESIAN_POINT('Ctrl Pts',(-1.37198126433139,-1.,-3.95469287283105));
#42643=CARTESIAN_POINT('Ctrl Pts',(-1.37120515615663,-1.,-3.96092458508407));
#42644=CARTESIAN_POINT('Ctrl Pts',(-1.37060761746027,-1.,-3.96560037975788));
#42645=CARTESIAN_POINT('Ctrl Pts',(-1.37020239094758,-1.,-3.9687184694173));
#42646=CARTESIAN_POINT('Ctrl Pts',(-1.36999806084572,-1.,-3.97027773754922));
#42647=CARTESIAN_POINT('',(-1.22531898815164,-1.,-4.01728681790024));
#42648=CARTESIAN_POINT('',(-1.36999806084572,-1.,-3.97027773754922));
#42649=CARTESIAN_POINT('',(-0.963899035118986,-1.,-3.62400312501199));
#42650=CARTESIAN_POINT('Ctrl Pts',(-1.22531898815164,-1.,-4.01728681790024));
#42651=CARTESIAN_POINT('Ctrl Pts',(-1.22423716681317,-1.,-4.01614544569895));
#42652=CARTESIAN_POINT('Ctrl Pts',(-1.22207656455845,-1.,-4.01386104433519));
#42653=CARTESIAN_POINT('Ctrl Pts',(-1.21884478244403,-1.,-4.01042947140789));
#42654=CARTESIAN_POINT('Ctrl Pts',(-1.21455398918133,-1.,-4.00584409522722));
#42655=CARTESIAN_POINT('Ctrl Pts',(-1.20922097029551,-1.,-4.00009577950721));
#42656=CARTESIAN_POINT('Ctrl Pts',(-1.20391852375139,-1.,-3.99433084799666));
#42657=CARTESIAN_POINT('Ctrl Pts',(-1.19864679609566,-1.,-3.98854928957189));
#42658=CARTESIAN_POINT('Ctrl Pts',(-1.19340598349475,-1.,-3.98275111052561));
#42659=CARTESIAN_POINT('Ctrl Pts',(-1.18819633715539,-1.,-3.97693634767754));
#42660=CARTESIAN_POINT('Ctrl Pts',(-1.18301815039831,-1.,-3.97110505165415));
#42661=CARTESIAN_POINT('Ctrl Pts',(-1.17787174135592,-1.,-3.96525726358159));
#42662=CARTESIAN_POINT('Ctrl Pts',(-1.17275743590361,-1.,-3.95939299213276));
#42663=CARTESIAN_POINT('Ctrl Pts',(-1.16767555244438,-1.,-3.95351219509876));
#42664=CARTESIAN_POINT('Ctrl Pts',(-1.16262637999157,-1.,-3.94761474780583));
#42665=CARTESIAN_POINT('Ctrl Pts',(-1.15761018340956,-1.,-3.94170046685203));
#42666=CARTESIAN_POINT('Ctrl Pts',(-1.1526272271632,-1.,-3.9357691705628));
#42667=CARTESIAN_POINT('Ctrl Pts',(-1.14767779451123,-1.,-3.92982073294257));
#42668=CARTESIAN_POINT('Ctrl Pts',(-1.14276220561593,-1.,-3.92385513133997));
#42669=CARTESIAN_POINT('Ctrl Pts',(-1.13788084225554,-1.,-3.91787251936827));
#42670=CARTESIAN_POINT('Ctrl Pts',(-1.13303414693896,-1.,-3.91187321145649));
#42671=CARTESIAN_POINT('Ctrl Pts',(-1.12822258281553,-1.,-3.90585753318737));
#42672=CARTESIAN_POINT('Ctrl Pts',(-1.12344660099043,-1.,-3.89982569750025));
#42673=CARTESIAN_POINT('Ctrl Pts',(-1.11870660794603,-1.,-3.89377768340344));
#42674=CARTESIAN_POINT('Ctrl Pts',(-1.11400292434429,-1.,-3.88771308285171));
#42675=CARTESIAN_POINT('Ctrl Pts',(-1.10933577224008,-1.,-3.88163105531724));
#42676=CARTESIAN_POINT('Ctrl Pts',(-1.10470536603287,-1.,-3.87553067187514));
#42677=CARTESIAN_POINT('Ctrl Pts',(-1.10011198761195,-1.,-3.86941120134849));
#42678=CARTESIAN_POINT('Ctrl Pts',(-1.09555606505013,-1.,-3.86327241021247));
#42679=CARTESIAN_POINT('Ctrl Pts',(-1.09103825516294,-1.,-3.85711487933931));
#42680=CARTESIAN_POINT('Ctrl Pts',(-1.08655950846384,-1.,-3.85094025222713));
#42681=CARTESIAN_POINT('Ctrl Pts',(-1.08212087917991,-1.,-3.8447504803063));
#42682=CARTESIAN_POINT('Ctrl Pts',(-1.07772335353858,-1.,-3.83854714117491));
#42683=CARTESIAN_POINT('Ctrl Pts',(-1.07336766633459,-1.,-3.83233071195144));
#42684=CARTESIAN_POINT('Ctrl Pts',(-1.06905413180359,-1.,-3.82609989967276));
#42685=CARTESIAN_POINT('Ctrl Pts',(-1.0647824403893,-1.,-3.81985083953012));
#42686=CARTESIAN_POINT('Ctrl Pts',(-1.06055206187299,-1.,-3.8135786611749));
#42687=CARTESIAN_POINT('Ctrl Pts',(-1.05636266918644,-1.,-3.80727913637791));
#42688=CARTESIAN_POINT('Ctrl Pts',(-1.05221457990016,-1.,-3.80095039790681));
#42689=CARTESIAN_POINT('Ctrl Pts',(-1.04810913267639,-1.,-3.79459440308786));
#42690=CARTESIAN_POINT('Ctrl Pts',(-1.04404924374422,-1.,-3.78821910787179));
#42691=CARTESIAN_POINT('Ctrl Pts',(-1.04003862055798,-1.,-3.7818353500817));
#42692=CARTESIAN_POINT('Ctrl Pts',(-1.03608074678008,-1.,-3.77545283140427));
#42693=CARTESIAN_POINT('Ctrl Pts',(-1.03217786604919,-1.,-3.76907609832516));
#42694=CARTESIAN_POINT('Ctrl Pts',(-1.02833014458184,-1.,-3.76270122291245));
#42695=CARTESIAN_POINT('Ctrl Pts',(-1.02453429444668,-1.,-3.75631037456224));
#42696=CARTESIAN_POINT('Ctrl Pts',(-1.02078510487439,-1.,-3.74987777155873));
#42697=CARTESIAN_POINT('Ctrl Pts',(-1.01707794311088,-1.,-3.74337942504993));
#42698=CARTESIAN_POINT('Ctrl Pts',(-1.01341114319906,-1.,-3.73680245055747));
#42699=CARTESIAN_POINT('Ctrl Pts',(-1.00978798539491,-1.,-3.73015276704407));
#42700=CARTESIAN_POINT('Ctrl Pts',(-1.00622000735696,-1.,-3.72346803750544));
#42701=CARTESIAN_POINT('Ctrl Pts',(-1.00272423396802,-1.,-3.71680667125047));
#42702=CARTESIAN_POINT('Ctrl Pts',(-0.999317260756344,-1.,-3.7102243971387));
#42703=CARTESIAN_POINT('Ctrl Pts',(-0.996009819772432,-1.,-3.70375282282107));
#42704=CARTESIAN_POINT('Ctrl Pts',(-0.992802218332104,-1.,-3.69738123415696));
#42705=CARTESIAN_POINT('Ctrl Pts',(-0.989676715398858,-1.,-3.69102682138955));
#42706=CARTESIAN_POINT('Ctrl Pts',(-0.986602639864286,-1.,-3.6845531792623));
#42707=CARTESIAN_POINT('Ctrl Pts',(-0.983550791470864,-1.,-3.67782408841876));
#42708=CARTESIAN_POINT('Ctrl Pts',(-0.980505922458494,-1.,-3.67074983340444));
#42709=CARTESIAN_POINT('Ctrl Pts',(-0.977478312751416,-1.,-3.66333049637403));
#42710=CARTESIAN_POINT('Ctrl Pts',(-0.974519971354139,-1.,-3.6557157673487));
#42711=CARTESIAN_POINT('Ctrl Pts',(-0.971722122060277,-1.,-3.64819756447072));
#42712=CARTESIAN_POINT('Ctrl Pts',(-0.969195124674829,-1.,-3.64113946505393));
#42713=CARTESIAN_POINT('Ctrl Pts',(-0.967052554540877,-1.,-3.6349212208096));
#42714=CARTESIAN_POINT('Ctrl Pts',(-0.965395153165716,-1.,-3.62988252139998));
#42715=CARTESIAN_POINT('Ctrl Pts',(-0.964373850166081,-1.,-3.62652618145252));
#42716=CARTESIAN_POINT('Ctrl Pts',(-0.963957782642589,-1.,-3.62489305727516));
#42717=CARTESIAN_POINT('Ctrl Pts',(-0.963861297423579,-1.,-3.62424461507455));
#42718=CARTESIAN_POINT('Ctrl Pts',(-0.963880158556713,-1.,-3.62404828878374));
#42719=CARTESIAN_POINT('Ctrl Pts',(-0.963899035118986,-1.,-3.62400312501199));
#42720=CARTESIAN_POINT('',(-0.786422660833743,-1.,-3.66661143271648));
#42721=CARTESIAN_POINT('Origin',(0.,-1.,0.));
#42722=CARTESIAN_POINT('',(-0.732042837400619,-1.,-4.13571194405636));
#42723=CARTESIAN_POINT('Ctrl Pts',(-0.786422660833743,-1.,-3.66661143271648));
#42724=CARTESIAN_POINT('Ctrl Pts',(-0.786459983896781,-1.,-3.66664310415236));
#42725=CARTESIAN_POINT('Ctrl Pts',(-0.78656591955989,-1.,-3.66680946938396));
#42726=CARTESIAN_POINT('Ctrl Pts',(-0.786774337198499,-1.,-3.66743103898844));
#42727=CARTESIAN_POINT('Ctrl Pts',(-0.787145041181589,-1.,-3.66907505398769));
#42728=CARTESIAN_POINT('Ctrl Pts',(-0.787758799995426,-1.,-3.672529236635));
#42729=CARTESIAN_POINT('Ctrl Pts',(-0.788569566220662,-1.,-3.67777119516438));
#42730=CARTESIAN_POINT('Ctrl Pts',(-0.789483546065158,-1.,-3.68428439784285));
#42731=CARTESIAN_POINT('Ctrl Pts',(-0.79043628498958,-1.,-3.69172044327754));
#42732=CARTESIAN_POINT('Ctrl Pts',(-0.791356575696509,-1.,-3.69968940808982));
#42733=CARTESIAN_POINT('Ctrl Pts',(-0.792177688845968,-1.,-3.70781724021879));
#42734=CARTESIAN_POINT('Ctrl Pts',(-0.792848377370115,-1.,-3.7158024239604));
#42735=CARTESIAN_POINT('Ctrl Pts',(-0.79334702378387,-1.,-3.7234879729357));
#42736=CARTESIAN_POINT('Ctrl Pts',(-0.793682750269347,-1.,-3.7308691469564));
#42737=CARTESIAN_POINT('Ctrl Pts',(-0.79388270093679,-1.,-3.73803280541576));
#42738=CARTESIAN_POINT('Ctrl Pts',(-0.79398270045988,-1.,-3.74511357728827));
#42739=CARTESIAN_POINT('Ctrl Pts',(-0.794017347371441,-1.,-3.75224692493895));
#42740=CARTESIAN_POINT('Ctrl Pts',(-0.794008429135047,-1.,-3.75951468666325));
#42741=CARTESIAN_POINT('Ctrl Pts',(-0.793961083689141,-1.,-3.76692626931184));
#42742=CARTESIAN_POINT('Ctrl Pts',(-0.793870523787515,-1.,-3.77444863801264));
#42743=CARTESIAN_POINT('Ctrl Pts',(-0.793726235781339,-1.,-3.78202460377617));
#42744=CARTESIAN_POINT('Ctrl Pts',(-0.793516871680966,-1.,-3.78959439439222));
#42745=CARTESIAN_POINT('Ctrl Pts',(-0.7932356129732,-1.,-3.79711921389862));
#42746=CARTESIAN_POINT('Ctrl Pts',(-0.792882695234693,-1.,-3.80459229925598));
#42747=CARTESIAN_POINT('Ctrl Pts',(-0.792462483517568,-1.,-3.81202588694726));
#42748=CARTESIAN_POINT('Ctrl Pts',(-0.791981740718606,-1.,-3.81944345442237));
#42749=CARTESIAN_POINT('Ctrl Pts',(-0.791447528662381,-1.,-3.82687033899799));
#42750=CARTESIAN_POINT('Ctrl Pts',(-0.79086501270534,-1.,-3.83432392054804));
#42751=CARTESIAN_POINT('Ctrl Pts',(-0.790236124191289,-1.,-3.84180762342476));
#42752=CARTESIAN_POINT('Ctrl Pts',(-0.789560798155619,-1.,-3.8493163780891));
#42753=CARTESIAN_POINT('Ctrl Pts',(-0.788837734090688,-1.,-3.85683995872536));
#42754=CARTESIAN_POINT('Ctrl Pts',(-0.788065315093771,-1.,-3.86436702561342));
#42755=CARTESIAN_POINT('Ctrl Pts',(-0.78724252761798,-1.,-3.87188916600905));
#42756=CARTESIAN_POINT('Ctrl Pts',(-0.786369675812592,-1.,-3.87940402818186));
#42757=CARTESIAN_POINT('Ctrl Pts',(-0.785447890340723,-1.,-3.88691313167399));
#42758=CARTESIAN_POINT('Ctrl Pts',(-0.784478799358336,-1.,-3.89442039235105));
#42759=CARTESIAN_POINT('Ctrl Pts',(-0.783464141529082,-1.,-3.90193039043971));
#42760=CARTESIAN_POINT('Ctrl Pts',(-0.782405395622759,-1.,-3.90944671004536));
#42761=CARTESIAN_POINT('Ctrl Pts',(-0.781303428618344,-1.,-3.9169703605466));
#42762=CARTESIAN_POINT('Ctrl Pts',(-0.780158678615507,-1.,-3.92450058323799));
#42763=CARTESIAN_POINT('Ctrl Pts',(-0.778971308134786,-1.,-3.93203552473153));
#42764=CARTESIAN_POINT('Ctrl Pts',(-0.77774137056855,-1.,-3.93957296768098));
#42765=CARTESIAN_POINT('Ctrl Pts',(-0.77646896669796,-1.,-3.94711101619471));
#42766=CARTESIAN_POINT('Ctrl Pts',(-0.775154418039441,-1.,-3.95464885452364));
#42767=CARTESIAN_POINT('Ctrl Pts',(-0.773798212026683,-1.,-3.96218649639876));
#42768=CARTESIAN_POINT('Ctrl Pts',(-0.772400931772239,-1.,-3.96972446532832));
#42769=CARTESIAN_POINT('Ctrl Pts',(-0.770963190030504,-1.,-3.97726349165507));
#42770=CARTESIAN_POINT('Ctrl Pts',(-0.769485566245459,-1.,-3.98480422348403));
#42771=CARTESIAN_POINT('Ctrl Pts',(-0.767968531377708,-1.,-3.99234687880892));
#42772=CARTESIAN_POINT('Ctrl Pts',(-0.766412457135786,-1.,-3.99989129179464));
#42773=CARTESIAN_POINT('Ctrl Pts',(-0.764817648784946,-1.,-4.00743706791366));
#42774=CARTESIAN_POINT('Ctrl Pts',(-0.763184371182827,-1.,-4.01498370680434));
#42775=CARTESIAN_POINT('Ctrl Pts',(-0.761512875859942,-1.,-4.02253072741347));
#42776=CARTESIAN_POINT('Ctrl Pts',(-0.759803433244166,-1.,-4.0300778195465));
#42777=CARTESIAN_POINT('Ctrl Pts',(-0.758056338885554,-1.,-4.03762485803468));
#42778=CARTESIAN_POINT('Ctrl Pts',(-0.756271902370187,-1.,-4.04517182654344));
#42779=CARTESIAN_POINT('Ctrl Pts',(-0.754450441816412,-1.,-4.05271876688106));
#42780=CARTESIAN_POINT('Ctrl Pts',(-0.752592276482869,-1.,-4.06026572221399));
#42781=CARTESIAN_POINT('Ctrl Pts',(-0.750697720483176,-1.,-4.06781267241886));
#42782=CARTESIAN_POINT('Ctrl Pts',(-0.748767076679177,-1.,-4.07535951055363));
#42783=CARTESIAN_POINT('Ctrl Pts',(-0.746800631490822,-1.,-4.08290608094789));
#42784=CARTESIAN_POINT('Ctrl Pts',(-0.744798649705514,-1.,-4.09045220253011));
#42785=CARTESIAN_POINT('Ctrl Pts',(-0.742761369690018,-1.,-4.09799769702712));
#42786=CARTESIAN_POINT('Ctrl Pts',(-0.740688998555152,-1.,-4.1055424175856));
#42787=CARTESIAN_POINT('Ctrl Pts',(-0.738581708229119,-1.,-4.11308626953795));
#42788=CARTESIAN_POINT('Ctrl Pts',(-0.736439634335347,-1.,-4.12062919626082));
#42789=CARTESIAN_POINT('Ctrl Pts',(-0.734698226767512,-1.,-4.12666277572794));
#42790=CARTESIAN_POINT('Ctrl Pts',(-0.733376589325634,-1.,-4.13118752796397));
#42791=CARTESIAN_POINT('Ctrl Pts',(-0.732488575135926,-1.,-4.13420383737278));
#42792=CARTESIAN_POINT('Ctrl Pts',(-0.732042837400619,-1.,-4.13571194405636));
#42793=CARTESIAN_POINT('',(-0.581791163835814,-1.,-4.15950947128175));
#42794=CARTESIAN_POINT('',(-0.732042837400619,-1.,-4.13571194405636));
#42795=CARTESIAN_POINT('',(-0.385112848332549,-1.,-3.73017266276632));
#42796=CARTESIAN_POINT('Ctrl Pts',(-0.581791163835814,-1.,-4.15950947128175));
#42797=CARTESIAN_POINT('Ctrl Pts',(-0.580901211462913,-1.,-4.15821291712391));
#42798=CARTESIAN_POINT('Ctrl Pts',(-0.579124568912543,-1.,-4.15561864787379));
#42799=CARTESIAN_POINT('Ctrl Pts',(-0.576469391673917,-1.,-4.1517237611974));
#42800=CARTESIAN_POINT('Ctrl Pts',(-0.572948736066277,-1.,-4.14652361065787));
#42801=CARTESIAN_POINT('Ctrl Pts',(-0.568580610187116,-1.,-4.14001179828669));
#42802=CARTESIAN_POINT('Ctrl Pts',(-0.564245279535705,-1.,-4.13348835726086));
#42803=CARTESIAN_POINT('Ctrl Pts',(-0.559942890594628,-1.,-4.12695329951859));
#42804=CARTESIAN_POINT('Ctrl Pts',(-0.555673636130778,-1.,-4.1204066619623));
#42805=CARTESIAN_POINT('Ctrl Pts',(-0.551437758498247,-1.,-4.11384852025578));
#42806=CARTESIAN_POINT('Ctrl Pts',(-0.54723553948676,-1.,-4.1072789702877));
#42807=CARTESIAN_POINT('Ctrl Pts',(-0.543067286878457,-1.,-4.10069810244473));
#42808=CARTESIAN_POINT('Ctrl Pts',(-0.538933321179921,-1.,-4.09410597627116));
#42809=CARTESIAN_POINT('Ctrl Pts',(-0.534833963476999,-1.,-4.08750259988693));
#42810=CARTESIAN_POINT('Ctrl Pts',(-0.530769518728075,-1.,-4.08088789536488));
#42811=CARTESIAN_POINT('Ctrl Pts',(-0.526740277227,-1.,-4.07426172299496));
#42812=CARTESIAN_POINT('Ctrl Pts',(-0.522746528602768,-1.,-4.06762394471075));
#42813=CARTESIAN_POINT('Ctrl Pts',(-0.51878857233681,-1.,-4.06097448037934));
#42814=CARTESIAN_POINT('Ctrl Pts',(-0.514866728193104,-1.,-4.05431335771261));
#42815=CARTESIAN_POINT('Ctrl Pts',(-0.510981349219174,-1.,-4.04764078815591));
#42816=CARTESIAN_POINT('Ctrl Pts',(-0.507132823288362,-1.,-4.04095715149074));
#42817=CARTESIAN_POINT('Ctrl Pts',(-0.503321556915514,-1.,-4.0342628417439));
#42818=CARTESIAN_POINT('Ctrl Pts',(-0.49954796234089,-1.,-4.0275581398015));
#42819=CARTESIAN_POINT('Ctrl Pts',(-0.495812444326223,-1.,-4.02084308851813));
#42820=CARTESIAN_POINT('Ctrl Pts',(-0.492115383417931,-1.,-4.01411733503486));
#42821=CARTESIAN_POINT('Ctrl Pts',(-0.488457130424531,-1.,-4.0073800839092));
#42822=CARTESIAN_POINT('Ctrl Pts',(-0.484838042421754,-1.,-4.00063045119234));
#42823=CARTESIAN_POINT('Ctrl Pts',(-0.481258512209638,-1.,-3.99386775880655));
#42824=CARTESIAN_POINT('Ctrl Pts',(-0.477718999122033,-1.,-3.98709184306743));
#42825=CARTESIAN_POINT('Ctrl Pts',(-0.474220061019542,-1.,-3.9803033804443));
#42826=CARTESIAN_POINT('Ctrl Pts',(-0.470762379613477,-1.,-3.97350414289415));
#42827=CARTESIAN_POINT('Ctrl Pts',(-0.467346690880672,-1.,-3.96669622273946));
#42828=CARTESIAN_POINT('Ctrl Pts',(-0.463973722115744,-1.,-3.95988133243543));
#42829=CARTESIAN_POINT('Ctrl Pts',(-0.460644124429119,-1.,-3.95306005817363));
#42830=CARTESIAN_POINT('Ctrl Pts',(-0.457358410451674,-1.,-3.94623117206675));
#42831=CARTESIAN_POINT('Ctrl Pts',(-0.454116879027576,-1.,-3.93939080846298));
#42832=CARTESIAN_POINT('Ctrl Pts',(-0.450919768356347,-1.,-3.93253407403128));
#42833=CARTESIAN_POINT('Ctrl Pts',(-0.447767416837297,-1.,-3.92565674143424));
#42834=CARTESIAN_POINT('Ctrl Pts',(-0.444660430230593,-1.,-3.91875701610721));
#42835=CARTESIAN_POINT('Ctrl Pts',(-0.441599824524047,-1.,-3.91183704069146));
#42836=CARTESIAN_POINT('Ctrl Pts',(-0.438587235458233,-1.,-3.90490512938546));
#42837=CARTESIAN_POINT('Ctrl Pts',(-0.435624629433506,-1.,-3.8979725665544));
#42838=CARTESIAN_POINT('Ctrl Pts',(-0.432713929544439,-1.,-3.89104947940592));
#42839=CARTESIAN_POINT('Ctrl Pts',(-0.429856640579734,-1.,-3.88414070943334));
#42840=CARTESIAN_POINT('Ctrl Pts',(-0.427053541173469,-1.,-3.87724240306609));
#42841=CARTESIAN_POINT('Ctrl Pts',(-0.424304173195142,-1.,-3.87033643487882));
#42842=CARTESIAN_POINT('Ctrl Pts',(-0.421607423177576,-1.,-3.86339652542749));
#42843=CARTESIAN_POINT('Ctrl Pts',(-0.41896246808681,-1.,-3.85639825648031));
#42844=CARTESIAN_POINT('Ctrl Pts',(-0.41636967805292,-1.,-3.8493286415751));
#42845=CARTESIAN_POINT('Ctrl Pts',(-0.413831367016727,-1.,-3.84219403994742));
#42846=CARTESIAN_POINT('Ctrl Pts',(-0.41135303879846,-1.,-3.83503345578645));
#42847=CARTESIAN_POINT('Ctrl Pts',(-0.408942371447377,-1.,-3.82790724256397));
#42848=CARTESIAN_POINT('Ctrl Pts',(-0.406607038258906,-1.,-3.82087303913741));
#42849=CARTESIAN_POINT('Ctrl Pts',(-0.404352694628236,-1.,-3.81396374287762));
#42850=CARTESIAN_POINT('Ctrl Pts',(-0.402181320148475,-1.,-3.80716881962763));
#42851=CARTESIAN_POINT('Ctrl Pts',(-0.400088346504727,-1.,-3.80040370384659));
#42852=CARTESIAN_POINT('Ctrl Pts',(-0.398064818684158,-1.,-3.79352887163457));
#42853=CARTESIAN_POINT('Ctrl Pts',(-0.396103205335029,-1.,-3.78640521279479));
#42854=CARTESIAN_POINT('Ctrl Pts',(-0.394202481011595,-1.,-3.77894173114368));
#42855=CARTESIAN_POINT('Ctrl Pts',(-0.392372786223347,-1.,-3.77114011595892));
#42856=CARTESIAN_POINT('Ctrl Pts',(-0.390642072979259,-1.,-3.76315635032993));
#42857=CARTESIAN_POINT('Ctrl Pts',(-0.389054775898251,-1.,-3.75529302894757));
#42858=CARTESIAN_POINT('Ctrl Pts',(-0.387663020050396,-1.,-3.74792651696269));
#42859=CARTESIAN_POINT('Ctrl Pts',(-0.386519576222035,-1.,-3.74144965781088));
#42860=CARTESIAN_POINT('Ctrl Pts',(-0.385670806454744,-1.,-3.73621371845475));
#42861=CARTESIAN_POINT('Ctrl Pts',(-0.385187124633965,-1.,-3.73273893363318));
#42862=CARTESIAN_POINT('Ctrl Pts',(-0.385031656499141,-1.,-3.73106082862399));
#42863=CARTESIAN_POINT('Ctrl Pts',(-0.385037797882046,-1.,-3.73040527620929));
#42864=CARTESIAN_POINT('Ctrl Pts',(-0.385087139001609,-1.,-3.73021431755218));
#42865=CARTESIAN_POINT('Ctrl Pts',(-0.385112848332549,-1.,-3.73017266276632));
#42866=CARTESIAN_POINT('',(-0.203156094897896,-1.,-3.74449296982994));
#42867=CARTESIAN_POINT('Origin',(0.,-1.,0.));
#42868=CARTESIAN_POINT('',(-0.0760622897878238,-1.,-4.19931119685982));
#42869=CARTESIAN_POINT('Ctrl Pts',(-0.203156094897896,-1.,-3.74449296982994));
#42870=CARTESIAN_POINT('Ctrl Pts',(-0.203188003947965,-1.,-3.74453008995129));
#42871=CARTESIAN_POINT('Ctrl Pts',(-0.203266610111264,-1.,-3.74471097893961));
#42872=CARTESIAN_POINT('Ctrl Pts',(-0.203375226874331,-1.,-3.74535749969262));
#42873=CARTESIAN_POINT('Ctrl Pts',(-0.203484186269315,-1.,-3.74703926501843));
#42874=CARTESIAN_POINT('Ctrl Pts',(-0.203550035479097,-1.,-3.75054693397716));
#42875=CARTESIAN_POINT('Ctrl Pts',(-0.203530796848404,-1.,-3.75585118707924));
#42876=CARTESIAN_POINT('Ctrl Pts',(-0.203414634707646,-1.,-3.76242717937273));
#42877=CARTESIAN_POINT('Ctrl Pts',(-0.203192390045337,-1.,-3.76992071595267));
#42878=CARTESIAN_POINT('Ctrl Pts',(-0.202854729699197,-1.,-3.77793553476879));
#42879=CARTESIAN_POINT('Ctrl Pts',(-0.202394260512193,-1.,-3.78609175019317));
#42880=CARTESIAN_POINT('Ctrl Pts',(-0.201807533800799,-1.,-3.79408354187274));
#42881=CARTESIAN_POINT('Ctrl Pts',(-0.201097756307252,-1.,-3.80175247447171));
#42882=CARTESIAN_POINT('Ctrl Pts',(-0.20027467943329,-1.,-3.80909529318501));
#42883=CARTESIAN_POINT('Ctrl Pts',(-0.199351525297396,-1.,-3.81620203429702));
#42884=CARTESIAN_POINT('Ctrl Pts',(-0.19834261690047,-1.,-3.82321127348981));
#42885=CARTESIAN_POINT('Ctrl Pts',(-0.197260935827375,-1.,-3.83026221776488));
#42886=CARTESIAN_POINT('Ctrl Pts',(-0.19611519897189,-1.,-3.83743910616265));
#42887=CARTESIAN_POINT('Ctrl Pts',(-0.194909009460255,-1.,-3.84475203347052));
#42888=CARTESIAN_POINT('Ctrl Pts',(-0.193642806777748,-1.,-3.85216762264019));
#42889=CARTESIAN_POINT('Ctrl Pts',(-0.19231515304498,-1.,-3.85962774407652));
#42890=CARTESIAN_POINT('Ctrl Pts',(-0.190924190418613,-1.,-3.8670715862477));
#42891=CARTESIAN_POINT('Ctrl Pts',(-0.189469253358254,-1.,-3.87445976418377));
#42892=CARTESIAN_POINT('Ctrl Pts',(-0.187951632512663,-1.,-3.88178563496187));
#42893=CARTESIAN_POINT('Ctrl Pts',(-0.186373724985263,-1.,-3.88906196725817));
#42894=CARTESIAN_POINT('Ctrl Pts',(-0.184738537728035,-1.,-3.89631300742633));
#42895=CARTESIAN_POINT('Ctrl Pts',(-0.183049081993193,-1.,-3.90356488555138));
#42896=CARTESIAN_POINT('Ctrl Pts',(-0.181307740731796,-1.,-3.91083557557193));
#42897=CARTESIAN_POINT('Ctrl Pts',(-0.179515885822895,-1.,-3.91812876180948));
#42898=CARTESIAN_POINT('Ctrl Pts',(-0.177674246152328,-1.,-3.92543942697672));
#42899=CARTESIAN_POINT('Ctrl Pts',(-0.175783136893873,-1.,-3.93275726771049));
#42900=CARTESIAN_POINT('Ctrl Pts',(-0.173842734974607,-1.,-3.94007083096214));
#42901=CARTESIAN_POINT('Ctrl Pts',(-0.171853355369233,-1.,-3.94737164900861));
#42902=CARTESIAN_POINT('Ctrl Pts',(-0.16981566637413,-1.,-3.95465744665263));
#42903=CARTESIAN_POINT('Ctrl Pts',(-0.167730547023312,-1.,-3.96192990160296));
#42904=CARTESIAN_POINT('Ctrl Pts',(-0.165598992851098,-1.,-3.9691931362141));
#42905=CARTESIAN_POINT('Ctrl Pts',(-0.163422004609999,-1.,-3.97645194630944));
#42906=CARTESIAN_POINT('Ctrl Pts',(-0.161200482186088,-1.,-3.98371010319866));
#42907=CARTESIAN_POINT('Ctrl Pts',(-0.158935123982796,-1.,-3.99096873945862));
#42908=CARTESIAN_POINT('Ctrl Pts',(-0.156626481393736,-1.,-3.99822717425869));
#42909=CARTESIAN_POINT('Ctrl Pts',(-0.15427500487231,-1.,-4.00548360245297));
#42910=CARTESIAN_POINT('Ctrl Pts',(-0.151881094022909,-1.,-4.01273584234684));
#42911=CARTESIAN_POINT('Ctrl Pts',(-0.149445144968708,-1.,-4.01998203715588));
#42912=CARTESIAN_POINT('Ctrl Pts',(-0.146967602878999,-1.,-4.02722143147048));
#42913=CARTESIAN_POINT('Ctrl Pts',(-0.144448947038352,-1.,-4.03445411510403));
#42914=CARTESIAN_POINT('Ctrl Pts',(-0.141889671485508,-1.,-4.04168069633842));
#42915=CARTESIAN_POINT('Ctrl Pts',(-0.13929026718006,-1.,-4.04890199238056));
#42916=CARTESIAN_POINT('Ctrl Pts',(-0.136651205046111,-1.,-4.05611873400122));
#42917=CARTESIAN_POINT('Ctrl Pts',(-0.133972916144225,-1.,-4.06333121018476));
#42918=CARTESIAN_POINT('Ctrl Pts',(-0.131255793548914,-1.,-4.07053931528579));
#42919=CARTESIAN_POINT('Ctrl Pts',(-0.128500200484814,-1.,-4.07774270738809));
#42920=CARTESIAN_POINT('Ctrl Pts',(-0.125706476822529,-1.,-4.08494093372315));
#42921=CARTESIAN_POINT('Ctrl Pts',(-0.122874946249119,-1.,-4.09213355850836));
#42922=CARTESIAN_POINT('Ctrl Pts',(-0.120005924388162,-1.,-4.09932031767243));
#42923=CARTESIAN_POINT('Ctrl Pts',(-0.117099722731705,-1.,-4.10650113382187));
#42924=CARTESIAN_POINT('Ctrl Pts',(-0.114156649609602,-1.,-4.11367603925313));
#42925=CARTESIAN_POINT('Ctrl Pts',(-0.111177012683377,-1.,-4.12084512502444));
#42926=CARTESIAN_POINT('Ctrl Pts',(-0.10816112052835,-1.,-4.12800848371386));
#42927=CARTESIAN_POINT('Ctrl Pts',(-0.105109286538864,-1.,-4.13516614458396));
#42928=CARTESIAN_POINT('Ctrl Pts',(-0.102021826577454,-1.,-4.14231804938737));
#42929=CARTESIAN_POINT('Ctrl Pts',(-0.0988990478899814,-1.,-4.1494640891762));
#42930=CARTESIAN_POINT('Ctrl Pts',(-0.095741240329707,-1.,-4.15660412653006));
#42931=CARTESIAN_POINT('Ctrl Pts',(-0.0925486672167692,-1.,-4.16373802265942));
#42932=CARTESIAN_POINT('Ctrl Pts',(-0.089321556085033,-1.,-4.17086566491823));
#42933=CARTESIAN_POINT('Ctrl Pts',(-0.0860600915552517,-1.,-4.17798698669991));
#42934=CARTESIAN_POINT('Ctrl Pts',(-0.0827644164389512,-1.,-4.1851019532944));
#42935=CARTESIAN_POINT('Ctrl Pts',(-0.0801005887117605,-1.,-4.19078883322483));
#42936=CARTESIAN_POINT('Ctrl Pts',(-0.0780873956244405,-1.,-4.19505112860624));
#42937=CARTESIAN_POINT('Ctrl Pts',(-0.0767384596142197,-1.,-4.19789138621624));
#42938=CARTESIAN_POINT('Ctrl Pts',(-0.0760622897878238,-1.,-4.19931119685982));
#42939=CARTESIAN_POINT('',(0.0760622897878244,-1.,-4.19931119685982));
#42940=CARTESIAN_POINT('',(-0.0760622897878238,-1.,-4.19931119685982));
#42941=CARTESIAN_POINT('',(0.2031560948961,-1.,-3.74449296983004));
#42942=CARTESIAN_POINT('Ctrl Pts',(0.0760622897878244,-1.,-4.19931119685982));
#42943=CARTESIAN_POINT('Ctrl Pts',(0.0767384596141462,-1.,-4.1978913862118));
#42944=CARTESIAN_POINT('Ctrl Pts',(0.0780873956242395,-1.,-4.19505112859416));
#42945=CARTESIAN_POINT('Ctrl Pts',(0.0801005887114317,-1.,-4.19078883320504));
#42946=CARTESIAN_POINT('Ctrl Pts',(0.0827644164385676,-1.,-4.18510195327123));
#42947=CARTESIAN_POINT('Ctrl Pts',(0.0860600915549394,-1.,-4.17798698668094));
#42948=CARTESIAN_POINT('Ctrl Pts',(0.0893215560848647,-1.,-4.17086566490794));
#42949=CARTESIAN_POINT('Ctrl Pts',(0.0925486672167528,-1.,-4.16373802265839));
#42950=CARTESIAN_POINT('Ctrl Pts',(0.0957412403298004,-1.,-4.15660412653577));
#42951=CARTESIAN_POINT('Ctrl Pts',(0.0988990478901223,-1.,-4.14946408918485));
#42952=CARTESIAN_POINT('Ctrl Pts',(0.102021826577584,-1.,-4.14231804939538));
#42953=CARTESIAN_POINT('Ctrl Pts',(0.105109286538945,-1.,-4.13516614458895));
#42954=CARTESIAN_POINT('Ctrl Pts',(0.108161120528369,-1.,-4.12800848371504));
#42955=CARTESIAN_POINT('Ctrl Pts',(0.111177012683346,-1.,-4.1208451250225));
#42956=CARTESIAN_POINT('Ctrl Pts',(0.114156649609545,-1.,-4.11367603924961));
#42957=CARTESIAN_POINT('Ctrl Pts',(0.117099722731648,-1.,-4.10650113381833));
#42958=CARTESIAN_POINT('Ctrl Pts',(0.120005924388124,-1.,-4.09932031767002));
#42959=CARTESIAN_POINT('Ctrl Pts',(0.122874946249107,-1.,-4.09213355850756));
#42960=CARTESIAN_POINT('Ctrl Pts',(0.12570647682254,-1.,-4.08494093372377));
#42961=CARTESIAN_POINT('Ctrl Pts',(0.128500200484837,-1.,-4.07774270738954));
#42962=CARTESIAN_POINT('Ctrl Pts',(0.13125579354894,-1.,-4.0705393152874));
#42963=CARTESIAN_POINT('Ctrl Pts',(0.133972916144245,-1.,-4.06333121018596));
#42964=CARTESIAN_POINT('Ctrl Pts',(0.136651205046119,-1.,-4.05611873400172));
#42965=CARTESIAN_POINT('Ctrl Pts',(0.139290267180057,-1.,-4.04890199238036));
#42966=CARTESIAN_POINT('Ctrl Pts',(0.1418896714855,-1.,-4.04168069633781));
#42967=CARTESIAN_POINT('Ctrl Pts',(0.144448947038344,-1.,-4.03445411510333));
#42968=CARTESIAN_POINT('Ctrl Pts',(0.146967602878994,-1.,-4.02722143146994));
#42969=CARTESIAN_POINT('Ctrl Pts',(0.149445144968707,-1.,-4.01998203715564));
#42970=CARTESIAN_POINT('Ctrl Pts',(0.15188109402291,-1.,-4.01273584234689));
#42971=CARTESIAN_POINT('Ctrl Pts',(0.15427500487231,-1.,-4.00548360245319));
#42972=CARTESIAN_POINT('Ctrl Pts',(0.156626481393734,-1.,-3.99822717425893));
#42973=CARTESIAN_POINT('Ctrl Pts',(0.158935123982793,-1.,-3.99096873945878));
#42974=CARTESIAN_POINT('Ctrl Pts',(0.161200482186084,-1.,-3.98371010319872));
#42975=CARTESIAN_POINT('Ctrl Pts',(0.163422004609999,-1.,-3.97645194630943));
#42976=CARTESIAN_POINT('Ctrl Pts',(0.165598992851102,-1.,-3.96919313621407));
#42977=CARTESIAN_POINT('Ctrl Pts',(0.167730547023319,-1.,-3.96192990160296));
#42978=CARTESIAN_POINT('Ctrl Pts',(0.169815666374139,-1.,-3.95465744665268));
#42979=CARTESIAN_POINT('Ctrl Pts',(0.17185335536924,-1.,-3.94737164900868));
#42980=CARTESIAN_POINT('Ctrl Pts',(0.173842734974609,-1.,-3.94007083096217));
#42981=CARTESIAN_POINT('Ctrl Pts',(0.175783136893868,-1.,-3.93275726771042));
#42982=CARTESIAN_POINT('Ctrl Pts',(0.177674246152317,-1.,-3.92543942697655));
#42983=CARTESIAN_POINT('Ctrl Pts',(0.179515885822881,-1.,-3.91812876180926));
#42984=CARTESIAN_POINT('Ctrl Pts',(0.181307740731785,-1.,-3.91083557557175));
#42985=CARTESIAN_POINT('Ctrl Pts',(0.18304908199319,-1.,-3.90356488555132));
#42986=CARTESIAN_POINT('Ctrl Pts',(0.184738537728043,-1.,-3.89631300742646));
#42987=CARTESIAN_POINT('Ctrl Pts',(0.18637372498528,-1.,-3.88906196725848));
#42988=CARTESIAN_POINT('Ctrl Pts',(0.187951632512685,-1.,-3.88178563496228));
#42989=CARTESIAN_POINT('Ctrl Pts',(0.189469253358272,-1.,-3.87445976418412));
#42990=CARTESIAN_POINT('Ctrl Pts',(0.19092419041862,-1.,-3.86707158624783));
#42991=CARTESIAN_POINT('Ctrl Pts',(0.19231515304497,-1.,-3.85962774407633));
#42992=CARTESIAN_POINT('Ctrl Pts',(0.193642806777723,-1.,-3.85216762263966));
#42993=CARTESIAN_POINT('Ctrl Pts',(0.19490900946022,-1.,-3.84475203346977));
#42994=CARTESIAN_POINT('Ctrl Pts',(0.196115198971859,-1.,-3.83743910616195));
#42995=CARTESIAN_POINT('Ctrl Pts',(0.197260935827361,-1.,-3.83026221776456));
#42996=CARTESIAN_POINT('Ctrl Pts',(0.198342616900486,-1.,-3.82321127349016));
#42997=CARTESIAN_POINT('Ctrl Pts',(0.199351525297447,-1.,-3.81620203429815));
#42998=CARTESIAN_POINT('Ctrl Pts',(0.200274679433364,-1.,-3.80909529318669));
#42999=CARTESIAN_POINT('Ctrl Pts',(0.201097756307326,-1.,-3.80175247447337));
#43000=CARTESIAN_POINT('Ctrl Pts',(0.201807533800837,-1.,-3.7940835418736));
#43001=CARTESIAN_POINT('Ctrl Pts',(0.20239426051216,-1.,-3.78609175019242));
#43002=CARTESIAN_POINT('Ctrl Pts',(0.202854729699081,-1.,-3.77793553476614));
#43003=CARTESIAN_POINT('Ctrl Pts',(0.203192390045164,-1.,-3.7699207159487));
#43004=CARTESIAN_POINT('Ctrl Pts',(0.203414634707478,-1.,-3.76242717936885));
#43005=CARTESIAN_POINT('Ctrl Pts',(0.203530796848321,-1.,-3.75585118707734));
#43006=CARTESIAN_POINT('Ctrl Pts',(0.203550035479166,-1.,-3.75054693397875));
#43007=CARTESIAN_POINT('Ctrl Pts',(0.203484186269415,-1.,-3.74703926501752));
#43008=CARTESIAN_POINT('Ctrl Pts',(0.203375226874121,-1.,-3.74535749969115));
#43009=CARTESIAN_POINT('Ctrl Pts',(0.203266610110531,-1.,-3.74471097893845));
#43010=CARTESIAN_POINT('Ctrl Pts',(0.203188003946657,-1.,-3.74453008995092));
#43011=CARTESIAN_POINT('Ctrl Pts',(0.2031560948961,-1.,-3.74449296983004));
#43012=CARTESIAN_POINT('',(0.385112848330761,-1.,-3.73017266276651));
#43013=CARTESIAN_POINT('Origin',(0.,-1.,0.));
#43014=CARTESIAN_POINT('',(0.581791163835815,-1.,-4.15950947128175));
#43015=CARTESIAN_POINT('Ctrl Pts',(0.385112848330761,-1.,-3.73017266276651));
#43016=CARTESIAN_POINT('Ctrl Pts',(0.385087139000374,-1.,-3.73021431755274));
#43017=CARTESIAN_POINT('Ctrl Pts',(0.385037797881504,-1.,-3.73040527621055));
#43018=CARTESIAN_POINT('Ctrl Pts',(0.385031656499164,-1.,-3.73106082862548));
#43019=CARTESIAN_POINT('Ctrl Pts',(0.385187124634206,-1.,-3.73273893363406));
#43020=CARTESIAN_POINT('Ctrl Pts',(0.385670806454565,-1.,-3.73621371845318));
#43021=CARTESIAN_POINT('Ctrl Pts',(0.386519576222251,-1.,-3.74144965781276));
#43022=CARTESIAN_POINT('Ctrl Pts',(0.387663020050836,-1.,-3.74792651696654));
#43023=CARTESIAN_POINT('Ctrl Pts',(0.389054775898701,-1.,-3.75529302895152));
#43024=CARTESIAN_POINT('Ctrl Pts',(0.390642072979559,-1.,-3.76315635033257));
#43025=CARTESIAN_POINT('Ctrl Pts',(0.392372786223432,-1.,-3.77114011595967));
#43026=CARTESIAN_POINT('Ctrl Pts',(0.394202481011499,-1.,-3.77894173114283));
#43027=CARTESIAN_POINT('Ctrl Pts',(0.39610320533484,-1.,-3.78640521279313));
#43028=CARTESIAN_POINT('Ctrl Pts',(0.398064818683969,-1.,-3.7935288716329));
#43029=CARTESIAN_POINT('Ctrl Pts',(0.4000883465046,-1.,-3.80040370384546));
#43030=CARTESIAN_POINT('Ctrl Pts',(0.402181320148435,-1.,-3.80716881962728));
#43031=CARTESIAN_POINT('Ctrl Pts',(0.404352694628273,-1.,-3.81396374287793));
#43032=CARTESIAN_POINT('Ctrl Pts',(0.406607038258985,-1.,-3.8208730391381));
#43033=CARTESIAN_POINT('Ctrl Pts',(0.408942371447459,-1.,-3.82790724256471));
#43034=CARTESIAN_POINT('Ctrl Pts',(0.411353038798518,-1.,-3.83503345578698));
#43035=CARTESIAN_POINT('Ctrl Pts',(0.413831367016748,-1.,-3.84219403994762));
#43036=CARTESIAN_POINT('Ctrl Pts',(0.416369678052906,-1.,-3.84932864157497));
#43037=CARTESIAN_POINT('Ctrl Pts',(0.418962468086773,-1.,-3.85639825647996));
#43038=CARTESIAN_POINT('Ctrl Pts',(0.421607423177534,-1.,-3.86339652542709));
#43039=CARTESIAN_POINT('Ctrl Pts',(0.42430417319511,-1.,-3.87033643487851));
#43040=CARTESIAN_POINT('Ctrl Pts',(0.427053541173457,-1.,-3.87724240306597));
#43041=CARTESIAN_POINT('Ctrl Pts',(0.429856640579741,-1.,-3.88414070943341));
#43042=CARTESIAN_POINT('Ctrl Pts',(0.432713929544458,-1.,-3.89104947940611));
#43043=CARTESIAN_POINT('Ctrl Pts',(0.435624629433527,-1.,-3.89797256655462));
#43044=CARTESIAN_POINT('Ctrl Pts',(0.438587235458249,-1.,-3.90490512938563));
#43045=CARTESIAN_POINT('Ctrl Pts',(0.441599824524054,-1.,-3.91183704069153));
#43046=CARTESIAN_POINT('Ctrl Pts',(0.44466043023059,-1.,-3.91875701610719));
#43047=CARTESIAN_POINT('Ctrl Pts',(0.447767416837292,-1.,-3.92565674143416));
#43048=CARTESIAN_POINT('Ctrl Pts',(0.450919768356348,-1.,-3.93253407403123));
#43049=CARTESIAN_POINT('Ctrl Pts',(0.454116879027584,-1.,-3.93939080846298));
#43050=CARTESIAN_POINT('Ctrl Pts',(0.457358410451682,-1.,-3.94623117206678));
#43051=CARTESIAN_POINT('Ctrl Pts',(0.460644124429121,-1.,-3.95306005817364));
#43052=CARTESIAN_POINT('Ctrl Pts',(0.463973722115733,-1.,-3.95988133243538));
#43053=CARTESIAN_POINT('Ctrl Pts',(0.467346690880643,-1.,-3.9666962227393));
#43054=CARTESIAN_POINT('Ctrl Pts',(0.470762379613439,-1.,-3.97350414289392));
#43055=CARTESIAN_POINT('Ctrl Pts',(0.474220061019509,-1.,-3.98030338044409));
#43056=CARTESIAN_POINT('Ctrl Pts',(0.477718999122027,-1.,-3.98709184306738));
#43057=CARTESIAN_POINT('Ctrl Pts',(0.481258512209675,-1.,-3.99386775880679));
#43058=CARTESIAN_POINT('Ctrl Pts',(0.484838042421834,-1.,-4.00063045119288));
#43059=CARTESIAN_POINT('Ctrl Pts',(0.488457130424633,-1.,-4.0073800839099));
#43060=CARTESIAN_POINT('Ctrl Pts',(0.492115383418018,-1.,-4.01411733503546));
#43061=CARTESIAN_POINT('Ctrl Pts',(0.495812444326251,-1.,-4.02084308851832));
#43062=CARTESIAN_POINT('Ctrl Pts',(0.499547962340821,-1.,-4.02755813980101));
#43063=CARTESIAN_POINT('Ctrl Pts',(0.503321556915346,-1.,-4.03426284174272));
#43064=CARTESIAN_POINT('Ctrl Pts',(0.507132823288136,-1.,-4.04095715148915));
#43065=CARTESIAN_POINT('Ctrl Pts',(0.51098134921897,-1.,-4.04764078815447));
#43066=CARTESIAN_POINT('Ctrl Pts',(0.514866728193016,-1.,-4.05431335771199));
#43067=CARTESIAN_POINT('Ctrl Pts',(0.518788572336923,-1.,-4.06097448038013));
#43068=CARTESIAN_POINT('Ctrl Pts',(0.522746528603107,-1.,-4.06762394471314));
#43069=CARTESIAN_POINT('Ctrl Pts',(0.526740277227498,-1.,-4.07426172299847));
#43070=CARTESIAN_POINT('Ctrl Pts',(0.53076951872857,-1.,-4.08088789536836));
#43071=CARTESIAN_POINT('Ctrl Pts',(0.534833963477273,-1.,-4.08750259988885));
#43072=CARTESIAN_POINT('Ctrl Pts',(0.538933321179755,-1.,-4.09410597627));
#43073=CARTESIAN_POINT('Ctrl Pts',(0.543067286877757,-1.,-4.10069810243979));
#43074=CARTESIAN_POINT('Ctrl Pts',(0.547235539485636,-1.,-4.10727897027977));
#43075=CARTESIAN_POINT('Ctrl Pts',(0.551437758497032,-1.,-4.11384852024721));
#43076=CARTESIAN_POINT('Ctrl Pts',(0.555673636129977,-1.,-4.12040666195664));
#43077=CARTESIAN_POINT('Ctrl Pts',(0.559942890594773,-1.,-4.12695329951961));
#43078=CARTESIAN_POINT('Ctrl Pts',(0.564245279537148,-1.,-4.13348835727104));
#43079=CARTESIAN_POINT('Ctrl Pts',(0.568580610189774,-1.,-4.14001179830547));
#43080=CARTESIAN_POINT('Ctrl Pts',(0.572948736069522,-1.,-4.14652361068081));
#43081=CARTESIAN_POINT('Ctrl Pts',(0.576469391676688,-1.,-4.151723761217));
#43082=CARTESIAN_POINT('Ctrl Pts',(0.579124568914235,-1.,-4.15561864788576));
#43083=CARTESIAN_POINT('Ctrl Pts',(0.580901211463535,-1.,-4.1582129171283));
#43084=CARTESIAN_POINT('Ctrl Pts',(0.581791163835815,-1.,-4.15950947128175));
#43085=CARTESIAN_POINT('',(0.73204283740062,-1.,-4.13571194405636));
#43086=CARTESIAN_POINT('',(0.581791163835815,-1.,-4.15950947128175));
#43087=CARTESIAN_POINT('',(0.786422660831985,-1.,-3.66661143271685));
#43088=CARTESIAN_POINT('Ctrl Pts',(0.73204283740062,-1.,-4.13571194405636));
#43089=CARTESIAN_POINT('Ctrl Pts',(0.732488575135159,-1.,-4.1342038373684));
#43090=CARTESIAN_POINT('Ctrl Pts',(0.733376589323546,-1.,-4.13118752795207));
#43091=CARTESIAN_POINT('Ctrl Pts',(0.734698226764092,-1.,-4.12666277570844));
#43092=CARTESIAN_POINT('Ctrl Pts',(0.736439634331344,-1.,-4.120629196238));
#43093=CARTESIAN_POINT('Ctrl Pts',(0.738581708225843,-1.,-4.11308626951927));
#43094=CARTESIAN_POINT('Ctrl Pts',(0.740688998553376,-1.,-4.10554241757547));
#43095=CARTESIAN_POINT('Ctrl Pts',(0.742761369689841,-1.,-4.09799769702611));
#43096=CARTESIAN_POINT('Ctrl Pts',(0.7447986497065,-1.,-4.09045220253573));
#43097=CARTESIAN_POINT('Ctrl Pts',(0.746800631492315,-1.,-4.08290608095642));
#43098=CARTESIAN_POINT('Ctrl Pts',(0.748767076680557,-1.,-4.07535951056152));
#43099=CARTESIAN_POINT('Ctrl Pts',(0.750697720484036,-1.,-4.06781267242378));
#43100=CARTESIAN_POINT('Ctrl Pts',(0.752592276483072,-1.,-4.06026572221515));
#43101=CARTESIAN_POINT('Ctrl Pts',(0.754450441816078,-1.,-4.05271876687915));
#43102=CARTESIAN_POINT('Ctrl Pts',(0.75627190236958,-1.,-4.04517182653997));
#43103=CARTESIAN_POINT('Ctrl Pts',(0.758056338884944,-1.,-4.03762485803119));
#43104=CARTESIAN_POINT('Ctrl Pts',(0.759803433243751,-1.,-4.03007781954412));
#43105=CARTESIAN_POINT('Ctrl Pts',(0.761512875859804,-1.,-4.02253072741268));
#43106=CARTESIAN_POINT('Ctrl Pts',(0.763184371182935,-1.,-4.01498370680496));
#43107=CARTESIAN_POINT('Ctrl Pts',(0.764817648785197,-1.,-4.00743706791509));
#43108=CARTESIAN_POINT('Ctrl Pts',(0.766412457136063,-1.,-3.99989129179622));
#43109=CARTESIAN_POINT('Ctrl Pts',(0.767968531377914,-1.,-3.9923468788101));
#43110=CARTESIAN_POINT('Ctrl Pts',(0.769485566245544,-1.,-3.98480422348451));
#43111=CARTESIAN_POINT('Ctrl Pts',(0.77096319003047,-1.,-3.97726349165488));
#43112=CARTESIAN_POINT('Ctrl Pts',(0.772400931772136,-1.,-3.96972446532772));
#43113=CARTESIAN_POINT('Ctrl Pts',(0.773798212026565,-1.,-3.96218649639807));
#43114=CARTESIAN_POINT('Ctrl Pts',(0.775154418039351,-1.,-3.9546488545231));
#43115=CARTESIAN_POINT('Ctrl Pts',(0.776468966697921,-1.,-3.94711101619447));
#43116=CARTESIAN_POINT('Ctrl Pts',(0.777741370568558,-1.,-3.93957296768103));
#43117=CARTESIAN_POINT('Ctrl Pts',(0.77897130813482,-1.,-3.93203552473174));
#43118=CARTESIAN_POINT('Ctrl Pts',(0.780158678615542,-1.,-3.92450058323823));
#43119=CARTESIAN_POINT('Ctrl Pts',(0.781303428618366,-1.,-3.91697036054676));
#43120=CARTESIAN_POINT('Ctrl Pts',(0.782405395622764,-1.,-3.90944671004542));
#43121=CARTESIAN_POINT('Ctrl Pts',(0.783464141529081,-1.,-3.9019303904397));
#43122=CARTESIAN_POINT('Ctrl Pts',(0.784478799358336,-1.,-3.89442039235103));
#43123=CARTESIAN_POINT('Ctrl Pts',(0.78544789034073,-1.,-3.88691313167398));
#43124=CARTESIAN_POINT('Ctrl Pts',(0.786369675812608,-1.,-3.8794040281819));
#43125=CARTESIAN_POINT('Ctrl Pts',(0.787242527617999,-1.,-3.87188916600912));
#43126=CARTESIAN_POINT('Ctrl Pts',(0.788065315093777,-1.,-3.86436702561345));
#43127=CARTESIAN_POINT('Ctrl Pts',(0.788837734090671,-1.,-3.85683995872529));
#43128=CARTESIAN_POINT('Ctrl Pts',(0.789560798155582,-1.,-3.84931637808894));
#43129=CARTESIAN_POINT('Ctrl Pts',(0.790236124191242,-1.,-3.84180762342454));
#43130=CARTESIAN_POINT('Ctrl Pts',(0.7908650127053,-1.,-3.83432392054786));
#43131=CARTESIAN_POINT('Ctrl Pts',(0.791447528662369,-1.,-3.82687033899792));
#43132=CARTESIAN_POINT('Ctrl Pts',(0.791981740718634,-1.,-3.81944345442249));
#43133=CARTESIAN_POINT('Ctrl Pts',(0.792462483517634,-1.,-3.81202588694756));
#43134=CARTESIAN_POINT('Ctrl Pts',(0.792882695234777,-1.,-3.80459229925637));
#43135=CARTESIAN_POINT('Ctrl Pts',(0.793235612973273,-1.,-3.79711921389897));
#43136=CARTESIAN_POINT('Ctrl Pts',(0.793516871680993,-1.,-3.78959439439235));
#43137=CARTESIAN_POINT('Ctrl Pts',(0.7937262357813,-1.,-3.78202460377598));
#43138=CARTESIAN_POINT('Ctrl Pts',(0.793870523787407,-1.,-3.77444863801212));
#43139=CARTESIAN_POINT('Ctrl Pts',(0.793961083688991,-1.,-3.76692626931111));
#43140=CARTESIAN_POINT('Ctrl Pts',(0.794008429134907,-1.,-3.75951468666257));
#43141=CARTESIAN_POINT('Ctrl Pts',(0.794017347371377,-1.,-3.75224692493864));
#43142=CARTESIAN_POINT('Ctrl Pts',(0.793982700459951,-1.,-3.74511357728861));
#43143=CARTESIAN_POINT('Ctrl Pts',(0.793882700937016,-1.,-3.73803280541687));
#43144=CARTESIAN_POINT('Ctrl Pts',(0.793682750269684,-1.,-3.73086914695805));
#43145=CARTESIAN_POINT('Ctrl Pts',(0.793347023784204,-1.,-3.72348797293734));
#43146=CARTESIAN_POINT('Ctrl Pts',(0.792848377370287,-1.,-3.71580242396124));
#43147=CARTESIAN_POINT('Ctrl Pts',(0.792177688845817,-1.,-3.70781724021806));
#43148=CARTESIAN_POINT('Ctrl Pts',(0.79135657569598,-1.,-3.69968940808721));
#43149=CARTESIAN_POINT('Ctrl Pts',(0.790436284988787,-1.,-3.69172044327364));
#43150=CARTESIAN_POINT('Ctrl Pts',(0.789483546064386,-1.,-3.68428439783905));
#43151=CARTESIAN_POINT('Ctrl Pts',(0.788569566220285,-1.,-3.67777119516252));
#43152=CARTESIAN_POINT('Ctrl Pts',(0.787758799995742,-1.,-3.67252923663655));
#43153=CARTESIAN_POINT('Ctrl Pts',(0.787145041181545,-1.,-3.66907505398677));
#43154=CARTESIAN_POINT('Ctrl Pts',(0.786774337198062,-1.,-3.66743103898702));
#43155=CARTESIAN_POINT('Ctrl Pts',(0.786565919558984,-1.,-3.66680946938292));
#43156=CARTESIAN_POINT('Ctrl Pts',(0.786459983895431,-1.,-3.6666431041522));
#43157=CARTESIAN_POINT('Ctrl Pts',(0.786422660831985,-1.,-3.66661143271685));
#43158=CARTESIAN_POINT('',(0.963899035117249,-1.,-3.62400312501245));
#43159=CARTESIAN_POINT('Origin',(0.,-1.,0.));
#43160=CARTESIAN_POINT('',(1.22531898815164,-1.,-4.01728681790024));
#43161=CARTESIAN_POINT('Ctrl Pts',(0.963899035117249,-1.,-3.62400312501245));
#43162=CARTESIAN_POINT('Ctrl Pts',(0.963880158555582,-1.,-3.6240482887845));
#43163=CARTESIAN_POINT('Ctrl Pts',(0.963861297423241,-1.,-3.62424461507588));
#43164=CARTESIAN_POINT('Ctrl Pts',(0.963957782642843,-1.,-3.62489305727662));
#43165=CARTESIAN_POINT('Ctrl Pts',(0.964373850166457,-1.,-3.62652618145335));
#43166=CARTESIAN_POINT('Ctrl Pts',(0.965395153165293,-1.,-3.62988252139846));
#43167=CARTESIAN_POINT('Ctrl Pts',(0.967052554541385,-1.,-3.63492122081143));
#43168=CARTESIAN_POINT('Ctrl Pts',(0.969195124675865,-1.,-3.64113946505766));
#43169=CARTESIAN_POINT('Ctrl Pts',(0.971722122061341,-1.,-3.64819756447455));
#43170=CARTESIAN_POINT('Ctrl Pts',(0.974519971354848,-1.,-3.65571576735126));
#43171=CARTESIAN_POINT('Ctrl Pts',(0.977478312751618,-1.,-3.66333049637475));
#43172=CARTESIAN_POINT('Ctrl Pts',(0.980505922458267,-1.,-3.67074983340361));
#43173=CARTESIAN_POINT('Ctrl Pts',(0.983550791470419,-1.,-3.67782408841715));
#43174=CARTESIAN_POINT('Ctrl Pts',(0.986602639863837,-1.,-3.68455317926068));
#43175=CARTESIAN_POINT('Ctrl Pts',(0.989676715398558,-1.,-3.69102682138847));
#43176=CARTESIAN_POINT('Ctrl Pts',(0.99280221833201,-1.,-3.69738123415662));
#43177=CARTESIAN_POINT('Ctrl Pts',(0.996009819772518,-1.,-3.70375282282138));
#43178=CARTESIAN_POINT('Ctrl Pts',(0.99931726075653,-1.,-3.71022439713938));
#43179=CARTESIAN_POINT('Ctrl Pts',(1.00272423396822,-1.,-3.71680667125119));
#43180=CARTESIAN_POINT('Ctrl Pts',(1.0062200073571,-1.,-3.72346803750596));
#43181=CARTESIAN_POINT('Ctrl Pts',(1.00978798539496,-1.,-3.73015276704426));
#43182=CARTESIAN_POINT('Ctrl Pts',(1.01341114319903,-1.,-3.73680245055734));
#43183=CARTESIAN_POINT('Ctrl Pts',(1.01707794311079,-1.,-3.74337942504959));
#43184=CARTESIAN_POINT('Ctrl Pts',(1.02078510487428,-1.,-3.74987777155834));
#43185=CARTESIAN_POINT('Ctrl Pts',(1.0245342944466,-1.,-3.75631037456194));
#43186=CARTESIAN_POINT('Ctrl Pts',(1.02833014458181,-1.,-3.76270122291232));
#43187=CARTESIAN_POINT('Ctrl Pts',(1.0321778660492,-1.,-3.76907609832522));
#43188=CARTESIAN_POINT('Ctrl Pts',(1.03608074678013,-1.,-3.77545283140445));
#43189=CARTESIAN_POINT('Ctrl Pts',(1.04003862055804,-1.,-3.78183535008192));
#43190=CARTESIAN_POINT('Ctrl Pts',(1.04404924374426,-1.,-3.78821910787195));
#43191=CARTESIAN_POINT('Ctrl Pts',(1.04810913267641,-1.,-3.79459440308793));
#43192=CARTESIAN_POINT('Ctrl Pts',(1.05221457990015,-1.,-3.80095039790678));
#43193=CARTESIAN_POINT('Ctrl Pts',(1.05636266918643,-1.,-3.80727913637784));
#43194=CARTESIAN_POINT('Ctrl Pts',(1.06055206187298,-1.,-3.81357866117485));
#43195=CARTESIAN_POINT('Ctrl Pts',(1.06478244038931,-1.,-3.81985083953012));
#43196=CARTESIAN_POINT('Ctrl Pts',(1.0690541318036,-1.,-3.82609989967278));
#43197=CARTESIAN_POINT('Ctrl Pts',(1.0733676663346,-1.,-3.83233071195145));
#43198=CARTESIAN_POINT('Ctrl Pts',(1.07772335353856,-1.,-3.83854714117486));
#43199=CARTESIAN_POINT('Ctrl Pts',(1.08212087917986,-1.,-3.84475048030615));
#43200=CARTESIAN_POINT('Ctrl Pts',(1.08655950846377,-1.,-3.85094025222691));
#43201=CARTESIAN_POINT('Ctrl Pts',(1.09103825516288,-1.,-3.85711487933911));
#43202=CARTESIAN_POINT('Ctrl Pts',(1.09555606505012,-1.,-3.86327241021242));
#43203=CARTESIAN_POINT('Ctrl Pts',(1.10011198761202,-1.,-3.86941120134872));
#43204=CARTESIAN_POINT('Ctrl Pts',(1.10470536603303,-1.,-3.87553067187566));
#43205=CARTESIAN_POINT('Ctrl Pts',(1.10933577224029,-1.,-3.88163105531791));
#43206=CARTESIAN_POINT('Ctrl Pts',(1.11400292434447,-1.,-3.88771308285229));
#43207=CARTESIAN_POINT('Ctrl Pts',(1.11870660794609,-1.,-3.89377768340362));
#43208=CARTESIAN_POINT('Ctrl Pts',(1.12344660099029,-1.,-3.89982569749978));
#43209=CARTESIAN_POINT('Ctrl Pts',(1.12822258281518,-1.,-3.90585753318622));
#43210=CARTESIAN_POINT('Ctrl Pts',(1.13303414693849,-1.,-3.91187321145495));
#43211=CARTESIAN_POINT('Ctrl Pts',(1.13788084225511,-1.,-3.91787251936688));
#43212=CARTESIAN_POINT('Ctrl Pts',(1.14276220561575,-1.,-3.92385513133937));
#43213=CARTESIAN_POINT('Ctrl Pts',(1.14767779451147,-1.,-3.92982073294334));
#43214=CARTESIAN_POINT('Ctrl Pts',(1.1526272271639,-1.,-3.9357691705651));
#43215=CARTESIAN_POINT('Ctrl Pts',(1.1576101834106,-1.,-3.94170046685542));
#43216=CARTESIAN_POINT('Ctrl Pts',(1.16262637999261,-1.,-3.9476147478092));
#43217=CARTESIAN_POINT('Ctrl Pts',(1.16767555244495,-1.,-3.95351219510062));
#43218=CARTESIAN_POINT('Ctrl Pts',(1.17275743590327,-1.,-3.95939299213164));
#43219=CARTESIAN_POINT('Ctrl Pts',(1.17787174135445,-1.,-3.96525726357682));
#43220=CARTESIAN_POINT('Ctrl Pts',(1.18301815039596,-1.,-3.9711050516465));
#43221=CARTESIAN_POINT('Ctrl Pts',(1.18819633715285,-1.,-3.97693634766926));
#43222=CARTESIAN_POINT('Ctrl Pts',(1.19340598349307,-1.,-3.98275111052015));
#43223=CARTESIAN_POINT('Ctrl Pts',(1.19864679609596,-1.,-3.98854928957287));
#43224=CARTESIAN_POINT('Ctrl Pts',(1.2039185237544,-1.,-3.99433084800649));
#43225=CARTESIAN_POINT('Ctrl Pts',(1.20922097030107,-1.,-4.00009577952534));
#43226=CARTESIAN_POINT('Ctrl Pts',(1.21455398918813,-1.,-4.00584409524937));
#43227=CARTESIAN_POINT('Ctrl Pts',(1.21884478244983,-1.,-4.01042947142681));
#43228=CARTESIAN_POINT('Ctrl Pts',(1.22207656456199,-1.,-4.01386104434674));
#43229=CARTESIAN_POINT('Ctrl Pts',(1.22423716681447,-1.,-4.0161454457032));
#43230=CARTESIAN_POINT('Ctrl Pts',(1.22531898815164,-1.,-4.01728681790024));
#43231=CARTESIAN_POINT('',(1.36999806084572,-1.,-3.97027773754922));
#43232=CARTESIAN_POINT('',(1.22531898815164,-1.,-4.01728681790024));
#43233=CARTESIAN_POINT('',(1.35032489087101,-1.,-3.4984457533445));
#43234=CARTESIAN_POINT('Ctrl Pts',(1.36999806084572,-1.,-3.97027773754922));
#43235=CARTESIAN_POINT('Ctrl Pts',(1.37020239094614,-1.,-3.9687184694131));
#43236=CARTESIAN_POINT('Ctrl Pts',(1.37060761745635,-1.,-3.96560037974645));
#43237=CARTESIAN_POINT('Ctrl Pts',(1.3712051561502,-1.,-3.96092458506535));
#43238=CARTESIAN_POINT('Ctrl Pts',(1.37198126432386,-1.,-3.95469287280914));
#43239=CARTESIAN_POINT('Ctrl Pts',(1.37291699202807,-1.,-3.94690771785133));
#43240=CARTESIAN_POINT('Ctrl Pts',(1.37381821967165,-1.,-3.93912709040818));
#43241=CARTESIAN_POINT('Ctrl Pts',(1.37468482215751,-1.,-3.93135106761844));
#43242=CARTESIAN_POINT('Ctrl Pts',(1.37551664448242,-1.,-3.92357976987672));
#43243=CARTESIAN_POINT('Ctrl Pts',(1.37631350505797,-1.,-3.91581337462644));
#43244=CARTESIAN_POINT('Ctrl Pts',(1.3770751963402,-1.,-3.90805209523486));
#43245=CARTESIAN_POINT('Ctrl Pts',(1.37780148512792,-1.,-3.90029615196727));
#43246=CARTESIAN_POINT('Ctrl Pts',(1.3784921128802,-1.,-3.89254574338496));
#43247=CARTESIAN_POINT('Ctrl Pts',(1.37914679719383,-1.,-3.88480102249278));
#43248=CARTESIAN_POINT('Ctrl Pts',(1.37976523097073,-1.,-3.87706205830532));
#43249=CARTESIAN_POINT('Ctrl Pts',(1.38034709213014,-1.,-3.86932885813068));
#43250=CARTESIAN_POINT('Ctrl Pts',(1.38089205992989,-1.,-3.86160143043959));
#43251=CARTESIAN_POINT('Ctrl Pts',(1.38139983115049,-1.,-3.85387983979481));
#43252=CARTESIAN_POINT('Ctrl Pts',(1.38187013346109,-1.,-3.84616425605764));
#43253=CARTESIAN_POINT('Ctrl Pts',(1.38230274828821,-1.,-3.83845502790746));
#43254=CARTESIAN_POINT('Ctrl Pts',(1.38269750245138,-1.,-3.8307526698229));
#43255=CARTESIAN_POINT('Ctrl Pts',(1.38305421262763,-1.,-3.82305771743829));
#43256=CARTESIAN_POINT('Ctrl Pts',(1.38337263902782,-1.,-3.81537060817811));
#43257=CARTESIAN_POINT('Ctrl Pts',(1.3836524404622,-1.,-3.80769156398411));
#43258=CARTESIAN_POINT('Ctrl Pts',(1.38389311766682,-1.,-3.80002044322111));
#43259=CARTESIAN_POINT('Ctrl Pts',(1.38409399694566,-1.,-3.79235669640841));
#43260=CARTESIAN_POINT('Ctrl Pts',(1.38425435883756,-1.,-3.78469969805082));
#43261=CARTESIAN_POINT('Ctrl Pts',(1.38437354551428,-1.,-3.77704902230418));
#43262=CARTESIAN_POINT('Ctrl Pts',(1.38445107339518,-1.,-3.76940473185779));
#43263=CARTESIAN_POINT('Ctrl Pts',(1.3844867525335,-1.,-3.76176768271367));
#43264=CARTESIAN_POINT('Ctrl Pts',(1.38448077997163,-1.,-3.7541397631875));
#43265=CARTESIAN_POINT('Ctrl Pts',(1.38443344984394,-1.,-3.74652317167876));
#43266=CARTESIAN_POINT('Ctrl Pts',(1.38434489156458,-1.,-3.73891976418104));
#43267=CARTESIAN_POINT('Ctrl Pts',(1.38421479111531,-1.,-3.73133035859282));
#43268=CARTESIAN_POINT('Ctrl Pts',(1.3840421342895,-1.,-3.72375409358803));
#43269=CARTESIAN_POINT('Ctrl Pts',(1.38382489984586,-1.,-3.7161876605181));
#43270=CARTESIAN_POINT('Ctrl Pts',(1.38356065402124,-1.,-3.70862680753347));
#43271=CARTESIAN_POINT('Ctrl Pts',(1.38324717612865,-1.,-3.701067921679));
#43272=CARTESIAN_POINT('Ctrl Pts',(1.3828831117165,-1.,-3.69350967899526));
#43273=CARTESIAN_POINT('Ctrl Pts',(1.38246852827182,-1.,-3.68595444983838));
#43274=CARTESIAN_POINT('Ctrl Pts',(1.3820057429062,-1.,-3.67841038482414));
#43275=CARTESIAN_POINT('Ctrl Pts',(1.38149812653868,-1.,-3.67088843112262));
#43276=CARTESIAN_POINT('Ctrl Pts',(1.38094856333552,-1.,-3.66339848520857));
#43277=CARTESIAN_POINT('Ctrl Pts',(1.38035791051212,-1.,-3.6559455440439));
#43278=CARTESIAN_POINT('Ctrl Pts',(1.37972372481603,-1.,-3.64852652756456));
#43279=CARTESIAN_POINT('Ctrl Pts',(1.37903818567359,-1.,-3.64112507791141));
#43280=CARTESIAN_POINT('Ctrl Pts',(1.37829035457339,-1.,-3.63371727442486));
#43281=CARTESIAN_POINT('Ctrl Pts',(1.37746987919881,-1.,-3.62628098665145));
#43282=CARTESIAN_POINT('Ctrl Pts',(1.37657053403107,-1.,-3.61880481160421));
#43283=CARTESIAN_POINT('Ctrl Pts',(1.37559314436634,-1.,-3.61129546591064));
#43284=CARTESIAN_POINT('Ctrl Pts',(1.37455051379623,-1.,-3.60379020123988));
#43285=CARTESIAN_POINT('Ctrl Pts',(1.37346320103157,-1.,-3.59634627869048));
#43286=CARTESIAN_POINT('Ctrl Pts',(1.37235053660976,-1.,-3.58901853846365));
#43287=CARTESIAN_POINT('Ctrl Pts',(1.37122241663062,-1.,-3.58183885982715));
#43288=CARTESIAN_POINT('Ctrl Pts',(1.37007229485659,-1.,-3.57479875549486));
#43289=CARTESIAN_POINT('Ctrl Pts',(1.36886584973389,-1.,-3.5678208030466));
#43290=CARTESIAN_POINT('Ctrl Pts',(1.36754771771233,-1.,-3.56077662028649));
#43291=CARTESIAN_POINT('Ctrl Pts',(1.3660614545677,-1.,-3.55353883995949));
#43292=CARTESIAN_POINT('Ctrl Pts',(1.36436666257597,-1.,-3.54602591832973));
#43293=CARTESIAN_POINT('Ctrl Pts',(1.36245507339307,-1.,-3.53824396424961));
#43294=CARTESIAN_POINT('Ctrl Pts',(1.36037259643734,-1.,-3.530344649616));
#43295=CARTESIAN_POINT('Ctrl Pts',(1.35821701528836,-1.,-3.52261776116748));
#43296=CARTESIAN_POINT('Ctrl Pts',(1.35611275237152,-1.,-3.51542230699556));
#43297=CARTESIAN_POINT('Ctrl Pts',(1.35419113575956,-1.,-3.50913227059999));
#43298=CARTESIAN_POINT('Ctrl Pts',(1.35257032843486,-1.,-3.50408168106261));
#43299=CARTESIAN_POINT('Ctrl Pts',(1.35142377279517,-1.,-3.5007660381649));
#43300=CARTESIAN_POINT('Ctrl Pts',(1.35080045218586,-1.,-3.49920025459723));
#43301=CARTESIAN_POINT('Ctrl Pts',(1.35049736560527,-1.,-3.49861894124827));
#43302=CARTESIAN_POINT('Ctrl Pts',(1.35036670892966,-1.,-3.49847119623846));
#43303=CARTESIAN_POINT('Ctrl Pts',(1.35032489087101,-1.,-3.4984457533445));
#43304=CARTESIAN_POINT('',(1.51895082866166,-1.,-3.42859860294378));
#43305=CARTESIAN_POINT('Origin',(0.,-1.,0.));
#43306=CARTESIAN_POINT('',(1.83867539237861,-1.,-3.77614523045147));
#43307=CARTESIAN_POINT('Ctrl Pts',(1.51895082866166,-1.,-3.42859860294378));
#43308=CARTESIAN_POINT('Ctrl Pts',(1.51893924967231,-1.,-3.42864616361967));
#43309=CARTESIAN_POINT('Ctrl Pts',(1.51895133295017,-1.,-3.42884302333978));
#43310=CARTESIAN_POINT('Ctrl Pts',(1.51914806898539,-1.,-3.42946838852728));
#43311=CARTESIAN_POINT('Ctrl Pts',(1.5198144909343,-1.,-3.43101631893491));
#43312=CARTESIAN_POINT('Ctrl Pts',(1.52134826724227,-1.,-3.43417156977749));
#43313=CARTESIAN_POINT('Ctrl Pts',(1.52377348950429,-1.,-3.43888895974182));
#43314=CARTESIAN_POINT('Ctrl Pts',(1.52686242875717,-1.,-3.44469547527));
#43315=CARTESIAN_POINT('Ctrl Pts',(1.530462444618,-1.,-3.45127136828667));
#43316=CARTESIAN_POINT('Ctrl Pts',(1.53440195378902,-1.,-3.45825932955273));
#43317=CARTESIAN_POINT('Ctrl Pts',(1.53851507915533,-1.,-3.46531752207222));
#43318=CARTESIAN_POINT('Ctrl Pts',(1.54266605398152,-1.,-3.47217189224576));
#43319=CARTESIAN_POINT('Ctrl Pts',(1.54678009290206,-1.,-3.47868272898599));
#43320=CARTESIAN_POINT('Ctrl Pts',(1.55084702970382,-1.,-3.48485155928414));
#43321=CARTESIAN_POINT('Ctrl Pts',(1.5548959590107,-1.,-3.49076460877317));
#43322=CARTESIAN_POINT('Ctrl Pts',(1.55897703097859,-1.,-3.49655185179623));
#43323=CARTESIAN_POINT('Ctrl Pts',(1.56314187758689,-1.,-3.50234321621607));
#43324=CARTESIAN_POINT('Ctrl Pts',(1.56742097575041,-1.,-3.50821771695427));
#43325=CARTESIAN_POINT('Ctrl Pts',(1.57181569799774,-1.,-3.51418598431733));
#43326=CARTESIAN_POINT('Ctrl Pts',(1.5763104998818,-1.,-3.52021847865961));
#43327=CARTESIAN_POINT('Ctrl Pts',(1.58088027227856,-1.,-3.52626275334899));
#43328=CARTESIAN_POINT('Ctrl Pts',(1.58549906268083,-1.,-3.53226378147068));
#43329=CARTESIAN_POINT('Ctrl Pts',(1.59014958368725,-1.,-3.53818616861045));
#43330=CARTESIAN_POINT('Ctrl Pts',(1.5948276694975,-1.,-3.544024581823));
#43331=CARTESIAN_POINT('Ctrl Pts',(1.59953698113444,-1.,-3.54979148634426));
#43332=CARTESIAN_POINT('Ctrl Pts',(1.60428584699848,-1.,-3.55550985096117));
#43333=CARTESIAN_POINT('Ctrl Pts',(1.60908344685459,-1.,-3.56120432482986));
#43334=CARTESIAN_POINT('Ctrl Pts',(1.61393581747522,-1.,-3.56689200468404));
#43335=CARTESIAN_POINT('Ctrl Pts',(1.61884340915412,-1.,-3.57257679609826));
#43336=CARTESIAN_POINT('Ctrl Pts',(1.62380329464851,-1.,-3.57825455954405));
#43337=CARTESIAN_POINT('Ctrl Pts',(1.62881051550748,-1.,-3.5839162577435));
#43338=CARTESIAN_POINT('Ctrl Pts',(1.63385971451259,-1.,-3.58955176627876));
#43339=CARTESIAN_POINT('Ctrl Pts',(1.63894676675349,-1.,-3.59515368334887));
#43340=CARTESIAN_POINT('Ctrl Pts',(1.6440700438558,-1.,-3.6007202851384));
#43341=CARTESIAN_POINT('Ctrl Pts',(1.64922952425833,-1.,-3.60625346556992));
#43342=CARTESIAN_POINT('Ctrl Pts',(1.65442619244327,-1.,-3.61175734965129));
#43343=CARTESIAN_POINT('Ctrl Pts',(1.65966133399186,-1.,-3.61723666482457));
#43344=CARTESIAN_POINT('Ctrl Pts',(1.66493585923853,-1.,-3.62269517989104));
#43345=CARTESIAN_POINT('Ctrl Pts',(1.67024966008037,-1.,-3.62813422105257));
#43346=CARTESIAN_POINT('Ctrl Pts',(1.67560193613145,-1.,-3.63355343201211));
#43347=CARTESIAN_POINT('Ctrl Pts',(1.68099146651577,-1.,-3.63895140887443));
#43348=CARTESIAN_POINT('Ctrl Pts',(1.68641690471455,-1.,-3.64432638915199));
#43349=CARTESIAN_POINT('Ctrl Pts',(1.691877054817,-1.,-3.64967689827393));
#43350=CARTESIAN_POINT('Ctrl Pts',(1.69737117722558,-1.,-3.65500246526798));
#43351=CARTESIAN_POINT('Ctrl Pts',(1.70289888566904,-1.,-3.6603033877491));
#43352=CARTESIAN_POINT('Ctrl Pts',(1.70846001610983,-1.,-3.6655804319893));
#43353=CARTESIAN_POINT('Ctrl Pts',(1.71405450210392,-1.,-3.67083454901629));
#43354=CARTESIAN_POINT('Ctrl Pts',(1.71968225581787,-1.,-3.67606660374665));
#43355=CARTESIAN_POINT('Ctrl Pts',(1.72534302437003,-1.,-3.68127704936472));
#43356=CARTESIAN_POINT('Ctrl Pts',(1.73103640956647,-1.,-3.68646597019188));
#43357=CARTESIAN_POINT('Ctrl Pts',(1.73676193254493,-1.,-3.69163322647906));
#43358=CARTESIAN_POINT('Ctrl Pts',(1.74251908492589,-1.,-3.6967785691046));
#43359=CARTESIAN_POINT('Ctrl Pts',(1.74830738046092,-1.,-3.70190175673422));
#43360=CARTESIAN_POINT('Ctrl Pts',(1.75412641804148,-1.,-3.70700269736876));
#43361=CARTESIAN_POINT('Ctrl Pts',(1.75997588499021,-1.,-3.71208146346455));
#43362=CARTESIAN_POINT('Ctrl Pts',(1.76585552124549,-1.,-3.71713822377676));
#43363=CARTESIAN_POINT('Ctrl Pts',(1.77176509401846,-1.,-3.72217319911429));
#43364=CARTESIAN_POINT('Ctrl Pts',(1.77770437039606,-1.,-3.72718661205504));
#43365=CARTESIAN_POINT('Ctrl Pts',(1.78367308442682,-1.,-3.73217863095022));
#43366=CARTESIAN_POINT('Ctrl Pts',(1.78967092823139,-1.,-3.73714934729962));
#43367=CARTESIAN_POINT('Ctrl Pts',(1.79569757859041,-1.,-3.74209880351667));
#43368=CARTESIAN_POINT('Ctrl Pts',(1.80175271485519,-1.,-3.74702700874954));
#43369=CARTESIAN_POINT('Ctrl Pts',(1.80783603939662,-1.,-3.75193395888069));
#43370=CARTESIAN_POINT('Ctrl Pts',(1.81394729834032,-1.,-3.75681965683995));
#43371=CARTESIAN_POINT('Ctrl Pts',(1.82008629694924,-1.,-3.76168412709652));
#43372=CARTESIAN_POINT('Ctrl Pts',(1.82625289221933,-1.,-3.76652740355856));
#43373=CARTESIAN_POINT('Ctrl Pts',(1.83120816956515,-1.,-3.77038509819777));
#43374=CARTESIAN_POINT('Ctrl Pts',(1.83493697935064,-1.,-3.77326886065484));
#43375=CARTESIAN_POINT('Ctrl Pts',(1.83742834010821,-1.,-3.77518714458232));
#43376=CARTESIAN_POINT('Ctrl Pts',(1.83867539237861,-1.,-3.77614523045147));
#43377=CARTESIAN_POINT('',(1.97421938526992,-1.,-3.70708211654725));
#43378=CARTESIAN_POINT('',(1.83867539237861,-1.,-3.77614523045147));
#43379=CARTESIAN_POINT('',(1.88097764062541,-1.,-3.24413672884902));
#43380=CARTESIAN_POINT('Ctrl Pts',(1.97421938526992,-1.,-3.70708211654725));
#43381=CARTESIAN_POINT('Ctrl Pts',(1.974177276451,-1.,-3.7055100813194));
#43382=CARTESIAN_POINT('Ctrl Pts',(1.97408973726149,-1.,-3.70236698911837));
#43383=CARTESIAN_POINT('Ctrl Pts',(1.97394846382288,-1.,-3.69765528558292));
#43384=CARTESIAN_POINT('Ctrl Pts',(1.97374016224397,-1.,-3.69137888597855));
#43385=CARTESIAN_POINT('Ctrl Pts',(1.9734465030363,-1.,-3.68354319913416));
#43386=CARTESIAN_POINT('Ctrl Pts',(1.97311947678035,-1.,-3.67571738106175));
#43387=CARTESIAN_POINT('Ctrl Pts',(1.9727589719863,-1.,-3.66790152751984));
#43388=CARTESIAN_POINT('Ctrl Pts',(1.97236485439317,-1.,-3.66009578166865));
#43389=CARTESIAN_POINT('Ctrl Pts',(1.97193697240645,-1.,-3.65230034717364));
#43390=CARTESIAN_POINT('Ctrl Pts',(1.97147515441539,-1.,-3.64451546724222));
#43391=CARTESIAN_POINT('Ctrl Pts',(1.97097920454698,-1.,-3.63674139590853));
#43392=CARTESIAN_POINT('Ctrl Pts',(1.97044889850518,-1.,-3.62897836973397));
#43393=CARTESIAN_POINT('Ctrl Pts',(1.96988398129888,-1.,-3.62122658401722));
#43394=CARTESIAN_POINT('Ctrl Pts',(1.96928416040712,-1.,-3.61348615496393));
#43395=CARTESIAN_POINT('Ctrl Pts',(1.96864911885775,-1.,-3.60575714017676));
#43396=CARTESIAN_POINT('Ctrl Pts',(1.96797854118257,-1.,-3.59803959819725));
#43397=CARTESIAN_POINT('Ctrl Pts',(1.96727213799507,-1.,-3.5903336402273));
#43398=CARTESIAN_POINT('Ctrl Pts',(1.9665296668894,-1.,-3.58263947663884));
#43399=CARTESIAN_POINT('Ctrl Pts',(1.96575096652857,-1.,-3.57495748601088));
#43400=CARTESIAN_POINT('Ctrl Pts',(1.96493594634643,-1.,-3.56728820357933));
#43401=CARTESIAN_POINT('Ctrl Pts',(1.96408450906868,-1.,-3.55963218706201));
#43402=CARTESIAN_POINT('Ctrl Pts',(1.96319648628667,-1.,-3.55198990600929));
#43403=CARTESIAN_POINT('Ctrl Pts',(1.96227157573058,-1.,-3.54436163300425));
#43404=CARTESIAN_POINT('Ctrl Pts',(1.96130926212661,-1.,-3.53674730625759));
#43405=CARTESIAN_POINT('Ctrl Pts',(1.96030879411534,-1.,-3.52914648844289));
#43406=CARTESIAN_POINT('Ctrl Pts',(1.95926936324436,-1.,-3.52155867431438));
#43407=CARTESIAN_POINT('Ctrl Pts',(1.95819025316768,-1.,-3.51398354617773));
#43408=CARTESIAN_POINT('Ctrl Pts',(1.95707099606513,-1.,-3.50642124159913));
#43409=CARTESIAN_POINT('Ctrl Pts',(1.9559115382367,-1.,-3.49887263575602));
#43410=CARTESIAN_POINT('Ctrl Pts',(1.95471236969653,-1.,-3.49133956289154));
#43411=CARTESIAN_POINT('Ctrl Pts',(1.95347412486316,-1.,-3.48382414832649));
#43412=CARTESIAN_POINT('Ctrl Pts',(1.95219722189878,-1.,-3.47632820495926));
#43413=CARTESIAN_POINT('Ctrl Pts',(1.95088147859876,-1.,-3.4688525897419));
#43414=CARTESIAN_POINT('Ctrl Pts',(1.94952575850196,-1.,-3.46139661060959));
#43415=CARTESIAN_POINT('Ctrl Pts',(1.94812754766524,-1.,-3.45395731584051));
#43416=CARTESIAN_POINT('Ctrl Pts',(1.94668377715332,-1.,-3.44653088665685));
#43417=CARTESIAN_POINT('Ctrl Pts',(1.94519168842883,-1.,-3.43911410197693));
#43418=CARTESIAN_POINT('Ctrl Pts',(1.94364973660285,-1.,-3.43170586602436));
#43419=CARTESIAN_POINT('Ctrl Pts',(1.94205835913692,-1.,-3.42430850941497));
#43420=CARTESIAN_POINT('Ctrl Pts',(1.94042111965237,-1.,-3.41692971994082));
#43421=CARTESIAN_POINT('Ctrl Pts',(1.93874306008132,-1.,-3.40957978266623));
#43422=CARTESIAN_POINT('Ctrl Pts',(1.93702857723089,-1.,-3.40226802104093));
#43423=CARTESIAN_POINT('Ctrl Pts',(1.93527929945982,-1.,-3.39499923640789));
#43424=CARTESIAN_POINT('Ctrl Pts',(1.93349233176794,-1.,-3.38777076883267));
#43425=CARTESIAN_POINT('Ctrl Pts',(1.93165739093292,-1.,-3.38056768525577));
#43426=CARTESIAN_POINT('Ctrl Pts',(1.92975993109897,-1.,-3.37336807068078));
#43427=CARTESIAN_POINT('Ctrl Pts',(1.92778626543803,-1.,-3.36615168657597));
#43428=CARTESIAN_POINT('Ctrl Pts',(1.92572846125763,-1.,-3.35890824422976));
#43429=CARTESIAN_POINT('Ctrl Pts',(1.92358838440518,-1.,-3.35164424847207));
#43430=CARTESIAN_POINT('Ctrl Pts',(1.92138450828378,-1.,-3.34439448941915));
#43431=CARTESIAN_POINT('Ctrl Pts',(1.91914609610173,-1.,-3.33721230709948));
#43432=CARTESIAN_POINT('Ctrl Pts',(1.91690081930297,-1.,-3.33014884257812));
#43433=CARTESIAN_POINT('Ctrl Pts',(1.91466343916612,-1.,-3.32323403454507));
#43434=CARTESIAN_POINT('Ctrl Pts',(1.91242616234459,-1.,-3.31646052426395));
#43435=CARTESIAN_POINT('Ctrl Pts',(1.91014297830502,-1.,-3.30975721158694));
#43436=CARTESIAN_POINT('Ctrl Pts',(1.90773912171424,-1.,-3.30300595568341));
#43437=CARTESIAN_POINT('Ctrl Pts',(1.9051389186417,-1.,-3.29608978722258));
#43438=CARTESIAN_POINT('Ctrl Pts',(1.9022897124757,-1.,-3.28893448600364));
#43439=CARTESIAN_POINT('Ctrl Pts',(1.89918429230424,-1.,-3.28154737912287));
#43440=CARTESIAN_POINT('Ctrl Pts',(1.89589172903662,-1.,-3.27407108932908));
#43441=CARTESIAN_POINT('Ctrl Pts',(1.89255393500769,-1.,-3.2667765388833));
#43442=CARTESIAN_POINT('Ctrl Pts',(1.88934996203508,-1.,-3.2599988519361));
#43443=CARTESIAN_POINT('Ctrl Pts',(1.88646802523372,-1.,-3.25408686339298));
#43444=CARTESIAN_POINT('Ctrl Pts',(1.88407708646435,-1.,-3.24935200512055));
#43445=CARTESIAN_POINT('Ctrl Pts',(1.88242596600422,-1.,-3.24625654410705));
#43446=CARTESIAN_POINT('Ctrl Pts',(1.88156537699118,-1.,-3.24480754675942));
#43447=CARTESIAN_POINT('Ctrl Pts',(1.88117508446657,-1.,-3.24428080352952));
#43448=CARTESIAN_POINT('Ctrl Pts',(1.88102292397987,-1.,-3.24415531671311));
#43449=CARTESIAN_POINT('Ctrl Pts',(1.88097764062541,-1.,-3.24413672884902));
#43450=CARTESIAN_POINT('',(2.03660101169564,-1.,-3.14877060440425));
#43451=CARTESIAN_POINT('Origin',(0.,-1.,0.));
#43452=CARTESIAN_POINT('',(2.40675750623143,-1.,-3.44202241512147));
#43453=CARTESIAN_POINT('Ctrl Pts',(2.03660101169564,-1.,-3.14877060440425));
#43454=CARTESIAN_POINT('Ctrl Pts',(2.03659701539175,-1.,-3.1488193908823));
#43455=CARTESIAN_POINT('Ctrl Pts',(2.03663974554941,-1.,-3.14901193669147));
#43456=CARTESIAN_POINT('Ctrl Pts',(2.03693188810614,-1.,-3.14959882629936));
#43457=CARTESIAN_POINT('Ctrl Pts',(2.03783225496023,-1.,-3.15102344775396));
#43458=CARTESIAN_POINT('Ctrl Pts',(2.03984073791432,-1.,-3.1538999167466));
#43459=CARTESIAN_POINT('Ctrl Pts',(2.04297406404132,-1.,-3.15817983946525));
#43460=CARTESIAN_POINT('Ctrl Pts',(2.0469333124766,-1.,-3.16343165059235));
#43461=CARTESIAN_POINT('Ctrl Pts',(2.05151770247452,-1.,-3.16936341689859));
#43462=CARTESIAN_POINT('Ctrl Pts',(2.05650186773279,-1.,-3.17564906975592));
#43463=CARTESIAN_POINT('Ctrl Pts',(2.06166849827143,-1.,-3.18197692964677));
#43464=CARTESIAN_POINT('Ctrl Pts',(2.06684062744065,-1.,-3.18809755562297));
#43465=CARTESIAN_POINT('Ctrl Pts',(2.07192253497765,-1.,-3.19388465568113));
#43466=CARTESIAN_POINT('Ctrl Pts',(2.0769044187063,-1.,-3.19934132835879));
#43467=CARTESIAN_POINT('Ctrl Pts',(2.08182850370816,-1.,-3.20454818630635));
#43468=CARTESIAN_POINT('Ctrl Pts',(2.08676465517435,-1.,-3.20962575845433));
#43469=CARTESIAN_POINT('Ctrl Pts',(2.0917841946046,-1.,-3.2146942960168));
#43470=CARTESIAN_POINT('Ctrl Pts',(2.09692958434933,-1.,-3.21982707347067));
#43471=CARTESIAN_POINT('Ctrl Pts',(2.10220384298533,-1.,-3.22503437553496));
#43472=CARTESIAN_POINT('Ctrl Pts',(2.1075869964248,-1.,-3.23028945793334));
#43473=CARTESIAN_POINT('Ctrl Pts',(2.11304604021784,-1.,-3.23554444767115));
#43474=CARTESIAN_POINT('Ctrl Pts',(2.11854673326972,-1.,-3.24074905517282));
#43475=CARTESIAN_POINT('Ctrl Pts',(2.12406646410943,-1.,-3.24587102613347));
#43476=CARTESIAN_POINT('Ctrl Pts',(2.1296002839681,-1.,-3.25090574493994));
#43477=CARTESIAN_POINT('Ctrl Pts',(2.13515375878786,-1.,-3.25586495065027));
#43478=CARTESIAN_POINT('Ctrl Pts',(2.14073870754257,-1.,-3.26077002641868));
#43479=CARTESIAN_POINT('Ctrl Pts',(2.14636805295663,-1.,-3.26564388189764));
#43480=CARTESIAN_POINT('Ctrl Pts',(2.15205043199818,-1.,-3.27050245897244));
#43481=CARTESIAN_POINT('Ctrl Pts',(2.15778690038359,-1.,-3.27534954469206));
#43482=CARTESIAN_POINT('Ctrl Pts',(2.16357391934434,-1.,-3.28018150841414));
#43483=CARTESIAN_POINT('Ctrl Pts',(2.16940517773459,-1.,-3.2849901997973));
#43484=CARTESIAN_POINT('Ctrl Pts',(2.17527380048422,-1.,-3.28976645712566));
#43485=CARTESIAN_POINT('Ctrl Pts',(2.18117455557062,-1.,-3.29450361500484));
#43486=CARTESIAN_POINT('Ctrl Pts',(2.18710556500325,-1.,-3.29920022557635));
#43487=CARTESIAN_POINT('Ctrl Pts',(2.19306710376112,-1.,-3.30385816281831));
#43488=CARTESIAN_POINT('Ctrl Pts',(2.19906078949924,-1.,-3.30848134694597));
#43489=CARTESIAN_POINT('Ctrl Pts',(2.20508863150608,-1.,-3.3130742460895));
#43490=CARTESIAN_POINT('Ctrl Pts',(2.21115211847872,-1.,-3.31764044024231));
#43491=CARTESIAN_POINT('Ctrl Pts',(2.21725135110889,-1.,-3.32218125618955));
#43492=CARTESIAN_POINT('Ctrl Pts',(2.22338548312758,-1.,-3.32669646722871));
#43493=CARTESIAN_POINT('Ctrl Pts',(2.22955308907221,-1.,-3.33118487773593));
#43494=CARTESIAN_POINT('Ctrl Pts',(2.23575256328809,-1.,-3.33564495756478));
#43495=CARTESIAN_POINT('Ctrl Pts',(2.24198249391437,-1.,-3.34007543738044));
#43496=CARTESIAN_POINT('Ctrl Pts',(2.24824207678287,-1.,-3.34447596770768));
#43497=CARTESIAN_POINT('Ctrl Pts',(2.25453097693524,-1.,-3.34884690292342));
#43498=CARTESIAN_POINT('Ctrl Pts',(2.26084915222484,-1.,-3.35318902552676));
#43499=CARTESIAN_POINT('Ctrl Pts',(2.26719668579921,-1.,-3.35750328523077));
#43500=CARTESIAN_POINT('Ctrl Pts',(2.27357362620902,-1.,-3.36179055004369));
#43501=CARTESIAN_POINT('Ctrl Pts',(2.27997979457968,-1.,-3.36605130712978));
#43502=CARTESIAN_POINT('Ctrl Pts',(2.28641481081045,-1.,-3.37028570206357));
#43503=CARTESIAN_POINT('Ctrl Pts',(2.2928781800731,-1.,-3.37449367172707));
#43504=CARTESIAN_POINT('Ctrl Pts',(2.29936936127588,-1.,-3.37867504959382));
#43505=CARTESIAN_POINT('Ctrl Pts',(2.30588783640389,-1.,-3.38282967336676));
#43506=CARTESIAN_POINT('Ctrl Pts',(2.31243319489505,-1.,-3.38695751492659));
#43507=CARTESIAN_POINT('Ctrl Pts',(2.31900513925627,-1.,-3.39105869475112));
#43508=CARTESIAN_POINT('Ctrl Pts',(2.32560343902683,-1.,-3.39513342020045));
#43509=CARTESIAN_POINT('Ctrl Pts',(2.33222789882601,-1.,-3.39918194578115));
#43510=CARTESIAN_POINT('Ctrl Pts',(2.33887832342715,-1.,-3.40320452776646));
#43511=CARTESIAN_POINT('Ctrl Pts',(2.34555447648901,-1.,-3.40720137403888));
#43512=CARTESIAN_POINT('Ctrl Pts',(2.35225606823649,-1.,-3.41117262313464));
#43513=CARTESIAN_POINT('Ctrl Pts',(2.35898278606449,-1.,-3.4151183675076));
#43514=CARTESIAN_POINT('Ctrl Pts',(2.36573431470313,-1.,-3.41903866635384));
#43515=CARTESIAN_POINT('Ctrl Pts',(2.37251035954351,-1.,-3.42293356216595));
#43516=CARTESIAN_POINT('Ctrl Pts',(2.37931067029517,-1.,-3.42680309755241));
#43517=CARTESIAN_POINT('Ctrl Pts',(2.38613505844641,-1.,-3.43064732714472));
#43518=CARTESIAN_POINT('Ctrl Pts',(2.39298338805823,-1.,-3.43446630680436));
#43519=CARTESIAN_POINT('Ctrl Pts',(2.39848113411428,-1.,-3.43750133066037));
#43520=CARTESIAN_POINT('Ctrl Pts',(2.40261515590099,-1.,-3.43976627485223));
#43521=CARTESIAN_POINT('Ctrl Pts',(2.40537592959345,-1.,-3.44127120683402));
#43522=CARTESIAN_POINT('Ctrl Pts',(2.40675750623143,-1.,-3.44202241512147));
#43523=CARTESIAN_POINT('',(2.52982887637028,-1.,-3.35260583073571));
#43524=CARTESIAN_POINT('',(2.40675750623143,-1.,-3.44202241512147));
#43525=CARTESIAN_POINT('',(2.36531447826073,-1.,-2.90994629141676));
#43526=CARTESIAN_POINT('Ctrl Pts',(2.52982887637028,-1.,-3.35260583073571));
#43527=CARTESIAN_POINT('Ctrl Pts',(2.5295413654909,-1.,-3.35105973714072));
#43528=CARTESIAN_POINT('Ctrl Pts',(2.52896321610703,-1.,-3.34796903576663));
#43529=CARTESIAN_POINT('Ctrl Pts',(2.52808660915689,-1.,-3.34333744115511));
#43530=CARTESIAN_POINT('Ctrl Pts',(2.52689902690158,-1.,-3.33717089999103));
#43531=CARTESIAN_POINT('Ctrl Pts',(2.52538321164634,-1.,-3.32947762187533));
#43532=CARTESIAN_POINT('Ctrl Pts',(2.5238359839626,-1.,-3.32179931078699));
#43533=CARTESIAN_POINT('Ctrl Pts',(2.52225724871313,-1.,-3.31413607874645));
#43534=CARTESIAN_POINT('Ctrl Pts',(2.52064689568511,-1.,-3.30648808815443));
#43535=CARTESIAN_POINT('Ctrl Pts',(2.51900480701068,-1.,-3.29885556388353));
#43536=CARTESIAN_POINT('Ctrl Pts',(2.51733085123797,-1.,-3.2912387729927));
#43537=CARTESIAN_POINT('Ctrl Pts',(2.51562487464514,-1.,-3.28363799702982));
#43538=CARTESIAN_POINT('Ctrl Pts',(2.513886692704,-1.,-3.27605350473142));
#43539=CARTESIAN_POINT('Ctrl Pts',(2.51211608411423,-1.,-3.26848552888116));
#43540=CARTESIAN_POINT('Ctrl Pts',(2.51031277813486,-1.,-3.26093423001434));
#43541=CARTESIAN_POINT('Ctrl Pts',(2.50847647070723,-1.,-3.25339971460982));
#43542=CARTESIAN_POINT('Ctrl Pts',(2.506606859405,-1.,-3.24588208983849));
#43543=CARTESIAN_POINT('Ctrl Pts',(2.5047036758003,-1.,-3.23838151080319));
#43544=CARTESIAN_POINT('Ctrl Pts',(2.50276671338111,-1.,-3.23089822320646));
#43545=CARTESIAN_POINT('Ctrl Pts',(2.50079587201957,-1.,-3.22343262620503));
#43546=CARTESIAN_POINT('Ctrl Pts',(2.4987911459939,-1.,-3.21598526261286));
#43547=CARTESIAN_POINT('Ctrl Pts',(2.4967525264737,-1.,-3.20855669849836));
#43548=CARTESIAN_POINT('Ctrl Pts',(2.49467992057755,-1.,-3.20114742397588));
#43549=CARTESIAN_POINT('Ctrl Pts',(2.49257307239848,-1.,-3.19375775555798));
#43550=CARTESIAN_POINT('Ctrl Pts',(2.49043146334059,-1.,-3.18638771282266));
#43551=CARTESIAN_POINT('Ctrl Pts',(2.48825428288201,-1.,-3.17903698136622));
#43552=CARTESIAN_POINT('Ctrl Pts',(2.48604065348587,-1.,-3.17170518863313));
#43553=CARTESIAN_POINT('Ctrl Pts',(2.48378981792725,-1.,-3.16439213290161));
#43554=CARTESIAN_POINT('Ctrl Pts',(2.48150133566571,-1.,-3.15709802322739));
#43555=CARTESIAN_POINT('Ctrl Pts',(2.47917529057029,-1.,-3.14982373241352));
#43556=CARTESIAN_POINT('Ctrl Pts',(2.47681245356109,-1.,-3.1425709954655));
#43557=CARTESIAN_POINT('Ctrl Pts',(2.47441378371932,-1.,-3.13534181229295));
#43558=CARTESIAN_POINT('Ctrl Pts',(2.47197997765871,-1.,-3.12813790805952));
#43559=CARTESIAN_POINT('Ctrl Pts',(2.46951098947469,-1.,-3.12096015766983));
#43560=CARTESIAN_POINT('Ctrl Pts',(2.46700558843506,-1.,-3.11380805536122));
#43561=CARTESIAN_POINT('Ctrl Pts',(2.46446082979646,-1.,-3.1066790790198));
#43562=CARTESIAN_POINT('Ctrl Pts',(2.46187308501884,-1.,-3.09956993697052));
#43563=CARTESIAN_POINT('Ctrl Pts',(2.4592391256388,-1.,-3.09247787931887));
#43564=CARTESIAN_POINT('Ctrl Pts',(2.45655725437039,-1.,-3.08540206545315));
#43565=CARTESIAN_POINT('Ctrl Pts',(2.4538282678779,-1.,-3.07834472886139));
#43566=CARTESIAN_POINT('Ctrl Pts',(2.45105688854422,-1.,-3.07131290521297));
#43567=CARTESIAN_POINT('Ctrl Pts',(2.44824970516543,-1.,-3.06431596421405));
#43568=CARTESIAN_POINT('Ctrl Pts',(2.44541251892556,-1.,-3.05736242671506));
#43569=CARTESIAN_POINT('Ctrl Pts',(2.44254768923105,-1.,-3.05045678021504));
#43570=CARTESIAN_POINT('Ctrl Pts',(2.43965194061857,-1.,-3.04359685040555));
#43571=CARTESIAN_POINT('Ctrl Pts',(2.43671278042414,-1.,-3.03676949672822));
#43572=CARTESIAN_POINT('Ctrl Pts',(2.43371241361488,-1.,-3.02995534946978));
#43573=CARTESIAN_POINT('Ctrl Pts',(2.43063415586637,-1.,-3.02313656036004));
#43574=CARTESIAN_POINT('Ctrl Pts',(2.42746856264168,-1.,-3.01630420830504));
#43575=CARTESIAN_POINT('Ctrl Pts',(2.42421849439613,-1.,-3.00946442616659));
#43576=CARTESIAN_POINT('Ctrl Pts',(2.42090763946779,-1.,-3.00264868585996));
#43577=CARTESIAN_POINT('Ctrl Pts',(2.41757324500514,-1.,-2.99590509293503));
#43578=CARTESIAN_POINT('Ctrl Pts',(2.41425064199586,-1.,-2.98927983005796));
#43579=CARTESIAN_POINT('Ctrl Pts',(2.41095909342571,-1.,-2.98280015815107));
#43580=CARTESIAN_POINT('Ctrl Pts',(2.40768975073713,-1.,-2.97646002822422));
#43581=CARTESIAN_POINT('Ctrl Pts',(2.40438604734919,-1.,-2.9701964131236));
#43582=CARTESIAN_POINT('Ctrl Pts',(2.4009556571164,-1.,-2.96390432240312));
#43583=CARTESIAN_POINT('Ctrl Pts',(2.39730553974516,-1.,-2.95748006482942));
#43584=CARTESIAN_POINT('Ctrl Pts',(2.39337207631667,-1.,-2.95085857128439));
#43585=CARTESIAN_POINT('Ctrl Pts',(2.38914929090759,-1.,-2.94404820669076));
#43586=CARTESIAN_POINT('Ctrl Pts',(2.38472771516311,-1.,-2.93717903280391));
#43587=CARTESIAN_POINT('Ctrl Pts',(2.38028989582073,-1.,-2.93049643640206));
#43588=CARTESIAN_POINT('Ctrl Pts',(2.3760651052403,-1.,-2.92430340582608));
#43589=CARTESIAN_POINT('Ctrl Pts',(2.37229381109821,-1.,-2.91891503791411));
#43590=CARTESIAN_POINT('Ctrl Pts',(2.36919161373173,-1.,-2.9146124988314));
#43591=CARTESIAN_POINT('Ctrl Pts',(2.36707658451664,-1.,-2.91181344022549));
#43592=CARTESIAN_POINT('Ctrl Pts',(2.36599991765749,-1.,-2.91051690822156));
#43593=CARTESIAN_POINT('Ctrl Pts',(2.36553202948613,-1.,-2.91005770527719));
#43594=CARTESIAN_POINT('Ctrl Pts',(2.36536211188453,-1.,-2.90995756655606));
#43595=CARTESIAN_POINT('Ctrl Pts',(2.36531447826073,-1.,-2.90994629141676));
#43596=CARTESIAN_POINT('',(2.50410331873042,-1.,-2.79140942341378));
#43597=CARTESIAN_POINT('Origin',(0.,-1.,0.));
#43598=CARTESIAN_POINT('',(2.91557726271063,-1.,-3.02314558451372));
#43599=CARTESIAN_POINT('Ctrl Pts',(2.50410331873042,-1.,-2.79140942341378));
#43600=CARTESIAN_POINT('Ctrl Pts',(2.50410700351426,-1.,-2.79145823440899));
#43601=CARTESIAN_POINT('Ctrl Pts',(2.50417932839343,-1.,-2.79164172519039));
#43602=CARTESIAN_POINT('Ctrl Pts',(2.50455968395235,-1.,-2.79217568804874));
#43603=CARTESIAN_POINT('Ctrl Pts',(2.50567182569153,-1.,-2.79344192164204));
#43604=CARTESIAN_POINT('Ctrl Pts',(2.50810555977564,-1.,-2.7959687805717));
#43605=CARTESIAN_POINT('Ctrl Pts',(2.51186983687947,-1.,-2.79970585014308));
#43606=CARTESIAN_POINT('Ctrl Pts',(2.51660190466067,-1.,-2.80427363984939));
#43607=CARTESIAN_POINT('Ctrl Pts',(2.52205778589922,-1.,-2.80941521967234));
#43608=CARTESIAN_POINT('Ctrl Pts',(2.52796388055457,-1.,-2.8148437904867));
#43609=CARTESIAN_POINT('Ctrl Pts',(2.53405679667463,-1.,-2.82028550483744));
#43610=CARTESIAN_POINT('Ctrl Pts',(2.54012272520141,-1.,-2.82552167649157));
#43611=CARTESIAN_POINT('Ctrl Pts',(2.54604736792542,-1.,-2.83044254225794));
#43612=CARTESIAN_POINT('Ctrl Pts',(2.55182152806964,-1.,-2.83505269592412));
#43613=CARTESIAN_POINT('Ctrl Pts',(2.55749952145165,-1.,-2.83942515220699));
#43614=CARTESIAN_POINT('Ctrl Pts',(2.56316920798489,-1.,-2.84366802680211));
#43615=CARTESIAN_POINT('Ctrl Pts',(2.56891984251743,-1.,-2.84788893329091));
#43616=CARTESIAN_POINT('Ctrl Pts',(2.57480482727128,-1.,-2.85215360144483));
#43617=CARTESIAN_POINT('Ctrl Pts',(2.58082875254407,-1.,-2.85647171715147));
#43618=CARTESIAN_POINT('Ctrl Pts',(2.5869677064356,-1.,-2.86081999003668));
#43619=CARTESIAN_POINT('Ctrl Pts',(2.59318160184921,-1.,-2.86515629953528));
#43620=CARTESIAN_POINT('Ctrl Pts',(2.59942875223202,-1.,-2.86943633170712));
#43621=CARTESIAN_POINT('Ctrl Pts',(2.6056817788128,-1.,-2.87363176656475));
#43622=CARTESIAN_POINT('Ctrl Pts',(2.61193507170928,-1.,-2.87773881947885));
#43623=CARTESIAN_POINT('Ctrl Pts',(2.61819596473087,-1.,-2.88176821427502));
#43624=CARTESIAN_POINT('Ctrl Pts',(2.62447947640253,-1.,-2.88573922195049));
#43625=CARTESIAN_POINT('Ctrl Pts',(2.63080195420771,-1.,-2.88967244854243));
#43626=CARTESIAN_POINT('Ctrl Pts',(2.63717442263944,-1.,-2.89358228854557));
#43627=CARTESIAN_POINT('Ctrl Pts',(2.64359851684146,-1.,-2.89747231723361));
#43628=CARTESIAN_POINT('Ctrl Pts',(2.65007017365576,-1.,-2.90133950224879));
#43629=CARTESIAN_POINT('Ctrl Pts',(2.65658188464287,-1.,-2.90517678087467));
#43630=CARTESIAN_POINT('Ctrl Pts',(2.66312542616808,-1.,-2.90897617968921));
#43631=CARTESIAN_POINT('Ctrl Pts',(2.66969458792627,-1.,-2.91273193382876));
#43632=CARTESIAN_POINT('Ctrl Pts',(2.67628728855309,-1.,-2.91644290704281));
#43633=CARTESIAN_POINT('Ctrl Pts',(2.68290409279689,-1.,-2.92011090722152));
#43634=CARTESIAN_POINT('Ctrl Pts',(2.68954721165342,-1.,-2.92373955325876));
#43635=CARTESIAN_POINT('Ctrl Pts',(2.69621932864302,-1.,-2.92733294395268));
#43636=CARTESIAN_POINT('Ctrl Pts',(2.70292247416881,-1.,-2.93089438233746));
#43637=CARTESIAN_POINT('Ctrl Pts',(2.70965695523776,-1.,-2.93442516311168));
#43638=CARTESIAN_POINT('Ctrl Pts',(2.71642190053575,-1.,-2.93792519474955));
#43639=CARTESIAN_POINT('Ctrl Pts',(2.72321571511322,-1.,-2.94139351933882));
#43640=CARTESIAN_POINT('Ctrl Pts',(2.73003657371613,-1.,-2.94482887675139));
#43641=CARTESIAN_POINT('Ctrl Pts',(2.73688288329825,-1.,-2.94823023414381));
#43642=CARTESIAN_POINT('Ctrl Pts',(2.7437537949221,-1.,-2.95159737214305));
#43643=CARTESIAN_POINT('Ctrl Pts',(2.75064903318996,-1.,-2.95493069316211));
#43644=CARTESIAN_POINT('Ctrl Pts',(2.75756867888393,-1.,-2.9582309766594));
#43645=CARTESIAN_POINT('Ctrl Pts',(2.76451296269571,-1.,-2.96149914764832));
#43646=CARTESIAN_POINT('Ctrl Pts',(2.77148206836464,-1.,-2.96473605585548));
#43647=CARTESIAN_POINT('Ctrl Pts',(2.77847589542767,-1.,-2.9679422104295));
#43648=CARTESIAN_POINT('Ctrl Pts',(2.78549409123657,-1.,-2.97111781461349));
#43649=CARTESIAN_POINT('Ctrl Pts',(2.79253615718147,-1.,-2.97426288347475));
#43650=CARTESIAN_POINT('Ctrl Pts',(2.79960153278186,-1.,-2.97737733718242));
#43651=CARTESIAN_POINT('Ctrl Pts',(2.80668968101162,-1.,-2.98046109647299));
#43652=CARTESIAN_POINT('Ctrl Pts',(2.81380019196454,-1.,-2.9835141977994));
#43653=CARTESIAN_POINT('Ctrl Pts',(2.82093279065704,-1.,-2.98653680669434));
#43654=CARTESIAN_POINT('Ctrl Pts',(2.82808728190402,-1.,-2.98952916401699));
#43655=CARTESIAN_POINT('Ctrl Pts',(2.83526351254383,-1.,-2.99249155170479));
#43656=CARTESIAN_POINT('Ctrl Pts',(2.84246132984334,-1.,-2.995424253416));
#43657=CARTESIAN_POINT('Ctrl Pts',(2.84968053289104,-1.,-2.99832751144566));
#43658=CARTESIAN_POINT('Ctrl Pts',(2.85692085715129,-1.,-3.0012015079552));
#43659=CARTESIAN_POINT('Ctrl Pts',(2.86418200833065,-1.,-3.00404638316245));
#43660=CARTESIAN_POINT('Ctrl Pts',(2.87146368430104,-1.,-3.00686224485374));
#43661=CARTESIAN_POINT('Ctrl Pts',(2.87876560072799,-1.,-3.0096491810855));
#43662=CARTESIAN_POINT('Ctrl Pts',(2.88608751706796,-1.,-3.01240727309568));
#43663=CARTESIAN_POINT('Ctrl Pts',(2.8934292556764,-1.,-3.01513660433291));
#43664=CARTESIAN_POINT('Ctrl Pts',(2.90079069102661,-1.,-3.01783725123646));
#43665=CARTESIAN_POINT('Ctrl Pts',(2.90669553303902,-1.,-3.01997487194926));
#43666=CARTESIAN_POINT('Ctrl Pts',(2.91113297349052,-1.,-3.02156522743299));
#43667=CARTESIAN_POINT('Ctrl Pts',(2.91409518070707,-1.,-3.02261975104912));
#43668=CARTESIAN_POINT('Ctrl Pts',(2.91557726271063,-1.,-3.02314558451372));
#43669=CARTESIAN_POINT('',(3.02314558451372,-1.,-2.91557726271063));
#43670=CARTESIAN_POINT('',(2.91557726271063,-1.,-3.02314558451372));
#43671=CARTESIAN_POINT('',(2.79140942341258,-1.,-2.50410331873176));
#43672=CARTESIAN_POINT('Ctrl Pts',(3.02314558451372,-1.,-2.91557726271063));
#43673=CARTESIAN_POINT('Ctrl Pts',(3.02261975104593,-1.,-2.91409518070399));
#43674=CARTESIAN_POINT('Ctrl Pts',(3.02156522742431,-1.,-2.91113297348212));
#43675=CARTESIAN_POINT('Ctrl Pts',(3.01997487193503,-1.,-2.90669553302526));
#43676=CARTESIAN_POINT('Ctrl Pts',(3.01783725121981,-1.,-2.9007906910105));
#43677=CARTESIAN_POINT('Ctrl Pts',(3.01513660431928,-1.,-2.89342925566321));
#43678=CARTESIAN_POINT('Ctrl Pts',(3.01240727308829,-1.,-2.8860875170608));
#43679=CARTESIAN_POINT('Ctrl Pts',(3.00964918108476,-1.,-2.87876560072727));
#43680=CARTESIAN_POINT('Ctrl Pts',(3.00686224485784,-1.,-2.87146368430502));
#43681=CARTESIAN_POINT('Ctrl Pts',(3.00404638316867,-1.,-2.86418200833667));
#43682=CARTESIAN_POINT('Ctrl Pts',(3.00120150796095,-1.,-2.85692085715686));
#43683=CARTESIAN_POINT('Ctrl Pts',(2.99832751144925,-1.,-2.84968053289451));
#43684=CARTESIAN_POINT('Ctrl Pts',(2.99542425341685,-1.,-2.84246132984415));
#43685=CARTESIAN_POINT('Ctrl Pts',(2.99249155170339,-1.,-2.83526351254248));
#43686=CARTESIAN_POINT('Ctrl Pts',(2.98952916401446,-1.,-2.82808728190157));
#43687=CARTESIAN_POINT('Ctrl Pts',(2.9865368066918,-1.,-2.82093279065457));
#43688=CARTESIAN_POINT('Ctrl Pts',(2.98351419779767,-1.,-2.81380019196286));
#43689=CARTESIAN_POINT('Ctrl Pts',(2.98046109647241,-1.,-2.80668968101106));
#43690=CARTESIAN_POINT('Ctrl Pts',(2.97737733718287,-1.,-2.7996015327823));
#43691=CARTESIAN_POINT('Ctrl Pts',(2.9742628834758,-1.,-2.79253615718248));
#43692=CARTESIAN_POINT('Ctrl Pts',(2.97111781461465,-1.,-2.78549409123769));
#43693=CARTESIAN_POINT('Ctrl Pts',(2.96794221043036,-1.,-2.7784758954285));
#43694=CARTESIAN_POINT('Ctrl Pts',(2.96473605585583,-1.,-2.77148206836498));
#43695=CARTESIAN_POINT('Ctrl Pts',(2.96149914764818,-1.,-2.76451296269557));
#43696=CARTESIAN_POINT('Ctrl Pts',(2.95823097665896,-1.,-2.7575686788835));
#43697=CARTESIAN_POINT('Ctrl Pts',(2.95493069316161,-1.,-2.75064903318947));
#43698=CARTESIAN_POINT('Ctrl Pts',(2.95159737214266,-1.,-2.74375379492172));
#43699=CARTESIAN_POINT('Ctrl Pts',(2.94823023414364,-1.,-2.73688288329808));
#43700=CARTESIAN_POINT('Ctrl Pts',(2.94482887675143,-1.,-2.73003657371617));
#43701=CARTESIAN_POINT('Ctrl Pts',(2.94139351933897,-1.,-2.72321571511337));
#43702=CARTESIAN_POINT('Ctrl Pts',(2.93792519474972,-1.,-2.71642190053592));
#43703=CARTESIAN_POINT('Ctrl Pts',(2.93442516311179,-1.,-2.70965695523787));
#43704=CARTESIAN_POINT('Ctrl Pts',(2.93089438233749,-1.,-2.70292247416885));
#43705=CARTESIAN_POINT('Ctrl Pts',(2.92733294395267,-1.,-2.69621932864301));
#43706=CARTESIAN_POINT('Ctrl Pts',(2.92373955325875,-1.,-2.68954721165339));
#43707=CARTESIAN_POINT('Ctrl Pts',(2.92011090722152,-1.,-2.68290409279688));
#43708=CARTESIAN_POINT('Ctrl Pts',(2.91644290704285,-1.,-2.67628728855312));
#43709=CARTESIAN_POINT('Ctrl Pts',(2.91273193382882,-1.,-2.66969458792631));
#43710=CARTESIAN_POINT('Ctrl Pts',(2.90897617968923,-1.,-2.6631254261681));
#43711=CARTESIAN_POINT('Ctrl Pts',(2.90517678087461,-1.,-2.65658188464282));
#43712=CARTESIAN_POINT('Ctrl Pts',(2.90133950224867,-1.,-2.65007017365564));
#43713=CARTESIAN_POINT('Ctrl Pts',(2.89747231723345,-1.,-2.64359851684131));
#43714=CARTESIAN_POINT('Ctrl Pts',(2.89358228854544,-1.,-2.63717442263932));
#43715=CARTESIAN_POINT('Ctrl Pts',(2.88967244854239,-1.,-2.63080195420767));
#43716=CARTESIAN_POINT('Ctrl Pts',(2.88573922195059,-1.,-2.62447947640262));
#43717=CARTESIAN_POINT('Ctrl Pts',(2.88176821427525,-1.,-2.61819596473108));
#43718=CARTESIAN_POINT('Ctrl Pts',(2.87773881947915,-1.,-2.61193507170955));
#43719=CARTESIAN_POINT('Ctrl Pts',(2.87363176656501,-1.,-2.60568177881303));
#43720=CARTESIAN_POINT('Ctrl Pts',(2.86943633170722,-1.,-2.5994287522321));
#43721=CARTESIAN_POINT('Ctrl Pts',(2.86515629953513,-1.,-2.59318160184908));
#43722=CARTESIAN_POINT('Ctrl Pts',(2.86081999003629,-1.,-2.58696770643524));
#43723=CARTESIAN_POINT('Ctrl Pts',(2.85647171715092,-1.,-2.58082875254357));
#43724=CARTESIAN_POINT('Ctrl Pts',(2.85215360144431,-1.,-2.57480482727081));
#43725=CARTESIAN_POINT('Ctrl Pts',(2.84788893329067,-1.,-2.56891984251721));
#43726=CARTESIAN_POINT('Ctrl Pts',(2.84366802680237,-1.,-2.56316920798513));
#43727=CARTESIAN_POINT('Ctrl Pts',(2.83942515220782,-1.,-2.55749952145241));
#43728=CARTESIAN_POINT('Ctrl Pts',(2.83505269592536,-1.,-2.55182152807077));
#43729=CARTESIAN_POINT('Ctrl Pts',(2.83044254225917,-1.,-2.54604736792655));
#43730=CARTESIAN_POINT('Ctrl Pts',(2.8255216764922,-1.,-2.54012272520199));
#43731=CARTESIAN_POINT('Ctrl Pts',(2.82028550483689,-1.,-2.53405679667412));
#43732=CARTESIAN_POINT('Ctrl Pts',(2.81484379048475,-1.,-2.52796388055278));
#43733=CARTESIAN_POINT('Ctrl Pts',(2.80941521966941,-1.,-2.52205778589653));
#43734=CARTESIAN_POINT('Ctrl Pts',(2.80427363984653,-1.,-2.51660190465805));
#43735=CARTESIAN_POINT('Ctrl Pts',(2.79970585014168,-1.,-2.51186983687818));
#43736=CARTESIAN_POINT('Ctrl Pts',(2.79596878057287,-1.,-2.50810555977671));
#43737=CARTESIAN_POINT('Ctrl Pts',(2.79344192164147,-1.,-2.50567182569081));
#43738=CARTESIAN_POINT('Ctrl Pts',(2.79217568804755,-1.,-2.50455968395146));
#43739=CARTESIAN_POINT('Ctrl Pts',(2.79164172518905,-1.,-2.50417932839313));
#43740=CARTESIAN_POINT('Ctrl Pts',(2.79145823440781,-1.,-2.50410700351493));
#43741=CARTESIAN_POINT('Ctrl Pts',(2.79140942341258,-1.,-2.50410331873176));
#43742=CARTESIAN_POINT('',(2.90994629141562,-1.,-2.36531447826213));
#43743=CARTESIAN_POINT('Origin',(0.,-1.,0.));
#43744=CARTESIAN_POINT('',(3.35260583073571,-1.,-2.52982887637028));
#43745=CARTESIAN_POINT('Ctrl Pts',(2.90994629141562,-1.,-2.36531447826213));
#43746=CARTESIAN_POINT('Ctrl Pts',(2.90995756655558,-1.,-2.3653621118858));
#43747=CARTESIAN_POINT('Ctrl Pts',(2.9100577052777,-1.,-2.36553202948741));
#43748=CARTESIAN_POINT('Ctrl Pts',(2.91051690822262,-1.,-2.36599991765853));
#43749=CARTESIAN_POINT('Ctrl Pts',(2.91181344022628,-1.,-2.36707658451709));
#43750=CARTESIAN_POINT('Ctrl Pts',(2.91461249883016,-1.,-2.36919161373074));
#43751=CARTESIAN_POINT('Ctrl Pts',(2.9189150379156,-1.,-2.37229381109939));
#43752=CARTESIAN_POINT('Ctrl Pts',(2.92430340582912,-1.,-2.37606510524271));
#43753=CARTESIAN_POINT('Ctrl Pts',(2.93049643640517,-1.,-2.3802898958232));
#43754=CARTESIAN_POINT('Ctrl Pts',(2.93717903280599,-1.,-2.38472771516476));
#43755=CARTESIAN_POINT('Ctrl Pts',(2.94404820669135,-1.,-2.38914929090806));
#43756=CARTESIAN_POINT('Ctrl Pts',(2.95085857128372,-1.,-2.39337207631613));
#43757=CARTESIAN_POINT('Ctrl Pts',(2.95748006482811,-1.,-2.39730553974412));
#43758=CARTESIAN_POINT('Ctrl Pts',(2.9639043224018,-1.,-2.40095565711535));
#43759=CARTESIAN_POINT('Ctrl Pts',(2.97019641312272,-1.,-2.40438604734848));
#43760=CARTESIAN_POINT('Ctrl Pts',(2.97646002822395,-1.,-2.40768975073691));
#43761=CARTESIAN_POINT('Ctrl Pts',(2.98280015815132,-1.,-2.41095909342591));
#43762=CARTESIAN_POINT('Ctrl Pts',(2.98927983005851,-1.,-2.4142506419963));
#43763=CARTESIAN_POINT('Ctrl Pts',(2.99590509293561,-1.,-2.4175732450056));
#43764=CARTESIAN_POINT('Ctrl Pts',(3.00264868586038,-1.,-2.42090763946812));
#43765=CARTESIAN_POINT('Ctrl Pts',(3.00946442616674,-1.,-2.42421849439625));
#43766=CARTESIAN_POINT('Ctrl Pts',(3.01630420830493,-1.,-2.4274685626416));
#43767=CARTESIAN_POINT('Ctrl Pts',(3.02313656035977,-1.,-2.43063415586615));
#43768=CARTESIAN_POINT('Ctrl Pts',(3.02995534946946,-1.,-2.43371241361462));
#43769=CARTESIAN_POINT('Ctrl Pts',(3.03676949672797,-1.,-2.43671278042394));
#43770=CARTESIAN_POINT('Ctrl Pts',(3.04359685040545,-1.,-2.43965194061849));
#43771=CARTESIAN_POINT('Ctrl Pts',(3.05045678021509,-1.,-2.44254768923109));
#43772=CARTESIAN_POINT('Ctrl Pts',(3.05736242671521,-1.,-2.44541251892568));
#43773=CARTESIAN_POINT('Ctrl Pts',(3.06431596421422,-1.,-2.44824970516558));
#43774=CARTESIAN_POINT('Ctrl Pts',(3.0713129052131,-1.,-2.45105688854432));
#43775=CARTESIAN_POINT('Ctrl Pts',(3.07834472886145,-1.,-2.45382826787795));
#43776=CARTESIAN_POINT('Ctrl Pts',(3.08540206545313,-1.,-2.45655725437037));
#43777=CARTESIAN_POINT('Ctrl Pts',(3.09247787931881,-1.,-2.45923912563875));
#43778=CARTESIAN_POINT('Ctrl Pts',(3.09956993697048,-1.,-2.4618730850188));
#43779=CARTESIAN_POINT('Ctrl Pts',(3.10667907901981,-1.,-2.46446082979645));
#43780=CARTESIAN_POINT('Ctrl Pts',(3.11380805536124,-1.,-2.46700558843507));
#43781=CARTESIAN_POINT('Ctrl Pts',(3.12096015766984,-1.,-2.4695109894747));
#43782=CARTESIAN_POINT('Ctrl Pts',(3.12813790805948,-1.,-2.47197997765868));
#43783=CARTESIAN_POINT('Ctrl Pts',(3.13534181229282,-1.,-2.47441378371923));
#43784=CARTESIAN_POINT('Ctrl Pts',(3.14257099546531,-1.,-2.47681245356095));
#43785=CARTESIAN_POINT('Ctrl Pts',(3.14982373241335,-1.,-2.47917529057016));
#43786=CARTESIAN_POINT('Ctrl Pts',(3.15709802322735,-1.,-2.48150133566568));
#43787=CARTESIAN_POINT('Ctrl Pts',(3.16439213290181,-1.,-2.48378981792739));
#43788=CARTESIAN_POINT('Ctrl Pts',(3.17170518863357,-1.,-2.48604065348619));
#43789=CARTESIAN_POINT('Ctrl Pts',(3.17903698136678,-1.,-2.48825428288243));
#43790=CARTESIAN_POINT('Ctrl Pts',(3.18638771282315,-1.,-2.49043146334095));
#43791=CARTESIAN_POINT('Ctrl Pts',(3.19375775555814,-1.,-2.4925730723986));
#43792=CARTESIAN_POINT('Ctrl Pts',(3.20114742397549,-1.,-2.49467992057726));
#43793=CARTESIAN_POINT('Ctrl Pts',(3.2085566984974,-1.,-2.49675252647298));
#43794=CARTESIAN_POINT('Ctrl Pts',(3.21598526261157,-1.,-2.49879114599293));
#43795=CARTESIAN_POINT('Ctrl Pts',(3.22343262620387,-1.,-2.5007958720187));
#43796=CARTESIAN_POINT('Ctrl Pts',(3.23089822320596,-1.,-2.50276671338074));
#43797=CARTESIAN_POINT('Ctrl Pts',(3.23838151080383,-1.,-2.50470367580078));
#43798=CARTESIAN_POINT('Ctrl Pts',(3.24588208984042,-1.,-2.50660685940645));
#43799=CARTESIAN_POINT('Ctrl Pts',(3.25339971461265,-1.,-2.50847647070936));
#43800=CARTESIAN_POINT('Ctrl Pts',(3.26093423001716,-1.,-2.51031277813697));
#43801=CARTESIAN_POINT('Ctrl Pts',(3.26848552888271,-1.,-2.51211608411539));
#43802=CARTESIAN_POINT('Ctrl Pts',(3.27605350473048,-1.,-2.51388669270329));
#43803=CARTESIAN_POINT('Ctrl Pts',(3.28363799702583,-1.,-2.51562487464215));
#43804=CARTESIAN_POINT('Ctrl Pts',(3.2912387729863,-1.,-2.51733085123316));
#43805=CARTESIAN_POINT('Ctrl Pts',(3.29885556387661,-1.,-2.51900480700548));
#43806=CARTESIAN_POINT('Ctrl Pts',(3.30648808814986,-1.,-2.52064689568167));
#43807=CARTESIAN_POINT('Ctrl Pts',(3.31413607874727,-1.,-2.52225724871375));
#43808=CARTESIAN_POINT('Ctrl Pts',(3.32179931079521,-1.,-2.52383598396878));
#43809=CARTESIAN_POINT('Ctrl Pts',(3.32947762189049,-1.,-2.52538321165774));
#43810=CARTESIAN_POINT('Ctrl Pts',(3.33717090000955,-1.,-2.52689902691551));
#43811=CARTESIAN_POINT('Ctrl Pts',(3.34333744117093,-1.,-2.52808660916879));
#43812=CARTESIAN_POINT('Ctrl Pts',(3.34796903577628,-1.,-2.5289632161143));
#43813=CARTESIAN_POINT('Ctrl Pts',(3.35105973714426,-1.,-2.52954136549357));
#43814=CARTESIAN_POINT('Ctrl Pts',(3.35260583073571,-1.,-2.52982887637028));
#43815=CARTESIAN_POINT('',(3.44202241512147,-1.,-2.40675750623143));
#43816=CARTESIAN_POINT('',(3.35260583073571,-1.,-2.52982887637028));
#43817=CARTESIAN_POINT('',(3.14877060440327,-1.,-2.03660101169714));
#43818=CARTESIAN_POINT('Ctrl Pts',(3.44202241512147,-1.,-2.40675750623143));
#43819=CARTESIAN_POINT('Ctrl Pts',(3.44127120683039,-1.,-2.4053759295909));
#43820=CARTESIAN_POINT('Ctrl Pts',(3.43976627484234,-1.,-2.40261515589405));
#43821=CARTESIAN_POINT('Ctrl Pts',(3.43750133064416,-1.,-2.39848113410292));
#43822=CARTESIAN_POINT('Ctrl Pts',(3.4344663067854,-1.,-2.39298338804493));
#43823=CARTESIAN_POINT('Ctrl Pts',(3.43064732712919,-1.,-2.38613505843552));
#43824=CARTESIAN_POINT('Ctrl Pts',(3.42680309754399,-1.,-2.37931067028926));
#43825=CARTESIAN_POINT('Ctrl Pts',(3.42293356216511,-1.,-2.37251035954292));
#43826=CARTESIAN_POINT('Ctrl Pts',(3.41903866635852,-1.,-2.36573431470642));
#43827=CARTESIAN_POINT('Ctrl Pts',(3.41511836751469,-1.,-2.35898278606946));
#43828=CARTESIAN_POINT('Ctrl Pts',(3.41117262314119,-1.,-2.35225606824109));
#43829=CARTESIAN_POINT('Ctrl Pts',(3.40720137404297,-1.,-2.34555447649188));
#43830=CARTESIAN_POINT('Ctrl Pts',(3.40320452776743,-1.,-2.33887832342782));
#43831=CARTESIAN_POINT('Ctrl Pts',(3.39918194577956,-1.,-2.33222789882489));
#43832=CARTESIAN_POINT('Ctrl Pts',(3.39513342019756,-1.,-2.3256034390248));
#43833=CARTESIAN_POINT('Ctrl Pts',(3.39105869474822,-1.,-2.31900513925424));
#43834=CARTESIAN_POINT('Ctrl Pts',(3.38695751492462,-1.,-2.31243319489367));
#43835=CARTESIAN_POINT('Ctrl Pts',(3.3828296733661,-1.,-2.30588783640343));
#43836=CARTESIAN_POINT('Ctrl Pts',(3.37867504959433,-1.,-2.29936936127624));
#43837=CARTESIAN_POINT('Ctrl Pts',(3.37449367172826,-1.,-2.29287818007393));
#43838=CARTESIAN_POINT('Ctrl Pts',(3.37028570206488,-1.,-2.28641481081137));
#43839=CARTESIAN_POINT('Ctrl Pts',(3.36605130713076,-1.,-2.27997979458037));
#43840=CARTESIAN_POINT('Ctrl Pts',(3.36179055004409,-1.,-2.2735736262093));
#43841=CARTESIAN_POINT('Ctrl Pts',(3.35750328523061,-1.,-2.2671966857991));
#43842=CARTESIAN_POINT('Ctrl Pts',(3.35318902552626,-1.,-2.26084915222449));
#43843=CARTESIAN_POINT('Ctrl Pts',(3.34884690292285,-1.,-2.25453097693483));
#43844=CARTESIAN_POINT('Ctrl Pts',(3.34447596770723,-1.,-2.24824207678256));
#43845=CARTESIAN_POINT('Ctrl Pts',(3.34007543738025,-1.,-2.24198249391422));
#43846=CARTESIAN_POINT('Ctrl Pts',(3.33564495756481,-1.,-2.23575256328812));
#43847=CARTESIAN_POINT('Ctrl Pts',(3.33118487773611,-1.,-2.22955308907233));
#43848=CARTESIAN_POINT('Ctrl Pts',(3.3266964672289,-1.,-2.22338548312772));
#43849=CARTESIAN_POINT('Ctrl Pts',(3.32218125618968,-1.,-2.21725135110898));
#43850=CARTESIAN_POINT('Ctrl Pts',(3.31764044024235,-1.,-2.21115211847875));
#43851=CARTESIAN_POINT('Ctrl Pts',(3.31307424608949,-1.,-2.20508863150607));
#43852=CARTESIAN_POINT('Ctrl Pts',(3.30848134694595,-1.,-2.19906078949923));
#43853=CARTESIAN_POINT('Ctrl Pts',(3.30385816281831,-1.,-2.19306710376111));
#43854=CARTESIAN_POINT('Ctrl Pts',(3.29920022557639,-1.,-2.18710556500327));
#43855=CARTESIAN_POINT('Ctrl Pts',(3.2945036150049,-1.,-2.18117455557065));
#43856=CARTESIAN_POINT('Ctrl Pts',(3.28976645712568,-1.,-2.17527380048423));
#43857=CARTESIAN_POINT('Ctrl Pts',(3.28499019979724,-1.,-2.16940517773455));
#43858=CARTESIAN_POINT('Ctrl Pts',(3.280181508414,-1.,-2.16357391934425));
#43859=CARTESIAN_POINT('Ctrl Pts',(3.27534954469187,-1.,-2.15778690038347));
#43860=CARTESIAN_POINT('Ctrl Pts',(3.27050245897228,-1.,-2.15205043199808));
#43861=CARTESIAN_POINT('Ctrl Pts',(3.26564388189759,-1.,-2.1463680529566));
#43862=CARTESIAN_POINT('Ctrl Pts',(3.26077002641879,-1.,-2.14073870754264));
#43863=CARTESIAN_POINT('Ctrl Pts',(3.25586495065054,-1.,-2.13515375878803));
#43864=CARTESIAN_POINT('Ctrl Pts',(3.25090574494028,-1.,-2.12960028396832));
#43865=CARTESIAN_POINT('Ctrl Pts',(3.24587102613376,-1.,-2.12406646410962));
#43866=CARTESIAN_POINT('Ctrl Pts',(3.24074905517293,-1.,-2.11854673326979));
#43867=CARTESIAN_POINT('Ctrl Pts',(3.23554444767099,-1.,-2.11304604021773));
#43868=CARTESIAN_POINT('Ctrl Pts',(3.23028945793289,-1.,-2.10758699642451));
#43869=CARTESIAN_POINT('Ctrl Pts',(3.22503437553434,-1.,-2.10220384298492));
#43870=CARTESIAN_POINT('Ctrl Pts',(3.21982707347009,-1.,-2.09692958434895));
#43871=CARTESIAN_POINT('Ctrl Pts',(3.21469429601654,-1.,-2.09178419460443));
#43872=CARTESIAN_POINT('Ctrl Pts',(3.20962575845463,-1.,-2.08676465517455));
#43873=CARTESIAN_POINT('Ctrl Pts',(3.2045481863073,-1.,-2.08182850370878));
#43874=CARTESIAN_POINT('Ctrl Pts',(3.19934132836019,-1.,-2.07690441870722));
#43875=CARTESIAN_POINT('Ctrl Pts',(3.19388465568252,-1.,-2.07192253497857));
#43876=CARTESIAN_POINT('Ctrl Pts',(3.18809755562368,-1.,-2.06684062744112));
#43877=CARTESIAN_POINT('Ctrl Pts',(3.18197692964614,-1.,-2.06166849827101));
#43878=CARTESIAN_POINT('Ctrl Pts',(3.17564906975371,-1.,-2.05650186773132));
#43879=CARTESIAN_POINT('Ctrl Pts',(3.16936341689527,-1.,-2.05151770247233));
#43880=CARTESIAN_POINT('Ctrl Pts',(3.16343165058912,-1.,-2.04693331247446));
#43881=CARTESIAN_POINT('Ctrl Pts',(3.15817983946367,-1.,-2.04297406404027));
#43882=CARTESIAN_POINT('Ctrl Pts',(3.15389991674792,-1.,-2.03984073791519));
#43883=CARTESIAN_POINT('Ctrl Pts',(3.15102344775328,-1.,-2.03783225495961));
#43884=CARTESIAN_POINT('Ctrl Pts',(3.14959882629805,-1.,-2.03693188810545));
#43885=CARTESIAN_POINT('Ctrl Pts',(3.1490119366901,-1.,-2.03663974554932));
#43886=CARTESIAN_POINT('Ctrl Pts',(3.14881939088124,-1.,-2.03659701539259));
#43887=CARTESIAN_POINT('Ctrl Pts',(3.14877060440327,-1.,-2.03660101169714));
#43888=CARTESIAN_POINT('',(3.24413672884812,-1.,-1.88097764062697));
#43889=CARTESIAN_POINT('Origin',(0.,-1.,0.));
#43890=CARTESIAN_POINT('',(3.70708211654725,-1.,-1.97421938526992));
#43891=CARTESIAN_POINT('Ctrl Pts',(3.24413672884812,-1.,-1.88097764062697));
#43892=CARTESIAN_POINT('Ctrl Pts',(3.24415531671284,-1.,-1.8810229239812));
#43893=CARTESIAN_POINT('Ctrl Pts',(3.24428080353022,-1.,-1.88117508446775));
#43894=CARTESIAN_POINT('Ctrl Pts',(3.24480754676064,-1.,-1.88156537699203));
#43895=CARTESIAN_POINT('Ctrl Pts',(3.2462565441079,-1.,-1.88242596600454));
#43896=CARTESIAN_POINT('Ctrl Pts',(3.24935200511918,-1.,-1.88407708646357));
#43897=CARTESIAN_POINT('Ctrl Pts',(3.25408686339463,-1.,-1.88646802523466));
#43898=CARTESIAN_POINT('Ctrl Pts',(3.25999885193947,-1.,-1.88934996203698));
#43899=CARTESIAN_POINT('Ctrl Pts',(3.26677653888676,-1.,-1.89255393500965));
#43900=CARTESIAN_POINT('Ctrl Pts',(3.27407108933139,-1.,-1.89589172903793));
#43901=CARTESIAN_POINT('Ctrl Pts',(3.28154737912352,-1.,-1.89918429230462));
#43902=CARTESIAN_POINT('Ctrl Pts',(3.2889344860029,-1.,-1.90228971247527));
#43903=CARTESIAN_POINT('Ctrl Pts',(3.29608978722113,-1.,-1.90513891864087));
#43904=CARTESIAN_POINT('Ctrl Pts',(3.30300595568195,-1.,-1.90773912171341));
#43905=CARTESIAN_POINT('Ctrl Pts',(3.30975721158596,-1.,-1.91014297830446));
#43906=CARTESIAN_POINT('Ctrl Pts',(3.31646052426364,-1.,-1.91242616234442));
#43907=CARTESIAN_POINT('Ctrl Pts',(3.32323403454535,-1.,-1.91466343916628));
#43908=CARTESIAN_POINT('Ctrl Pts',(3.33014884257873,-1.,-1.91690081930332));
#43909=CARTESIAN_POINT('Ctrl Pts',(3.33721230710012,-1.,-1.9191460961021));
#43910=CARTESIAN_POINT('Ctrl Pts',(3.34439448941961,-1.,-1.92138450828404));
#43911=CARTESIAN_POINT('Ctrl Pts',(3.35164424847223,-1.,-1.92358838440528));
#43912=CARTESIAN_POINT('Ctrl Pts',(3.35890824422965,-1.,-1.92572846125756));
#43913=CARTESIAN_POINT('Ctrl Pts',(3.36615168657567,-1.,-1.92778626543786));
#43914=CARTESIAN_POINT('Ctrl Pts',(3.37336807068043,-1.,-1.92975993109877));
#43915=CARTESIAN_POINT('Ctrl Pts',(3.3805676852555,-1.,-1.93165739093276));
#43916=CARTESIAN_POINT('Ctrl Pts',(3.38777076883256,-1.,-1.93349233176788));
#43917=CARTESIAN_POINT('Ctrl Pts',(3.39499923640795,-1.,-1.93527929945985));
#43918=CARTESIAN_POINT('Ctrl Pts',(3.40226802104109,-1.,-1.93702857723098));
#43919=CARTESIAN_POINT('Ctrl Pts',(3.40957978266642,-1.,-1.93874306008143));
#43920=CARTESIAN_POINT('Ctrl Pts',(3.41692971994096,-1.,-1.94042111965246));
#43921=CARTESIAN_POINT('Ctrl Pts',(3.42430850941503,-1.,-1.94205835913696));
#43922=CARTESIAN_POINT('Ctrl Pts',(3.43170586602434,-1.,-1.94364973660284));
#43923=CARTESIAN_POINT('Ctrl Pts',(3.43911410197687,-1.,-1.94519168842879));
#43924=CARTESIAN_POINT('Ctrl Pts',(3.44653088665681,-1.,-1.94668377715329));
#43925=CARTESIAN_POINT('Ctrl Pts',(3.45395731584051,-1.,-1.94812754766524));
#43926=CARTESIAN_POINT('Ctrl Pts',(3.46139661060962,-1.,-1.94952575850197));
#43927=CARTESIAN_POINT('Ctrl Pts',(3.46885258974191,-1.,-1.95088147859877));
#43928=CARTESIAN_POINT('Ctrl Pts',(3.47632820495921,-1.,-1.95219722189876));
#43929=CARTESIAN_POINT('Ctrl Pts',(3.48382414832634,-1.,-1.95347412486309));
#43930=CARTESIAN_POINT('Ctrl Pts',(3.49133956289133,-1.,-1.95471236969643));
#43931=CARTESIAN_POINT('Ctrl Pts',(3.49887263575583,-1.,-1.95591153823661));
#43932=CARTESIAN_POINT('Ctrl Pts',(3.50642124159909,-1.,-1.95707099606511));
#43933=CARTESIAN_POINT('Ctrl Pts',(3.51398354617794,-1.,-1.95819025316779));
#43934=CARTESIAN_POINT('Ctrl Pts',(3.52155867431486,-1.,-1.95926936324461));
#43935=CARTESIAN_POINT('Ctrl Pts',(3.52914648844351,-1.,-1.96030879411566));
#43936=CARTESIAN_POINT('Ctrl Pts',(3.53674730625813,-1.,-1.96130926212689));
#43937=CARTESIAN_POINT('Ctrl Pts',(3.54436163300443,-1.,-1.96227157573067));
#43938=CARTESIAN_POINT('Ctrl Pts',(3.55198990600886,-1.,-1.96319648628644));
#43939=CARTESIAN_POINT('Ctrl Pts',(3.55963218706096,-1.,-1.96408450906812));
#43940=CARTESIAN_POINT('Ctrl Pts',(3.56728820357791,-1.,-1.96493594634567));
#43941=CARTESIAN_POINT('Ctrl Pts',(3.57495748600959,-1.,-1.96575096652789));
#43942=CARTESIAN_POINT('Ctrl Pts',(3.58263947663829,-1.,-1.96652966688911));
#43943=CARTESIAN_POINT('Ctrl Pts',(3.59033364022801,-1.,-1.96727213799544));
#43944=CARTESIAN_POINT('Ctrl Pts',(3.59803959819938,-1.,-1.96797854118369));
#43945=CARTESIAN_POINT('Ctrl Pts',(3.60575714017989,-1.,-1.9686491188594));
#43946=CARTESIAN_POINT('Ctrl Pts',(3.61348615496704,-1.,-1.96928416040877));
#43947=CARTESIAN_POINT('Ctrl Pts',(3.62122658401893,-1.,-1.96988398129978));
#43948=CARTESIAN_POINT('Ctrl Pts',(3.62897836973293,-1.,-1.97044889850463));
#43949=CARTESIAN_POINT('Ctrl Pts',(3.63674139590412,-1.,-1.97097920454464));
#43950=CARTESIAN_POINT('Ctrl Pts',(3.64451546723514,-1.,-1.97147515441164));
#43951=CARTESIAN_POINT('Ctrl Pts',(3.652300347166,-1.,-1.9719369724024));
#43952=CARTESIAN_POINT('Ctrl Pts',(3.6600957816636,-1.,-1.9723648543905));
#43953=CARTESIAN_POINT('Ctrl Pts',(3.66790152752075,-1.,-1.97275897198678));
#43954=CARTESIAN_POINT('Ctrl Pts',(3.67571738107084,-1.,-1.97311947678517));
#43955=CARTESIAN_POINT('Ctrl Pts',(3.68354319915092,-1.,-1.97344650304519));
#43956=CARTESIAN_POINT('Ctrl Pts',(3.69137888599902,-1.,-1.97374016225483));
#43957=CARTESIAN_POINT('Ctrl Pts',(3.6976552856004,-1.,-1.97394846383216));
#43958=CARTESIAN_POINT('Ctrl Pts',(3.70236698912904,-1.,-1.97408973726715));
#43959=CARTESIAN_POINT('Ctrl Pts',(3.70551008132332,-1.,-1.97417727645308));
#43960=CARTESIAN_POINT('Ctrl Pts',(3.70708211654725,-1.,-1.97421938526992));
#43961=CARTESIAN_POINT('',(3.77614523045147,-1.,-1.83867539237861));
#43962=CARTESIAN_POINT('',(3.70708211654725,-1.,-1.97421938526992));
#43963=CARTESIAN_POINT('',(3.42859860294305,-1.,-1.5189508286633));
#43964=CARTESIAN_POINT('Ctrl Pts',(3.77614523045147,-1.,-1.83867539237861));
#43965=CARTESIAN_POINT('Ctrl Pts',(3.77518714457833,-1.,-1.83742834010626));
#43966=CARTESIAN_POINT('Ctrl Pts',(3.77326886064398,-1.,-1.83493697934534));
#43967=CARTESIAN_POINT('Ctrl Pts',(3.77038509817999,-1.,-1.83120816955646));
#43968=CARTESIAN_POINT('Ctrl Pts',(3.76652740353775,-1.,-1.82625289220915));
#43969=CARTESIAN_POINT('Ctrl Pts',(3.76168412707948,-1.,-1.82008629694091));
#43970=CARTESIAN_POINT('Ctrl Pts',(3.75681965683071,-1.,-1.8139472983358));
#43971=CARTESIAN_POINT('Ctrl Pts',(3.75193395887977,-1.,-1.80783603939617));
#43972=CARTESIAN_POINT('Ctrl Pts',(3.74702700875467,-1.,-1.8017527148577));
#43973=CARTESIAN_POINT('Ctrl Pts',(3.74209880352445,-1.,-1.79569757859422));
#43974=CARTESIAN_POINT('Ctrl Pts',(3.73714934730681,-1.,-1.78967092823491));
#43975=CARTESIAN_POINT('Ctrl Pts',(3.7321786309547,-1.,-1.78367308442901));
#43976=CARTESIAN_POINT('Ctrl Pts',(3.72718661205609,-1.,-1.77770437039658));
#43977=CARTESIAN_POINT('Ctrl Pts',(3.72217319911254,-1.,-1.77176509401761));
#43978=CARTESIAN_POINT('Ctrl Pts',(3.71713822377359,-1.,-1.76585552124394));
#43979=CARTESIAN_POINT('Ctrl Pts',(3.71208146346136,-1.,-1.75997588498865));
#43980=CARTESIAN_POINT('Ctrl Pts',(3.70700269736659,-1.,-1.75412641804042));
#43981=CARTESIAN_POINT('Ctrl Pts',(3.7019017567335,-1.,-1.74830738046057));
#43982=CARTESIAN_POINT('Ctrl Pts',(3.69677856910517,-1.,-1.74251908492617));
#43983=CARTESIAN_POINT('Ctrl Pts',(3.69163322648036,-1.,-1.73676193254557));
#43984=CARTESIAN_POINT('Ctrl Pts',(3.68646597019332,-1.,-1.73103640956717));
#43985=CARTESIAN_POINT('Ctrl Pts',(3.68127704936579,-1.,-1.72534302437056));
#43986=CARTESIAN_POINT('Ctrl Pts',(3.67606660374709,-1.,-1.71968225581808));
#43987=CARTESIAN_POINT('Ctrl Pts',(3.67083454901611,-1.,-1.71405450210384));
#43988=CARTESIAN_POINT('Ctrl Pts',(3.66558043198876,-1.,-1.70846001610956));
#43989=CARTESIAN_POINT('Ctrl Pts',(3.66030338774847,-1.,-1.70289888566873));
#43990=CARTESIAN_POINT('Ctrl Pts',(3.65500246526749,-1.,-1.69737117722534));
#43991=CARTESIAN_POINT('Ctrl Pts',(3.64967689827371,-1.,-1.69187705481689));
#43992=CARTESIAN_POINT('Ctrl Pts',(3.64432638915203,-1.,-1.68641690471457));
#43993=CARTESIAN_POINT('Ctrl Pts',(3.63895140887462,-1.,-1.68099146651586));
#43994=CARTESIAN_POINT('Ctrl Pts',(3.63355343201232,-1.,-1.67560193613156));
#43995=CARTESIAN_POINT('Ctrl Pts',(3.62813422105271,-1.,-1.67024966008045));
#43996=CARTESIAN_POINT('Ctrl Pts',(3.62269517989109,-1.,-1.66493585923855));
#43997=CARTESIAN_POINT('Ctrl Pts',(3.61723666482456,-1.,-1.65966133399186));
#43998=CARTESIAN_POINT('Ctrl Pts',(3.61175734965127,-1.,-1.65442619244325));
#43999=CARTESIAN_POINT('Ctrl Pts',(3.60625346556992,-1.,-1.64922952425832));
#44000=CARTESIAN_POINT('Ctrl Pts',(3.60072028513845,-1.,-1.64407004385582));
#44001=CARTESIAN_POINT('Ctrl Pts',(3.59515368334893,-1.,-1.63894676675352));
#44002=CARTESIAN_POINT('Ctrl Pts',(3.58955176627879,-1.,-1.6338597145126));
#44003=CARTESIAN_POINT('Ctrl Pts',(3.58391625774343,-1.,-1.62881051550745));
#44004=CARTESIAN_POINT('Ctrl Pts',(3.5782545595439,-1.,-1.62380329464844));
#44005=CARTESIAN_POINT('Ctrl Pts',(3.57257679609806,-1.,-1.61884340915404));
#44006=CARTESIAN_POINT('Ctrl Pts',(3.56689200468387,-1.,-1.61393581747514));
#44007=CARTESIAN_POINT('Ctrl Pts',(3.5612043248298,-1.,-1.60908344685457));
#44008=CARTESIAN_POINT('Ctrl Pts',(3.55550985096129,-1.,-1.60428584699853));
#44009=CARTESIAN_POINT('Ctrl Pts',(3.54979148634454,-1.,-1.59953698113457));
#44010=CARTESIAN_POINT('Ctrl Pts',(3.54402458182337,-1.,-1.59482766949766));
#44011=CARTESIAN_POINT('Ctrl Pts',(3.53818616861077,-1.,-1.59014958368739));
#44012=CARTESIAN_POINT('Ctrl Pts',(3.5322637814708,-1.,-1.58549906268088));
#44013=CARTESIAN_POINT('Ctrl Pts',(3.52626275334881,-1.,-1.58088027227848));
#44014=CARTESIAN_POINT('Ctrl Pts',(3.52021847865912,-1.,-1.57631049988158));
#44015=CARTESIAN_POINT('Ctrl Pts',(3.51418598431665,-1.,-1.57181569799743));
#44016=CARTESIAN_POINT('Ctrl Pts',(3.50821771695363,-1.,-1.56742097575012));
#44017=CARTESIAN_POINT('Ctrl Pts',(3.50234321621578,-1.,-1.56314187758675));
#44018=CARTESIAN_POINT('Ctrl Pts',(3.49655185179655,-1.,-1.55897703097874));
#44019=CARTESIAN_POINT('Ctrl Pts',(3.4907646087742,-1.,-1.55489595901116));
#44020=CARTESIAN_POINT('Ctrl Pts',(3.48485155928567,-1.,-1.55084702970452));
#44021=CARTESIAN_POINT('Ctrl Pts',(3.47868272898751,-1.,-1.54678009290276));
#44022=CARTESIAN_POINT('Ctrl Pts',(3.47217189224653,-1.,-1.54266605398188));
#44023=CARTESIAN_POINT('Ctrl Pts',(3.46531752207153,-1.,-1.53851507915502));
#44024=CARTESIAN_POINT('Ctrl Pts',(3.45825932955032,-1.,-1.53440195378792));
#44025=CARTESIAN_POINT('Ctrl Pts',(3.45127136828305,-1.,-1.53046244461635));
#44026=CARTESIAN_POINT('Ctrl Pts',(3.44469547526647,-1.,-1.52686242875556));
#44027=CARTESIAN_POINT('Ctrl Pts',(3.4388889597401,-1.,-1.5237734895035));
#44028=CARTESIAN_POINT('Ctrl Pts',(3.43417156977893,-1.,-1.52134826724293));
#44029=CARTESIAN_POINT('Ctrl Pts',(3.43101631893414,-1.,-1.5198144909338));
#44030=CARTESIAN_POINT('Ctrl Pts',(3.42946838852587,-1.,-1.51914806898491));
#44031=CARTESIAN_POINT('Ctrl Pts',(3.42884302333841,-1.,-1.5189513329503));
#44032=CARTESIAN_POINT('Ctrl Pts',(3.42864616361875,-1.,-1.51893924967331));
#44033=CARTESIAN_POINT('Ctrl Pts',(3.42859860294305,-1.,-1.5189508286633));
#44034=CARTESIAN_POINT('',(3.49844575334386,-1.,-1.35032489087269));
#44035=CARTESIAN_POINT('Origin',(0.,-1.,0.));
#44036=CARTESIAN_POINT('',(3.97027773754922,-1.,-1.36999806084572));
#44037=CARTESIAN_POINT('Ctrl Pts',(3.49844575334386,-1.,-1.35032489087269));
#44038=CARTESIAN_POINT('Ctrl Pts',(3.49847119623841,-1.,-1.35036670893102));
#44039=CARTESIAN_POINT('Ctrl Pts',(3.49861894124915,-1.,-1.35049736560633));
#44040=CARTESIAN_POINT('Ctrl Pts',(3.49920025459856,-1.,-1.35080045218652));
#44041=CARTESIAN_POINT('Ctrl Pts',(3.5007660381658,-1.,-1.35142377279535));
#44042=CARTESIAN_POINT('Ctrl Pts',(3.50408168106113,-1.,-1.3525703284343));
#44043=CARTESIAN_POINT('Ctrl Pts',(3.50913227060177,-1.,-1.35419113576022));
#44044=CARTESIAN_POINT('Ctrl Pts',(3.51542230699919,-1.,-1.35611275237288));
#44045=CARTESIAN_POINT('Ctrl Pts',(3.52261776117121,-1.,-1.35821701528975));
#44046=CARTESIAN_POINT('Ctrl Pts',(3.53034464961849,-1.,-1.36037259643827));
#44047=CARTESIAN_POINT('Ctrl Pts',(3.53824396425032,-1.,-1.36245507339334));
#44048=CARTESIAN_POINT('Ctrl Pts',(3.54602591832893,-1.,-1.36436666257568));
#44049=CARTESIAN_POINT('Ctrl Pts',(3.55353883995793,-1.,-1.36606145456711));
#44050=CARTESIAN_POINT('Ctrl Pts',(3.56077662028492,-1.,-1.36754771771174));
#44051=CARTESIAN_POINT('Ctrl Pts',(3.56782080304554,-1.,-1.36886584973349));
#44052=CARTESIAN_POINT('Ctrl Pts',(3.57479875549453,-1.,-1.37007229485646));
#44053=CARTESIAN_POINT('Ctrl Pts',(3.58183885982745,-1.,-1.37122241663073));
#44054=CARTESIAN_POINT('Ctrl Pts',(3.5890185384643,-1.,-1.37235053661));
#44055=CARTESIAN_POINT('Ctrl Pts',(3.59634627869117,-1.,-1.37346320103184));
#44056=CARTESIAN_POINT('Ctrl Pts',(3.60379020124038,-1.,-1.37455051379642));
#44057=CARTESIAN_POINT('Ctrl Pts',(3.61129546591082,-1.,-1.37559314436641));
#44058=CARTESIAN_POINT('Ctrl Pts',(3.61880481160408,-1.,-1.37657053403102));
#44059=CARTESIAN_POINT('Ctrl Pts',(3.62628098665112,-1.,-1.37746987919868));
#44060=CARTESIAN_POINT('Ctrl Pts',(3.63371727442448,-1.,-1.37829035457325));
#44061=CARTESIAN_POINT('Ctrl Pts',(3.64112507791112,-1.,-1.37903818567347));
#44062=CARTESIAN_POINT('Ctrl Pts',(3.64852652756444,-1.,-1.37972372481598));
#44063=CARTESIAN_POINT('Ctrl Pts',(3.65594554404396,-1.,-1.38035791051215));
#44064=CARTESIAN_POINT('Ctrl Pts',(3.66339848520874,-1.,-1.38094856333558));
#44065=CARTESIAN_POINT('Ctrl Pts',(3.67088843112282,-1.,-1.38149812653876));
#44066=CARTESIAN_POINT('Ctrl Pts',(3.6784103848243,-1.,-1.38200574290626));
#44067=CARTESIAN_POINT('Ctrl Pts',(3.68595444983844,-1.,-1.38246852827185));
#44068=CARTESIAN_POINT('Ctrl Pts',(3.69350967899523,-1.,-1.38288311171649));
#44069=CARTESIAN_POINT('Ctrl Pts',(3.70106792167894,-1.,-1.38324717612862));
#44070=CARTESIAN_POINT('Ctrl Pts',(3.70862680753343,-1.,-1.38356065402122));
#44071=CARTESIAN_POINT('Ctrl Pts',(3.7161876605181,-1.,-1.38382489984585));
#44072=CARTESIAN_POINT('Ctrl Pts',(3.72375409358805,-1.,-1.3840421342895));
#44073=CARTESIAN_POINT('Ctrl Pts',(3.73133035859283,-1.,-1.38421479111531));
#44074=CARTESIAN_POINT('Ctrl Pts',(3.73891976418099,-1.,-1.38434489156456));
#44075=CARTESIAN_POINT('Ctrl Pts',(3.7465231716786,-1.,-1.38443344984389));
#44076=CARTESIAN_POINT('Ctrl Pts',(3.75413976318727,-1.,-1.38448077997155));
#44077=CARTESIAN_POINT('Ctrl Pts',(3.76176768271347,-1.,-1.38448675253343));
#44078=CARTESIAN_POINT('Ctrl Pts',(3.76940473185775,-1.,-1.38445107339517));
#44079=CARTESIAN_POINT('Ctrl Pts',(3.77704902230441,-1.,-1.38437354551435));
#44080=CARTESIAN_POINT('Ctrl Pts',(3.78469969805134,-1.,-1.38425435883773));
#44081=CARTESIAN_POINT('Ctrl Pts',(3.79235669640907,-1.,-1.38409399694589));
#44082=CARTESIAN_POINT('Ctrl Pts',(3.80002044322169,-1.,-1.38389311766701));
#44083=CARTESIAN_POINT('Ctrl Pts',(3.80769156398429,-1.,-1.38365244046226));
#44084=CARTESIAN_POINT('Ctrl Pts',(3.81537060817765,-1.,-1.38337263902766));
#44085=CARTESIAN_POINT('Ctrl Pts',(3.82305771743715,-1.,-1.38305421262724));
#44086=CARTESIAN_POINT('Ctrl Pts',(3.83075266982138,-1.,-1.38269750245086));
#44087=CARTESIAN_POINT('Ctrl Pts',(3.83845502790609,-1.,-1.38230274828774));
#44088=CARTESIAN_POINT('Ctrl Pts',(3.84616425605705,-1.,-1.38187013346089));
#44089=CARTESIAN_POINT('Ctrl Pts',(3.85387983979557,-1.,-1.38139983115075));
#44090=CARTESIAN_POINT('Ctrl Pts',(3.86160143044187,-1.,-1.38089205993068));
#44091=CARTESIAN_POINT('Ctrl Pts',(3.86932885813403,-1.,-1.38034709213129));
#44092=CARTESIAN_POINT('Ctrl Pts',(3.87706205830865,-1.,-1.37976523097187));
#44093=CARTESIAN_POINT('Ctrl Pts',(3.88480102249461,-1.,-1.37914679719446));
#44094=CARTESIAN_POINT('Ctrl Pts',(3.89254574338385,-1.,-1.37849211287981));
#44095=CARTESIAN_POINT('Ctrl Pts',(3.90029615196255,-1.,-1.3778014851263));
#44096=CARTESIAN_POINT('Ctrl Pts',(3.90805209522729,-1.,-1.3770751963376));
#44097=CARTESIAN_POINT('Ctrl Pts',(3.91581337461825,-1.,-1.37631350505516));
#44098=CARTESIAN_POINT('Ctrl Pts',(3.92357976987132,-1.,-1.37551664448057));
#44099=CARTESIAN_POINT('Ctrl Pts',(3.93135106761941,-1.,-1.37468482215784));
#44100=CARTESIAN_POINT('Ctrl Pts',(3.93912709041791,-1.,-1.37381821967499));
#44101=CARTESIAN_POINT('Ctrl Pts',(3.94690771786926,-1.,-1.37291699203423));
#44102=CARTESIAN_POINT('Ctrl Pts',(3.95469287283105,-1.,-1.37198126433139));
#44103=CARTESIAN_POINT('Ctrl Pts',(3.96092458508407,-1.,-1.37120515615663));
#44104=CARTESIAN_POINT('Ctrl Pts',(3.96560037975788,-1.,-1.37060761746027));
#44105=CARTESIAN_POINT('Ctrl Pts',(3.9687184694173,-1.,-1.37020239094758));
#44106=CARTESIAN_POINT('Ctrl Pts',(3.97027773754922,-1.,-1.36999806084572));
#44107=CARTESIAN_POINT('',(4.01728681790024,-1.,-1.22531898815164));
#44108=CARTESIAN_POINT('',(3.97027773754922,-1.,-1.36999806084572));
#44109=CARTESIAN_POINT('',(3.62400312501199,-1.,-0.963899035118986));
#44110=CARTESIAN_POINT('Ctrl Pts',(4.01728681790024,-1.,-1.22531898815164));
#44111=CARTESIAN_POINT('Ctrl Pts',(4.01614544569895,-1.,-1.22423716681317));
#44112=CARTESIAN_POINT('Ctrl Pts',(4.01386104433519,-1.,-1.22207656455845));
#44113=CARTESIAN_POINT('Ctrl Pts',(4.01042947140789,-1.,-1.21884478244403));
#44114=CARTESIAN_POINT('Ctrl Pts',(4.00584409522722,-1.,-1.21455398918133));
#44115=CARTESIAN_POINT('Ctrl Pts',(4.00009577950721,-1.,-1.20922097029551));
#44116=CARTESIAN_POINT('Ctrl Pts',(3.99433084799666,-1.,-1.20391852375139));
#44117=CARTESIAN_POINT('Ctrl Pts',(3.98854928957189,-1.,-1.19864679609566));
#44118=CARTESIAN_POINT('Ctrl Pts',(3.98275111052561,-1.,-1.19340598349475));
#44119=CARTESIAN_POINT('Ctrl Pts',(3.97693634767754,-1.,-1.18819633715539));
#44120=CARTESIAN_POINT('Ctrl Pts',(3.97110505165415,-1.,-1.18301815039831));
#44121=CARTESIAN_POINT('Ctrl Pts',(3.96525726358159,-1.,-1.17787174135592));
#44122=CARTESIAN_POINT('Ctrl Pts',(3.95939299213276,-1.,-1.17275743590361));
#44123=CARTESIAN_POINT('Ctrl Pts',(3.95351219509876,-1.,-1.16767555244438));
#44124=CARTESIAN_POINT('Ctrl Pts',(3.94761474780583,-1.,-1.16262637999157));
#44125=CARTESIAN_POINT('Ctrl Pts',(3.94170046685203,-1.,-1.15761018340956));
#44126=CARTESIAN_POINT('Ctrl Pts',(3.9357691705628,-1.,-1.1526272271632));
#44127=CARTESIAN_POINT('Ctrl Pts',(3.92982073294257,-1.,-1.14767779451124));
#44128=CARTESIAN_POINT('Ctrl Pts',(3.92385513133997,-1.,-1.14276220561593));
#44129=CARTESIAN_POINT('Ctrl Pts',(3.91787251936827,-1.,-1.13788084225554));
#44130=CARTESIAN_POINT('Ctrl Pts',(3.91187321145649,-1.,-1.13303414693896));
#44131=CARTESIAN_POINT('Ctrl Pts',(3.90585753318737,-1.,-1.12822258281553));
#44132=CARTESIAN_POINT('Ctrl Pts',(3.89982569750025,-1.,-1.12344660099043));
#44133=CARTESIAN_POINT('Ctrl Pts',(3.89377768340344,-1.,-1.11870660794603));
#44134=CARTESIAN_POINT('Ctrl Pts',(3.88771308285171,-1.,-1.11400292434429));
#44135=CARTESIAN_POINT('Ctrl Pts',(3.88163105531724,-1.,-1.10933577224008));
#44136=CARTESIAN_POINT('Ctrl Pts',(3.87553067187514,-1.,-1.10470536603287));
#44137=CARTESIAN_POINT('Ctrl Pts',(3.86941120134849,-1.,-1.10011198761195));
#44138=CARTESIAN_POINT('Ctrl Pts',(3.86327241021247,-1.,-1.09555606505013));
#44139=CARTESIAN_POINT('Ctrl Pts',(3.85711487933931,-1.,-1.09103825516294));
#44140=CARTESIAN_POINT('Ctrl Pts',(3.85094025222713,-1.,-1.08655950846384));
#44141=CARTESIAN_POINT('Ctrl Pts',(3.8447504803063,-1.,-1.08212087917991));
#44142=CARTESIAN_POINT('Ctrl Pts',(3.83854714117491,-1.,-1.07772335353858));
#44143=CARTESIAN_POINT('Ctrl Pts',(3.83233071195144,-1.,-1.07336766633459));
#44144=CARTESIAN_POINT('Ctrl Pts',(3.82609989967276,-1.,-1.06905413180359));
#44145=CARTESIAN_POINT('Ctrl Pts',(3.81985083953012,-1.,-1.0647824403893));
#44146=CARTESIAN_POINT('Ctrl Pts',(3.8135786611749,-1.,-1.06055206187299));
#44147=CARTESIAN_POINT('Ctrl Pts',(3.80727913637791,-1.,-1.05636266918644));
#44148=CARTESIAN_POINT('Ctrl Pts',(3.80095039790681,-1.,-1.05221457990016));
#44149=CARTESIAN_POINT('Ctrl Pts',(3.79459440308786,-1.,-1.04810913267639));
#44150=CARTESIAN_POINT('Ctrl Pts',(3.78821910787179,-1.,-1.04404924374422));
#44151=CARTESIAN_POINT('Ctrl Pts',(3.7818353500817,-1.,-1.04003862055798));
#44152=CARTESIAN_POINT('Ctrl Pts',(3.77545283140427,-1.,-1.03608074678008));
#44153=CARTESIAN_POINT('Ctrl Pts',(3.76907609832516,-1.,-1.03217786604919));
#44154=CARTESIAN_POINT('Ctrl Pts',(3.76270122291245,-1.,-1.02833014458184));
#44155=CARTESIAN_POINT('Ctrl Pts',(3.75631037456224,-1.,-1.02453429444668));
#44156=CARTESIAN_POINT('Ctrl Pts',(3.74987777155873,-1.,-1.02078510487439));
#44157=CARTESIAN_POINT('Ctrl Pts',(3.74337942504993,-1.,-1.01707794311088));
#44158=CARTESIAN_POINT('Ctrl Pts',(3.73680245055747,-1.,-1.01341114319906));
#44159=CARTESIAN_POINT('Ctrl Pts',(3.73015276704407,-1.,-1.00978798539491));
#44160=CARTESIAN_POINT('Ctrl Pts',(3.72346803750544,-1.,-1.00622000735696));
#44161=CARTESIAN_POINT('Ctrl Pts',(3.71680667125047,-1.,-1.00272423396802));
#44162=CARTESIAN_POINT('Ctrl Pts',(3.7102243971387,-1.,-0.999317260756345));
#44163=CARTESIAN_POINT('Ctrl Pts',(3.70375282282107,-1.,-0.996009819772432));
#44164=CARTESIAN_POINT('Ctrl Pts',(3.69738123415696,-1.,-0.992802218332104));
#44165=CARTESIAN_POINT('Ctrl Pts',(3.69102682138955,-1.,-0.989676715398859));
#44166=CARTESIAN_POINT('Ctrl Pts',(3.6845531792623,-1.,-0.986602639864286));
#44167=CARTESIAN_POINT('Ctrl Pts',(3.67782408841876,-1.,-0.983550791470865));
#44168=CARTESIAN_POINT('Ctrl Pts',(3.67074983340444,-1.,-0.980505922458495));
#44169=CARTESIAN_POINT('Ctrl Pts',(3.66333049637403,-1.,-0.977478312751416));
#44170=CARTESIAN_POINT('Ctrl Pts',(3.6557157673487,-1.,-0.974519971354139));
#44171=CARTESIAN_POINT('Ctrl Pts',(3.64819756447072,-1.,-0.971722122060278));
#44172=CARTESIAN_POINT('Ctrl Pts',(3.64113946505393,-1.,-0.969195124674829));
#44173=CARTESIAN_POINT('Ctrl Pts',(3.6349212208096,-1.,-0.967052554540878));
#44174=CARTESIAN_POINT('Ctrl Pts',(3.62988252139998,-1.,-0.965395153165716));
#44175=CARTESIAN_POINT('Ctrl Pts',(3.62652618145252,-1.,-0.964373850166081));
#44176=CARTESIAN_POINT('Ctrl Pts',(3.62489305727516,-1.,-0.963957782642589));
#44177=CARTESIAN_POINT('Ctrl Pts',(3.62424461507455,-1.,-0.963861297423579));
#44178=CARTESIAN_POINT('Ctrl Pts',(3.62404828878374,-1.,-0.963880158556713));
#44179=CARTESIAN_POINT('Ctrl Pts',(3.62400312501199,-1.,-0.963899035118986));
#44180=CARTESIAN_POINT('',(3.66661143271648,-1.,-0.786422660833743));
#44181=CARTESIAN_POINT('Origin',(0.,-1.,0.));
#44182=CARTESIAN_POINT('',(4.13571194405636,-1.,-0.73204283740062));
#44183=CARTESIAN_POINT('Ctrl Pts',(3.66661143271648,-1.,-0.786422660833743));
#44184=CARTESIAN_POINT('Ctrl Pts',(3.66664310415236,-1.,-0.786459983896781));
#44185=CARTESIAN_POINT('Ctrl Pts',(3.66680946938396,-1.,-0.78656591955989));
#44186=CARTESIAN_POINT('Ctrl Pts',(3.66743103898844,-1.,-0.7867743371985));
#44187=CARTESIAN_POINT('Ctrl Pts',(3.66907505398769,-1.,-0.787145041181589));
#44188=CARTESIAN_POINT('Ctrl Pts',(3.672529236635,-1.,-0.787758799995427));
#44189=CARTESIAN_POINT('Ctrl Pts',(3.67777119516438,-1.,-0.788569566220663));
#44190=CARTESIAN_POINT('Ctrl Pts',(3.68428439784285,-1.,-0.789483546065159));
#44191=CARTESIAN_POINT('Ctrl Pts',(3.69172044327754,-1.,-0.79043628498958));
#44192=CARTESIAN_POINT('Ctrl Pts',(3.69968940808982,-1.,-0.791356575696509));
#44193=CARTESIAN_POINT('Ctrl Pts',(3.70781724021879,-1.,-0.792177688845968));
#44194=CARTESIAN_POINT('Ctrl Pts',(3.7158024239604,-1.,-0.792848377370116));
#44195=CARTESIAN_POINT('Ctrl Pts',(3.7234879729357,-1.,-0.793347023783871));
#44196=CARTESIAN_POINT('Ctrl Pts',(3.7308691469564,-1.,-0.793682750269348));
#44197=CARTESIAN_POINT('Ctrl Pts',(3.73803280541576,-1.,-0.793882700936791));
#44198=CARTESIAN_POINT('Ctrl Pts',(3.74511357728827,-1.,-0.79398270045988));
#44199=CARTESIAN_POINT('Ctrl Pts',(3.75224692493895,-1.,-0.794017347371441));
#44200=CARTESIAN_POINT('Ctrl Pts',(3.75951468666325,-1.,-0.794008429135047));
#44201=CARTESIAN_POINT('Ctrl Pts',(3.76692626931184,-1.,-0.793961083689141));
#44202=CARTESIAN_POINT('Ctrl Pts',(3.77444863801264,-1.,-0.793870523787515));
#44203=CARTESIAN_POINT('Ctrl Pts',(3.78202460377617,-1.,-0.79372623578134));
#44204=CARTESIAN_POINT('Ctrl Pts',(3.78959439439222,-1.,-0.793516871680966));
#44205=CARTESIAN_POINT('Ctrl Pts',(3.79711921389862,-1.,-0.793235612973201));
#44206=CARTESIAN_POINT('Ctrl Pts',(3.80459229925598,-1.,-0.792882695234693));
#44207=CARTESIAN_POINT('Ctrl Pts',(3.81202588694726,-1.,-0.792462483517568));
#44208=CARTESIAN_POINT('Ctrl Pts',(3.81944345442237,-1.,-0.791981740718607));
#44209=CARTESIAN_POINT('Ctrl Pts',(3.82687033899799,-1.,-0.791447528662381));
#44210=CARTESIAN_POINT('Ctrl Pts',(3.83432392054804,-1.,-0.79086501270534));
#44211=CARTESIAN_POINT('Ctrl Pts',(3.84180762342476,-1.,-0.790236124191289));
#44212=CARTESIAN_POINT('Ctrl Pts',(3.8493163780891,-1.,-0.789560798155619));
#44213=CARTESIAN_POINT('Ctrl Pts',(3.85683995872536,-1.,-0.788837734090688));
#44214=CARTESIAN_POINT('Ctrl Pts',(3.86436702561342,-1.,-0.788065315093771));
#44215=CARTESIAN_POINT('Ctrl Pts',(3.87188916600905,-1.,-0.787242527617981));
#44216=CARTESIAN_POINT('Ctrl Pts',(3.87940402818186,-1.,-0.786369675812592));
#44217=CARTESIAN_POINT('Ctrl Pts',(3.88691313167399,-1.,-0.785447890340723));
#44218=CARTESIAN_POINT('Ctrl Pts',(3.89442039235105,-1.,-0.784478799358336));
#44219=CARTESIAN_POINT('Ctrl Pts',(3.90193039043971,-1.,-0.783464141529083));
#44220=CARTESIAN_POINT('Ctrl Pts',(3.90944671004536,-1.,-0.782405395622759));
#44221=CARTESIAN_POINT('Ctrl Pts',(3.9169703605466,-1.,-0.781303428618344));
#44222=CARTESIAN_POINT('Ctrl Pts',(3.92450058323799,-1.,-0.780158678615507));
#44223=CARTESIAN_POINT('Ctrl Pts',(3.93203552473153,-1.,-0.778971308134786));
#44224=CARTESIAN_POINT('Ctrl Pts',(3.93957296768098,-1.,-0.77774137056855));
#44225=CARTESIAN_POINT('Ctrl Pts',(3.94711101619471,-1.,-0.77646896669796));
#44226=CARTESIAN_POINT('Ctrl Pts',(3.95464885452364,-1.,-0.775154418039442));
#44227=CARTESIAN_POINT('Ctrl Pts',(3.96218649639876,-1.,-0.773798212026683));
#44228=CARTESIAN_POINT('Ctrl Pts',(3.96972446532832,-1.,-0.772400931772239));
#44229=CARTESIAN_POINT('Ctrl Pts',(3.97726349165507,-1.,-0.770963190030504));
#44230=CARTESIAN_POINT('Ctrl Pts',(3.98480422348403,-1.,-0.76948556624546));
#44231=CARTESIAN_POINT('Ctrl Pts',(3.99234687880892,-1.,-0.767968531377708));
#44232=CARTESIAN_POINT('Ctrl Pts',(3.99989129179464,-1.,-0.766412457135786));
#44233=CARTESIAN_POINT('Ctrl Pts',(4.00743706791366,-1.,-0.764817648784947));
#44234=CARTESIAN_POINT('Ctrl Pts',(4.01498370680434,-1.,-0.763184371182827));
#44235=CARTESIAN_POINT('Ctrl Pts',(4.02253072741347,-1.,-0.761512875859942));
#44236=CARTESIAN_POINT('Ctrl Pts',(4.0300778195465,-1.,-0.759803433244166));
#44237=CARTESIAN_POINT('Ctrl Pts',(4.03762485803468,-1.,-0.758056338885554));
#44238=CARTESIAN_POINT('Ctrl Pts',(4.04517182654344,-1.,-0.756271902370187));
#44239=CARTESIAN_POINT('Ctrl Pts',(4.05271876688106,-1.,-0.754450441816412));
#44240=CARTESIAN_POINT('Ctrl Pts',(4.06026572221399,-1.,-0.752592276482869));
#44241=CARTESIAN_POINT('Ctrl Pts',(4.06781267241886,-1.,-0.750697720483176));
#44242=CARTESIAN_POINT('Ctrl Pts',(4.07535951055363,-1.,-0.748767076679177));
#44243=CARTESIAN_POINT('Ctrl Pts',(4.08290608094789,-1.,-0.746800631490822));
#44244=CARTESIAN_POINT('Ctrl Pts',(4.09045220253011,-1.,-0.744798649705514));
#44245=CARTESIAN_POINT('Ctrl Pts',(4.09799769702712,-1.,-0.742761369690018));
#44246=CARTESIAN_POINT('Ctrl Pts',(4.1055424175856,-1.,-0.740688998555152));
#44247=CARTESIAN_POINT('Ctrl Pts',(4.11308626953795,-1.,-0.738581708229119));
#44248=CARTESIAN_POINT('Ctrl Pts',(4.12062919626082,-1.,-0.736439634335347));
#44249=CARTESIAN_POINT('Ctrl Pts',(4.12666277572794,-1.,-0.734698226767513));
#44250=CARTESIAN_POINT('Ctrl Pts',(4.13118752796397,-1.,-0.733376589325634));
#44251=CARTESIAN_POINT('Ctrl Pts',(4.13420383737278,-1.,-0.732488575135926));
#44252=CARTESIAN_POINT('Ctrl Pts',(4.13571194405636,-1.,-0.73204283740062));
#44253=CARTESIAN_POINT('',(4.15950947128175,-1.,-0.581791163835815));
#44254=CARTESIAN_POINT('',(4.13571194405636,-1.,-0.73204283740062));
#44255=CARTESIAN_POINT('',(3.73017266276632,-1.,-0.385112848332549));
#44256=CARTESIAN_POINT('Ctrl Pts',(4.15950947128175,-1.,-0.581791163835815));
#44257=CARTESIAN_POINT('Ctrl Pts',(4.15821291712391,-1.,-0.580901211462913));
#44258=CARTESIAN_POINT('Ctrl Pts',(4.15561864787379,-1.,-0.579124568912544));
#44259=CARTESIAN_POINT('Ctrl Pts',(4.1517237611974,-1.,-0.576469391673917));
#44260=CARTESIAN_POINT('Ctrl Pts',(4.14652361065787,-1.,-0.572948736066277));
#44261=CARTESIAN_POINT('Ctrl Pts',(4.14001179828669,-1.,-0.568580610187116));
#44262=CARTESIAN_POINT('Ctrl Pts',(4.13348835726086,-1.,-0.564245279535706));
#44263=CARTESIAN_POINT('Ctrl Pts',(4.12695329951859,-1.,-0.559942890594628));
#44264=CARTESIAN_POINT('Ctrl Pts',(4.1204066619623,-1.,-0.555673636130778));
#44265=CARTESIAN_POINT('Ctrl Pts',(4.11384852025578,-1.,-0.551437758498247));
#44266=CARTESIAN_POINT('Ctrl Pts',(4.1072789702877,-1.,-0.54723553948676));
#44267=CARTESIAN_POINT('Ctrl Pts',(4.10069810244473,-1.,-0.543067286878457));
#44268=CARTESIAN_POINT('Ctrl Pts',(4.09410597627116,-1.,-0.538933321179921));
#44269=CARTESIAN_POINT('Ctrl Pts',(4.08750259988693,-1.,-0.534833963477));
#44270=CARTESIAN_POINT('Ctrl Pts',(4.08088789536488,-1.,-0.530769518728076));
#44271=CARTESIAN_POINT('Ctrl Pts',(4.07426172299496,-1.,-0.526740277227));
#44272=CARTESIAN_POINT('Ctrl Pts',(4.06762394471075,-1.,-0.522746528602768));
#44273=CARTESIAN_POINT('Ctrl Pts',(4.06097448037934,-1.,-0.51878857233681));
#44274=CARTESIAN_POINT('Ctrl Pts',(4.05431335771261,-1.,-0.514866728193104));
#44275=CARTESIAN_POINT('Ctrl Pts',(4.04764078815591,-1.,-0.510981349219174));
#44276=CARTESIAN_POINT('Ctrl Pts',(4.04095715149074,-1.,-0.507132823288362));
#44277=CARTESIAN_POINT('Ctrl Pts',(4.0342628417439,-1.,-0.503321556915514));
#44278=CARTESIAN_POINT('Ctrl Pts',(4.0275581398015,-1.,-0.49954796234089));
#44279=CARTESIAN_POINT('Ctrl Pts',(4.02084308851813,-1.,-0.495812444326223));
#44280=CARTESIAN_POINT('Ctrl Pts',(4.01411733503486,-1.,-0.492115383417931));
#44281=CARTESIAN_POINT('Ctrl Pts',(4.0073800839092,-1.,-0.488457130424531));
#44282=CARTESIAN_POINT('Ctrl Pts',(4.00063045119234,-1.,-0.484838042421754));
#44283=CARTESIAN_POINT('Ctrl Pts',(3.99386775880655,-1.,-0.481258512209638));
#44284=CARTESIAN_POINT('Ctrl Pts',(3.98709184306743,-1.,-0.477718999122033));
#44285=CARTESIAN_POINT('Ctrl Pts',(3.9803033804443,-1.,-0.474220061019542));
#44286=CARTESIAN_POINT('Ctrl Pts',(3.97350414289415,-1.,-0.470762379613478));
#44287=CARTESIAN_POINT('Ctrl Pts',(3.96669622273946,-1.,-0.467346690880672));
#44288=CARTESIAN_POINT('Ctrl Pts',(3.95988133243543,-1.,-0.463973722115745));
#44289=CARTESIAN_POINT('Ctrl Pts',(3.95306005817363,-1.,-0.460644124429119));
#44290=CARTESIAN_POINT('Ctrl Pts',(3.94623117206675,-1.,-0.457358410451674));
#44291=CARTESIAN_POINT('Ctrl Pts',(3.93939080846298,-1.,-0.454116879027576));
#44292=CARTESIAN_POINT('Ctrl Pts',(3.93253407403128,-1.,-0.450919768356347));
#44293=CARTESIAN_POINT('Ctrl Pts',(3.92565674143424,-1.,-0.447767416837297));
#44294=CARTESIAN_POINT('Ctrl Pts',(3.91875701610721,-1.,-0.444660430230593));
#44295=CARTESIAN_POINT('Ctrl Pts',(3.91183704069146,-1.,-0.441599824524048));
#44296=CARTESIAN_POINT('Ctrl Pts',(3.90490512938546,-1.,-0.438587235458234));
#44297=CARTESIAN_POINT('Ctrl Pts',(3.8979725665544,-1.,-0.435624629433506));
#44298=CARTESIAN_POINT('Ctrl Pts',(3.89104947940592,-1.,-0.43271392954444));
#44299=CARTESIAN_POINT('Ctrl Pts',(3.88414070943334,-1.,-0.429856640579734));
#44300=CARTESIAN_POINT('Ctrl Pts',(3.87724240306609,-1.,-0.427053541173469));
#44301=CARTESIAN_POINT('Ctrl Pts',(3.87033643487882,-1.,-0.424304173195143));
#44302=CARTESIAN_POINT('Ctrl Pts',(3.86339652542749,-1.,-0.421607423177576));
#44303=CARTESIAN_POINT('Ctrl Pts',(3.85639825648031,-1.,-0.41896246808681));
#44304=CARTESIAN_POINT('Ctrl Pts',(3.8493286415751,-1.,-0.41636967805292));
#44305=CARTESIAN_POINT('Ctrl Pts',(3.84219403994742,-1.,-0.413831367016727));
#44306=CARTESIAN_POINT('Ctrl Pts',(3.83503345578645,-1.,-0.41135303879846));
#44307=CARTESIAN_POINT('Ctrl Pts',(3.82790724256397,-1.,-0.408942371447377));
#44308=CARTESIAN_POINT('Ctrl Pts',(3.82087303913741,-1.,-0.406607038258907));
#44309=CARTESIAN_POINT('Ctrl Pts',(3.81396374287762,-1.,-0.404352694628237));
#44310=CARTESIAN_POINT('Ctrl Pts',(3.80716881962763,-1.,-0.402181320148475));
#44311=CARTESIAN_POINT('Ctrl Pts',(3.80040370384659,-1.,-0.400088346504727));
#44312=CARTESIAN_POINT('Ctrl Pts',(3.79352887163457,-1.,-0.398064818684159));
#44313=CARTESIAN_POINT('Ctrl Pts',(3.78640521279479,-1.,-0.396103205335029));
#44314=CARTESIAN_POINT('Ctrl Pts',(3.77894173114368,-1.,-0.394202481011595));
#44315=CARTESIAN_POINT('Ctrl Pts',(3.77114011595892,-1.,-0.392372786223347));
#44316=CARTESIAN_POINT('Ctrl Pts',(3.76315635032993,-1.,-0.390642072979259));
#44317=CARTESIAN_POINT('Ctrl Pts',(3.75529302894757,-1.,-0.389054775898251));
#44318=CARTESIAN_POINT('Ctrl Pts',(3.74792651696269,-1.,-0.387663020050396));
#44319=CARTESIAN_POINT('Ctrl Pts',(3.74144965781088,-1.,-0.386519576222036));
#44320=CARTESIAN_POINT('Ctrl Pts',(3.73621371845475,-1.,-0.385670806454744));
#44321=CARTESIAN_POINT('Ctrl Pts',(3.73273893363318,-1.,-0.385187124633965));
#44322=CARTESIAN_POINT('Ctrl Pts',(3.73106082862399,-1.,-0.385031656499142));
#44323=CARTESIAN_POINT('Ctrl Pts',(3.73040527620929,-1.,-0.385037797882046));
#44324=CARTESIAN_POINT('Ctrl Pts',(3.73021431755218,-1.,-0.385087139001609));
#44325=CARTESIAN_POINT('Ctrl Pts',(3.73017266276632,-1.,-0.385112848332549));
#44326=CARTESIAN_POINT('',(3.74449296982994,-1.,-0.203156094897896));
#44327=CARTESIAN_POINT('Origin',(0.,-1.,0.));
#44328=CARTESIAN_POINT('',(4.19931119685982,-1.,-0.0760622897878241));
#44329=CARTESIAN_POINT('Ctrl Pts',(3.74449296982994,-1.,-0.203156094897896));
#44330=CARTESIAN_POINT('Ctrl Pts',(3.74453008995129,-1.,-0.203188003947965));
#44331=CARTESIAN_POINT('Ctrl Pts',(3.74471097893961,-1.,-0.203266610111264));
#44332=CARTESIAN_POINT('Ctrl Pts',(3.74535749969262,-1.,-0.203375226874332));
#44333=CARTESIAN_POINT('Ctrl Pts',(3.74703926501843,-1.,-0.203484186269315));
#44334=CARTESIAN_POINT('Ctrl Pts',(3.75054693397716,-1.,-0.203550035479097));
#44335=CARTESIAN_POINT('Ctrl Pts',(3.75585118707924,-1.,-0.203530796848404));
#44336=CARTESIAN_POINT('Ctrl Pts',(3.76242717937273,-1.,-0.203414634707647));
#44337=CARTESIAN_POINT('Ctrl Pts',(3.76992071595267,-1.,-0.203192390045338));
#44338=CARTESIAN_POINT('Ctrl Pts',(3.77793553476879,-1.,-0.202854729699197));
#44339=CARTESIAN_POINT('Ctrl Pts',(3.78609175019317,-1.,-0.202394260512193));
#44340=CARTESIAN_POINT('Ctrl Pts',(3.79408354187274,-1.,-0.201807533800799));
#44341=CARTESIAN_POINT('Ctrl Pts',(3.80175247447171,-1.,-0.201097756307252));
#44342=CARTESIAN_POINT('Ctrl Pts',(3.80909529318501,-1.,-0.20027467943329));
#44343=CARTESIAN_POINT('Ctrl Pts',(3.81620203429702,-1.,-0.199351525297397));
#44344=CARTESIAN_POINT('Ctrl Pts',(3.82321127348981,-1.,-0.19834261690047));
#44345=CARTESIAN_POINT('Ctrl Pts',(3.83026221776488,-1.,-0.197260935827375));
#44346=CARTESIAN_POINT('Ctrl Pts',(3.83743910616265,-1.,-0.19611519897189));
#44347=CARTESIAN_POINT('Ctrl Pts',(3.84475203347052,-1.,-0.194909009460255));
#44348=CARTESIAN_POINT('Ctrl Pts',(3.85216762264019,-1.,-0.193642806777748));
#44349=CARTESIAN_POINT('Ctrl Pts',(3.85962774407652,-1.,-0.19231515304498));
#44350=CARTESIAN_POINT('Ctrl Pts',(3.8670715862477,-1.,-0.190924190418613));
#44351=CARTESIAN_POINT('Ctrl Pts',(3.87445976418377,-1.,-0.189469253358255));
#44352=CARTESIAN_POINT('Ctrl Pts',(3.88178563496187,-1.,-0.187951632512664));
#44353=CARTESIAN_POINT('Ctrl Pts',(3.88906196725817,-1.,-0.186373724985263));
#44354=CARTESIAN_POINT('Ctrl Pts',(3.89631300742633,-1.,-0.184738537728035));
#44355=CARTESIAN_POINT('Ctrl Pts',(3.90356488555138,-1.,-0.183049081993193));
#44356=CARTESIAN_POINT('Ctrl Pts',(3.91083557557193,-1.,-0.181307740731796));
#44357=CARTESIAN_POINT('Ctrl Pts',(3.91812876180948,-1.,-0.179515885822895));
#44358=CARTESIAN_POINT('Ctrl Pts',(3.92543942697672,-1.,-0.177674246152328));
#44359=CARTESIAN_POINT('Ctrl Pts',(3.93275726771049,-1.,-0.175783136893873));
#44360=CARTESIAN_POINT('Ctrl Pts',(3.94007083096214,-1.,-0.173842734974608));
#44361=CARTESIAN_POINT('Ctrl Pts',(3.94737164900861,-1.,-0.171853355369233));
#44362=CARTESIAN_POINT('Ctrl Pts',(3.95465744665263,-1.,-0.16981566637413));
#44363=CARTESIAN_POINT('Ctrl Pts',(3.96192990160296,-1.,-0.167730547023312));
#44364=CARTESIAN_POINT('Ctrl Pts',(3.9691931362141,-1.,-0.165598992851098));
#44365=CARTESIAN_POINT('Ctrl Pts',(3.97645194630944,-1.,-0.163422004609999));
#44366=CARTESIAN_POINT('Ctrl Pts',(3.98371010319866,-1.,-0.161200482186088));
#44367=CARTESIAN_POINT('Ctrl Pts',(3.99096873945862,-1.,-0.158935123982796));
#44368=CARTESIAN_POINT('Ctrl Pts',(3.99822717425869,-1.,-0.156626481393736));
#44369=CARTESIAN_POINT('Ctrl Pts',(4.00548360245297,-1.,-0.15427500487231));
#44370=CARTESIAN_POINT('Ctrl Pts',(4.01273584234684,-1.,-0.151881094022909));
#44371=CARTESIAN_POINT('Ctrl Pts',(4.01998203715588,-1.,-0.149445144968708));
#44372=CARTESIAN_POINT('Ctrl Pts',(4.02722143147048,-1.,-0.146967602878999));
#44373=CARTESIAN_POINT('Ctrl Pts',(4.03445411510403,-1.,-0.144448947038352));
#44374=CARTESIAN_POINT('Ctrl Pts',(4.04168069633842,-1.,-0.141889671485508));
#44375=CARTESIAN_POINT('Ctrl Pts',(4.04890199238056,-1.,-0.13929026718006));
#44376=CARTESIAN_POINT('Ctrl Pts',(4.05611873400122,-1.,-0.136651205046111));
#44377=CARTESIAN_POINT('Ctrl Pts',(4.06333121018476,-1.,-0.133972916144225));
#44378=CARTESIAN_POINT('Ctrl Pts',(4.07053931528579,-1.,-0.131255793548914));
#44379=CARTESIAN_POINT('Ctrl Pts',(4.07774270738809,-1.,-0.128500200484814));
#44380=CARTESIAN_POINT('Ctrl Pts',(4.08494093372315,-1.,-0.12570647682253));
#44381=CARTESIAN_POINT('Ctrl Pts',(4.09213355850836,-1.,-0.122874946249119));
#44382=CARTESIAN_POINT('Ctrl Pts',(4.09932031767243,-1.,-0.120005924388162));
#44383=CARTESIAN_POINT('Ctrl Pts',(4.10650113382187,-1.,-0.117099722731705));
#44384=CARTESIAN_POINT('Ctrl Pts',(4.11367603925313,-1.,-0.114156649609602));
#44385=CARTESIAN_POINT('Ctrl Pts',(4.12084512502444,-1.,-0.111177012683378));
#44386=CARTESIAN_POINT('Ctrl Pts',(4.12800848371386,-1.,-0.10816112052835));
#44387=CARTESIAN_POINT('Ctrl Pts',(4.13516614458396,-1.,-0.105109286538864));
#44388=CARTESIAN_POINT('Ctrl Pts',(4.14231804938737,-1.,-0.102021826577454));
#44389=CARTESIAN_POINT('Ctrl Pts',(4.1494640891762,-1.,-0.0988990478899816));
#44390=CARTESIAN_POINT('Ctrl Pts',(4.15660412653006,-1.,-0.0957412403297072));
#44391=CARTESIAN_POINT('Ctrl Pts',(4.16373802265942,-1.,-0.0925486672167695));
#44392=CARTESIAN_POINT('Ctrl Pts',(4.17086566491823,-1.,-0.0893215560850332));
#44393=CARTESIAN_POINT('Ctrl Pts',(4.17798698669991,-1.,-0.086060091555252));
#44394=CARTESIAN_POINT('Ctrl Pts',(4.1851019532944,-1.,-0.0827644164389515));
#44395=CARTESIAN_POINT('Ctrl Pts',(4.19078883322483,-1.,-0.0801005887117608));
#44396=CARTESIAN_POINT('Ctrl Pts',(4.19505112860624,-1.,-0.0780873956244407));
#44397=CARTESIAN_POINT('Ctrl Pts',(4.19789138621624,-1.,-0.07673845961422));
#44398=CARTESIAN_POINT('Ctrl Pts',(4.19931119685982,-1.,-0.0760622897878241));
#44399=CARTESIAN_POINT('',(4.19931119685982,-1.,0.0760622897878241));
#44400=CARTESIAN_POINT('',(4.19931119685982,-1.,-0.0760622897878241));
#44401=CARTESIAN_POINT('',(3.74449296983004,-1.,0.2031560948961));
#44402=CARTESIAN_POINT('Ctrl Pts',(4.19931119685982,-1.,0.0760622897878241));
#44403=CARTESIAN_POINT('Ctrl Pts',(4.1978913862118,-1.,0.0767384596141459));
#44404=CARTESIAN_POINT('Ctrl Pts',(4.19505112859416,-1.,0.0780873956242392));
#44405=CARTESIAN_POINT('Ctrl Pts',(4.19078883320504,-1.,0.0801005887114315));
#44406=CARTESIAN_POINT('Ctrl Pts',(4.18510195327123,-1.,0.0827644164385674));
#44407=CARTESIAN_POINT('Ctrl Pts',(4.17798698668094,-1.,0.0860600915549391));
#44408=CARTESIAN_POINT('Ctrl Pts',(4.17086566490794,-1.,0.0893215560848644));
#44409=CARTESIAN_POINT('Ctrl Pts',(4.16373802265839,-1.,0.0925486672167526));
#44410=CARTESIAN_POINT('Ctrl Pts',(4.15660412653577,-1.,0.0957412403298002));
#44411=CARTESIAN_POINT('Ctrl Pts',(4.14946408918485,-1.,0.0988990478901221));
#44412=CARTESIAN_POINT('Ctrl Pts',(4.14231804939538,-1.,0.102021826577583));
#44413=CARTESIAN_POINT('Ctrl Pts',(4.13516614458895,-1.,0.105109286538945));
#44414=CARTESIAN_POINT('Ctrl Pts',(4.12800848371504,-1.,0.108161120528369));
#44415=CARTESIAN_POINT('Ctrl Pts',(4.1208451250225,-1.,0.111177012683346));
#44416=CARTESIAN_POINT('Ctrl Pts',(4.11367603924961,-1.,0.114156649609545));
#44417=CARTESIAN_POINT('Ctrl Pts',(4.10650113381833,-1.,0.117099722731648));
#44418=CARTESIAN_POINT('Ctrl Pts',(4.09932031767002,-1.,0.120005924388124));
#44419=CARTESIAN_POINT('Ctrl Pts',(4.09213355850756,-1.,0.122874946249106));
#44420=CARTESIAN_POINT('Ctrl Pts',(4.08494093372377,-1.,0.125706476822539));
#44421=CARTESIAN_POINT('Ctrl Pts',(4.07774270738954,-1.,0.128500200484837));
#44422=CARTESIAN_POINT('Ctrl Pts',(4.0705393152874,-1.,0.13125579354894));
#44423=CARTESIAN_POINT('Ctrl Pts',(4.06333121018596,-1.,0.133972916144244));
#44424=CARTESIAN_POINT('Ctrl Pts',(4.05611873400172,-1.,0.136651205046119));
#44425=CARTESIAN_POINT('Ctrl Pts',(4.04890199238036,-1.,0.139290267180057));
#44426=CARTESIAN_POINT('Ctrl Pts',(4.04168069633781,-1.,0.1418896714855));
#44427=CARTESIAN_POINT('Ctrl Pts',(4.03445411510333,-1.,0.144448947038344));
#44428=CARTESIAN_POINT('Ctrl Pts',(4.02722143146994,-1.,0.146967602878994));
#44429=CARTESIAN_POINT('Ctrl Pts',(4.01998203715564,-1.,0.149445144968706));
#44430=CARTESIAN_POINT('Ctrl Pts',(4.01273584234689,-1.,0.15188109402291));
#44431=CARTESIAN_POINT('Ctrl Pts',(4.00548360245319,-1.,0.15427500487231));
#44432=CARTESIAN_POINT('Ctrl Pts',(3.99822717425893,-1.,0.156626481393734));
#44433=CARTESIAN_POINT('Ctrl Pts',(3.99096873945878,-1.,0.158935123982793));
#44434=CARTESIAN_POINT('Ctrl Pts',(3.98371010319872,-1.,0.161200482186084));
#44435=CARTESIAN_POINT('Ctrl Pts',(3.97645194630943,-1.,0.163422004609999));
#44436=CARTESIAN_POINT('Ctrl Pts',(3.96919313621407,-1.,0.165598992851102));
#44437=CARTESIAN_POINT('Ctrl Pts',(3.96192990160296,-1.,0.167730547023319));
#44438=CARTESIAN_POINT('Ctrl Pts',(3.95465744665268,-1.,0.169815666374138));
#44439=CARTESIAN_POINT('Ctrl Pts',(3.94737164900868,-1.,0.17185335536924));
#44440=CARTESIAN_POINT('Ctrl Pts',(3.94007083096217,-1.,0.173842734974609));
#44441=CARTESIAN_POINT('Ctrl Pts',(3.93275726771042,-1.,0.175783136893867));
#44442=CARTESIAN_POINT('Ctrl Pts',(3.92543942697655,-1.,0.177674246152317));
#44443=CARTESIAN_POINT('Ctrl Pts',(3.91812876180926,-1.,0.179515885822881));
#44444=CARTESIAN_POINT('Ctrl Pts',(3.91083557557175,-1.,0.181307740731785));
#44445=CARTESIAN_POINT('Ctrl Pts',(3.90356488555132,-1.,0.18304908199319));
#44446=CARTESIAN_POINT('Ctrl Pts',(3.89631300742646,-1.,0.184738537728042));
#44447=CARTESIAN_POINT('Ctrl Pts',(3.88906196725848,-1.,0.18637372498528));
#44448=CARTESIAN_POINT('Ctrl Pts',(3.88178563496228,-1.,0.187951632512684));
#44449=CARTESIAN_POINT('Ctrl Pts',(3.87445976418412,-1.,0.189469253358272));
#44450=CARTESIAN_POINT('Ctrl Pts',(3.86707158624783,-1.,0.190924190418619));
#44451=CARTESIAN_POINT('Ctrl Pts',(3.85962774407633,-1.,0.19231515304497));
#44452=CARTESIAN_POINT('Ctrl Pts',(3.85216762263966,-1.,0.193642806777722));
#44453=CARTESIAN_POINT('Ctrl Pts',(3.84475203346977,-1.,0.19490900946022));
#44454=CARTESIAN_POINT('Ctrl Pts',(3.83743910616195,-1.,0.196115198971858));
#44455=CARTESIAN_POINT('Ctrl Pts',(3.83026221776456,-1.,0.197260935827361));
#44456=CARTESIAN_POINT('Ctrl Pts',(3.82321127349016,-1.,0.198342616900486));
#44457=CARTESIAN_POINT('Ctrl Pts',(3.81620203429815,-1.,0.199351525297447));
#44458=CARTESIAN_POINT('Ctrl Pts',(3.80909529318669,-1.,0.200274679433364));
#44459=CARTESIAN_POINT('Ctrl Pts',(3.80175247447337,-1.,0.201097756307325));
#44460=CARTESIAN_POINT('Ctrl Pts',(3.7940835418736,-1.,0.201807533800837));
#44461=CARTESIAN_POINT('Ctrl Pts',(3.78609175019242,-1.,0.20239426051216));
#44462=CARTESIAN_POINT('Ctrl Pts',(3.77793553476614,-1.,0.20285472969908));
#44463=CARTESIAN_POINT('Ctrl Pts',(3.7699207159487,-1.,0.203192390045164));
#44464=CARTESIAN_POINT('Ctrl Pts',(3.76242717936885,-1.,0.203414634707478));
#44465=CARTESIAN_POINT('Ctrl Pts',(3.75585118707734,-1.,0.203530796848321));
#44466=CARTESIAN_POINT('Ctrl Pts',(3.75054693397875,-1.,0.203550035479166));
#44467=CARTESIAN_POINT('Ctrl Pts',(3.74703926501752,-1.,0.203484186269415));
#44468=CARTESIAN_POINT('Ctrl Pts',(3.74535749969115,-1.,0.203375226874121));
#44469=CARTESIAN_POINT('Ctrl Pts',(3.74471097893845,-1.,0.20326661011053));
#44470=CARTESIAN_POINT('Ctrl Pts',(3.74453008995092,-1.,0.203188003946656));
#44471=CARTESIAN_POINT('Ctrl Pts',(3.74449296983004,-1.,0.2031560948961));
#44472=CARTESIAN_POINT('',(3.73017266276651,-1.,0.385112848330762));
#44473=CARTESIAN_POINT('Origin',(0.,-1.,0.));
#44474=CARTESIAN_POINT('',(4.15950947128175,-1.,0.581791163835816));
#44475=CARTESIAN_POINT('Ctrl Pts',(3.73017266276651,-1.,0.385112848330762));
#44476=CARTESIAN_POINT('Ctrl Pts',(3.73021431755274,-1.,0.385087139000375));
#44477=CARTESIAN_POINT('Ctrl Pts',(3.73040527621055,-1.,0.385037797881504));
#44478=CARTESIAN_POINT('Ctrl Pts',(3.73106082862548,-1.,0.385031656499164));
#44479=CARTESIAN_POINT('Ctrl Pts',(3.73273893363406,-1.,0.385187124634207));
#44480=CARTESIAN_POINT('Ctrl Pts',(3.73621371845318,-1.,0.385670806454566));
#44481=CARTESIAN_POINT('Ctrl Pts',(3.74144965781276,-1.,0.386519576222252));
#44482=CARTESIAN_POINT('Ctrl Pts',(3.74792651696654,-1.,0.387663020050836));
#44483=CARTESIAN_POINT('Ctrl Pts',(3.75529302895152,-1.,0.389054775898702));
#44484=CARTESIAN_POINT('Ctrl Pts',(3.76315635033257,-1.,0.39064207297956));
#44485=CARTESIAN_POINT('Ctrl Pts',(3.77114011595967,-1.,0.392372786223433));
#44486=CARTESIAN_POINT('Ctrl Pts',(3.77894173114283,-1.,0.3942024810115));
#44487=CARTESIAN_POINT('Ctrl Pts',(3.78640521279313,-1.,0.396103205334841));
#44488=CARTESIAN_POINT('Ctrl Pts',(3.7935288716329,-1.,0.39806481868397));
#44489=CARTESIAN_POINT('Ctrl Pts',(3.80040370384546,-1.,0.400088346504601));
#44490=CARTESIAN_POINT('Ctrl Pts',(3.80716881962728,-1.,0.402181320148436));
#44491=CARTESIAN_POINT('Ctrl Pts',(3.81396374287793,-1.,0.404352694628274));
#44492=CARTESIAN_POINT('Ctrl Pts',(3.8208730391381,-1.,0.406607038258986));
#44493=CARTESIAN_POINT('Ctrl Pts',(3.82790724256471,-1.,0.40894237144746));
#44494=CARTESIAN_POINT('Ctrl Pts',(3.83503345578698,-1.,0.411353038798519));
#44495=CARTESIAN_POINT('Ctrl Pts',(3.84219403994762,-1.,0.413831367016748));
#44496=CARTESIAN_POINT('Ctrl Pts',(3.84932864157497,-1.,0.416369678052907));
#44497=CARTESIAN_POINT('Ctrl Pts',(3.85639825647996,-1.,0.418962468086773));
#44498=CARTESIAN_POINT('Ctrl Pts',(3.86339652542709,-1.,0.421607423177534));
#44499=CARTESIAN_POINT('Ctrl Pts',(3.87033643487851,-1.,0.424304173195111));
#44500=CARTESIAN_POINT('Ctrl Pts',(3.87724240306597,-1.,0.427053541173458));
#44501=CARTESIAN_POINT('Ctrl Pts',(3.88414070943341,-1.,0.429856640579741));
#44502=CARTESIAN_POINT('Ctrl Pts',(3.89104947940611,-1.,0.432713929544459));
#44503=CARTESIAN_POINT('Ctrl Pts',(3.89797256655462,-1.,0.435624629433528));
#44504=CARTESIAN_POINT('Ctrl Pts',(3.90490512938563,-1.,0.43858723545825));
#44505=CARTESIAN_POINT('Ctrl Pts',(3.91183704069153,-1.,0.441599824524055));
#44506=CARTESIAN_POINT('Ctrl Pts',(3.91875701610719,-1.,0.444660430230591));
#44507=CARTESIAN_POINT('Ctrl Pts',(3.92565674143416,-1.,0.447767416837293));
#44508=CARTESIAN_POINT('Ctrl Pts',(3.93253407403123,-1.,0.450919768356349));
#44509=CARTESIAN_POINT('Ctrl Pts',(3.93939080846298,-1.,0.454116879027584));
#44510=CARTESIAN_POINT('Ctrl Pts',(3.94623117206678,-1.,0.457358410451683));
#44511=CARTESIAN_POINT('Ctrl Pts',(3.95306005817364,-1.,0.460644124429122));
#44512=CARTESIAN_POINT('Ctrl Pts',(3.95988133243538,-1.,0.463973722115734));
#44513=CARTESIAN_POINT('Ctrl Pts',(3.9666962227393,-1.,0.467346690880644));
#44514=CARTESIAN_POINT('Ctrl Pts',(3.97350414289392,-1.,0.47076237961344));
#44515=CARTESIAN_POINT('Ctrl Pts',(3.98030338044409,-1.,0.47422006101951));
#44516=CARTESIAN_POINT('Ctrl Pts',(3.98709184306738,-1.,0.477718999122028));
#44517=CARTESIAN_POINT('Ctrl Pts',(3.99386775880679,-1.,0.481258512209676));
#44518=CARTESIAN_POINT('Ctrl Pts',(4.00063045119288,-1.,0.484838042421835));
#44519=CARTESIAN_POINT('Ctrl Pts',(4.0073800839099,-1.,0.488457130424634));
#44520=CARTESIAN_POINT('Ctrl Pts',(4.01411733503546,-1.,0.492115383418019));
#44521=CARTESIAN_POINT('Ctrl Pts',(4.02084308851832,-1.,0.495812444326251));
#44522=CARTESIAN_POINT('Ctrl Pts',(4.02755813980101,-1.,0.499547962340822));
#44523=CARTESIAN_POINT('Ctrl Pts',(4.03426284174272,-1.,0.503321556915346));
#44524=CARTESIAN_POINT('Ctrl Pts',(4.04095715148915,-1.,0.507132823288137));
#44525=CARTESIAN_POINT('Ctrl Pts',(4.04764078815447,-1.,0.510981349218971));
#44526=CARTESIAN_POINT('Ctrl Pts',(4.05431335771199,-1.,0.514866728193017));
#44527=CARTESIAN_POINT('Ctrl Pts',(4.06097448038013,-1.,0.518788572336924));
#44528=CARTESIAN_POINT('Ctrl Pts',(4.06762394471314,-1.,0.522746528603108));
#44529=CARTESIAN_POINT('Ctrl Pts',(4.07426172299847,-1.,0.526740277227498));
#44530=CARTESIAN_POINT('Ctrl Pts',(4.08088789536836,-1.,0.530769518728571));
#44531=CARTESIAN_POINT('Ctrl Pts',(4.08750259988885,-1.,0.534833963477273));
#44532=CARTESIAN_POINT('Ctrl Pts',(4.09410597627,-1.,0.538933321179756));
#44533=CARTESIAN_POINT('Ctrl Pts',(4.10069810243979,-1.,0.543067286877758));
#44534=CARTESIAN_POINT('Ctrl Pts',(4.10727897027977,-1.,0.547235539485637));
#44535=CARTESIAN_POINT('Ctrl Pts',(4.11384852024721,-1.,0.551437758497033));
#44536=CARTESIAN_POINT('Ctrl Pts',(4.12040666195664,-1.,0.555673636129978));
#44537=CARTESIAN_POINT('Ctrl Pts',(4.12695329951961,-1.,0.559942890594774));
#44538=CARTESIAN_POINT('Ctrl Pts',(4.13348835727104,-1.,0.564245279537149));
#44539=CARTESIAN_POINT('Ctrl Pts',(4.14001179830547,-1.,0.568580610189775));
#44540=CARTESIAN_POINT('Ctrl Pts',(4.14652361068081,-1.,0.572948736069523));
#44541=CARTESIAN_POINT('Ctrl Pts',(4.151723761217,-1.,0.576469391676689));
#44542=CARTESIAN_POINT('Ctrl Pts',(4.15561864788576,-1.,0.579124568914236));
#44543=CARTESIAN_POINT('Ctrl Pts',(4.1582129171283,-1.,0.580901211463535));
#44544=CARTESIAN_POINT('Ctrl Pts',(4.15950947128175,-1.,0.581791163835816));
#44545=CARTESIAN_POINT('',(4.13571194405636,-1.,0.732042837400621));
#44546=CARTESIAN_POINT('',(4.15950947128175,-1.,0.581791163835816));
#44547=CARTESIAN_POINT('Ctrl Pts',(4.13571194405636,-1.,0.732042837400621));
#44548=CARTESIAN_POINT('Ctrl Pts',(4.1342038373684,-1.,0.73248857513516));
#44549=CARTESIAN_POINT('Ctrl Pts',(4.13118752795207,-1.,0.733376589323547));
#44550=CARTESIAN_POINT('Ctrl Pts',(4.12666277570844,-1.,0.734698226764093));
#44551=CARTESIAN_POINT('Ctrl Pts',(4.120629196238,-1.,0.736439634331345));
#44552=CARTESIAN_POINT('Ctrl Pts',(4.11308626951927,-1.,0.738581708225844));
#44553=CARTESIAN_POINT('Ctrl Pts',(4.10554241757547,-1.,0.740688998553377));
#44554=CARTESIAN_POINT('Ctrl Pts',(4.09799769702611,-1.,0.742761369689842));
#44555=CARTESIAN_POINT('Ctrl Pts',(4.09045220253573,-1.,0.744798649706501));
#44556=CARTESIAN_POINT('Ctrl Pts',(4.08290608095642,-1.,0.746800631492316));
#44557=CARTESIAN_POINT('Ctrl Pts',(4.07535951056152,-1.,0.748767076680558));
#44558=CARTESIAN_POINT('Ctrl Pts',(4.06781267242378,-1.,0.750697720484037));
#44559=CARTESIAN_POINT('Ctrl Pts',(4.06026572221515,-1.,0.752592276483073));
#44560=CARTESIAN_POINT('Ctrl Pts',(4.05271876687915,-1.,0.754450441816078));
#44561=CARTESIAN_POINT('Ctrl Pts',(4.04517182653997,-1.,0.756271902369581));
#44562=CARTESIAN_POINT('Ctrl Pts',(4.03762485803119,-1.,0.758056338884945));
#44563=CARTESIAN_POINT('Ctrl Pts',(4.03007781954412,-1.,0.759803433243752));
#44564=CARTESIAN_POINT('Ctrl Pts',(4.02253072741268,-1.,0.761512875859805));
#44565=CARTESIAN_POINT('Ctrl Pts',(4.01498370680496,-1.,0.763184371182936));
#44566=CARTESIAN_POINT('Ctrl Pts',(4.00743706791509,-1.,0.764817648785198));
#44567=CARTESIAN_POINT('Ctrl Pts',(3.99989129179622,-1.,0.766412457136064));
#44568=CARTESIAN_POINT('Ctrl Pts',(3.9923468788101,-1.,0.767968531377915));
#44569=CARTESIAN_POINT('Ctrl Pts',(3.98480422348451,-1.,0.769485566245545));
#44570=CARTESIAN_POINT('Ctrl Pts',(3.97726349165488,-1.,0.770963190030471));
#44571=CARTESIAN_POINT('Ctrl Pts',(3.96972446532772,-1.,0.772400931772137));
#44572=CARTESIAN_POINT('Ctrl Pts',(3.96218649639807,-1.,0.773798212026566));
#44573=CARTESIAN_POINT('Ctrl Pts',(3.9546488545231,-1.,0.775154418039352));
#44574=CARTESIAN_POINT('Ctrl Pts',(3.94711101619447,-1.,0.776468966697922));
#44575=CARTESIAN_POINT('Ctrl Pts',(3.93957296768103,-1.,0.777741370568559));
#44576=CARTESIAN_POINT('Ctrl Pts',(3.93203552473174,-1.,0.778971308134821));
#44577=CARTESIAN_POINT('Ctrl Pts',(3.92450058323823,-1.,0.780158678615543));
#44578=CARTESIAN_POINT('Ctrl Pts',(3.91697036054676,-1.,0.781303428618367));
#44579=CARTESIAN_POINT('Ctrl Pts',(3.90944671004542,-1.,0.782405395622765));
#44580=CARTESIAN_POINT('Ctrl Pts',(3.9019303904397,-1.,0.783464141529082));
#44581=CARTESIAN_POINT('Ctrl Pts',(3.89442039235103,-1.,0.784478799358337));
#44582=CARTESIAN_POINT('Ctrl Pts',(3.88691313167398,-1.,0.785447890340731));
#44583=CARTESIAN_POINT('Ctrl Pts',(3.8794040281819,-1.,0.786369675812609));
#44584=CARTESIAN_POINT('Ctrl Pts',(3.87188916600912,-1.,0.787242527617999));
#44585=CARTESIAN_POINT('Ctrl Pts',(3.86436702561345,-1.,0.788065315093778));
#44586=CARTESIAN_POINT('Ctrl Pts',(3.85683995872529,-1.,0.788837734090672));
#44587=CARTESIAN_POINT('Ctrl Pts',(3.84931637808894,-1.,0.789560798155583));
#44588=CARTESIAN_POINT('Ctrl Pts',(3.84180762342454,-1.,0.790236124191243));
#44589=CARTESIAN_POINT('Ctrl Pts',(3.83432392054786,-1.,0.790865012705301));
#44590=CARTESIAN_POINT('Ctrl Pts',(3.82687033899792,-1.,0.791447528662369));
#44591=CARTESIAN_POINT('Ctrl Pts',(3.81944345442249,-1.,0.791981740718635));
#44592=CARTESIAN_POINT('Ctrl Pts',(3.81202588694756,-1.,0.792462483517635));
#44593=CARTESIAN_POINT('Ctrl Pts',(3.80459229925637,-1.,0.792882695234778));
#44594=CARTESIAN_POINT('Ctrl Pts',(3.79711921389897,-1.,0.793235612973274));
#44595=CARTESIAN_POINT('Ctrl Pts',(3.78959439439235,-1.,0.793516871680994));
#44596=CARTESIAN_POINT('Ctrl Pts',(3.78202460377598,-1.,0.793726235781301));
#44597=CARTESIAN_POINT('Ctrl Pts',(3.77444863801212,-1.,0.793870523787408));
#44598=CARTESIAN_POINT('Ctrl Pts',(3.76692626931111,-1.,0.793961083688992));
#44599=CARTESIAN_POINT('Ctrl Pts',(3.75951468666257,-1.,0.794008429134908));
#44600=CARTESIAN_POINT('Ctrl Pts',(3.75224692493864,-1.,0.794017347371378));
#44601=CARTESIAN_POINT('Ctrl Pts',(3.74511357728861,-1.,0.793982700459952));
#44602=CARTESIAN_POINT('Ctrl Pts',(3.73803280541687,-1.,0.793882700937017));
#44603=CARTESIAN_POINT('Ctrl Pts',(3.73086914695805,-1.,0.793682750269684));
#44604=CARTESIAN_POINT('Ctrl Pts',(3.72348797293734,-1.,0.793347023784205));
#44605=CARTESIAN_POINT('Ctrl Pts',(3.71580242396124,-1.,0.792848377370287));
#44606=CARTESIAN_POINT('Ctrl Pts',(3.70781724021806,-1.,0.792177688845818));
#44607=CARTESIAN_POINT('Ctrl Pts',(3.69968940808721,-1.,0.79135657569598));
#44608=CARTESIAN_POINT('Ctrl Pts',(3.69172044327364,-1.,0.790436284988788));
#44609=CARTESIAN_POINT('Ctrl Pts',(3.68428439783905,-1.,0.789483546064387));
#44610=CARTESIAN_POINT('Ctrl Pts',(3.67777119516252,-1.,0.788569566220286));
#44611=CARTESIAN_POINT('Ctrl Pts',(3.67252923663655,-1.,0.787758799995743));
#44612=CARTESIAN_POINT('Ctrl Pts',(3.66907505398677,-1.,0.787145041181546));
#44613=CARTESIAN_POINT('Ctrl Pts',(3.66743103898702,-1.,0.786774337198063));
#44614=CARTESIAN_POINT('Ctrl Pts',(3.66680946938292,-1.,0.786565919558984));
#44615=CARTESIAN_POINT('Ctrl Pts',(3.6666431041522,-1.,0.786459983895432));
#44616=CARTESIAN_POINT('Ctrl Pts',(3.66661143271685,-1.,0.786422660831985));
#44617=CARTESIAN_POINT('Origin',(0.,-1.,0.));
#44618=CARTESIAN_POINT('Origin',(0.,0.,0.));
#44619=CARTESIAN_POINT('Origin',(0.,2.2,0.));
#44620=CARTESIAN_POINT('Origin',(0.,1.,0.));
#44621=CARTESIAN_POINT('',(-2.,2.2,2.44929359829471E-16));
#44622=CARTESIAN_POINT('Origin',(0.,2.2,0.));
#44623=CARTESIAN_POINT('',(-2.,1.,2.44929359829471E-16));
#44624=CARTESIAN_POINT('',(-2.,1.,2.44929359829471E-16));
#44625=CARTESIAN_POINT('Origin',(0.,1.,0.));
#44626=CARTESIAN_POINT('Origin',(0.,2.2,0.));
#44627=CARTESIAN_POINT('Ctrl Pts',(4.15950947128175,-1.,0.581791163835816));
#44628=CARTESIAN_POINT('Ctrl Pts',(4.15950947128175,1.,0.581791163835816));
#44629=CARTESIAN_POINT('Ctrl Pts',(4.1582129171283,-1.,0.580901211463535));
#44630=CARTESIAN_POINT('Ctrl Pts',(4.1582129171283,1.,0.580901211463535));
#44631=CARTESIAN_POINT('Ctrl Pts',(4.15561864788576,-1.,0.579124568914236));
#44632=CARTESIAN_POINT('Ctrl Pts',(4.15561864788576,1.,0.579124568914236));
#44633=CARTESIAN_POINT('Ctrl Pts',(4.151723761217,-1.,0.576469391676689));
#44634=CARTESIAN_POINT('Ctrl Pts',(4.151723761217,1.,0.576469391676689));
#44635=CARTESIAN_POINT('Ctrl Pts',(4.14652361068081,-1.,0.572948736069523));
#44636=CARTESIAN_POINT('Ctrl Pts',(4.14652361068081,1.,0.572948736069523));
#44637=CARTESIAN_POINT('Ctrl Pts',(4.14001179830547,-1.,0.568580610189775));
#44638=CARTESIAN_POINT('Ctrl Pts',(4.14001179830547,1.,0.568580610189775));
#44639=CARTESIAN_POINT('Ctrl Pts',(4.13348835727104,-1.,0.564245279537149));
#44640=CARTESIAN_POINT('Ctrl Pts',(4.13348835727104,1.,0.564245279537149));
#44641=CARTESIAN_POINT('Ctrl Pts',(4.12695329951961,-1.,0.559942890594774));
#44642=CARTESIAN_POINT('Ctrl Pts',(4.12695329951961,1.,0.559942890594774));
#44643=CARTESIAN_POINT('Ctrl Pts',(4.12040666195664,-1.,0.555673636129978));
#44644=CARTESIAN_POINT('Ctrl Pts',(4.12040666195664,1.,0.555673636129978));
#44645=CARTESIAN_POINT('Ctrl Pts',(4.11384852024721,-1.,0.551437758497033));
#44646=CARTESIAN_POINT('Ctrl Pts',(4.11384852024721,1.,0.551437758497033));
#44647=CARTESIAN_POINT('Ctrl Pts',(4.10727897027977,-1.,0.547235539485637));
#44648=CARTESIAN_POINT('Ctrl Pts',(4.10727897027977,1.,0.547235539485637));
#44649=CARTESIAN_POINT('Ctrl Pts',(4.10069810243979,-1.,0.543067286877758));
#44650=CARTESIAN_POINT('Ctrl Pts',(4.10069810243979,1.,0.543067286877758));
#44651=CARTESIAN_POINT('Ctrl Pts',(4.09410597627,-1.,0.538933321179756));
#44652=CARTESIAN_POINT('Ctrl Pts',(4.09410597627,1.,0.538933321179756));
#44653=CARTESIAN_POINT('Ctrl Pts',(4.08750259988885,-1.,0.534833963477273));
#44654=CARTESIAN_POINT('Ctrl Pts',(4.08750259988885,1.,0.534833963477273));
#44655=CARTESIAN_POINT('Ctrl Pts',(4.08088789536836,-1.,0.530769518728571));
#44656=CARTESIAN_POINT('Ctrl Pts',(4.08088789536836,1.,0.530769518728571));
#44657=CARTESIAN_POINT('Ctrl Pts',(4.07426172299847,-1.,0.526740277227498));
#44658=CARTESIAN_POINT('Ctrl Pts',(4.07426172299847,1.,0.526740277227498));
#44659=CARTESIAN_POINT('Ctrl Pts',(4.06762394471314,-1.,0.522746528603108));
#44660=CARTESIAN_POINT('Ctrl Pts',(4.06762394471314,1.,0.522746528603108));
#44661=CARTESIAN_POINT('Ctrl Pts',(4.06097448038013,-1.,0.518788572336924));
#44662=CARTESIAN_POINT('Ctrl Pts',(4.06097448038013,1.,0.518788572336924));
#44663=CARTESIAN_POINT('Ctrl Pts',(4.05431335771199,-1.,0.514866728193017));
#44664=CARTESIAN_POINT('Ctrl Pts',(4.05431335771199,1.,0.514866728193017));
#44665=CARTESIAN_POINT('Ctrl Pts',(4.04764078815447,-1.,0.510981349218971));
#44666=CARTESIAN_POINT('Ctrl Pts',(4.04764078815447,1.,0.510981349218971));
#44667=CARTESIAN_POINT('Ctrl Pts',(4.04095715148915,-1.,0.507132823288137));
#44668=CARTESIAN_POINT('Ctrl Pts',(4.04095715148915,1.,0.507132823288137));
#44669=CARTESIAN_POINT('Ctrl Pts',(4.03426284174272,-1.,0.503321556915346));
#44670=CARTESIAN_POINT('Ctrl Pts',(4.03426284174272,1.,0.503321556915346));
#44671=CARTESIAN_POINT('Ctrl Pts',(4.02755813980101,-1.,0.499547962340822));
#44672=CARTESIAN_POINT('Ctrl Pts',(4.02755813980101,1.,0.499547962340822));
#44673=CARTESIAN_POINT('Ctrl Pts',(4.02084308851832,-1.,0.495812444326251));
#44674=CARTESIAN_POINT('Ctrl Pts',(4.02084308851832,1.,0.495812444326251));
#44675=CARTESIAN_POINT('Ctrl Pts',(4.01411733503546,-1.,0.492115383418019));
#44676=CARTESIAN_POINT('Ctrl Pts',(4.01411733503546,1.,0.492115383418019));
#44677=CARTESIAN_POINT('Ctrl Pts',(4.0073800839099,-1.,0.488457130424634));
#44678=CARTESIAN_POINT('Ctrl Pts',(4.0073800839099,1.,0.488457130424634));
#44679=CARTESIAN_POINT('Ctrl Pts',(4.00063045119288,-1.,0.484838042421835));
#44680=CARTESIAN_POINT('Ctrl Pts',(4.00063045119288,1.,0.484838042421835));
#44681=CARTESIAN_POINT('Ctrl Pts',(3.99386775880679,-1.,0.481258512209676));
#44682=CARTESIAN_POINT('Ctrl Pts',(3.99386775880679,1.,0.481258512209676));
#44683=CARTESIAN_POINT('Ctrl Pts',(3.98709184306738,-1.,0.477718999122028));
#44684=CARTESIAN_POINT('Ctrl Pts',(3.98709184306738,1.,0.477718999122028));
#44685=CARTESIAN_POINT('Ctrl Pts',(3.98030338044409,-1.,0.47422006101951));
#44686=CARTESIAN_POINT('Ctrl Pts',(3.98030338044409,1.,0.47422006101951));
#44687=CARTESIAN_POINT('Ctrl Pts',(3.97350414289392,-1.,0.47076237961344));
#44688=CARTESIAN_POINT('Ctrl Pts',(3.97350414289392,1.,0.47076237961344));
#44689=CARTESIAN_POINT('Ctrl Pts',(3.9666962227393,-1.,0.467346690880644));
#44690=CARTESIAN_POINT('Ctrl Pts',(3.9666962227393,1.,0.467346690880644));
#44691=CARTESIAN_POINT('Ctrl Pts',(3.95988133243538,-1.,0.463973722115734));
#44692=CARTESIAN_POINT('Ctrl Pts',(3.95988133243538,1.,0.463973722115734));
#44693=CARTESIAN_POINT('Ctrl Pts',(3.95306005817364,-1.,0.460644124429122));
#44694=CARTESIAN_POINT('Ctrl Pts',(3.95306005817364,1.,0.460644124429122));
#44695=CARTESIAN_POINT('Ctrl Pts',(3.94623117206678,-1.,0.457358410451683));
#44696=CARTESIAN_POINT('Ctrl Pts',(3.94623117206678,1.,0.457358410451683));
#44697=CARTESIAN_POINT('Ctrl Pts',(3.93939080846298,-1.,0.454116879027584));
#44698=CARTESIAN_POINT('Ctrl Pts',(3.93939080846298,1.,0.454116879027584));
#44699=CARTESIAN_POINT('Ctrl Pts',(3.93253407403123,-1.,0.450919768356349));
#44700=CARTESIAN_POINT('Ctrl Pts',(3.93253407403123,1.,0.450919768356349));
#44701=CARTESIAN_POINT('Ctrl Pts',(3.92565674143416,-1.,0.447767416837293));
#44702=CARTESIAN_POINT('Ctrl Pts',(3.92565674143416,1.,0.447767416837293));
#44703=CARTESIAN_POINT('Ctrl Pts',(3.91875701610719,-1.,0.444660430230591));
#44704=CARTESIAN_POINT('Ctrl Pts',(3.91875701610719,1.,0.444660430230591));
#44705=CARTESIAN_POINT('Ctrl Pts',(3.91183704069153,-1.,0.441599824524055));
#44706=CARTESIAN_POINT('Ctrl Pts',(3.91183704069153,1.,0.441599824524055));
#44707=CARTESIAN_POINT('Ctrl Pts',(3.90490512938563,-1.,0.43858723545825));
#44708=CARTESIAN_POINT('Ctrl Pts',(3.90490512938563,1.,0.43858723545825));
#44709=CARTESIAN_POINT('Ctrl Pts',(3.89797256655462,-1.,0.435624629433528));
#44710=CARTESIAN_POINT('Ctrl Pts',(3.89797256655462,1.,0.435624629433528));
#44711=CARTESIAN_POINT('Ctrl Pts',(3.89104947940611,-1.,0.432713929544459));
#44712=CARTESIAN_POINT('Ctrl Pts',(3.89104947940611,1.,0.432713929544459));
#44713=CARTESIAN_POINT('Ctrl Pts',(3.88414070943341,-1.,0.429856640579741));
#44714=CARTESIAN_POINT('Ctrl Pts',(3.88414070943341,1.,0.429856640579741));
#44715=CARTESIAN_POINT('Ctrl Pts',(3.87724240306597,-1.,0.427053541173458));
#44716=CARTESIAN_POINT('Ctrl Pts',(3.87724240306597,1.,0.427053541173458));
#44717=CARTESIAN_POINT('Ctrl Pts',(3.87033643487851,-1.,0.424304173195111));
#44718=CARTESIAN_POINT('Ctrl Pts',(3.87033643487851,1.,0.424304173195111));
#44719=CARTESIAN_POINT('Ctrl Pts',(3.86339652542709,-1.,0.421607423177534));
#44720=CARTESIAN_POINT('Ctrl Pts',(3.86339652542709,1.,0.421607423177534));
#44721=CARTESIAN_POINT('Ctrl Pts',(3.85639825647996,-1.,0.418962468086773));
#44722=CARTESIAN_POINT('Ctrl Pts',(3.85639825647996,1.,0.418962468086773));
#44723=CARTESIAN_POINT('Ctrl Pts',(3.84932864157497,-1.,0.416369678052907));
#44724=CARTESIAN_POINT('Ctrl Pts',(3.84932864157497,1.,0.416369678052907));
#44725=CARTESIAN_POINT('Ctrl Pts',(3.84219403994762,-1.,0.413831367016748));
#44726=CARTESIAN_POINT('Ctrl Pts',(3.84219403994762,1.,0.413831367016748));
#44727=CARTESIAN_POINT('Ctrl Pts',(3.83503345578698,-1.,0.411353038798519));
#44728=CARTESIAN_POINT('Ctrl Pts',(3.83503345578698,1.,0.411353038798519));
#44729=CARTESIAN_POINT('Ctrl Pts',(3.82790724256471,-1.,0.40894237144746));
#44730=CARTESIAN_POINT('Ctrl Pts',(3.82790724256471,1.,0.40894237144746));
#44731=CARTESIAN_POINT('Ctrl Pts',(3.8208730391381,-1.,0.406607038258986));
#44732=CARTESIAN_POINT('Ctrl Pts',(3.8208730391381,1.,0.406607038258986));
#44733=CARTESIAN_POINT('Ctrl Pts',(3.81396374287793,-1.,0.404352694628274));
#44734=CARTESIAN_POINT('Ctrl Pts',(3.81396374287793,1.,0.404352694628274));
#44735=CARTESIAN_POINT('Ctrl Pts',(3.80716881962728,-1.,0.402181320148436));
#44736=CARTESIAN_POINT('Ctrl Pts',(3.80716881962728,1.,0.402181320148436));
#44737=CARTESIAN_POINT('Ctrl Pts',(3.80040370384546,-1.,0.400088346504601));
#44738=CARTESIAN_POINT('Ctrl Pts',(3.80040370384546,1.,0.400088346504601));
#44739=CARTESIAN_POINT('Ctrl Pts',(3.7935288716329,-1.,0.39806481868397));
#44740=CARTESIAN_POINT('Ctrl Pts',(3.7935288716329,1.,0.39806481868397));
#44741=CARTESIAN_POINT('Ctrl Pts',(3.78640521279313,-1.,0.396103205334841));
#44742=CARTESIAN_POINT('Ctrl Pts',(3.78640521279313,1.,0.396103205334841));
#44743=CARTESIAN_POINT('Ctrl Pts',(3.77894173114283,-1.,0.3942024810115));
#44744=CARTESIAN_POINT('Ctrl Pts',(3.77894173114283,1.,0.3942024810115));
#44745=CARTESIAN_POINT('Ctrl Pts',(3.77114011595967,-1.,0.392372786223433));
#44746=CARTESIAN_POINT('Ctrl Pts',(3.77114011595967,1.,0.392372786223433));
#44747=CARTESIAN_POINT('Ctrl Pts',(3.76315635033257,-1.,0.39064207297956));
#44748=CARTESIAN_POINT('Ctrl Pts',(3.76315635033257,1.,0.39064207297956));
#44749=CARTESIAN_POINT('Ctrl Pts',(3.75529302895152,-1.,0.389054775898702));
#44750=CARTESIAN_POINT('Ctrl Pts',(3.75529302895152,1.,0.389054775898702));
#44751=CARTESIAN_POINT('Ctrl Pts',(3.74792651696654,-1.,0.387663020050836));
#44752=CARTESIAN_POINT('Ctrl Pts',(3.74792651696654,1.,0.387663020050836));
#44753=CARTESIAN_POINT('Ctrl Pts',(3.74144965781276,-1.,0.386519576222252));
#44754=CARTESIAN_POINT('Ctrl Pts',(3.74144965781276,1.,0.386519576222252));
#44755=CARTESIAN_POINT('Ctrl Pts',(3.73621371845318,-1.,0.385670806454566));
#44756=CARTESIAN_POINT('Ctrl Pts',(3.73621371845318,1.,0.385670806454566));
#44757=CARTESIAN_POINT('Ctrl Pts',(3.73245705638843,-1.,0.385147887988952));
#44758=CARTESIAN_POINT('Ctrl Pts',(3.73245705638843,1.,0.385147887988952));
#44759=CARTESIAN_POINT('Ctrl Pts',(3.73072465900175,-1.,0.385001870183213));
#44760=CARTESIAN_POINT('Ctrl Pts',(3.73072465900175,1.,0.385001870183213));
#44761=CARTESIAN_POINT('Ctrl Pts',(3.73015851028356,-1.,0.385047711603463));
#44762=CARTESIAN_POINT('Ctrl Pts',(3.73015851028356,1.,0.385047711603463));
#44763=CARTESIAN_POINT('Ctrl Pts',(3.73010668803042,-1.,0.385147278814643));
#44764=CARTESIAN_POINT('Ctrl Pts',(3.73010668803042,1.,0.385147278814643));
#44765=CARTESIAN_POINT('Ctrl Pts',(3.73016218570874,-1.,0.38521431477633));
#44766=CARTESIAN_POINT('Ctrl Pts',(3.73016218570874,1.,0.38521431477633));
#44767=CARTESIAN_POINT('',(3.73017266276651,1.,0.385112848330762));
#44768=CARTESIAN_POINT('Ctrl Pts',(3.73017266276651,1.,0.385112848330762));
#44769=CARTESIAN_POINT('Ctrl Pts',(3.73017266276651,0.666666666666667,0.385112848330762));
#44770=CARTESIAN_POINT('Ctrl Pts',(3.73017266276651,0.333333333333333,0.385112848330762));
#44771=CARTESIAN_POINT('Ctrl Pts',(3.73017266276651,-0.333333333333333,
0.385112848330762));
#44772=CARTESIAN_POINT('Ctrl Pts',(3.73017266276651,-0.666666666666667,
0.385112848330763));
#44773=CARTESIAN_POINT('Ctrl Pts',(3.73017266276651,-1.,0.385112848330763));
#44774=CARTESIAN_POINT('',(4.15950947128175,1.,0.581791163835816));
#44775=CARTESIAN_POINT('Ctrl Pts',(4.15950947128175,1.,0.581791163835816));
#44776=CARTESIAN_POINT('Ctrl Pts',(4.1582129171283,1.,0.580901211463535));
#44777=CARTESIAN_POINT('Ctrl Pts',(4.15561864788576,1.,0.579124568914236));
#44778=CARTESIAN_POINT('Ctrl Pts',(4.151723761217,1.,0.576469391676689));
#44779=CARTESIAN_POINT('Ctrl Pts',(4.14652361068081,1.,0.572948736069523));
#44780=CARTESIAN_POINT('Ctrl Pts',(4.14001179830547,1.,0.568580610189775));
#44781=CARTESIAN_POINT('Ctrl Pts',(4.13348835727104,1.,0.564245279537149));
#44782=CARTESIAN_POINT('Ctrl Pts',(4.12695329951961,1.,0.559942890594774));
#44783=CARTESIAN_POINT('Ctrl Pts',(4.12040666195664,1.,0.555673636129978));
#44784=CARTESIAN_POINT('Ctrl Pts',(4.11384852024721,1.,0.551437758497033));
#44785=CARTESIAN_POINT('Ctrl Pts',(4.10727897027977,1.,0.547235539485637));
#44786=CARTESIAN_POINT('Ctrl Pts',(4.10069810243979,1.,0.543067286877758));
#44787=CARTESIAN_POINT('Ctrl Pts',(4.09410597627,1.,0.538933321179756));
#44788=CARTESIAN_POINT('Ctrl Pts',(4.08750259988885,1.,0.534833963477273));
#44789=CARTESIAN_POINT('Ctrl Pts',(4.08088789536836,1.,0.530769518728571));
#44790=CARTESIAN_POINT('Ctrl Pts',(4.07426172299847,1.,0.526740277227498));
#44791=CARTESIAN_POINT('Ctrl Pts',(4.06762394471314,1.,0.522746528603108));
#44792=CARTESIAN_POINT('Ctrl Pts',(4.06097448038013,1.,0.518788572336924));
#44793=CARTESIAN_POINT('Ctrl Pts',(4.05431335771199,1.,0.514866728193017));
#44794=CARTESIAN_POINT('Ctrl Pts',(4.04764078815447,1.,0.510981349218971));
#44795=CARTESIAN_POINT('Ctrl Pts',(4.04095715148915,1.,0.507132823288137));
#44796=CARTESIAN_POINT('Ctrl Pts',(4.03426284174272,1.,0.503321556915346));
#44797=CARTESIAN_POINT('Ctrl Pts',(4.02755813980101,1.,0.499547962340822));
#44798=CARTESIAN_POINT('Ctrl Pts',(4.02084308851832,1.,0.495812444326251));
#44799=CARTESIAN_POINT('Ctrl Pts',(4.01411733503546,1.,0.492115383418019));
#44800=CARTESIAN_POINT('Ctrl Pts',(4.0073800839099,1.,0.488457130424634));
#44801=CARTESIAN_POINT('Ctrl Pts',(4.00063045119288,1.,0.484838042421835));
#44802=CARTESIAN_POINT('Ctrl Pts',(3.99386775880679,1.,0.481258512209676));
#44803=CARTESIAN_POINT('Ctrl Pts',(3.98709184306738,1.,0.477718999122028));
#44804=CARTESIAN_POINT('Ctrl Pts',(3.98030338044409,1.,0.47422006101951));
#44805=CARTESIAN_POINT('Ctrl Pts',(3.97350414289392,1.,0.47076237961344));
#44806=CARTESIAN_POINT('Ctrl Pts',(3.9666962227393,1.,0.467346690880644));
#44807=CARTESIAN_POINT('Ctrl Pts',(3.95988133243538,1.,0.463973722115734));
#44808=CARTESIAN_POINT('Ctrl Pts',(3.95306005817364,1.,0.460644124429122));
#44809=CARTESIAN_POINT('Ctrl Pts',(3.94623117206678,1.,0.457358410451683));
#44810=CARTESIAN_POINT('Ctrl Pts',(3.93939080846298,1.,0.454116879027584));
#44811=CARTESIAN_POINT('Ctrl Pts',(3.93253407403123,1.,0.450919768356349));
#44812=CARTESIAN_POINT('Ctrl Pts',(3.92565674143416,1.,0.447767416837293));
#44813=CARTESIAN_POINT('Ctrl Pts',(3.91875701610719,1.,0.444660430230591));
#44814=CARTESIAN_POINT('Ctrl Pts',(3.91183704069153,1.,0.441599824524055));
#44815=CARTESIAN_POINT('Ctrl Pts',(3.90490512938563,1.,0.43858723545825));
#44816=CARTESIAN_POINT('Ctrl Pts',(3.89797256655462,1.,0.435624629433528));
#44817=CARTESIAN_POINT('Ctrl Pts',(3.89104947940611,1.,0.432713929544459));
#44818=CARTESIAN_POINT('Ctrl Pts',(3.88414070943341,1.,0.429856640579741));
#44819=CARTESIAN_POINT('Ctrl Pts',(3.87724240306597,1.,0.427053541173458));
#44820=CARTESIAN_POINT('Ctrl Pts',(3.87033643487851,1.,0.424304173195111));
#44821=CARTESIAN_POINT('Ctrl Pts',(3.86339652542709,1.,0.421607423177534));
#44822=CARTESIAN_POINT('Ctrl Pts',(3.85639825647996,1.,0.418962468086773));
#44823=CARTESIAN_POINT('Ctrl Pts',(3.84932864157497,1.,0.416369678052907));
#44824=CARTESIAN_POINT('Ctrl Pts',(3.84219403994762,1.,0.413831367016748));
#44825=CARTESIAN_POINT('Ctrl Pts',(3.83503345578698,1.,0.411353038798519));
#44826=CARTESIAN_POINT('Ctrl Pts',(3.82790724256471,1.,0.40894237144746));
#44827=CARTESIAN_POINT('Ctrl Pts',(3.8208730391381,1.,0.406607038258986));
#44828=CARTESIAN_POINT('Ctrl Pts',(3.81396374287793,1.,0.404352694628274));
#44829=CARTESIAN_POINT('Ctrl Pts',(3.80716881962728,1.,0.402181320148436));
#44830=CARTESIAN_POINT('Ctrl Pts',(3.80040370384546,1.,0.400088346504601));
#44831=CARTESIAN_POINT('Ctrl Pts',(3.7935288716329,1.,0.39806481868397));
#44832=CARTESIAN_POINT('Ctrl Pts',(3.78640521279313,1.,0.396103205334841));
#44833=CARTESIAN_POINT('Ctrl Pts',(3.77894173114283,1.,0.3942024810115));
#44834=CARTESIAN_POINT('Ctrl Pts',(3.77114011595967,1.,0.392372786223433));
#44835=CARTESIAN_POINT('Ctrl Pts',(3.76315635033257,1.,0.39064207297956));
#44836=CARTESIAN_POINT('Ctrl Pts',(3.75529302895152,1.,0.389054775898702));
#44837=CARTESIAN_POINT('Ctrl Pts',(3.74792651696654,1.,0.387663020050836));
#44838=CARTESIAN_POINT('Ctrl Pts',(3.74144965781276,1.,0.386519576222252));
#44839=CARTESIAN_POINT('Ctrl Pts',(3.73621371845318,1.,0.385670806454566));
#44840=CARTESIAN_POINT('Ctrl Pts',(3.73273893363406,1.,0.385187124634207));
#44841=CARTESIAN_POINT('Ctrl Pts',(3.73106082862548,1.,0.385031656499164));
#44842=CARTESIAN_POINT('Ctrl Pts',(3.73040527621055,1.,0.385037797881504));
#44843=CARTESIAN_POINT('Ctrl Pts',(3.73021431755274,1.,0.385087139000375));
#44844=CARTESIAN_POINT('Ctrl Pts',(3.73017266276651,1.,0.385112848330762));
#44845=CARTESIAN_POINT('',(4.15950947128175,0.,0.581791163835816));
#44846=CARTESIAN_POINT('Ctrl Pts',(3.66663282329846,-1.,0.7863229229206));
#44847=CARTESIAN_POINT('Ctrl Pts',(3.66663282329846,1.,0.7863229229206));
#44848=CARTESIAN_POINT('Ctrl Pts',(3.66655932661986,-1.,0.786369528183326));
#44849=CARTESIAN_POINT('Ctrl Pts',(3.66655932661986,1.,0.786369528183326));
#44850=CARTESIAN_POINT('Ctrl Pts',(3.66657784455334,-1.,0.786480236185697));
#44851=CARTESIAN_POINT('Ctrl Pts',(3.66657784455334,1.,0.786480236185697));
#44852=CARTESIAN_POINT('Ctrl Pts',(3.66710211820482,-1.,0.786698783542764));
#44853=CARTESIAN_POINT('Ctrl Pts',(3.66710211820482,1.,0.786698783542764));
#44854=CARTESIAN_POINT('Ctrl Pts',(3.66879484801113,-1.,0.787095252590501));
#44855=CARTESIAN_POINT('Ctrl Pts',(3.66879484801113,1.,0.787095252590501));
#44856=CARTESIAN_POINT('Ctrl Pts',(3.67252923663655,-1.,0.787758799995743));
#44857=CARTESIAN_POINT('Ctrl Pts',(3.67252923663655,1.,0.787758799995743));
#44858=CARTESIAN_POINT('Ctrl Pts',(3.67777119516252,-1.,0.788569566220286));
#44859=CARTESIAN_POINT('Ctrl Pts',(3.67777119516252,1.,0.788569566220286));
#44860=CARTESIAN_POINT('Ctrl Pts',(3.68428439783905,-1.,0.789483546064387));
#44861=CARTESIAN_POINT('Ctrl Pts',(3.68428439783905,1.,0.789483546064387));
#44862=CARTESIAN_POINT('Ctrl Pts',(3.69172044327364,-1.,0.790436284988788));
#44863=CARTESIAN_POINT('Ctrl Pts',(3.69172044327364,1.,0.790436284988788));
#44864=CARTESIAN_POINT('Ctrl Pts',(3.69968940808721,-1.,0.79135657569598));
#44865=CARTESIAN_POINT('Ctrl Pts',(3.69968940808721,1.,0.79135657569598));
#44866=CARTESIAN_POINT('Ctrl Pts',(3.70781724021806,-1.,0.792177688845818));
#44867=CARTESIAN_POINT('Ctrl Pts',(3.70781724021806,1.,0.792177688845818));
#44868=CARTESIAN_POINT('Ctrl Pts',(3.71580242396124,-1.,0.792848377370287));
#44869=CARTESIAN_POINT('Ctrl Pts',(3.71580242396124,1.,0.792848377370287));
#44870=CARTESIAN_POINT('Ctrl Pts',(3.72348797293734,-1.,0.793347023784205));
#44871=CARTESIAN_POINT('Ctrl Pts',(3.72348797293734,1.,0.793347023784205));
#44872=CARTESIAN_POINT('Ctrl Pts',(3.73086914695805,-1.,0.793682750269684));
#44873=CARTESIAN_POINT('Ctrl Pts',(3.73086914695805,1.,0.793682750269684));
#44874=CARTESIAN_POINT('Ctrl Pts',(3.73803280541687,-1.,0.793882700937017));
#44875=CARTESIAN_POINT('Ctrl Pts',(3.73803280541687,1.,0.793882700937017));
#44876=CARTESIAN_POINT('Ctrl Pts',(3.74511357728861,-1.,0.793982700459952));
#44877=CARTESIAN_POINT('Ctrl Pts',(3.74511357728861,1.,0.793982700459952));
#44878=CARTESIAN_POINT('Ctrl Pts',(3.75224692493864,-1.,0.794017347371378));
#44879=CARTESIAN_POINT('Ctrl Pts',(3.75224692493864,1.,0.794017347371378));
#44880=CARTESIAN_POINT('Ctrl Pts',(3.75951468666257,-1.,0.794008429134908));
#44881=CARTESIAN_POINT('Ctrl Pts',(3.75951468666257,1.,0.794008429134908));
#44882=CARTESIAN_POINT('Ctrl Pts',(3.76692626931111,-1.,0.793961083688992));
#44883=CARTESIAN_POINT('Ctrl Pts',(3.76692626931111,1.,0.793961083688992));
#44884=CARTESIAN_POINT('Ctrl Pts',(3.77444863801212,-1.,0.793870523787408));
#44885=CARTESIAN_POINT('Ctrl Pts',(3.77444863801212,1.,0.793870523787408));
#44886=CARTESIAN_POINT('Ctrl Pts',(3.78202460377598,-1.,0.793726235781301));
#44887=CARTESIAN_POINT('Ctrl Pts',(3.78202460377598,1.,0.793726235781301));
#44888=CARTESIAN_POINT('Ctrl Pts',(3.78959439439235,-1.,0.793516871680994));
#44889=CARTESIAN_POINT('Ctrl Pts',(3.78959439439235,1.,0.793516871680994));
#44890=CARTESIAN_POINT('Ctrl Pts',(3.79711921389897,-1.,0.793235612973274));
#44891=CARTESIAN_POINT('Ctrl Pts',(3.79711921389897,1.,0.793235612973274));
#44892=CARTESIAN_POINT('Ctrl Pts',(3.80459229925637,-1.,0.792882695234778));
#44893=CARTESIAN_POINT('Ctrl Pts',(3.80459229925637,1.,0.792882695234778));
#44894=CARTESIAN_POINT('Ctrl Pts',(3.81202588694756,-1.,0.792462483517635));
#44895=CARTESIAN_POINT('Ctrl Pts',(3.81202588694756,1.,0.792462483517635));
#44896=CARTESIAN_POINT('Ctrl Pts',(3.81944345442249,-1.,0.791981740718635));
#44897=CARTESIAN_POINT('Ctrl Pts',(3.81944345442249,1.,0.791981740718635));
#44898=CARTESIAN_POINT('Ctrl Pts',(3.82687033899792,-1.,0.791447528662369));
#44899=CARTESIAN_POINT('Ctrl Pts',(3.82687033899792,1.,0.791447528662369));
#44900=CARTESIAN_POINT('Ctrl Pts',(3.83432392054786,-1.,0.790865012705301));
#44901=CARTESIAN_POINT('Ctrl Pts',(3.83432392054786,1.,0.790865012705301));
#44902=CARTESIAN_POINT('Ctrl Pts',(3.84180762342454,-1.,0.790236124191243));
#44903=CARTESIAN_POINT('Ctrl Pts',(3.84180762342454,1.,0.790236124191243));
#44904=CARTESIAN_POINT('Ctrl Pts',(3.84931637808894,-1.,0.789560798155583));
#44905=CARTESIAN_POINT('Ctrl Pts',(3.84931637808894,1.,0.789560798155583));
#44906=CARTESIAN_POINT('Ctrl Pts',(3.85683995872529,-1.,0.788837734090672));
#44907=CARTESIAN_POINT('Ctrl Pts',(3.85683995872529,1.,0.788837734090672));
#44908=CARTESIAN_POINT('Ctrl Pts',(3.86436702561345,-1.,0.788065315093778));
#44909=CARTESIAN_POINT('Ctrl Pts',(3.86436702561345,1.,0.788065315093778));
#44910=CARTESIAN_POINT('Ctrl Pts',(3.87188916600912,-1.,0.787242527617999));
#44911=CARTESIAN_POINT('Ctrl Pts',(3.87188916600912,1.,0.787242527617999));
#44912=CARTESIAN_POINT('Ctrl Pts',(3.8794040281819,-1.,0.786369675812609));
#44913=CARTESIAN_POINT('Ctrl Pts',(3.8794040281819,1.,0.786369675812609));
#44914=CARTESIAN_POINT('Ctrl Pts',(3.88691313167398,-1.,0.785447890340731));
#44915=CARTESIAN_POINT('Ctrl Pts',(3.88691313167398,1.,0.785447890340731));
#44916=CARTESIAN_POINT('Ctrl Pts',(3.89442039235103,-1.,0.784478799358337));
#44917=CARTESIAN_POINT('Ctrl Pts',(3.89442039235103,1.,0.784478799358337));
#44918=CARTESIAN_POINT('Ctrl Pts',(3.9019303904397,-1.,0.783464141529082));
#44919=CARTESIAN_POINT('Ctrl Pts',(3.9019303904397,1.,0.783464141529082));
#44920=CARTESIAN_POINT('Ctrl Pts',(3.90944671004542,-1.,0.782405395622765));
#44921=CARTESIAN_POINT('Ctrl Pts',(3.90944671004542,1.,0.782405395622765));
#44922=CARTESIAN_POINT('Ctrl Pts',(3.91697036054676,-1.,0.781303428618367));
#44923=CARTESIAN_POINT('Ctrl Pts',(3.91697036054676,1.,0.781303428618367));
#44924=CARTESIAN_POINT('Ctrl Pts',(3.92450058323823,-1.,0.780158678615543));
#44925=CARTESIAN_POINT('Ctrl Pts',(3.92450058323823,1.,0.780158678615543));
#44926=CARTESIAN_POINT('Ctrl Pts',(3.93203552473174,-1.,0.778971308134821));
#44927=CARTESIAN_POINT('Ctrl Pts',(3.93203552473174,1.,0.778971308134821));
#44928=CARTESIAN_POINT('Ctrl Pts',(3.93957296768103,-1.,0.777741370568559));
#44929=CARTESIAN_POINT('Ctrl Pts',(3.93957296768103,1.,0.777741370568559));
#44930=CARTESIAN_POINT('Ctrl Pts',(3.94711101619447,-1.,0.776468966697922));
#44931=CARTESIAN_POINT('Ctrl Pts',(3.94711101619447,1.,0.776468966697922));
#44932=CARTESIAN_POINT('Ctrl Pts',(3.9546488545231,-1.,0.775154418039352));
#44933=CARTESIAN_POINT('Ctrl Pts',(3.9546488545231,1.,0.775154418039352));
#44934=CARTESIAN_POINT('Ctrl Pts',(3.96218649639807,-1.,0.773798212026566));
#44935=CARTESIAN_POINT('Ctrl Pts',(3.96218649639807,1.,0.773798212026566));
#44936=CARTESIAN_POINT('Ctrl Pts',(3.96972446532772,-1.,0.772400931772137));
#44937=CARTESIAN_POINT('Ctrl Pts',(3.96972446532772,1.,0.772400931772137));
#44938=CARTESIAN_POINT('Ctrl Pts',(3.97726349165488,-1.,0.770963190030471));
#44939=CARTESIAN_POINT('Ctrl Pts',(3.97726349165488,1.,0.770963190030471));
#44940=CARTESIAN_POINT('Ctrl Pts',(3.98480422348451,-1.,0.769485566245545));
#44941=CARTESIAN_POINT('Ctrl Pts',(3.98480422348451,1.,0.769485566245545));
#44942=CARTESIAN_POINT('Ctrl Pts',(3.9923468788101,-1.,0.767968531377915));
#44943=CARTESIAN_POINT('Ctrl Pts',(3.9923468788101,1.,0.767968531377915));
#44944=CARTESIAN_POINT('Ctrl Pts',(3.99989129179622,-1.,0.766412457136064));
#44945=CARTESIAN_POINT('Ctrl Pts',(3.99989129179622,1.,0.766412457136064));
#44946=CARTESIAN_POINT('Ctrl Pts',(4.00743706791509,-1.,0.764817648785198));
#44947=CARTESIAN_POINT('Ctrl Pts',(4.00743706791509,1.,0.764817648785198));
#44948=CARTESIAN_POINT('Ctrl Pts',(4.01498370680496,-1.,0.763184371182936));
#44949=CARTESIAN_POINT('Ctrl Pts',(4.01498370680496,1.,0.763184371182936));
#44950=CARTESIAN_POINT('Ctrl Pts',(4.02253072741268,-1.,0.761512875859805));
#44951=CARTESIAN_POINT('Ctrl Pts',(4.02253072741268,1.,0.761512875859805));
#44952=CARTESIAN_POINT('Ctrl Pts',(4.03007781954412,-1.,0.759803433243752));
#44953=CARTESIAN_POINT('Ctrl Pts',(4.03007781954412,1.,0.759803433243752));
#44954=CARTESIAN_POINT('Ctrl Pts',(4.03762485803119,-1.,0.758056338884945));
#44955=CARTESIAN_POINT('Ctrl Pts',(4.03762485803119,1.,0.758056338884945));
#44956=CARTESIAN_POINT('Ctrl Pts',(4.04517182653997,-1.,0.756271902369581));
#44957=CARTESIAN_POINT('Ctrl Pts',(4.04517182653997,1.,0.756271902369581));
#44958=CARTESIAN_POINT('Ctrl Pts',(4.05271876687915,-1.,0.754450441816078));
#44959=CARTESIAN_POINT('Ctrl Pts',(4.05271876687915,1.,0.754450441816078));
#44960=CARTESIAN_POINT('Ctrl Pts',(4.06026572221515,-1.,0.752592276483073));
#44961=CARTESIAN_POINT('Ctrl Pts',(4.06026572221515,1.,0.752592276483073));
#44962=CARTESIAN_POINT('Ctrl Pts',(4.06781267242378,-1.,0.750697720484037));
#44963=CARTESIAN_POINT('Ctrl Pts',(4.06781267242378,1.,0.750697720484037));
#44964=CARTESIAN_POINT('Ctrl Pts',(4.07535951056152,-1.,0.748767076680558));
#44965=CARTESIAN_POINT('Ctrl Pts',(4.07535951056152,1.,0.748767076680558));
#44966=CARTESIAN_POINT('Ctrl Pts',(4.08290608095642,-1.,0.746800631492316));
#44967=CARTESIAN_POINT('Ctrl Pts',(4.08290608095642,1.,0.746800631492316));
#44968=CARTESIAN_POINT('Ctrl Pts',(4.09045220253573,-1.,0.744798649706501));
#44969=CARTESIAN_POINT('Ctrl Pts',(4.09045220253573,1.,0.744798649706501));
#44970=CARTESIAN_POINT('Ctrl Pts',(4.09799769702611,-1.,0.742761369689842));
#44971=CARTESIAN_POINT('Ctrl Pts',(4.09799769702611,1.,0.742761369689842));
#44972=CARTESIAN_POINT('Ctrl Pts',(4.10554241757547,-1.,0.740688998553377));
#44973=CARTESIAN_POINT('Ctrl Pts',(4.10554241757547,1.,0.740688998553377));
#44974=CARTESIAN_POINT('Ctrl Pts',(4.11308626951927,-1.,0.738581708225844));
#44975=CARTESIAN_POINT('Ctrl Pts',(4.11308626951927,1.,0.738581708225844));
#44976=CARTESIAN_POINT('Ctrl Pts',(4.120629196238,-1.,0.736439634331345));
#44977=CARTESIAN_POINT('Ctrl Pts',(4.120629196238,1.,0.736439634331345));
#44978=CARTESIAN_POINT('Ctrl Pts',(4.12666277570844,-1.,0.734698226764093));
#44979=CARTESIAN_POINT('Ctrl Pts',(4.12666277570844,1.,0.734698226764093));
#44980=CARTESIAN_POINT('Ctrl Pts',(4.13118752795207,-1.,0.733376589323547));
#44981=CARTESIAN_POINT('Ctrl Pts',(4.13118752795207,1.,0.733376589323547));
#44982=CARTESIAN_POINT('Ctrl Pts',(4.1342038373684,-1.,0.73248857513516));
#44983=CARTESIAN_POINT('Ctrl Pts',(4.1342038373684,1.,0.73248857513516));
#44984=CARTESIAN_POINT('Ctrl Pts',(4.13571194405636,-1.,0.732042837400621));
#44985=CARTESIAN_POINT('Ctrl Pts',(4.13571194405636,1.,0.732042837400621));
#44986=CARTESIAN_POINT('',(3.66661143271685,1.,0.786422660831985));
#44987=CARTESIAN_POINT('Ctrl Pts',(3.66661143271685,-1.,0.786422660831986));
#44988=CARTESIAN_POINT('Ctrl Pts',(3.66661143271685,-0.666666666666667,
0.786422660831986));
#44989=CARTESIAN_POINT('Ctrl Pts',(3.66661143271685,-0.333333333333333,
0.786422660831986));
#44990=CARTESIAN_POINT('Ctrl Pts',(3.66661143271685,0.333333333333333,0.786422660831986));
#44991=CARTESIAN_POINT('Ctrl Pts',(3.66661143271685,0.666666666666667,0.786422660831986));
#44992=CARTESIAN_POINT('Ctrl Pts',(3.66661143271685,1.,0.786422660831986));
#44993=CARTESIAN_POINT('',(4.13571194405636,1.,0.732042837400621));
#44994=CARTESIAN_POINT('',(4.13571194405636,0.,0.732042837400621));
#44995=CARTESIAN_POINT('Ctrl Pts',(3.66661143271685,1.,0.786422660831985));
#44996=CARTESIAN_POINT('Ctrl Pts',(3.6666431041522,1.,0.786459983895432));
#44997=CARTESIAN_POINT('Ctrl Pts',(3.66680946938292,1.,0.786565919558984));
#44998=CARTESIAN_POINT('Ctrl Pts',(3.66743103898702,1.,0.786774337198063));
#44999=CARTESIAN_POINT('Ctrl Pts',(3.66907505398677,1.,0.787145041181546));
#45000=CARTESIAN_POINT('Ctrl Pts',(3.67252923663655,1.,0.787758799995743));
#45001=CARTESIAN_POINT('Ctrl Pts',(3.67777119516252,1.,0.788569566220286));
#45002=CARTESIAN_POINT('Ctrl Pts',(3.68428439783905,1.,0.789483546064387));
#45003=CARTESIAN_POINT('Ctrl Pts',(3.69172044327364,1.,0.790436284988788));
#45004=CARTESIAN_POINT('Ctrl Pts',(3.69968940808721,1.,0.79135657569598));
#45005=CARTESIAN_POINT('Ctrl Pts',(3.70781724021806,1.,0.792177688845818));
#45006=CARTESIAN_POINT('Ctrl Pts',(3.71580242396124,1.,0.792848377370287));
#45007=CARTESIAN_POINT('Ctrl Pts',(3.72348797293734,1.,0.793347023784205));
#45008=CARTESIAN_POINT('Ctrl Pts',(3.73086914695805,1.,0.793682750269684));
#45009=CARTESIAN_POINT('Ctrl Pts',(3.73803280541687,1.,0.793882700937017));
#45010=CARTESIAN_POINT('Ctrl Pts',(3.74511357728861,1.,0.793982700459952));
#45011=CARTESIAN_POINT('Ctrl Pts',(3.75224692493864,1.,0.794017347371378));
#45012=CARTESIAN_POINT('Ctrl Pts',(3.75951468666257,1.,0.794008429134908));
#45013=CARTESIAN_POINT('Ctrl Pts',(3.76692626931111,1.,0.793961083688992));
#45014=CARTESIAN_POINT('Ctrl Pts',(3.77444863801212,1.,0.793870523787408));
#45015=CARTESIAN_POINT('Ctrl Pts',(3.78202460377598,1.,0.793726235781301));
#45016=CARTESIAN_POINT('Ctrl Pts',(3.78959439439235,1.,0.793516871680994));
#45017=CARTESIAN_POINT('Ctrl Pts',(3.79711921389897,1.,0.793235612973274));
#45018=CARTESIAN_POINT('Ctrl Pts',(3.80459229925637,1.,0.792882695234778));
#45019=CARTESIAN_POINT('Ctrl Pts',(3.81202588694756,1.,0.792462483517635));
#45020=CARTESIAN_POINT('Ctrl Pts',(3.81944345442249,1.,0.791981740718635));
#45021=CARTESIAN_POINT('Ctrl Pts',(3.82687033899792,1.,0.791447528662369));
#45022=CARTESIAN_POINT('Ctrl Pts',(3.83432392054786,1.,0.790865012705301));
#45023=CARTESIAN_POINT('Ctrl Pts',(3.84180762342454,1.,0.790236124191243));
#45024=CARTESIAN_POINT('Ctrl Pts',(3.84931637808894,1.,0.789560798155583));
#45025=CARTESIAN_POINT('Ctrl Pts',(3.85683995872529,1.,0.788837734090672));
#45026=CARTESIAN_POINT('Ctrl Pts',(3.86436702561345,1.,0.788065315093778));
#45027=CARTESIAN_POINT('Ctrl Pts',(3.87188916600912,1.,0.787242527617999));
#45028=CARTESIAN_POINT('Ctrl Pts',(3.8794040281819,1.,0.786369675812609));
#45029=CARTESIAN_POINT('Ctrl Pts',(3.88691313167398,1.,0.785447890340731));
#45030=CARTESIAN_POINT('Ctrl Pts',(3.89442039235103,1.,0.784478799358337));
#45031=CARTESIAN_POINT('Ctrl Pts',(3.9019303904397,1.,0.783464141529082));
#45032=CARTESIAN_POINT('Ctrl Pts',(3.90944671004542,1.,0.782405395622765));
#45033=CARTESIAN_POINT('Ctrl Pts',(3.91697036054676,1.,0.781303428618367));
#45034=CARTESIAN_POINT('Ctrl Pts',(3.92450058323823,1.,0.780158678615543));
#45035=CARTESIAN_POINT('Ctrl Pts',(3.93203552473174,1.,0.778971308134821));
#45036=CARTESIAN_POINT('Ctrl Pts',(3.93957296768103,1.,0.777741370568559));
#45037=CARTESIAN_POINT('Ctrl Pts',(3.94711101619447,1.,0.776468966697922));
#45038=CARTESIAN_POINT('Ctrl Pts',(3.9546488545231,1.,0.775154418039352));
#45039=CARTESIAN_POINT('Ctrl Pts',(3.96218649639807,1.,0.773798212026566));
#45040=CARTESIAN_POINT('Ctrl Pts',(3.96972446532772,1.,0.772400931772137));
#45041=CARTESIAN_POINT('Ctrl Pts',(3.97726349165488,1.,0.770963190030471));
#45042=CARTESIAN_POINT('Ctrl Pts',(3.98480422348451,1.,0.769485566245545));
#45043=CARTESIAN_POINT('Ctrl Pts',(3.9923468788101,1.,0.767968531377915));
#45044=CARTESIAN_POINT('Ctrl Pts',(3.99989129179622,1.,0.766412457136064));
#45045=CARTESIAN_POINT('Ctrl Pts',(4.00743706791509,1.,0.764817648785198));
#45046=CARTESIAN_POINT('Ctrl Pts',(4.01498370680496,1.,0.763184371182936));
#45047=CARTESIAN_POINT('Ctrl Pts',(4.02253072741268,1.,0.761512875859805));
#45048=CARTESIAN_POINT('Ctrl Pts',(4.03007781954412,1.,0.759803433243752));
#45049=CARTESIAN_POINT('Ctrl Pts',(4.03762485803119,1.,0.758056338884945));
#45050=CARTESIAN_POINT('Ctrl Pts',(4.04517182653997,1.,0.756271902369581));
#45051=CARTESIAN_POINT('Ctrl Pts',(4.05271876687915,1.,0.754450441816078));
#45052=CARTESIAN_POINT('Ctrl Pts',(4.06026572221515,1.,0.752592276483073));
#45053=CARTESIAN_POINT('Ctrl Pts',(4.06781267242378,1.,0.750697720484037));
#45054=CARTESIAN_POINT('Ctrl Pts',(4.07535951056152,1.,0.748767076680558));
#45055=CARTESIAN_POINT('Ctrl Pts',(4.08290608095642,1.,0.746800631492316));
#45056=CARTESIAN_POINT('Ctrl Pts',(4.09045220253573,1.,0.744798649706501));
#45057=CARTESIAN_POINT('Ctrl Pts',(4.09799769702611,1.,0.742761369689842));
#45058=CARTESIAN_POINT('Ctrl Pts',(4.10554241757547,1.,0.740688998553377));
#45059=CARTESIAN_POINT('Ctrl Pts',(4.11308626951927,1.,0.738581708225844));
#45060=CARTESIAN_POINT('Ctrl Pts',(4.120629196238,1.,0.736439634331345));
#45061=CARTESIAN_POINT('Ctrl Pts',(4.12666277570844,1.,0.734698226764093));
#45062=CARTESIAN_POINT('Ctrl Pts',(4.13118752795207,1.,0.733376589323547));
#45063=CARTESIAN_POINT('Ctrl Pts',(4.1342038373684,1.,0.73248857513516));
#45064=CARTESIAN_POINT('Ctrl Pts',(4.13571194405636,1.,0.732042837400621));
#45065=CARTESIAN_POINT('Origin',(4.13571194405636,0.,0.732042837400621));
#45066=CARTESIAN_POINT('',(4.15950947128175,1.,0.581791163835816));
#45067=CARTESIAN_POINT('Origin',(0.,0.,0.));
#45068=CARTESIAN_POINT('',(3.62400312501245,1.,0.963899035117249));
#45069=CARTESIAN_POINT('Origin',(0.,1.,0.));
#45070=CARTESIAN_POINT('Ctrl Pts',(3.62400312501245,1.,0.963899035117249));
#45071=CARTESIAN_POINT('Ctrl Pts',(3.62400312501245,0.666666666666667,0.963899035117249));
#45072=CARTESIAN_POINT('Ctrl Pts',(3.62400312501245,0.333333333333333,0.963899035117249));
#45073=CARTESIAN_POINT('Ctrl Pts',(3.62400312501245,-0.333333333333333,
0.963899035117249));
#45074=CARTESIAN_POINT('Ctrl Pts',(3.62400312501245,-0.666666666666667,
0.96389903511725));
#45075=CARTESIAN_POINT('Ctrl Pts',(3.62400312501245,-1.,0.96389903511725));
#45076=CARTESIAN_POINT('Ctrl Pts',(4.01728681790024,-1.,1.22531898815164));
#45077=CARTESIAN_POINT('Ctrl Pts',(4.01728681790024,1.,1.22531898815164));
#45078=CARTESIAN_POINT('Ctrl Pts',(4.0161454457032,-1.,1.22423716681447));
#45079=CARTESIAN_POINT('Ctrl Pts',(4.0161454457032,1.,1.22423716681447));
#45080=CARTESIAN_POINT('Ctrl Pts',(4.01386104434674,-1.,1.22207656456199));
#45081=CARTESIAN_POINT('Ctrl Pts',(4.01386104434674,1.,1.22207656456199));
#45082=CARTESIAN_POINT('Ctrl Pts',(4.01042947142681,-1.,1.21884478244983));
#45083=CARTESIAN_POINT('Ctrl Pts',(4.01042947142681,1.,1.21884478244983));
#45084=CARTESIAN_POINT('Ctrl Pts',(4.00584409524937,-1.,1.21455398918813));
#45085=CARTESIAN_POINT('Ctrl Pts',(4.00584409524937,1.,1.21455398918813));
#45086=CARTESIAN_POINT('Ctrl Pts',(4.00009577952534,-1.,1.20922097030107));
#45087=CARTESIAN_POINT('Ctrl Pts',(4.00009577952534,1.,1.20922097030107));
#45088=CARTESIAN_POINT('Ctrl Pts',(3.99433084800649,-1.,1.2039185237544));
#45089=CARTESIAN_POINT('Ctrl Pts',(3.99433084800649,1.,1.2039185237544));
#45090=CARTESIAN_POINT('Ctrl Pts',(3.98854928957287,-1.,1.19864679609596));
#45091=CARTESIAN_POINT('Ctrl Pts',(3.98854928957287,1.,1.19864679609596));
#45092=CARTESIAN_POINT('Ctrl Pts',(3.98275111052015,-1.,1.19340598349307));
#45093=CARTESIAN_POINT('Ctrl Pts',(3.98275111052015,1.,1.19340598349307));
#45094=CARTESIAN_POINT('Ctrl Pts',(3.97693634766926,-1.,1.18819633715285));
#45095=CARTESIAN_POINT('Ctrl Pts',(3.97693634766926,1.,1.18819633715285));
#45096=CARTESIAN_POINT('Ctrl Pts',(3.9711050516465,-1.,1.18301815039596));
#45097=CARTESIAN_POINT('Ctrl Pts',(3.9711050516465,1.,1.18301815039596));
#45098=CARTESIAN_POINT('Ctrl Pts',(3.96525726357682,-1.,1.17787174135446));
#45099=CARTESIAN_POINT('Ctrl Pts',(3.96525726357682,1.,1.17787174135446));
#45100=CARTESIAN_POINT('Ctrl Pts',(3.95939299213164,-1.,1.17275743590327));
#45101=CARTESIAN_POINT('Ctrl Pts',(3.95939299213164,1.,1.17275743590327));
#45102=CARTESIAN_POINT('Ctrl Pts',(3.95351219510062,-1.,1.16767555244495));
#45103=CARTESIAN_POINT('Ctrl Pts',(3.95351219510062,1.,1.16767555244495));
#45104=CARTESIAN_POINT('Ctrl Pts',(3.9476147478092,-1.,1.16262637999261));
#45105=CARTESIAN_POINT('Ctrl Pts',(3.9476147478092,1.,1.16262637999261));
#45106=CARTESIAN_POINT('Ctrl Pts',(3.94170046685542,-1.,1.15761018341061));
#45107=CARTESIAN_POINT('Ctrl Pts',(3.94170046685542,1.,1.15761018341061));
#45108=CARTESIAN_POINT('Ctrl Pts',(3.9357691705651,-1.,1.15262722716391));
#45109=CARTESIAN_POINT('Ctrl Pts',(3.9357691705651,1.,1.15262722716391));
#45110=CARTESIAN_POINT('Ctrl Pts',(3.92982073294334,-1.,1.14767779451147));
#45111=CARTESIAN_POINT('Ctrl Pts',(3.92982073294334,1.,1.14767779451147));
#45112=CARTESIAN_POINT('Ctrl Pts',(3.92385513133937,-1.,1.14276220561575));
#45113=CARTESIAN_POINT('Ctrl Pts',(3.92385513133937,1.,1.14276220561575));
#45114=CARTESIAN_POINT('Ctrl Pts',(3.91787251936688,-1.,1.13788084225511));
#45115=CARTESIAN_POINT('Ctrl Pts',(3.91787251936688,1.,1.13788084225511));
#45116=CARTESIAN_POINT('Ctrl Pts',(3.91187321145495,-1.,1.13303414693849));
#45117=CARTESIAN_POINT('Ctrl Pts',(3.91187321145495,1.,1.13303414693849));
#45118=CARTESIAN_POINT('Ctrl Pts',(3.90585753318622,-1.,1.12822258281518));
#45119=CARTESIAN_POINT('Ctrl Pts',(3.90585753318622,1.,1.12822258281518));
#45120=CARTESIAN_POINT('Ctrl Pts',(3.89982569749978,-1.,1.12344660099029));
#45121=CARTESIAN_POINT('Ctrl Pts',(3.89982569749978,1.,1.12344660099029));
#45122=CARTESIAN_POINT('Ctrl Pts',(3.89377768340362,-1.,1.11870660794609));
#45123=CARTESIAN_POINT('Ctrl Pts',(3.89377768340362,1.,1.11870660794609));
#45124=CARTESIAN_POINT('Ctrl Pts',(3.88771308285229,-1.,1.11400292434447));
#45125=CARTESIAN_POINT('Ctrl Pts',(3.88771308285229,1.,1.11400292434447));
#45126=CARTESIAN_POINT('Ctrl Pts',(3.88163105531791,-1.,1.10933577224029));
#45127=CARTESIAN_POINT('Ctrl Pts',(3.88163105531791,1.,1.10933577224029));
#45128=CARTESIAN_POINT('Ctrl Pts',(3.87553067187566,-1.,1.10470536603303));
#45129=CARTESIAN_POINT('Ctrl Pts',(3.87553067187566,1.,1.10470536603303));
#45130=CARTESIAN_POINT('Ctrl Pts',(3.86941120134872,-1.,1.10011198761203));
#45131=CARTESIAN_POINT('Ctrl Pts',(3.86941120134872,1.,1.10011198761203));
#45132=CARTESIAN_POINT('Ctrl Pts',(3.86327241021242,-1.,1.09555606505012));
#45133=CARTESIAN_POINT('Ctrl Pts',(3.86327241021242,1.,1.09555606505012));
#45134=CARTESIAN_POINT('Ctrl Pts',(3.85711487933911,-1.,1.09103825516288));
#45135=CARTESIAN_POINT('Ctrl Pts',(3.85711487933911,1.,1.09103825516288));
#45136=CARTESIAN_POINT('Ctrl Pts',(3.8509402522269,-1.,1.08655950846377));
#45137=CARTESIAN_POINT('Ctrl Pts',(3.8509402522269,1.,1.08655950846377));
#45138=CARTESIAN_POINT('Ctrl Pts',(3.84475048030615,-1.,1.08212087917986));
#45139=CARTESIAN_POINT('Ctrl Pts',(3.84475048030615,1.,1.08212087917986));
#45140=CARTESIAN_POINT('Ctrl Pts',(3.83854714117486,-1.,1.07772335353856));
#45141=CARTESIAN_POINT('Ctrl Pts',(3.83854714117486,1.,1.07772335353856));
#45142=CARTESIAN_POINT('Ctrl Pts',(3.83233071195145,-1.,1.0733676663346));
#45143=CARTESIAN_POINT('Ctrl Pts',(3.83233071195145,1.,1.0733676663346));
#45144=CARTESIAN_POINT('Ctrl Pts',(3.82609989967278,-1.,1.0690541318036));
#45145=CARTESIAN_POINT('Ctrl Pts',(3.82609989967278,1.,1.0690541318036));
#45146=CARTESIAN_POINT('Ctrl Pts',(3.81985083953012,-1.,1.06478244038931));
#45147=CARTESIAN_POINT('Ctrl Pts',(3.81985083953012,1.,1.06478244038931));
#45148=CARTESIAN_POINT('Ctrl Pts',(3.81357866117485,-1.,1.06055206187298));
#45149=CARTESIAN_POINT('Ctrl Pts',(3.81357866117485,1.,1.06055206187298));
#45150=CARTESIAN_POINT('Ctrl Pts',(3.80727913637784,-1.,1.05636266918643));
#45151=CARTESIAN_POINT('Ctrl Pts',(3.80727913637784,1.,1.05636266918643));
#45152=CARTESIAN_POINT('Ctrl Pts',(3.80095039790678,-1.,1.05221457990015));
#45153=CARTESIAN_POINT('Ctrl Pts',(3.80095039790678,1.,1.05221457990015));
#45154=CARTESIAN_POINT('Ctrl Pts',(3.79459440308793,-1.,1.04810913267641));
#45155=CARTESIAN_POINT('Ctrl Pts',(3.79459440308793,1.,1.04810913267641));
#45156=CARTESIAN_POINT('Ctrl Pts',(3.78821910787195,-1.,1.04404924374426));
#45157=CARTESIAN_POINT('Ctrl Pts',(3.78821910787195,1.,1.04404924374426));
#45158=CARTESIAN_POINT('Ctrl Pts',(3.78183535008192,-1.,1.04003862055804));
#45159=CARTESIAN_POINT('Ctrl Pts',(3.78183535008192,1.,1.04003862055804));
#45160=CARTESIAN_POINT('Ctrl Pts',(3.77545283140445,-1.,1.03608074678013));
#45161=CARTESIAN_POINT('Ctrl Pts',(3.77545283140445,1.,1.03608074678013));
#45162=CARTESIAN_POINT('Ctrl Pts',(3.76907609832522,-1.,1.0321778660492));
#45163=CARTESIAN_POINT('Ctrl Pts',(3.76907609832522,1.,1.0321778660492));
#45164=CARTESIAN_POINT('Ctrl Pts',(3.76270122291232,-1.,1.02833014458181));
#45165=CARTESIAN_POINT('Ctrl Pts',(3.76270122291232,1.,1.02833014458181));
#45166=CARTESIAN_POINT('Ctrl Pts',(3.75631037456194,-1.,1.0245342944466));
#45167=CARTESIAN_POINT('Ctrl Pts',(3.75631037456194,1.,1.0245342944466));
#45168=CARTESIAN_POINT('Ctrl Pts',(3.74987777155834,-1.,1.02078510487428));
#45169=CARTESIAN_POINT('Ctrl Pts',(3.74987777155834,1.,1.02078510487428));
#45170=CARTESIAN_POINT('Ctrl Pts',(3.74337942504959,-1.,1.01707794311079));
#45171=CARTESIAN_POINT('Ctrl Pts',(3.74337942504959,1.,1.01707794311079));
#45172=CARTESIAN_POINT('Ctrl Pts',(3.73680245055734,-1.,1.01341114319903));
#45173=CARTESIAN_POINT('Ctrl Pts',(3.73680245055734,1.,1.01341114319903));
#45174=CARTESIAN_POINT('Ctrl Pts',(3.73015276704426,-1.,1.00978798539496));
#45175=CARTESIAN_POINT('Ctrl Pts',(3.73015276704426,1.,1.00978798539496));
#45176=CARTESIAN_POINT('Ctrl Pts',(3.72346803750595,-1.,1.0062200073571));
#45177=CARTESIAN_POINT('Ctrl Pts',(3.72346803750595,1.,1.0062200073571));
#45178=CARTESIAN_POINT('Ctrl Pts',(3.71680667125118,-1.,1.00272423396822));
#45179=CARTESIAN_POINT('Ctrl Pts',(3.71680667125118,1.,1.00272423396822));
#45180=CARTESIAN_POINT('Ctrl Pts',(3.71022439713938,-1.,0.999317260756531));
#45181=CARTESIAN_POINT('Ctrl Pts',(3.71022439713938,1.,0.999317260756531));
#45182=CARTESIAN_POINT('Ctrl Pts',(3.70375282282138,-1.,0.996009819772518));
#45183=CARTESIAN_POINT('Ctrl Pts',(3.70375282282138,1.,0.996009819772518));
#45184=CARTESIAN_POINT('Ctrl Pts',(3.69738123415662,-1.,0.992802218332011));
#45185=CARTESIAN_POINT('Ctrl Pts',(3.69738123415662,1.,0.992802218332011));
#45186=CARTESIAN_POINT('Ctrl Pts',(3.69102682138846,-1.,0.989676715398559));
#45187=CARTESIAN_POINT('Ctrl Pts',(3.69102682138846,1.,0.989676715398559));
#45188=CARTESIAN_POINT('Ctrl Pts',(3.68455317926068,-1.,0.986602639863838));
#45189=CARTESIAN_POINT('Ctrl Pts',(3.68455317926068,1.,0.986602639863838));
#45190=CARTESIAN_POINT('Ctrl Pts',(3.67782408841715,-1.,0.98355079147042));
#45191=CARTESIAN_POINT('Ctrl Pts',(3.67782408841715,1.,0.98355079147042));
#45192=CARTESIAN_POINT('Ctrl Pts',(3.67074983340361,-1.,0.980505922458267));
#45193=CARTESIAN_POINT('Ctrl Pts',(3.67074983340361,1.,0.980505922458267));
#45194=CARTESIAN_POINT('Ctrl Pts',(3.66333049637475,-1.,0.977478312751618));
#45195=CARTESIAN_POINT('Ctrl Pts',(3.66333049637475,1.,0.977478312751618));
#45196=CARTESIAN_POINT('Ctrl Pts',(3.65571576735126,-1.,0.974519971354849));
#45197=CARTESIAN_POINT('Ctrl Pts',(3.65571576735126,1.,0.974519971354849));
#45198=CARTESIAN_POINT('Ctrl Pts',(3.64819756447455,-1.,0.971722122061341));
#45199=CARTESIAN_POINT('Ctrl Pts',(3.64819756447455,1.,0.971722122061341));
#45200=CARTESIAN_POINT('Ctrl Pts',(3.64113946505766,-1.,0.969195124675866));
#45201=CARTESIAN_POINT('Ctrl Pts',(3.64113946505766,1.,0.969195124675866));
#45202=CARTESIAN_POINT('Ctrl Pts',(3.63492122081143,-1.,0.967052554541386));
#45203=CARTESIAN_POINT('Ctrl Pts',(3.63492122081143,1.,0.967052554541386));
#45204=CARTESIAN_POINT('Ctrl Pts',(3.62988252139846,-1.,0.965395153165294));
#45205=CARTESIAN_POINT('Ctrl Pts',(3.62988252139846,1.,0.965395153165294));
#45206=CARTESIAN_POINT('Ctrl Pts',(3.62625391254797,-1.,0.964291001273288));
#45207=CARTESIAN_POINT('Ctrl Pts',(3.62625391254797,1.,0.964291001273288));
#45208=CARTESIAN_POINT('Ctrl Pts',(3.6245656860652,-1.,0.96387577453062));
#45209=CARTESIAN_POINT('Ctrl Pts',(3.6245656860652,1.,0.96387577453062));
#45210=CARTESIAN_POINT('Ctrl Pts',(3.62399933639914,-1.,0.963832486395052));
#45211=CARTESIAN_POINT('Ctrl Pts',(3.62399933639914,1.,0.963832486395052));
#45212=CARTESIAN_POINT('Ctrl Pts',(3.62393257642052,-1.,0.963922720982194));
#45213=CARTESIAN_POINT('Ctrl Pts',(3.62393257642052,1.,0.963922720982194));
#45214=CARTESIAN_POINT('Ctrl Pts',(3.62397690409552,-1.,0.963997613369571));
#45215=CARTESIAN_POINT('Ctrl Pts',(3.62397690409552,1.,0.963997613369571));
#45216=CARTESIAN_POINT('',(4.01728681790024,1.,1.22531898815164));
#45217=CARTESIAN_POINT('Ctrl Pts',(4.01728681790024,1.,1.22531898815164));
#45218=CARTESIAN_POINT('Ctrl Pts',(4.0161454457032,1.,1.22423716681447));
#45219=CARTESIAN_POINT('Ctrl Pts',(4.01386104434674,1.,1.22207656456199));
#45220=CARTESIAN_POINT('Ctrl Pts',(4.01042947142681,1.,1.21884478244983));
#45221=CARTESIAN_POINT('Ctrl Pts',(4.00584409524937,1.,1.21455398918813));
#45222=CARTESIAN_POINT('Ctrl Pts',(4.00009577952534,1.,1.20922097030107));
#45223=CARTESIAN_POINT('Ctrl Pts',(3.99433084800649,1.,1.2039185237544));
#45224=CARTESIAN_POINT('Ctrl Pts',(3.98854928957287,1.,1.19864679609596));
#45225=CARTESIAN_POINT('Ctrl Pts',(3.98275111052015,1.,1.19340598349307));
#45226=CARTESIAN_POINT('Ctrl Pts',(3.97693634766926,1.,1.18819633715285));
#45227=CARTESIAN_POINT('Ctrl Pts',(3.9711050516465,1.,1.18301815039596));
#45228=CARTESIAN_POINT('Ctrl Pts',(3.96525726357682,1.,1.17787174135446));
#45229=CARTESIAN_POINT('Ctrl Pts',(3.95939299213164,1.,1.17275743590327));
#45230=CARTESIAN_POINT('Ctrl Pts',(3.95351219510062,1.,1.16767555244495));
#45231=CARTESIAN_POINT('Ctrl Pts',(3.9476147478092,1.,1.16262637999261));
#45232=CARTESIAN_POINT('Ctrl Pts',(3.94170046685542,1.,1.15761018341061));
#45233=CARTESIAN_POINT('Ctrl Pts',(3.9357691705651,1.,1.15262722716391));
#45234=CARTESIAN_POINT('Ctrl Pts',(3.92982073294334,1.,1.14767779451147));
#45235=CARTESIAN_POINT('Ctrl Pts',(3.92385513133937,1.,1.14276220561575));
#45236=CARTESIAN_POINT('Ctrl Pts',(3.91787251936688,1.,1.13788084225511));
#45237=CARTESIAN_POINT('Ctrl Pts',(3.91187321145495,1.,1.13303414693849));
#45238=CARTESIAN_POINT('Ctrl Pts',(3.90585753318622,1.,1.12822258281518));
#45239=CARTESIAN_POINT('Ctrl Pts',(3.89982569749978,1.,1.12344660099029));
#45240=CARTESIAN_POINT('Ctrl Pts',(3.89377768340362,1.,1.11870660794609));
#45241=CARTESIAN_POINT('Ctrl Pts',(3.88771308285229,1.,1.11400292434447));
#45242=CARTESIAN_POINT('Ctrl Pts',(3.88163105531791,1.,1.10933577224029));
#45243=CARTESIAN_POINT('Ctrl Pts',(3.87553067187566,1.,1.10470536603303));
#45244=CARTESIAN_POINT('Ctrl Pts',(3.86941120134872,1.,1.10011198761203));
#45245=CARTESIAN_POINT('Ctrl Pts',(3.86327241021242,1.,1.09555606505012));
#45246=CARTESIAN_POINT('Ctrl Pts',(3.85711487933911,1.,1.09103825516288));
#45247=CARTESIAN_POINT('Ctrl Pts',(3.8509402522269,1.,1.08655950846377));
#45248=CARTESIAN_POINT('Ctrl Pts',(3.84475048030615,1.,1.08212087917986));
#45249=CARTESIAN_POINT('Ctrl Pts',(3.83854714117486,1.,1.07772335353856));
#45250=CARTESIAN_POINT('Ctrl Pts',(3.83233071195145,1.,1.0733676663346));
#45251=CARTESIAN_POINT('Ctrl Pts',(3.82609989967278,1.,1.0690541318036));
#45252=CARTESIAN_POINT('Ctrl Pts',(3.81985083953012,1.,1.06478244038931));
#45253=CARTESIAN_POINT('Ctrl Pts',(3.81357866117485,1.,1.06055206187298));
#45254=CARTESIAN_POINT('Ctrl Pts',(3.80727913637784,1.,1.05636266918643));
#45255=CARTESIAN_POINT('Ctrl Pts',(3.80095039790678,1.,1.05221457990015));
#45256=CARTESIAN_POINT('Ctrl Pts',(3.79459440308793,1.,1.04810913267641));
#45257=CARTESIAN_POINT('Ctrl Pts',(3.78821910787195,1.,1.04404924374426));
#45258=CARTESIAN_POINT('Ctrl Pts',(3.78183535008192,1.,1.04003862055804));
#45259=CARTESIAN_POINT('Ctrl Pts',(3.77545283140445,1.,1.03608074678013));
#45260=CARTESIAN_POINT('Ctrl Pts',(3.76907609832522,1.,1.0321778660492));
#45261=CARTESIAN_POINT('Ctrl Pts',(3.76270122291232,1.,1.02833014458181));
#45262=CARTESIAN_POINT('Ctrl Pts',(3.75631037456194,1.,1.0245342944466));
#45263=CARTESIAN_POINT('Ctrl Pts',(3.74987777155834,1.,1.02078510487428));
#45264=CARTESIAN_POINT('Ctrl Pts',(3.74337942504959,1.,1.01707794311079));
#45265=CARTESIAN_POINT('Ctrl Pts',(3.73680245055734,1.,1.01341114319903));
#45266=CARTESIAN_POINT('Ctrl Pts',(3.73015276704426,1.,1.00978798539496));
#45267=CARTESIAN_POINT('Ctrl Pts',(3.72346803750595,1.,1.0062200073571));
#45268=CARTESIAN_POINT('Ctrl Pts',(3.71680667125118,1.,1.00272423396822));
#45269=CARTESIAN_POINT('Ctrl Pts',(3.71022439713938,1.,0.999317260756531));
#45270=CARTESIAN_POINT('Ctrl Pts',(3.70375282282138,1.,0.996009819772518));
#45271=CARTESIAN_POINT('Ctrl Pts',(3.69738123415662,1.,0.992802218332011));
#45272=CARTESIAN_POINT('Ctrl Pts',(3.69102682138846,1.,0.989676715398559));
#45273=CARTESIAN_POINT('Ctrl Pts',(3.68455317926068,1.,0.986602639863838));
#45274=CARTESIAN_POINT('Ctrl Pts',(3.67782408841715,1.,0.98355079147042));
#45275=CARTESIAN_POINT('Ctrl Pts',(3.67074983340361,1.,0.980505922458267));
#45276=CARTESIAN_POINT('Ctrl Pts',(3.66333049637475,1.,0.977478312751618));
#45277=CARTESIAN_POINT('Ctrl Pts',(3.65571576735126,1.,0.974519971354849));
#45278=CARTESIAN_POINT('Ctrl Pts',(3.64819756447455,1.,0.971722122061341));
#45279=CARTESIAN_POINT('Ctrl Pts',(3.64113946505766,1.,0.969195124675866));
#45280=CARTESIAN_POINT('Ctrl Pts',(3.63492122081143,1.,0.967052554541386));
#45281=CARTESIAN_POINT('Ctrl Pts',(3.62988252139846,1.,0.965395153165294));
#45282=CARTESIAN_POINT('Ctrl Pts',(3.62652618145335,1.,0.964373850166458));
#45283=CARTESIAN_POINT('Ctrl Pts',(3.62489305727662,1.,0.963957782642844));
#45284=CARTESIAN_POINT('Ctrl Pts',(3.62424461507588,1.,0.963861297423241));
#45285=CARTESIAN_POINT('Ctrl Pts',(3.6240482887845,1.,0.963880158555582));
#45286=CARTESIAN_POINT('Ctrl Pts',(3.62400312501245,1.,0.963899035117249));
#45287=CARTESIAN_POINT('',(4.01728681790024,0.,1.22531898815164));
#45288=CARTESIAN_POINT('Ctrl Pts',(3.49848248301936,-1.,1.35022972712301));
#45289=CARTESIAN_POINT('Ctrl Pts',(3.49848248301936,1.,1.35022972712301));
#45290=CARTESIAN_POINT('Ctrl Pts',(3.4984026005375,-1.,1.35026426118402));
#45291=CARTESIAN_POINT('Ctrl Pts',(3.4984026005375,1.,1.35026426118402));
#45292=CARTESIAN_POINT('Ctrl Pts',(3.49840357193736,-1.,1.35037650303019));
#45293=CARTESIAN_POINT('Ctrl Pts',(3.49840357193736,1.,1.35037650303019));
#45294=CARTESIAN_POINT('Ctrl Pts',(3.49888720257132,-1.,1.35067437417484));
#45295=CARTESIAN_POINT('Ctrl Pts',(3.49888720257132,1.,1.35067437417484));
#45296=CARTESIAN_POINT('Ctrl Pts',(3.5004970706414,-1.,1.3513307633124));
#45297=CARTESIAN_POINT('Ctrl Pts',(3.5004970706414,1.,1.3513307633124));
#45298=CARTESIAN_POINT('Ctrl Pts',(3.50408168106261,-1.,1.35257032843486));
#45299=CARTESIAN_POINT('Ctrl Pts',(3.50408168106261,1.,1.35257032843486));
#45300=CARTESIAN_POINT('Ctrl Pts',(3.50913227059999,-1.,1.35419113575956));
#45301=CARTESIAN_POINT('Ctrl Pts',(3.50913227059999,1.,1.35419113575956));
#45302=CARTESIAN_POINT('Ctrl Pts',(3.51542230699556,-1.,1.35611275237152));
#45303=CARTESIAN_POINT('Ctrl Pts',(3.51542230699556,1.,1.35611275237152));
#45304=CARTESIAN_POINT('Ctrl Pts',(3.52261776116748,-1.,1.35821701528836));
#45305=CARTESIAN_POINT('Ctrl Pts',(3.52261776116748,1.,1.35821701528836));
#45306=CARTESIAN_POINT('Ctrl Pts',(3.530344649616,-1.,1.36037259643734));
#45307=CARTESIAN_POINT('Ctrl Pts',(3.530344649616,1.,1.36037259643734));
#45308=CARTESIAN_POINT('Ctrl Pts',(3.53824396424961,-1.,1.36245507339307));
#45309=CARTESIAN_POINT('Ctrl Pts',(3.53824396424961,1.,1.36245507339307));
#45310=CARTESIAN_POINT('Ctrl Pts',(3.54602591832973,-1.,1.36436666257598));
#45311=CARTESIAN_POINT('Ctrl Pts',(3.54602591832973,1.,1.36436666257598));
#45312=CARTESIAN_POINT('Ctrl Pts',(3.55353883995949,-1.,1.3660614545677));
#45313=CARTESIAN_POINT('Ctrl Pts',(3.55353883995949,1.,1.3660614545677));
#45314=CARTESIAN_POINT('Ctrl Pts',(3.56077662028649,-1.,1.36754771771233));
#45315=CARTESIAN_POINT('Ctrl Pts',(3.56077662028649,1.,1.36754771771233));
#45316=CARTESIAN_POINT('Ctrl Pts',(3.5678208030466,-1.,1.36886584973389));
#45317=CARTESIAN_POINT('Ctrl Pts',(3.5678208030466,1.,1.36886584973389));
#45318=CARTESIAN_POINT('Ctrl Pts',(3.57479875549486,-1.,1.37007229485659));
#45319=CARTESIAN_POINT('Ctrl Pts',(3.57479875549486,1.,1.37007229485659));
#45320=CARTESIAN_POINT('Ctrl Pts',(3.58183885982715,-1.,1.37122241663062));
#45321=CARTESIAN_POINT('Ctrl Pts',(3.58183885982715,1.,1.37122241663062));
#45322=CARTESIAN_POINT('Ctrl Pts',(3.58901853846365,-1.,1.37235053660976));
#45323=CARTESIAN_POINT('Ctrl Pts',(3.58901853846365,1.,1.37235053660976));
#45324=CARTESIAN_POINT('Ctrl Pts',(3.59634627869048,-1.,1.37346320103157));
#45325=CARTESIAN_POINT('Ctrl Pts',(3.59634627869048,1.,1.37346320103157));
#45326=CARTESIAN_POINT('Ctrl Pts',(3.60379020123988,-1.,1.37455051379623));
#45327=CARTESIAN_POINT('Ctrl Pts',(3.60379020123988,1.,1.37455051379623));
#45328=CARTESIAN_POINT('Ctrl Pts',(3.61129546591064,-1.,1.37559314436634));
#45329=CARTESIAN_POINT('Ctrl Pts',(3.61129546591064,1.,1.37559314436634));
#45330=CARTESIAN_POINT('Ctrl Pts',(3.6188048116042,-1.,1.37657053403107));
#45331=CARTESIAN_POINT('Ctrl Pts',(3.6188048116042,1.,1.37657053403107));
#45332=CARTESIAN_POINT('Ctrl Pts',(3.62628098665145,-1.,1.37746987919881));
#45333=CARTESIAN_POINT('Ctrl Pts',(3.62628098665145,1.,1.37746987919881));
#45334=CARTESIAN_POINT('Ctrl Pts',(3.63371727442486,-1.,1.37829035457339));
#45335=CARTESIAN_POINT('Ctrl Pts',(3.63371727442486,1.,1.37829035457339));
#45336=CARTESIAN_POINT('Ctrl Pts',(3.64112507791141,-1.,1.37903818567359));
#45337=CARTESIAN_POINT('Ctrl Pts',(3.64112507791141,1.,1.37903818567359));
#45338=CARTESIAN_POINT('Ctrl Pts',(3.64852652756456,-1.,1.37972372481603));
#45339=CARTESIAN_POINT('Ctrl Pts',(3.64852652756456,1.,1.37972372481603));
#45340=CARTESIAN_POINT('Ctrl Pts',(3.6559455440439,-1.,1.38035791051213));
#45341=CARTESIAN_POINT('Ctrl Pts',(3.6559455440439,1.,1.38035791051213));
#45342=CARTESIAN_POINT('Ctrl Pts',(3.66339848520857,-1.,1.38094856333552));
#45343=CARTESIAN_POINT('Ctrl Pts',(3.66339848520857,1.,1.38094856333552));
#45344=CARTESIAN_POINT('Ctrl Pts',(3.67088843112262,-1.,1.38149812653868));
#45345=CARTESIAN_POINT('Ctrl Pts',(3.67088843112262,1.,1.38149812653868));
#45346=CARTESIAN_POINT('Ctrl Pts',(3.67841038482414,-1.,1.3820057429062));
#45347=CARTESIAN_POINT('Ctrl Pts',(3.67841038482414,1.,1.3820057429062));
#45348=CARTESIAN_POINT('Ctrl Pts',(3.68595444983837,-1.,1.38246852827182));
#45349=CARTESIAN_POINT('Ctrl Pts',(3.68595444983837,1.,1.38246852827182));
#45350=CARTESIAN_POINT('Ctrl Pts',(3.69350967899526,-1.,1.38288311171651));
#45351=CARTESIAN_POINT('Ctrl Pts',(3.69350967899526,1.,1.38288311171651));
#45352=CARTESIAN_POINT('Ctrl Pts',(3.701067921679,-1.,1.38324717612865));
#45353=CARTESIAN_POINT('Ctrl Pts',(3.701067921679,1.,1.38324717612865));
#45354=CARTESIAN_POINT('Ctrl Pts',(3.70862680753347,-1.,1.38356065402124));
#45355=CARTESIAN_POINT('Ctrl Pts',(3.70862680753347,1.,1.38356065402124));
#45356=CARTESIAN_POINT('Ctrl Pts',(3.7161876605181,-1.,1.38382489984586));
#45357=CARTESIAN_POINT('Ctrl Pts',(3.7161876605181,1.,1.38382489984586));
#45358=CARTESIAN_POINT('Ctrl Pts',(3.72375409358803,-1.,1.3840421342895));
#45359=CARTESIAN_POINT('Ctrl Pts',(3.72375409358803,1.,1.3840421342895));
#45360=CARTESIAN_POINT('Ctrl Pts',(3.73133035859282,-1.,1.38421479111531));
#45361=CARTESIAN_POINT('Ctrl Pts',(3.73133035859282,1.,1.38421479111531));
#45362=CARTESIAN_POINT('Ctrl Pts',(3.73891976418104,-1.,1.38434489156458));
#45363=CARTESIAN_POINT('Ctrl Pts',(3.73891976418104,1.,1.38434489156458));
#45364=CARTESIAN_POINT('Ctrl Pts',(3.74652317167876,-1.,1.38443344984394));
#45365=CARTESIAN_POINT('Ctrl Pts',(3.74652317167876,1.,1.38443344984394));
#45366=CARTESIAN_POINT('Ctrl Pts',(3.7541397631875,-1.,1.38448077997163));
#45367=CARTESIAN_POINT('Ctrl Pts',(3.7541397631875,1.,1.38448077997163));
#45368=CARTESIAN_POINT('Ctrl Pts',(3.76176768271367,-1.,1.3844867525335));
#45369=CARTESIAN_POINT('Ctrl Pts',(3.76176768271367,1.,1.3844867525335));
#45370=CARTESIAN_POINT('Ctrl Pts',(3.76940473185779,-1.,1.38445107339518));
#45371=CARTESIAN_POINT('Ctrl Pts',(3.76940473185779,1.,1.38445107339518));
#45372=CARTESIAN_POINT('Ctrl Pts',(3.77704902230418,-1.,1.38437354551428));
#45373=CARTESIAN_POINT('Ctrl Pts',(3.77704902230418,1.,1.38437354551428));
#45374=CARTESIAN_POINT('Ctrl Pts',(3.78469969805082,-1.,1.38425435883756));
#45375=CARTESIAN_POINT('Ctrl Pts',(3.78469969805082,1.,1.38425435883756));
#45376=CARTESIAN_POINT('Ctrl Pts',(3.79235669640841,-1.,1.38409399694566));
#45377=CARTESIAN_POINT('Ctrl Pts',(3.79235669640841,1.,1.38409399694566));
#45378=CARTESIAN_POINT('Ctrl Pts',(3.80002044322111,-1.,1.38389311766682));
#45379=CARTESIAN_POINT('Ctrl Pts',(3.80002044322111,1.,1.38389311766682));
#45380=CARTESIAN_POINT('Ctrl Pts',(3.80769156398411,-1.,1.3836524404622));
#45381=CARTESIAN_POINT('Ctrl Pts',(3.80769156398411,1.,1.3836524404622));
#45382=CARTESIAN_POINT('Ctrl Pts',(3.81537060817811,-1.,1.38337263902782));
#45383=CARTESIAN_POINT('Ctrl Pts',(3.81537060817811,1.,1.38337263902782));
#45384=CARTESIAN_POINT('Ctrl Pts',(3.82305771743829,-1.,1.38305421262763));
#45385=CARTESIAN_POINT('Ctrl Pts',(3.82305771743829,1.,1.38305421262763));
#45386=CARTESIAN_POINT('Ctrl Pts',(3.8307526698229,-1.,1.38269750245138));
#45387=CARTESIAN_POINT('Ctrl Pts',(3.8307526698229,1.,1.38269750245138));
#45388=CARTESIAN_POINT('Ctrl Pts',(3.83845502790746,-1.,1.38230274828822));
#45389=CARTESIAN_POINT('Ctrl Pts',(3.83845502790746,1.,1.38230274828822));
#45390=CARTESIAN_POINT('Ctrl Pts',(3.84616425605764,-1.,1.38187013346109));
#45391=CARTESIAN_POINT('Ctrl Pts',(3.84616425605764,1.,1.38187013346109));
#45392=CARTESIAN_POINT('Ctrl Pts',(3.85387983979481,-1.,1.3813998311505));
#45393=CARTESIAN_POINT('Ctrl Pts',(3.85387983979481,1.,1.3813998311505));
#45394=CARTESIAN_POINT('Ctrl Pts',(3.86160143043959,-1.,1.3808920599299));
#45395=CARTESIAN_POINT('Ctrl Pts',(3.86160143043959,1.,1.3808920599299));
#45396=CARTESIAN_POINT('Ctrl Pts',(3.86932885813068,-1.,1.38034709213014));
#45397=CARTESIAN_POINT('Ctrl Pts',(3.86932885813068,1.,1.38034709213014));
#45398=CARTESIAN_POINT('Ctrl Pts',(3.87706205830532,-1.,1.37976523097073));
#45399=CARTESIAN_POINT('Ctrl Pts',(3.87706205830532,1.,1.37976523097073));
#45400=CARTESIAN_POINT('Ctrl Pts',(3.88480102249277,-1.,1.37914679719383));
#45401=CARTESIAN_POINT('Ctrl Pts',(3.88480102249277,1.,1.37914679719383));
#45402=CARTESIAN_POINT('Ctrl Pts',(3.89254574338496,-1.,1.3784921128802));
#45403=CARTESIAN_POINT('Ctrl Pts',(3.89254574338496,1.,1.3784921128802));
#45404=CARTESIAN_POINT('Ctrl Pts',(3.90029615196727,-1.,1.37780148512792));
#45405=CARTESIAN_POINT('Ctrl Pts',(3.90029615196727,1.,1.37780148512792));
#45406=CARTESIAN_POINT('Ctrl Pts',(3.90805209523486,-1.,1.3770751963402));
#45407=CARTESIAN_POINT('Ctrl Pts',(3.90805209523486,1.,1.3770751963402));
#45408=CARTESIAN_POINT('Ctrl Pts',(3.91581337462644,-1.,1.37631350505797));
#45409=CARTESIAN_POINT('Ctrl Pts',(3.91581337462644,1.,1.37631350505797));
#45410=CARTESIAN_POINT('Ctrl Pts',(3.92357976987672,-1.,1.37551664448242));
#45411=CARTESIAN_POINT('Ctrl Pts',(3.92357976987672,1.,1.37551664448242));
#45412=CARTESIAN_POINT('Ctrl Pts',(3.93135106761844,-1.,1.37468482215751));
#45413=CARTESIAN_POINT('Ctrl Pts',(3.93135106761844,1.,1.37468482215751));
#45414=CARTESIAN_POINT('Ctrl Pts',(3.93912709040818,-1.,1.37381821967165));
#45415=CARTESIAN_POINT('Ctrl Pts',(3.93912709040818,1.,1.37381821967165));
#45416=CARTESIAN_POINT('Ctrl Pts',(3.94690771785133,-1.,1.37291699202807));
#45417=CARTESIAN_POINT('Ctrl Pts',(3.94690771785133,1.,1.37291699202807));
#45418=CARTESIAN_POINT('Ctrl Pts',(3.95469287280914,-1.,1.37198126432386));
#45419=CARTESIAN_POINT('Ctrl Pts',(3.95469287280914,1.,1.37198126432386));
#45420=CARTESIAN_POINT('Ctrl Pts',(3.96092458506535,-1.,1.3712051561502));
#45421=CARTESIAN_POINT('Ctrl Pts',(3.96092458506535,1.,1.3712051561502));
#45422=CARTESIAN_POINT('Ctrl Pts',(3.96560037974645,-1.,1.37060761745635));
#45423=CARTESIAN_POINT('Ctrl Pts',(3.96560037974645,1.,1.37060761745635));
#45424=CARTESIAN_POINT('Ctrl Pts',(3.9687184694131,-1.,1.37020239094614));
#45425=CARTESIAN_POINT('Ctrl Pts',(3.9687184694131,1.,1.37020239094614));
#45426=CARTESIAN_POINT('Ctrl Pts',(3.97027773754922,-1.,1.36999806084573));
#45427=CARTESIAN_POINT('Ctrl Pts',(3.97027773754922,1.,1.36999806084573));
#45428=CARTESIAN_POINT('',(3.4984457533445,1.,1.35032489087101));
#45429=CARTESIAN_POINT('Ctrl Pts',(3.4984457533445,-1.,1.35032489087101));
#45430=CARTESIAN_POINT('Ctrl Pts',(3.4984457533445,-0.666666666666667,1.35032489087101));
#45431=CARTESIAN_POINT('Ctrl Pts',(3.4984457533445,-0.333333333333333,1.35032489087101));
#45432=CARTESIAN_POINT('Ctrl Pts',(3.4984457533445,0.333333333333333,1.35032489087101));
#45433=CARTESIAN_POINT('Ctrl Pts',(3.4984457533445,0.666666666666667,1.35032489087101));
#45434=CARTESIAN_POINT('Ctrl Pts',(3.4984457533445,1.,1.35032489087101));
#45435=CARTESIAN_POINT('',(3.97027773754922,1.,1.36999806084573));
#45436=CARTESIAN_POINT('',(3.97027773754922,0.,1.36999806084573));
#45437=CARTESIAN_POINT('Ctrl Pts',(3.4984457533445,1.,1.35032489087101));
#45438=CARTESIAN_POINT('Ctrl Pts',(3.49847119623846,1.,1.35036670892966));
#45439=CARTESIAN_POINT('Ctrl Pts',(3.49861894124827,1.,1.35049736560527));
#45440=CARTESIAN_POINT('Ctrl Pts',(3.49920025459723,1.,1.35080045218587));
#45441=CARTESIAN_POINT('Ctrl Pts',(3.5007660381649,1.,1.35142377279517));
#45442=CARTESIAN_POINT('Ctrl Pts',(3.50408168106261,1.,1.35257032843486));
#45443=CARTESIAN_POINT('Ctrl Pts',(3.50913227059999,1.,1.35419113575956));
#45444=CARTESIAN_POINT('Ctrl Pts',(3.51542230699556,1.,1.35611275237152));
#45445=CARTESIAN_POINT('Ctrl Pts',(3.52261776116748,1.,1.35821701528836));
#45446=CARTESIAN_POINT('Ctrl Pts',(3.530344649616,1.,1.36037259643734));
#45447=CARTESIAN_POINT('Ctrl Pts',(3.53824396424961,1.,1.36245507339307));
#45448=CARTESIAN_POINT('Ctrl Pts',(3.54602591832973,1.,1.36436666257598));
#45449=CARTESIAN_POINT('Ctrl Pts',(3.55353883995949,1.,1.3660614545677));
#45450=CARTESIAN_POINT('Ctrl Pts',(3.56077662028649,1.,1.36754771771233));
#45451=CARTESIAN_POINT('Ctrl Pts',(3.5678208030466,1.,1.36886584973389));
#45452=CARTESIAN_POINT('Ctrl Pts',(3.57479875549486,1.,1.37007229485659));
#45453=CARTESIAN_POINT('Ctrl Pts',(3.58183885982715,1.,1.37122241663062));
#45454=CARTESIAN_POINT('Ctrl Pts',(3.58901853846365,1.,1.37235053660976));
#45455=CARTESIAN_POINT('Ctrl Pts',(3.59634627869048,1.,1.37346320103157));
#45456=CARTESIAN_POINT('Ctrl Pts',(3.60379020123988,1.,1.37455051379623));
#45457=CARTESIAN_POINT('Ctrl Pts',(3.61129546591064,1.,1.37559314436634));
#45458=CARTESIAN_POINT('Ctrl Pts',(3.6188048116042,1.,1.37657053403107));
#45459=CARTESIAN_POINT('Ctrl Pts',(3.62628098665145,1.,1.37746987919881));
#45460=CARTESIAN_POINT('Ctrl Pts',(3.63371727442486,1.,1.37829035457339));
#45461=CARTESIAN_POINT('Ctrl Pts',(3.64112507791141,1.,1.37903818567359));
#45462=CARTESIAN_POINT('Ctrl Pts',(3.64852652756456,1.,1.37972372481603));
#45463=CARTESIAN_POINT('Ctrl Pts',(3.6559455440439,1.,1.38035791051213));
#45464=CARTESIAN_POINT('Ctrl Pts',(3.66339848520857,1.,1.38094856333552));
#45465=CARTESIAN_POINT('Ctrl Pts',(3.67088843112262,1.,1.38149812653868));
#45466=CARTESIAN_POINT('Ctrl Pts',(3.67841038482414,1.,1.3820057429062));
#45467=CARTESIAN_POINT('Ctrl Pts',(3.68595444983837,1.,1.38246852827182));
#45468=CARTESIAN_POINT('Ctrl Pts',(3.69350967899526,1.,1.38288311171651));
#45469=CARTESIAN_POINT('Ctrl Pts',(3.701067921679,1.,1.38324717612865));
#45470=CARTESIAN_POINT('Ctrl Pts',(3.70862680753347,1.,1.38356065402124));
#45471=CARTESIAN_POINT('Ctrl Pts',(3.7161876605181,1.,1.38382489984586));
#45472=CARTESIAN_POINT('Ctrl Pts',(3.72375409358803,1.,1.3840421342895));
#45473=CARTESIAN_POINT('Ctrl Pts',(3.73133035859282,1.,1.38421479111531));
#45474=CARTESIAN_POINT('Ctrl Pts',(3.73891976418104,1.,1.38434489156458));
#45475=CARTESIAN_POINT('Ctrl Pts',(3.74652317167876,1.,1.38443344984394));
#45476=CARTESIAN_POINT('Ctrl Pts',(3.7541397631875,1.,1.38448077997163));
#45477=CARTESIAN_POINT('Ctrl Pts',(3.76176768271367,1.,1.3844867525335));
#45478=CARTESIAN_POINT('Ctrl Pts',(3.76940473185779,1.,1.38445107339518));
#45479=CARTESIAN_POINT('Ctrl Pts',(3.77704902230418,1.,1.38437354551428));
#45480=CARTESIAN_POINT('Ctrl Pts',(3.78469969805082,1.,1.38425435883756));
#45481=CARTESIAN_POINT('Ctrl Pts',(3.79235669640841,1.,1.38409399694566));
#45482=CARTESIAN_POINT('Ctrl Pts',(3.80002044322111,1.,1.38389311766682));
#45483=CARTESIAN_POINT('Ctrl Pts',(3.80769156398411,1.,1.3836524404622));
#45484=CARTESIAN_POINT('Ctrl Pts',(3.81537060817811,1.,1.38337263902782));
#45485=CARTESIAN_POINT('Ctrl Pts',(3.82305771743829,1.,1.38305421262763));
#45486=CARTESIAN_POINT('Ctrl Pts',(3.8307526698229,1.,1.38269750245138));
#45487=CARTESIAN_POINT('Ctrl Pts',(3.83845502790746,1.,1.38230274828822));
#45488=CARTESIAN_POINT('Ctrl Pts',(3.84616425605764,1.,1.38187013346109));
#45489=CARTESIAN_POINT('Ctrl Pts',(3.85387983979481,1.,1.3813998311505));
#45490=CARTESIAN_POINT('Ctrl Pts',(3.86160143043959,1.,1.3808920599299));
#45491=CARTESIAN_POINT('Ctrl Pts',(3.86932885813068,1.,1.38034709213014));
#45492=CARTESIAN_POINT('Ctrl Pts',(3.87706205830532,1.,1.37976523097073));
#45493=CARTESIAN_POINT('Ctrl Pts',(3.88480102249277,1.,1.37914679719383));
#45494=CARTESIAN_POINT('Ctrl Pts',(3.89254574338496,1.,1.3784921128802));
#45495=CARTESIAN_POINT('Ctrl Pts',(3.90029615196727,1.,1.37780148512792));
#45496=CARTESIAN_POINT('Ctrl Pts',(3.90805209523486,1.,1.3770751963402));
#45497=CARTESIAN_POINT('Ctrl Pts',(3.91581337462644,1.,1.37631350505797));
#45498=CARTESIAN_POINT('Ctrl Pts',(3.92357976987672,1.,1.37551664448242));
#45499=CARTESIAN_POINT('Ctrl Pts',(3.93135106761844,1.,1.37468482215751));
#45500=CARTESIAN_POINT('Ctrl Pts',(3.93912709040818,1.,1.37381821967165));
#45501=CARTESIAN_POINT('Ctrl Pts',(3.94690771785133,1.,1.37291699202807));
#45502=CARTESIAN_POINT('Ctrl Pts',(3.95469287280914,1.,1.37198126432386));
#45503=CARTESIAN_POINT('Ctrl Pts',(3.96092458506535,1.,1.3712051561502));
#45504=CARTESIAN_POINT('Ctrl Pts',(3.96560037974645,1.,1.37060761745635));
#45505=CARTESIAN_POINT('Ctrl Pts',(3.9687184694131,1.,1.37020239094614));
#45506=CARTESIAN_POINT('Ctrl Pts',(3.97027773754922,1.,1.36999806084573));
#45507=CARTESIAN_POINT('Origin',(3.97027773754922,0.,1.36999806084573));
#45508=CARTESIAN_POINT('',(4.01728681790024,1.,1.22531898815164));
#45509=CARTESIAN_POINT('Origin',(0.,0.,0.));
#45510=CARTESIAN_POINT('',(3.42859860294378,1.,1.51895082866166));
#45511=CARTESIAN_POINT('Origin',(0.,1.,0.));
#45512=CARTESIAN_POINT('Ctrl Pts',(3.42859860294378,1.,1.51895082866166));
#45513=CARTESIAN_POINT('Ctrl Pts',(3.42859860294378,0.666666666666667,1.51895082866166));
#45514=CARTESIAN_POINT('Ctrl Pts',(3.42859860294378,0.333333333333333,1.51895082866166));
#45515=CARTESIAN_POINT('Ctrl Pts',(3.42859860294378,-0.333333333333333,
1.51895082866166));
#45516=CARTESIAN_POINT('Ctrl Pts',(3.42859860294378,-0.666666666666667,
1.51895082866166));
#45517=CARTESIAN_POINT('Ctrl Pts',(3.42859860294378,-1.,1.51895082866166));
#45518=CARTESIAN_POINT('Ctrl Pts',(3.77614523045147,-1.,1.83867539237861));
#45519=CARTESIAN_POINT('Ctrl Pts',(3.77614523045147,1.,1.83867539237861));
#45520=CARTESIAN_POINT('Ctrl Pts',(3.77518714458232,-1.,1.83742834010821));
#45521=CARTESIAN_POINT('Ctrl Pts',(3.77518714458232,1.,1.83742834010821));
#45522=CARTESIAN_POINT('Ctrl Pts',(3.77326886065484,-1.,1.83493697935064));
#45523=CARTESIAN_POINT('Ctrl Pts',(3.77326886065484,1.,1.83493697935064));
#45524=CARTESIAN_POINT('Ctrl Pts',(3.77038509819777,-1.,1.83120816956515));
#45525=CARTESIAN_POINT('Ctrl Pts',(3.77038509819777,1.,1.83120816956515));
#45526=CARTESIAN_POINT('Ctrl Pts',(3.76652740355856,-1.,1.82625289221933));
#45527=CARTESIAN_POINT('Ctrl Pts',(3.76652740355856,1.,1.82625289221933));
#45528=CARTESIAN_POINT('Ctrl Pts',(3.76168412709652,-1.,1.82008629694924));
#45529=CARTESIAN_POINT('Ctrl Pts',(3.76168412709652,1.,1.82008629694924));
#45530=CARTESIAN_POINT('Ctrl Pts',(3.75681965683995,-1.,1.81394729834032));
#45531=CARTESIAN_POINT('Ctrl Pts',(3.75681965683995,1.,1.81394729834032));
#45532=CARTESIAN_POINT('Ctrl Pts',(3.75193395888069,-1.,1.80783603939662));
#45533=CARTESIAN_POINT('Ctrl Pts',(3.75193395888069,1.,1.80783603939662));
#45534=CARTESIAN_POINT('Ctrl Pts',(3.74702700874954,-1.,1.80175271485519));
#45535=CARTESIAN_POINT('Ctrl Pts',(3.74702700874954,1.,1.80175271485519));
#45536=CARTESIAN_POINT('Ctrl Pts',(3.74209880351667,-1.,1.79569757859041));
#45537=CARTESIAN_POINT('Ctrl Pts',(3.74209880351667,1.,1.79569757859041));
#45538=CARTESIAN_POINT('Ctrl Pts',(3.73714934729962,-1.,1.78967092823139));
#45539=CARTESIAN_POINT('Ctrl Pts',(3.73714934729962,1.,1.78967092823139));
#45540=CARTESIAN_POINT('Ctrl Pts',(3.73217863095022,-1.,1.78367308442682));
#45541=CARTESIAN_POINT('Ctrl Pts',(3.73217863095022,1.,1.78367308442682));
#45542=CARTESIAN_POINT('Ctrl Pts',(3.72718661205504,-1.,1.77770437039606));
#45543=CARTESIAN_POINT('Ctrl Pts',(3.72718661205504,1.,1.77770437039606));
#45544=CARTESIAN_POINT('Ctrl Pts',(3.72217319911429,-1.,1.77176509401846));
#45545=CARTESIAN_POINT('Ctrl Pts',(3.72217319911429,1.,1.77176509401846));
#45546=CARTESIAN_POINT('Ctrl Pts',(3.71713822377675,-1.,1.76585552124549));
#45547=CARTESIAN_POINT('Ctrl Pts',(3.71713822377675,1.,1.76585552124549));
#45548=CARTESIAN_POINT('Ctrl Pts',(3.71208146346454,-1.,1.75997588499021));
#45549=CARTESIAN_POINT('Ctrl Pts',(3.71208146346454,1.,1.75997588499021));
#45550=CARTESIAN_POINT('Ctrl Pts',(3.70700269736876,-1.,1.75412641804148));
#45551=CARTESIAN_POINT('Ctrl Pts',(3.70700269736876,1.,1.75412641804148));
#45552=CARTESIAN_POINT('Ctrl Pts',(3.70190175673422,-1.,1.74830738046092));
#45553=CARTESIAN_POINT('Ctrl Pts',(3.70190175673422,1.,1.74830738046092));
#45554=CARTESIAN_POINT('Ctrl Pts',(3.6967785691046,-1.,1.74251908492589));
#45555=CARTESIAN_POINT('Ctrl Pts',(3.6967785691046,1.,1.74251908492589));
#45556=CARTESIAN_POINT('Ctrl Pts',(3.69163322647906,-1.,1.73676193254493));
#45557=CARTESIAN_POINT('Ctrl Pts',(3.69163322647906,1.,1.73676193254493));
#45558=CARTESIAN_POINT('Ctrl Pts',(3.68646597019188,-1.,1.73103640956647));
#45559=CARTESIAN_POINT('Ctrl Pts',(3.68646597019188,1.,1.73103640956647));
#45560=CARTESIAN_POINT('Ctrl Pts',(3.68127704936472,-1.,1.72534302437003));
#45561=CARTESIAN_POINT('Ctrl Pts',(3.68127704936472,1.,1.72534302437003));
#45562=CARTESIAN_POINT('Ctrl Pts',(3.67606660374665,-1.,1.71968225581787));
#45563=CARTESIAN_POINT('Ctrl Pts',(3.67606660374665,1.,1.71968225581787));
#45564=CARTESIAN_POINT('Ctrl Pts',(3.67083454901629,-1.,1.71405450210392));
#45565=CARTESIAN_POINT('Ctrl Pts',(3.67083454901629,1.,1.71405450210392));
#45566=CARTESIAN_POINT('Ctrl Pts',(3.6655804319893,-1.,1.70846001610983));
#45567=CARTESIAN_POINT('Ctrl Pts',(3.6655804319893,1.,1.70846001610983));
#45568=CARTESIAN_POINT('Ctrl Pts',(3.6603033877491,-1.,1.70289888566904));
#45569=CARTESIAN_POINT('Ctrl Pts',(3.6603033877491,1.,1.70289888566904));
#45570=CARTESIAN_POINT('Ctrl Pts',(3.65500246526798,-1.,1.69737117722559));
#45571=CARTESIAN_POINT('Ctrl Pts',(3.65500246526798,1.,1.69737117722559));
#45572=CARTESIAN_POINT('Ctrl Pts',(3.64967689827393,-1.,1.691877054817));
#45573=CARTESIAN_POINT('Ctrl Pts',(3.64967689827393,1.,1.691877054817));
#45574=CARTESIAN_POINT('Ctrl Pts',(3.64432638915199,-1.,1.68641690471455));
#45575=CARTESIAN_POINT('Ctrl Pts',(3.64432638915199,1.,1.68641690471455));
#45576=CARTESIAN_POINT('Ctrl Pts',(3.63895140887443,-1.,1.68099146651577));
#45577=CARTESIAN_POINT('Ctrl Pts',(3.63895140887443,1.,1.68099146651577));
#45578=CARTESIAN_POINT('Ctrl Pts',(3.63355343201211,-1.,1.67560193613145));
#45579=CARTESIAN_POINT('Ctrl Pts',(3.63355343201211,1.,1.67560193613145));
#45580=CARTESIAN_POINT('Ctrl Pts',(3.62813422105257,-1.,1.67024966008037));
#45581=CARTESIAN_POINT('Ctrl Pts',(3.62813422105257,1.,1.67024966008037));
#45582=CARTESIAN_POINT('Ctrl Pts',(3.62269517989104,-1.,1.66493585923853));
#45583=CARTESIAN_POINT('Ctrl Pts',(3.62269517989104,1.,1.66493585923853));
#45584=CARTESIAN_POINT('Ctrl Pts',(3.61723666482457,-1.,1.65966133399186));
#45585=CARTESIAN_POINT('Ctrl Pts',(3.61723666482457,1.,1.65966133399186));
#45586=CARTESIAN_POINT('Ctrl Pts',(3.61175734965129,-1.,1.65442619244327));
#45587=CARTESIAN_POINT('Ctrl Pts',(3.61175734965129,1.,1.65442619244327));
#45588=CARTESIAN_POINT('Ctrl Pts',(3.60625346556992,-1.,1.64922952425833));
#45589=CARTESIAN_POINT('Ctrl Pts',(3.60625346556992,1.,1.64922952425833));
#45590=CARTESIAN_POINT('Ctrl Pts',(3.6007202851384,-1.,1.6440700438558));
#45591=CARTESIAN_POINT('Ctrl Pts',(3.6007202851384,1.,1.6440700438558));
#45592=CARTESIAN_POINT('Ctrl Pts',(3.59515368334887,-1.,1.63894676675349));
#45593=CARTESIAN_POINT('Ctrl Pts',(3.59515368334887,1.,1.63894676675349));
#45594=CARTESIAN_POINT('Ctrl Pts',(3.58955176627876,-1.,1.63385971451259));
#45595=CARTESIAN_POINT('Ctrl Pts',(3.58955176627876,1.,1.63385971451259));
#45596=CARTESIAN_POINT('Ctrl Pts',(3.5839162577435,-1.,1.62881051550748));
#45597=CARTESIAN_POINT('Ctrl Pts',(3.5839162577435,1.,1.62881051550748));
#45598=CARTESIAN_POINT('Ctrl Pts',(3.57825455954405,-1.,1.62380329464851));
#45599=CARTESIAN_POINT('Ctrl Pts',(3.57825455954405,1.,1.62380329464851));
#45600=CARTESIAN_POINT('Ctrl Pts',(3.57257679609826,-1.,1.61884340915412));
#45601=CARTESIAN_POINT('Ctrl Pts',(3.57257679609826,1.,1.61884340915412));
#45602=CARTESIAN_POINT('Ctrl Pts',(3.56689200468404,-1.,1.61393581747522));
#45603=CARTESIAN_POINT('Ctrl Pts',(3.56689200468404,1.,1.61393581747522));
#45604=CARTESIAN_POINT('Ctrl Pts',(3.56120432482986,-1.,1.60908344685459));
#45605=CARTESIAN_POINT('Ctrl Pts',(3.56120432482986,1.,1.60908344685459));
#45606=CARTESIAN_POINT('Ctrl Pts',(3.55550985096117,-1.,1.60428584699848));
#45607=CARTESIAN_POINT('Ctrl Pts',(3.55550985096117,1.,1.60428584699848));
#45608=CARTESIAN_POINT('Ctrl Pts',(3.54979148634426,-1.,1.59953698113444));
#45609=CARTESIAN_POINT('Ctrl Pts',(3.54979148634426,1.,1.59953698113444));
#45610=CARTESIAN_POINT('Ctrl Pts',(3.544024581823,-1.,1.5948276694975));
#45611=CARTESIAN_POINT('Ctrl Pts',(3.544024581823,1.,1.5948276694975));
#45612=CARTESIAN_POINT('Ctrl Pts',(3.53818616861045,-1.,1.59014958368725));
#45613=CARTESIAN_POINT('Ctrl Pts',(3.53818616861045,1.,1.59014958368725));
#45614=CARTESIAN_POINT('Ctrl Pts',(3.53226378147068,-1.,1.58549906268083));
#45615=CARTESIAN_POINT('Ctrl Pts',(3.53226378147068,1.,1.58549906268083));
#45616=CARTESIAN_POINT('Ctrl Pts',(3.52626275334899,-1.,1.58088027227856));
#45617=CARTESIAN_POINT('Ctrl Pts',(3.52626275334899,1.,1.58088027227856));
#45618=CARTESIAN_POINT('Ctrl Pts',(3.52021847865961,-1.,1.5763104998818));
#45619=CARTESIAN_POINT('Ctrl Pts',(3.52021847865961,1.,1.5763104998818));
#45620=CARTESIAN_POINT('Ctrl Pts',(3.51418598431733,-1.,1.57181569799774));
#45621=CARTESIAN_POINT('Ctrl Pts',(3.51418598431733,1.,1.57181569799774));
#45622=CARTESIAN_POINT('Ctrl Pts',(3.50821771695427,-1.,1.56742097575041));
#45623=CARTESIAN_POINT('Ctrl Pts',(3.50821771695427,1.,1.56742097575041));
#45624=CARTESIAN_POINT('Ctrl Pts',(3.50234321621607,-1.,1.56314187758689));
#45625=CARTESIAN_POINT('Ctrl Pts',(3.50234321621607,1.,1.56314187758689));
#45626=CARTESIAN_POINT('Ctrl Pts',(3.49655185179623,-1.,1.55897703097859));
#45627=CARTESIAN_POINT('Ctrl Pts',(3.49655185179623,1.,1.55897703097859));
#45628=CARTESIAN_POINT('Ctrl Pts',(3.49076460877317,-1.,1.5548959590107));
#45629=CARTESIAN_POINT('Ctrl Pts',(3.49076460877317,1.,1.5548959590107));
#45630=CARTESIAN_POINT('Ctrl Pts',(3.48485155928414,-1.,1.55084702970382));
#45631=CARTESIAN_POINT('Ctrl Pts',(3.48485155928414,1.,1.55084702970382));
#45632=CARTESIAN_POINT('Ctrl Pts',(3.47868272898599,-1.,1.54678009290207));
#45633=CARTESIAN_POINT('Ctrl Pts',(3.47868272898599,1.,1.54678009290207));
#45634=CARTESIAN_POINT('Ctrl Pts',(3.47217189224576,-1.,1.54266605398152));
#45635=CARTESIAN_POINT('Ctrl Pts',(3.47217189224576,1.,1.54266605398152));
#45636=CARTESIAN_POINT('Ctrl Pts',(3.46531752207222,-1.,1.53851507915533));
#45637=CARTESIAN_POINT('Ctrl Pts',(3.46531752207222,1.,1.53851507915533));
#45638=CARTESIAN_POINT('Ctrl Pts',(3.45825932955273,-1.,1.53440195378902));
#45639=CARTESIAN_POINT('Ctrl Pts',(3.45825932955273,1.,1.53440195378902));
#45640=CARTESIAN_POINT('Ctrl Pts',(3.45127136828667,-1.,1.530462444618));
#45641=CARTESIAN_POINT('Ctrl Pts',(3.45127136828667,1.,1.530462444618));
#45642=CARTESIAN_POINT('Ctrl Pts',(3.44469547527,-1.,1.52686242875717));
#45643=CARTESIAN_POINT('Ctrl Pts',(3.44469547527,1.,1.52686242875717));
#45644=CARTESIAN_POINT('Ctrl Pts',(3.43888895974182,-1.,1.52377348950429));
#45645=CARTESIAN_POINT('Ctrl Pts',(3.43888895974182,1.,1.52377348950429));
#45646=CARTESIAN_POINT('Ctrl Pts',(3.43417156977749,-1.,1.52134826724227));
#45647=CARTESIAN_POINT('Ctrl Pts',(3.43417156977749,1.,1.52134826724227));
#45648=CARTESIAN_POINT('Ctrl Pts',(3.43076036253384,-1.,1.51969006980792));
#45649=CARTESIAN_POINT('Ctrl Pts',(3.43076036253384,1.,1.51969006980792));
#45650=CARTESIAN_POINT('Ctrl Pts',(3.42915787669388,-1.,1.51901585838879));
#45651=CARTESIAN_POINT('Ctrl Pts',(3.42915787669388,1.,1.51901585838879));
#45652=CARTESIAN_POINT('Ctrl Pts',(3.42860527148835,-1.,1.51888450659497));
#45653=CARTESIAN_POINT('Ctrl Pts',(3.42860527148835,1.,1.51888450659497));
#45654=CARTESIAN_POINT('Ctrl Pts',(3.42852521763648,-1.,1.51896318668306));
#45655=CARTESIAN_POINT('Ctrl Pts',(3.42852521763648,1.,1.51896318668306));
#45656=CARTESIAN_POINT('Ctrl Pts',(3.42855728381368,-1.,1.519044091397));
#45657=CARTESIAN_POINT('Ctrl Pts',(3.42855728381368,1.,1.519044091397));
#45658=CARTESIAN_POINT('',(3.77614523045147,1.,1.83867539237861));
#45659=CARTESIAN_POINT('Ctrl Pts',(3.77614523045147,1.,1.83867539237861));
#45660=CARTESIAN_POINT('Ctrl Pts',(3.77518714458232,1.,1.83742834010821));
#45661=CARTESIAN_POINT('Ctrl Pts',(3.77326886065484,1.,1.83493697935064));
#45662=CARTESIAN_POINT('Ctrl Pts',(3.77038509819777,1.,1.83120816956515));
#45663=CARTESIAN_POINT('Ctrl Pts',(3.76652740355856,1.,1.82625289221933));
#45664=CARTESIAN_POINT('Ctrl Pts',(3.76168412709652,1.,1.82008629694924));
#45665=CARTESIAN_POINT('Ctrl Pts',(3.75681965683995,1.,1.81394729834032));
#45666=CARTESIAN_POINT('Ctrl Pts',(3.75193395888069,1.,1.80783603939662));
#45667=CARTESIAN_POINT('Ctrl Pts',(3.74702700874954,1.,1.80175271485519));
#45668=CARTESIAN_POINT('Ctrl Pts',(3.74209880351667,1.,1.79569757859041));
#45669=CARTESIAN_POINT('Ctrl Pts',(3.73714934729962,1.,1.78967092823139));
#45670=CARTESIAN_POINT('Ctrl Pts',(3.73217863095022,1.,1.78367308442682));
#45671=CARTESIAN_POINT('Ctrl Pts',(3.72718661205504,1.,1.77770437039606));
#45672=CARTESIAN_POINT('Ctrl Pts',(3.72217319911429,1.,1.77176509401846));
#45673=CARTESIAN_POINT('Ctrl Pts',(3.71713822377675,1.,1.76585552124549));
#45674=CARTESIAN_POINT('Ctrl Pts',(3.71208146346454,1.,1.75997588499021));
#45675=CARTESIAN_POINT('Ctrl Pts',(3.70700269736876,1.,1.75412641804148));
#45676=CARTESIAN_POINT('Ctrl Pts',(3.70190175673422,1.,1.74830738046092));
#45677=CARTESIAN_POINT('Ctrl Pts',(3.6967785691046,1.,1.74251908492589));
#45678=CARTESIAN_POINT('Ctrl Pts',(3.69163322647906,1.,1.73676193254493));
#45679=CARTESIAN_POINT('Ctrl Pts',(3.68646597019188,1.,1.73103640956647));
#45680=CARTESIAN_POINT('Ctrl Pts',(3.68127704936472,1.,1.72534302437003));
#45681=CARTESIAN_POINT('Ctrl Pts',(3.67606660374665,1.,1.71968225581787));
#45682=CARTESIAN_POINT('Ctrl Pts',(3.67083454901629,1.,1.71405450210392));
#45683=CARTESIAN_POINT('Ctrl Pts',(3.6655804319893,1.,1.70846001610983));
#45684=CARTESIAN_POINT('Ctrl Pts',(3.6603033877491,1.,1.70289888566904));
#45685=CARTESIAN_POINT('Ctrl Pts',(3.65500246526798,1.,1.69737117722559));
#45686=CARTESIAN_POINT('Ctrl Pts',(3.64967689827393,1.,1.691877054817));
#45687=CARTESIAN_POINT('Ctrl Pts',(3.64432638915199,1.,1.68641690471455));
#45688=CARTESIAN_POINT('Ctrl Pts',(3.63895140887443,1.,1.68099146651577));
#45689=CARTESIAN_POINT('Ctrl Pts',(3.63355343201211,1.,1.67560193613145));
#45690=CARTESIAN_POINT('Ctrl Pts',(3.62813422105257,1.,1.67024966008037));
#45691=CARTESIAN_POINT('Ctrl Pts',(3.62269517989104,1.,1.66493585923853));
#45692=CARTESIAN_POINT('Ctrl Pts',(3.61723666482457,1.,1.65966133399186));
#45693=CARTESIAN_POINT('Ctrl Pts',(3.61175734965129,1.,1.65442619244327));
#45694=CARTESIAN_POINT('Ctrl Pts',(3.60625346556992,1.,1.64922952425833));
#45695=CARTESIAN_POINT('Ctrl Pts',(3.6007202851384,1.,1.6440700438558));
#45696=CARTESIAN_POINT('Ctrl Pts',(3.59515368334887,1.,1.63894676675349));
#45697=CARTESIAN_POINT('Ctrl Pts',(3.58955176627876,1.,1.63385971451259));
#45698=CARTESIAN_POINT('Ctrl Pts',(3.5839162577435,1.,1.62881051550748));
#45699=CARTESIAN_POINT('Ctrl Pts',(3.57825455954405,1.,1.62380329464851));
#45700=CARTESIAN_POINT('Ctrl Pts',(3.57257679609826,1.,1.61884340915412));
#45701=CARTESIAN_POINT('Ctrl Pts',(3.56689200468404,1.,1.61393581747522));
#45702=CARTESIAN_POINT('Ctrl Pts',(3.56120432482986,1.,1.60908344685459));
#45703=CARTESIAN_POINT('Ctrl Pts',(3.55550985096117,1.,1.60428584699848));
#45704=CARTESIAN_POINT('Ctrl Pts',(3.54979148634426,1.,1.59953698113444));
#45705=CARTESIAN_POINT('Ctrl Pts',(3.544024581823,1.,1.5948276694975));
#45706=CARTESIAN_POINT('Ctrl Pts',(3.53818616861045,1.,1.59014958368725));
#45707=CARTESIAN_POINT('Ctrl Pts',(3.53226378147068,1.,1.58549906268083));
#45708=CARTESIAN_POINT('Ctrl Pts',(3.52626275334899,1.,1.58088027227856));
#45709=CARTESIAN_POINT('Ctrl Pts',(3.52021847865961,1.,1.5763104998818));
#45710=CARTESIAN_POINT('Ctrl Pts',(3.51418598431733,1.,1.57181569799774));
#45711=CARTESIAN_POINT('Ctrl Pts',(3.50821771695427,1.,1.56742097575041));
#45712=CARTESIAN_POINT('Ctrl Pts',(3.50234321621607,1.,1.56314187758689));
#45713=CARTESIAN_POINT('Ctrl Pts',(3.49655185179623,1.,1.55897703097859));
#45714=CARTESIAN_POINT('Ctrl Pts',(3.49076460877317,1.,1.5548959590107));
#45715=CARTESIAN_POINT('Ctrl Pts',(3.48485155928414,1.,1.55084702970382));
#45716=CARTESIAN_POINT('Ctrl Pts',(3.47868272898599,1.,1.54678009290207));
#45717=CARTESIAN_POINT('Ctrl Pts',(3.47217189224576,1.,1.54266605398152));
#45718=CARTESIAN_POINT('Ctrl Pts',(3.46531752207222,1.,1.53851507915533));
#45719=CARTESIAN_POINT('Ctrl Pts',(3.45825932955273,1.,1.53440195378902));
#45720=CARTESIAN_POINT('Ctrl Pts',(3.45127136828667,1.,1.530462444618));
#45721=CARTESIAN_POINT('Ctrl Pts',(3.44469547527,1.,1.52686242875717));
#45722=CARTESIAN_POINT('Ctrl Pts',(3.43888895974182,1.,1.52377348950429));
#45723=CARTESIAN_POINT('Ctrl Pts',(3.43417156977749,1.,1.52134826724227));
#45724=CARTESIAN_POINT('Ctrl Pts',(3.4310163189349,1.,1.5198144909343));
#45725=CARTESIAN_POINT('Ctrl Pts',(3.42946838852728,1.,1.51914806898539));
#45726=CARTESIAN_POINT('Ctrl Pts',(3.42884302333978,1.,1.51895133295017));
#45727=CARTESIAN_POINT('Ctrl Pts',(3.42864616361967,1.,1.51893924967231));
#45728=CARTESIAN_POINT('Ctrl Pts',(3.42859860294378,1.,1.51895082866166));
#45729=CARTESIAN_POINT('',(3.77614523045147,0.,1.83867539237861));
#45730=CARTESIAN_POINT('Ctrl Pts',(3.24418789321065,-1.,1.88088939428811));
#45731=CARTESIAN_POINT('Ctrl Pts',(3.24418789321065,1.,1.88088939428811));
#45732=CARTESIAN_POINT('Ctrl Pts',(3.24410359189733,-1.,1.8809110068042));
#45733=CARTESIAN_POINT('Ctrl Pts',(3.24410359189733,1.,1.8809110068042));
#45734=CARTESIAN_POINT('Ctrl Pts',(3.24408699284449,-1.,1.8810220187274));
#45735=CARTESIAN_POINT('Ctrl Pts',(3.24408699284449,1.,1.8810220187274));
#45736=CARTESIAN_POINT('Ctrl Pts',(3.24451807186964,-1.,1.88139187908347));
#45737=CARTESIAN_POINT('Ctrl Pts',(3.24451807186964,1.,1.88139187908347));
#45738=CARTESIAN_POINT('Ctrl Pts',(3.24600543790876,-1.,1.88229202583187));
#45739=CARTESIAN_POINT('Ctrl Pts',(3.24600543790876,1.,1.88229202583187));
#45740=CARTESIAN_POINT('Ctrl Pts',(3.24935200512055,-1.,1.88407708646435));
#45741=CARTESIAN_POINT('Ctrl Pts',(3.24935200512055,1.,1.88407708646435));
#45742=CARTESIAN_POINT('Ctrl Pts',(3.25408686339298,-1.,1.88646802523372));
#45743=CARTESIAN_POINT('Ctrl Pts',(3.25408686339298,1.,1.88646802523372));
#45744=CARTESIAN_POINT('Ctrl Pts',(3.2599988519361,-1.,1.88934996203508));
#45745=CARTESIAN_POINT('Ctrl Pts',(3.2599988519361,1.,1.88934996203508));
#45746=CARTESIAN_POINT('Ctrl Pts',(3.2667765388833,-1.,1.89255393500769));
#45747=CARTESIAN_POINT('Ctrl Pts',(3.2667765388833,1.,1.89255393500769));
#45748=CARTESIAN_POINT('Ctrl Pts',(3.27407108932908,-1.,1.89589172903662));
#45749=CARTESIAN_POINT('Ctrl Pts',(3.27407108932908,1.,1.89589172903662));
#45750=CARTESIAN_POINT('Ctrl Pts',(3.28154737912287,-1.,1.89918429230425));
#45751=CARTESIAN_POINT('Ctrl Pts',(3.28154737912287,1.,1.89918429230425));
#45752=CARTESIAN_POINT('Ctrl Pts',(3.28893448600364,-1.,1.9022897124757));
#45753=CARTESIAN_POINT('Ctrl Pts',(3.28893448600364,1.,1.9022897124757));
#45754=CARTESIAN_POINT('Ctrl Pts',(3.29608978722258,-1.,1.9051389186417));
#45755=CARTESIAN_POINT('Ctrl Pts',(3.29608978722258,1.,1.9051389186417));
#45756=CARTESIAN_POINT('Ctrl Pts',(3.30300595568341,-1.,1.90773912171424));
#45757=CARTESIAN_POINT('Ctrl Pts',(3.30300595568341,1.,1.90773912171424));
#45758=CARTESIAN_POINT('Ctrl Pts',(3.30975721158694,-1.,1.91014297830502));
#45759=CARTESIAN_POINT('Ctrl Pts',(3.30975721158694,1.,1.91014297830502));
#45760=CARTESIAN_POINT('Ctrl Pts',(3.31646052426395,-1.,1.91242616234459));
#45761=CARTESIAN_POINT('Ctrl Pts',(3.31646052426395,1.,1.91242616234459));
#45762=CARTESIAN_POINT('Ctrl Pts',(3.32323403454507,-1.,1.91466343916612));
#45763=CARTESIAN_POINT('Ctrl Pts',(3.32323403454507,1.,1.91466343916612));
#45764=CARTESIAN_POINT('Ctrl Pts',(3.33014884257812,-1.,1.91690081930297));
#45765=CARTESIAN_POINT('Ctrl Pts',(3.33014884257812,1.,1.91690081930297));
#45766=CARTESIAN_POINT('Ctrl Pts',(3.33721230709948,-1.,1.91914609610173));
#45767=CARTESIAN_POINT('Ctrl Pts',(3.33721230709948,1.,1.91914609610173));
#45768=CARTESIAN_POINT('Ctrl Pts',(3.34439448941915,-1.,1.92138450828378));
#45769=CARTESIAN_POINT('Ctrl Pts',(3.34439448941915,1.,1.92138450828378));
#45770=CARTESIAN_POINT('Ctrl Pts',(3.35164424847206,-1.,1.92358838440518));
#45771=CARTESIAN_POINT('Ctrl Pts',(3.35164424847206,1.,1.92358838440518));
#45772=CARTESIAN_POINT('Ctrl Pts',(3.35890824422976,-1.,1.92572846125763));
#45773=CARTESIAN_POINT('Ctrl Pts',(3.35890824422976,1.,1.92572846125763));
#45774=CARTESIAN_POINT('Ctrl Pts',(3.36615168657597,-1.,1.92778626543803));
#45775=CARTESIAN_POINT('Ctrl Pts',(3.36615168657597,1.,1.92778626543803));
#45776=CARTESIAN_POINT('Ctrl Pts',(3.37336807068078,-1.,1.92975993109897));
#45777=CARTESIAN_POINT('Ctrl Pts',(3.37336807068078,1.,1.92975993109897));
#45778=CARTESIAN_POINT('Ctrl Pts',(3.38056768525577,-1.,1.93165739093292));
#45779=CARTESIAN_POINT('Ctrl Pts',(3.38056768525577,1.,1.93165739093292));
#45780=CARTESIAN_POINT('Ctrl Pts',(3.38777076883267,-1.,1.93349233176794));
#45781=CARTESIAN_POINT('Ctrl Pts',(3.38777076883267,1.,1.93349233176794));
#45782=CARTESIAN_POINT('Ctrl Pts',(3.39499923640789,-1.,1.93527929945982));
#45783=CARTESIAN_POINT('Ctrl Pts',(3.39499923640789,1.,1.93527929945982));
#45784=CARTESIAN_POINT('Ctrl Pts',(3.40226802104093,-1.,1.93702857723089));
#45785=CARTESIAN_POINT('Ctrl Pts',(3.40226802104093,1.,1.93702857723089));
#45786=CARTESIAN_POINT('Ctrl Pts',(3.40957978266622,-1.,1.93874306008132));
#45787=CARTESIAN_POINT('Ctrl Pts',(3.40957978266622,1.,1.93874306008132));
#45788=CARTESIAN_POINT('Ctrl Pts',(3.41692971994082,-1.,1.94042111965237));
#45789=CARTESIAN_POINT('Ctrl Pts',(3.41692971994082,1.,1.94042111965237));
#45790=CARTESIAN_POINT('Ctrl Pts',(3.42430850941497,-1.,1.94205835913692));
#45791=CARTESIAN_POINT('Ctrl Pts',(3.42430850941497,1.,1.94205835913692));
#45792=CARTESIAN_POINT('Ctrl Pts',(3.43170586602436,-1.,1.94364973660285));
#45793=CARTESIAN_POINT('Ctrl Pts',(3.43170586602436,1.,1.94364973660285));
#45794=CARTESIAN_POINT('Ctrl Pts',(3.43911410197693,-1.,1.94519168842883));
#45795=CARTESIAN_POINT('Ctrl Pts',(3.43911410197693,1.,1.94519168842883));
#45796=CARTESIAN_POINT('Ctrl Pts',(3.44653088665685,-1.,1.94668377715332));
#45797=CARTESIAN_POINT('Ctrl Pts',(3.44653088665685,1.,1.94668377715332));
#45798=CARTESIAN_POINT('Ctrl Pts',(3.45395731584051,-1.,1.94812754766524));
#45799=CARTESIAN_POINT('Ctrl Pts',(3.45395731584051,1.,1.94812754766524));
#45800=CARTESIAN_POINT('Ctrl Pts',(3.46139661060959,-1.,1.94952575850196));
#45801=CARTESIAN_POINT('Ctrl Pts',(3.46139661060959,1.,1.94952575850196));
#45802=CARTESIAN_POINT('Ctrl Pts',(3.4688525897419,-1.,1.95088147859876));
#45803=CARTESIAN_POINT('Ctrl Pts',(3.4688525897419,1.,1.95088147859876));
#45804=CARTESIAN_POINT('Ctrl Pts',(3.47632820495926,-1.,1.95219722189878));
#45805=CARTESIAN_POINT('Ctrl Pts',(3.47632820495926,1.,1.95219722189878));
#45806=CARTESIAN_POINT('Ctrl Pts',(3.48382414832648,-1.,1.95347412486316));
#45807=CARTESIAN_POINT('Ctrl Pts',(3.48382414832648,1.,1.95347412486316));
#45808=CARTESIAN_POINT('Ctrl Pts',(3.49133956289154,-1.,1.95471236969653));
#45809=CARTESIAN_POINT('Ctrl Pts',(3.49133956289154,1.,1.95471236969653));
#45810=CARTESIAN_POINT('Ctrl Pts',(3.49887263575602,-1.,1.9559115382367));
#45811=CARTESIAN_POINT('Ctrl Pts',(3.49887263575602,1.,1.9559115382367));
#45812=CARTESIAN_POINT('Ctrl Pts',(3.50642124159913,-1.,1.95707099606514));
#45813=CARTESIAN_POINT('Ctrl Pts',(3.50642124159913,1.,1.95707099606514));
#45814=CARTESIAN_POINT('Ctrl Pts',(3.51398354617772,-1.,1.95819025316768));
#45815=CARTESIAN_POINT('Ctrl Pts',(3.51398354617772,1.,1.95819025316768));
#45816=CARTESIAN_POINT('Ctrl Pts',(3.52155867431438,-1.,1.95926936324436));
#45817=CARTESIAN_POINT('Ctrl Pts',(3.52155867431438,1.,1.95926936324436));
#45818=CARTESIAN_POINT('Ctrl Pts',(3.52914648844289,-1.,1.96030879411534));
#45819=CARTESIAN_POINT('Ctrl Pts',(3.52914648844289,1.,1.96030879411534));
#45820=CARTESIAN_POINT('Ctrl Pts',(3.53674730625759,-1.,1.96130926212661));
#45821=CARTESIAN_POINT('Ctrl Pts',(3.53674730625759,1.,1.96130926212661));
#45822=CARTESIAN_POINT('Ctrl Pts',(3.54436163300425,-1.,1.96227157573058));
#45823=CARTESIAN_POINT('Ctrl Pts',(3.54436163300425,1.,1.96227157573058));
#45824=CARTESIAN_POINT('Ctrl Pts',(3.55198990600929,-1.,1.96319648628667));
#45825=CARTESIAN_POINT('Ctrl Pts',(3.55198990600929,1.,1.96319648628667));
#45826=CARTESIAN_POINT('Ctrl Pts',(3.55963218706201,-1.,1.96408450906868));
#45827=CARTESIAN_POINT('Ctrl Pts',(3.55963218706201,1.,1.96408450906868));
#45828=CARTESIAN_POINT('Ctrl Pts',(3.56728820357933,-1.,1.96493594634643));
#45829=CARTESIAN_POINT('Ctrl Pts',(3.56728820357933,1.,1.96493594634643));
#45830=CARTESIAN_POINT('Ctrl Pts',(3.57495748601088,-1.,1.96575096652857));
#45831=CARTESIAN_POINT('Ctrl Pts',(3.57495748601088,1.,1.96575096652857));
#45832=CARTESIAN_POINT('Ctrl Pts',(3.58263947663884,-1.,1.9665296668894));
#45833=CARTESIAN_POINT('Ctrl Pts',(3.58263947663884,1.,1.9665296668894));
#45834=CARTESIAN_POINT('Ctrl Pts',(3.5903336402273,-1.,1.96727213799507));
#45835=CARTESIAN_POINT('Ctrl Pts',(3.5903336402273,1.,1.96727213799507));
#45836=CARTESIAN_POINT('Ctrl Pts',(3.59803959819725,-1.,1.96797854118257));
#45837=CARTESIAN_POINT('Ctrl Pts',(3.59803959819725,1.,1.96797854118257));
#45838=CARTESIAN_POINT('Ctrl Pts',(3.60575714017676,-1.,1.96864911885775));
#45839=CARTESIAN_POINT('Ctrl Pts',(3.60575714017676,1.,1.96864911885775));
#45840=CARTESIAN_POINT('Ctrl Pts',(3.61348615496393,-1.,1.96928416040712));
#45841=CARTESIAN_POINT('Ctrl Pts',(3.61348615496393,1.,1.96928416040712));
#45842=CARTESIAN_POINT('Ctrl Pts',(3.62122658401722,-1.,1.96988398129888));
#45843=CARTESIAN_POINT('Ctrl Pts',(3.62122658401722,1.,1.96988398129888));
#45844=CARTESIAN_POINT('Ctrl Pts',(3.62897836973397,-1.,1.97044889850518));
#45845=CARTESIAN_POINT('Ctrl Pts',(3.62897836973397,1.,1.97044889850518));
#45846=CARTESIAN_POINT('Ctrl Pts',(3.63674139590853,-1.,1.97097920454698));
#45847=CARTESIAN_POINT('Ctrl Pts',(3.63674139590853,1.,1.97097920454698));
#45848=CARTESIAN_POINT('Ctrl Pts',(3.64451546724221,-1.,1.97147515441539));
#45849=CARTESIAN_POINT('Ctrl Pts',(3.64451546724221,1.,1.97147515441539));
#45850=CARTESIAN_POINT('Ctrl Pts',(3.65230034717364,-1.,1.97193697240645));
#45851=CARTESIAN_POINT('Ctrl Pts',(3.65230034717364,1.,1.97193697240645));
#45852=CARTESIAN_POINT('Ctrl Pts',(3.66009578166865,-1.,1.97236485439317));
#45853=CARTESIAN_POINT('Ctrl Pts',(3.66009578166865,1.,1.97236485439317));
#45854=CARTESIAN_POINT('Ctrl Pts',(3.66790152751984,-1.,1.9727589719863));
#45855=CARTESIAN_POINT('Ctrl Pts',(3.66790152751984,1.,1.9727589719863));
#45856=CARTESIAN_POINT('Ctrl Pts',(3.67571738106175,-1.,1.97311947678035));
#45857=CARTESIAN_POINT('Ctrl Pts',(3.67571738106175,1.,1.97311947678035));
#45858=CARTESIAN_POINT('Ctrl Pts',(3.68354319913416,-1.,1.97344650303631));
#45859=CARTESIAN_POINT('Ctrl Pts',(3.68354319913416,1.,1.97344650303631));
#45860=CARTESIAN_POINT('Ctrl Pts',(3.69137888597855,-1.,1.97374016224397));
#45861=CARTESIAN_POINT('Ctrl Pts',(3.69137888597855,1.,1.97374016224397));
#45862=CARTESIAN_POINT('Ctrl Pts',(3.69765528558292,-1.,1.97394846382289));
#45863=CARTESIAN_POINT('Ctrl Pts',(3.69765528558292,1.,1.97394846382289));
#45864=CARTESIAN_POINT('Ctrl Pts',(3.70236698911837,-1.,1.97408973726149));
#45865=CARTESIAN_POINT('Ctrl Pts',(3.70236698911837,1.,1.97408973726149));
#45866=CARTESIAN_POINT('Ctrl Pts',(3.7055100813194,-1.,1.974177276451));
#45867=CARTESIAN_POINT('Ctrl Pts',(3.7055100813194,1.,1.974177276451));
#45868=CARTESIAN_POINT('Ctrl Pts',(3.70708211654725,-1.,1.97421938526992));
#45869=CARTESIAN_POINT('Ctrl Pts',(3.70708211654725,1.,1.97421938526992));
#45870=CARTESIAN_POINT('',(3.24413672884902,1.,1.88097764062542));
#45871=CARTESIAN_POINT('Ctrl Pts',(3.24413672884902,-1.,1.88097764062542));
#45872=CARTESIAN_POINT('Ctrl Pts',(3.24413672884902,-0.666666666666667,
1.88097764062542));
#45873=CARTESIAN_POINT('Ctrl Pts',(3.24413672884902,-0.333333333333333,
1.88097764062542));
#45874=CARTESIAN_POINT('Ctrl Pts',(3.24413672884902,0.333333333333333,1.88097764062542));
#45875=CARTESIAN_POINT('Ctrl Pts',(3.24413672884902,0.666666666666667,1.88097764062541));
#45876=CARTESIAN_POINT('Ctrl Pts',(3.24413672884902,1.,1.88097764062541));
#45877=CARTESIAN_POINT('',(3.70708211654725,1.,1.97421938526992));
#45878=CARTESIAN_POINT('',(3.70708211654725,0.,1.97421938526992));
#45879=CARTESIAN_POINT('Ctrl Pts',(3.24413672884902,1.,1.88097764062542));
#45880=CARTESIAN_POINT('Ctrl Pts',(3.24415531671311,1.,1.88102292397987));
#45881=CARTESIAN_POINT('Ctrl Pts',(3.24428080352952,1.,1.88117508446657));
#45882=CARTESIAN_POINT('Ctrl Pts',(3.24480754675942,1.,1.88156537699118));
#45883=CARTESIAN_POINT('Ctrl Pts',(3.24625654410705,1.,1.88242596600422));
#45884=CARTESIAN_POINT('Ctrl Pts',(3.24935200512055,1.,1.88407708646435));
#45885=CARTESIAN_POINT('Ctrl Pts',(3.25408686339298,1.,1.88646802523372));
#45886=CARTESIAN_POINT('Ctrl Pts',(3.2599988519361,1.,1.88934996203508));
#45887=CARTESIAN_POINT('Ctrl Pts',(3.2667765388833,1.,1.89255393500769));
#45888=CARTESIAN_POINT('Ctrl Pts',(3.27407108932908,1.,1.89589172903662));
#45889=CARTESIAN_POINT('Ctrl Pts',(3.28154737912287,1.,1.89918429230425));
#45890=CARTESIAN_POINT('Ctrl Pts',(3.28893448600364,1.,1.9022897124757));
#45891=CARTESIAN_POINT('Ctrl Pts',(3.29608978722258,1.,1.9051389186417));
#45892=CARTESIAN_POINT('Ctrl Pts',(3.30300595568341,1.,1.90773912171424));
#45893=CARTESIAN_POINT('Ctrl Pts',(3.30975721158694,1.,1.91014297830502));
#45894=CARTESIAN_POINT('Ctrl Pts',(3.31646052426395,1.,1.91242616234459));
#45895=CARTESIAN_POINT('Ctrl Pts',(3.32323403454507,1.,1.91466343916612));
#45896=CARTESIAN_POINT('Ctrl Pts',(3.33014884257812,1.,1.91690081930297));
#45897=CARTESIAN_POINT('Ctrl Pts',(3.33721230709948,1.,1.91914609610173));
#45898=CARTESIAN_POINT('Ctrl Pts',(3.34439448941915,1.,1.92138450828378));
#45899=CARTESIAN_POINT('Ctrl Pts',(3.35164424847206,1.,1.92358838440518));
#45900=CARTESIAN_POINT('Ctrl Pts',(3.35890824422976,1.,1.92572846125763));
#45901=CARTESIAN_POINT('Ctrl Pts',(3.36615168657597,1.,1.92778626543803));
#45902=CARTESIAN_POINT('Ctrl Pts',(3.37336807068078,1.,1.92975993109897));
#45903=CARTESIAN_POINT('Ctrl Pts',(3.38056768525577,1.,1.93165739093292));
#45904=CARTESIAN_POINT('Ctrl Pts',(3.38777076883267,1.,1.93349233176794));
#45905=CARTESIAN_POINT('Ctrl Pts',(3.39499923640789,1.,1.93527929945982));
#45906=CARTESIAN_POINT('Ctrl Pts',(3.40226802104093,1.,1.93702857723089));
#45907=CARTESIAN_POINT('Ctrl Pts',(3.40957978266622,1.,1.93874306008132));
#45908=CARTESIAN_POINT('Ctrl Pts',(3.41692971994082,1.,1.94042111965237));
#45909=CARTESIAN_POINT('Ctrl Pts',(3.42430850941497,1.,1.94205835913692));
#45910=CARTESIAN_POINT('Ctrl Pts',(3.43170586602436,1.,1.94364973660285));
#45911=CARTESIAN_POINT('Ctrl Pts',(3.43911410197693,1.,1.94519168842883));
#45912=CARTESIAN_POINT('Ctrl Pts',(3.44653088665685,1.,1.94668377715332));
#45913=CARTESIAN_POINT('Ctrl Pts',(3.45395731584051,1.,1.94812754766524));
#45914=CARTESIAN_POINT('Ctrl Pts',(3.46139661060959,1.,1.94952575850196));
#45915=CARTESIAN_POINT('Ctrl Pts',(3.4688525897419,1.,1.95088147859876));
#45916=CARTESIAN_POINT('Ctrl Pts',(3.47632820495926,1.,1.95219722189878));
#45917=CARTESIAN_POINT('Ctrl Pts',(3.48382414832648,1.,1.95347412486316));
#45918=CARTESIAN_POINT('Ctrl Pts',(3.49133956289154,1.,1.95471236969653));
#45919=CARTESIAN_POINT('Ctrl Pts',(3.49887263575602,1.,1.9559115382367));
#45920=CARTESIAN_POINT('Ctrl Pts',(3.50642124159913,1.,1.95707099606514));
#45921=CARTESIAN_POINT('Ctrl Pts',(3.51398354617772,1.,1.95819025316768));
#45922=CARTESIAN_POINT('Ctrl Pts',(3.52155867431438,1.,1.95926936324436));
#45923=CARTESIAN_POINT('Ctrl Pts',(3.52914648844289,1.,1.96030879411534));
#45924=CARTESIAN_POINT('Ctrl Pts',(3.53674730625759,1.,1.96130926212661));
#45925=CARTESIAN_POINT('Ctrl Pts',(3.54436163300425,1.,1.96227157573058));
#45926=CARTESIAN_POINT('Ctrl Pts',(3.55198990600929,1.,1.96319648628667));
#45927=CARTESIAN_POINT('Ctrl Pts',(3.55963218706201,1.,1.96408450906868));
#45928=CARTESIAN_POINT('Ctrl Pts',(3.56728820357933,1.,1.96493594634643));
#45929=CARTESIAN_POINT('Ctrl Pts',(3.57495748601088,1.,1.96575096652857));
#45930=CARTESIAN_POINT('Ctrl Pts',(3.58263947663884,1.,1.9665296668894));
#45931=CARTESIAN_POINT('Ctrl Pts',(3.5903336402273,1.,1.96727213799507));
#45932=CARTESIAN_POINT('Ctrl Pts',(3.59803959819725,1.,1.96797854118257));
#45933=CARTESIAN_POINT('Ctrl Pts',(3.60575714017676,1.,1.96864911885775));
#45934=CARTESIAN_POINT('Ctrl Pts',(3.61348615496393,1.,1.96928416040712));
#45935=CARTESIAN_POINT('Ctrl Pts',(3.62122658401722,1.,1.96988398129888));
#45936=CARTESIAN_POINT('Ctrl Pts',(3.62897836973397,1.,1.97044889850518));
#45937=CARTESIAN_POINT('Ctrl Pts',(3.63674139590853,1.,1.97097920454698));
#45938=CARTESIAN_POINT('Ctrl Pts',(3.64451546724221,1.,1.97147515441539));
#45939=CARTESIAN_POINT('Ctrl Pts',(3.65230034717364,1.,1.97193697240645));
#45940=CARTESIAN_POINT('Ctrl Pts',(3.66009578166865,1.,1.97236485439317));
#45941=CARTESIAN_POINT('Ctrl Pts',(3.66790152751984,1.,1.9727589719863));
#45942=CARTESIAN_POINT('Ctrl Pts',(3.67571738106175,1.,1.97311947678035));
#45943=CARTESIAN_POINT('Ctrl Pts',(3.68354319913416,1.,1.97344650303631));
#45944=CARTESIAN_POINT('Ctrl Pts',(3.69137888597855,1.,1.97374016224397));
#45945=CARTESIAN_POINT('Ctrl Pts',(3.69765528558292,1.,1.97394846382289));
#45946=CARTESIAN_POINT('Ctrl Pts',(3.70236698911837,1.,1.97408973726149));
#45947=CARTESIAN_POINT('Ctrl Pts',(3.7055100813194,1.,1.974177276451));
#45948=CARTESIAN_POINT('Ctrl Pts',(3.70708211654725,1.,1.97421938526992));
#45949=CARTESIAN_POINT('Origin',(3.70708211654725,0.,1.97421938526992));
#45950=CARTESIAN_POINT('',(3.77614523045147,1.,1.83867539237861));
#45951=CARTESIAN_POINT('Origin',(0.,0.,0.));
#45952=CARTESIAN_POINT('',(3.14877060440425,1.,2.03660101169564));
#45953=CARTESIAN_POINT('Origin',(0.,1.,0.));
#45954=CARTESIAN_POINT('Ctrl Pts',(3.14877060440425,1.,2.03660101169564));
#45955=CARTESIAN_POINT('Ctrl Pts',(3.14877060440425,0.666666666666667,2.03660101169564));
#45956=CARTESIAN_POINT('Ctrl Pts',(3.14877060440425,0.333333333333333,2.03660101169564));
#45957=CARTESIAN_POINT('Ctrl Pts',(3.14877060440425,-0.333333333333333,
2.03660101169564));
#45958=CARTESIAN_POINT('Ctrl Pts',(3.14877060440425,-0.666666666666667,
2.03660101169564));
#45959=CARTESIAN_POINT('Ctrl Pts',(3.14877060440425,-1.,2.03660101169564));
#45960=CARTESIAN_POINT('Ctrl Pts',(3.44202241512147,-1.,2.40675750623143));
#45961=CARTESIAN_POINT('Ctrl Pts',(3.44202241512147,1.,2.40675750623143));
#45962=CARTESIAN_POINT('Ctrl Pts',(3.44127120683402,-1.,2.40537592959345));
#45963=CARTESIAN_POINT('Ctrl Pts',(3.44127120683402,1.,2.40537592959345));
#45964=CARTESIAN_POINT('Ctrl Pts',(3.43976627485223,-1.,2.40261515590099));
#45965=CARTESIAN_POINT('Ctrl Pts',(3.43976627485223,1.,2.40261515590099));
#45966=CARTESIAN_POINT('Ctrl Pts',(3.43750133066036,-1.,2.39848113411429));
#45967=CARTESIAN_POINT('Ctrl Pts',(3.43750133066036,1.,2.39848113411429));
#45968=CARTESIAN_POINT('Ctrl Pts',(3.43446630680436,-1.,2.39298338805823));
#45969=CARTESIAN_POINT('Ctrl Pts',(3.43446630680436,1.,2.39298338805823));
#45970=CARTESIAN_POINT('Ctrl Pts',(3.43064732714472,-1.,2.38613505844641));
#45971=CARTESIAN_POINT('Ctrl Pts',(3.43064732714472,1.,2.38613505844641));
#45972=CARTESIAN_POINT('Ctrl Pts',(3.42680309755241,-1.,2.37931067029517));
#45973=CARTESIAN_POINT('Ctrl Pts',(3.42680309755241,1.,2.37931067029517));
#45974=CARTESIAN_POINT('Ctrl Pts',(3.42293356216595,-1.,2.37251035954351));
#45975=CARTESIAN_POINT('Ctrl Pts',(3.42293356216595,1.,2.37251035954351));
#45976=CARTESIAN_POINT('Ctrl Pts',(3.41903866635384,-1.,2.36573431470314));
#45977=CARTESIAN_POINT('Ctrl Pts',(3.41903866635384,1.,2.36573431470314));
#45978=CARTESIAN_POINT('Ctrl Pts',(3.4151183675076,-1.,2.35898278606449));
#45979=CARTESIAN_POINT('Ctrl Pts',(3.4151183675076,1.,2.35898278606449));
#45980=CARTESIAN_POINT('Ctrl Pts',(3.41117262313464,-1.,2.35225606823649));
#45981=CARTESIAN_POINT('Ctrl Pts',(3.41117262313464,1.,2.35225606823649));
#45982=CARTESIAN_POINT('Ctrl Pts',(3.40720137403888,-1.,2.34555447648901));
#45983=CARTESIAN_POINT('Ctrl Pts',(3.40720137403888,1.,2.34555447648901));
#45984=CARTESIAN_POINT('Ctrl Pts',(3.40320452776646,-1.,2.33887832342715));
#45985=CARTESIAN_POINT('Ctrl Pts',(3.40320452776646,1.,2.33887832342715));
#45986=CARTESIAN_POINT('Ctrl Pts',(3.39918194578115,-1.,2.33222789882601));
#45987=CARTESIAN_POINT('Ctrl Pts',(3.39918194578115,1.,2.33222789882601));
#45988=CARTESIAN_POINT('Ctrl Pts',(3.39513342020045,-1.,2.32560343902683));
#45989=CARTESIAN_POINT('Ctrl Pts',(3.39513342020045,1.,2.32560343902683));
#45990=CARTESIAN_POINT('Ctrl Pts',(3.39105869475112,-1.,2.31900513925627));
#45991=CARTESIAN_POINT('Ctrl Pts',(3.39105869475112,1.,2.31900513925627));
#45992=CARTESIAN_POINT('Ctrl Pts',(3.38695751492659,-1.,2.31243319489505));
#45993=CARTESIAN_POINT('Ctrl Pts',(3.38695751492659,1.,2.31243319489505));
#45994=CARTESIAN_POINT('Ctrl Pts',(3.38282967336676,-1.,2.30588783640389));
#45995=CARTESIAN_POINT('Ctrl Pts',(3.38282967336676,1.,2.30588783640389));
#45996=CARTESIAN_POINT('Ctrl Pts',(3.37867504959382,-1.,2.29936936127588));
#45997=CARTESIAN_POINT('Ctrl Pts',(3.37867504959382,1.,2.29936936127588));
#45998=CARTESIAN_POINT('Ctrl Pts',(3.37449367172707,-1.,2.2928781800731));
#45999=CARTESIAN_POINT('Ctrl Pts',(3.37449367172707,1.,2.2928781800731));
#46000=CARTESIAN_POINT('Ctrl Pts',(3.37028570206357,-1.,2.28641481081045));
#46001=CARTESIAN_POINT('Ctrl Pts',(3.37028570206357,1.,2.28641481081045));
#46002=CARTESIAN_POINT('Ctrl Pts',(3.36605130712978,-1.,2.27997979457968));
#46003=CARTESIAN_POINT('Ctrl Pts',(3.36605130712978,1.,2.27997979457968));
#46004=CARTESIAN_POINT('Ctrl Pts',(3.36179055004369,-1.,2.27357362620902));
#46005=CARTESIAN_POINT('Ctrl Pts',(3.36179055004369,1.,2.27357362620902));
#46006=CARTESIAN_POINT('Ctrl Pts',(3.35750328523077,-1.,2.26719668579921));
#46007=CARTESIAN_POINT('Ctrl Pts',(3.35750328523077,1.,2.26719668579921));
#46008=CARTESIAN_POINT('Ctrl Pts',(3.35318902552676,-1.,2.26084915222484));
#46009=CARTESIAN_POINT('Ctrl Pts',(3.35318902552676,1.,2.26084915222484));
#46010=CARTESIAN_POINT('Ctrl Pts',(3.34884690292342,-1.,2.25453097693524));
#46011=CARTESIAN_POINT('Ctrl Pts',(3.34884690292342,1.,2.25453097693524));
#46012=CARTESIAN_POINT('Ctrl Pts',(3.34447596770768,-1.,2.24824207678288));
#46013=CARTESIAN_POINT('Ctrl Pts',(3.34447596770768,1.,2.24824207678288));
#46014=CARTESIAN_POINT('Ctrl Pts',(3.34007543738044,-1.,2.24198249391437));
#46015=CARTESIAN_POINT('Ctrl Pts',(3.34007543738044,1.,2.24198249391437));
#46016=CARTESIAN_POINT('Ctrl Pts',(3.33564495756478,-1.,2.2357525632881));
#46017=CARTESIAN_POINT('Ctrl Pts',(3.33564495756478,1.,2.2357525632881));
#46018=CARTESIAN_POINT('Ctrl Pts',(3.33118487773593,-1.,2.22955308907221));
#46019=CARTESIAN_POINT('Ctrl Pts',(3.33118487773593,1.,2.22955308907221));
#46020=CARTESIAN_POINT('Ctrl Pts',(3.32669646722871,-1.,2.22338548312759));
#46021=CARTESIAN_POINT('Ctrl Pts',(3.32669646722871,1.,2.22338548312759));
#46022=CARTESIAN_POINT('Ctrl Pts',(3.32218125618955,-1.,2.21725135110889));
#46023=CARTESIAN_POINT('Ctrl Pts',(3.32218125618955,1.,2.21725135110889));
#46024=CARTESIAN_POINT('Ctrl Pts',(3.31764044024231,-1.,2.21115211847872));
#46025=CARTESIAN_POINT('Ctrl Pts',(3.31764044024231,1.,2.21115211847872));
#46026=CARTESIAN_POINT('Ctrl Pts',(3.3130742460895,-1.,2.20508863150608));
#46027=CARTESIAN_POINT('Ctrl Pts',(3.3130742460895,1.,2.20508863150608));
#46028=CARTESIAN_POINT('Ctrl Pts',(3.30848134694596,-1.,2.19906078949925));
#46029=CARTESIAN_POINT('Ctrl Pts',(3.30848134694596,1.,2.19906078949925));
#46030=CARTESIAN_POINT('Ctrl Pts',(3.30385816281831,-1.,2.19306710376112));
#46031=CARTESIAN_POINT('Ctrl Pts',(3.30385816281831,1.,2.19306710376112));
#46032=CARTESIAN_POINT('Ctrl Pts',(3.29920022557635,-1.,2.18710556500325));
#46033=CARTESIAN_POINT('Ctrl Pts',(3.29920022557635,1.,2.18710556500325));
#46034=CARTESIAN_POINT('Ctrl Pts',(3.29450361500484,-1.,2.18117455557062));
#46035=CARTESIAN_POINT('Ctrl Pts',(3.29450361500484,1.,2.18117455557062));
#46036=CARTESIAN_POINT('Ctrl Pts',(3.28976645712566,-1.,2.17527380048422));
#46037=CARTESIAN_POINT('Ctrl Pts',(3.28976645712566,1.,2.17527380048422));
#46038=CARTESIAN_POINT('Ctrl Pts',(3.2849901997973,-1.,2.16940517773459));
#46039=CARTESIAN_POINT('Ctrl Pts',(3.2849901997973,1.,2.16940517773459));
#46040=CARTESIAN_POINT('Ctrl Pts',(3.28018150841414,-1.,2.16357391934434));
#46041=CARTESIAN_POINT('Ctrl Pts',(3.28018150841414,1.,2.16357391934434));
#46042=CARTESIAN_POINT('Ctrl Pts',(3.27534954469206,-1.,2.15778690038359));
#46043=CARTESIAN_POINT('Ctrl Pts',(3.27534954469206,1.,2.15778690038359));
#46044=CARTESIAN_POINT('Ctrl Pts',(3.27050245897244,-1.,2.15205043199818));
#46045=CARTESIAN_POINT('Ctrl Pts',(3.27050245897244,1.,2.15205043199818));
#46046=CARTESIAN_POINT('Ctrl Pts',(3.26564388189764,-1.,2.14636805295663));
#46047=CARTESIAN_POINT('Ctrl Pts',(3.26564388189764,1.,2.14636805295663));
#46048=CARTESIAN_POINT('Ctrl Pts',(3.26077002641868,-1.,2.14073870754258));
#46049=CARTESIAN_POINT('Ctrl Pts',(3.26077002641868,1.,2.14073870754258));
#46050=CARTESIAN_POINT('Ctrl Pts',(3.25586495065027,-1.,2.13515375878786));
#46051=CARTESIAN_POINT('Ctrl Pts',(3.25586495065027,1.,2.13515375878786));
#46052=CARTESIAN_POINT('Ctrl Pts',(3.25090574493994,-1.,2.1296002839681));
#46053=CARTESIAN_POINT('Ctrl Pts',(3.25090574493994,1.,2.1296002839681));
#46054=CARTESIAN_POINT('Ctrl Pts',(3.24587102613347,-1.,2.12406646410943));
#46055=CARTESIAN_POINT('Ctrl Pts',(3.24587102613347,1.,2.12406646410943));
#46056=CARTESIAN_POINT('Ctrl Pts',(3.24074905517282,-1.,2.11854673326972));
#46057=CARTESIAN_POINT('Ctrl Pts',(3.24074905517282,1.,2.11854673326972));
#46058=CARTESIAN_POINT('Ctrl Pts',(3.23554444767115,-1.,2.11304604021784));
#46059=CARTESIAN_POINT('Ctrl Pts',(3.23554444767115,1.,2.11304604021784));
#46060=CARTESIAN_POINT('Ctrl Pts',(3.23028945793334,-1.,2.1075869964248));
#46061=CARTESIAN_POINT('Ctrl Pts',(3.23028945793334,1.,2.1075869964248));
#46062=CARTESIAN_POINT('Ctrl Pts',(3.22503437553496,-1.,2.10220384298534));
#46063=CARTESIAN_POINT('Ctrl Pts',(3.22503437553496,1.,2.10220384298534));
#46064=CARTESIAN_POINT('Ctrl Pts',(3.21982707347067,-1.,2.09692958434933));
#46065=CARTESIAN_POINT('Ctrl Pts',(3.21982707347067,1.,2.09692958434933));
#46066=CARTESIAN_POINT('Ctrl Pts',(3.2146942960168,-1.,2.0917841946046));
#46067=CARTESIAN_POINT('Ctrl Pts',(3.2146942960168,1.,2.0917841946046));
#46068=CARTESIAN_POINT('Ctrl Pts',(3.20962575845433,-1.,2.08676465517435));
#46069=CARTESIAN_POINT('Ctrl Pts',(3.20962575845433,1.,2.08676465517435));
#46070=CARTESIAN_POINT('Ctrl Pts',(3.20454818630635,-1.,2.08182850370816));
#46071=CARTESIAN_POINT('Ctrl Pts',(3.20454818630635,1.,2.08182850370816));
#46072=CARTESIAN_POINT('Ctrl Pts',(3.19934132835879,-1.,2.0769044187063));
#46073=CARTESIAN_POINT('Ctrl Pts',(3.19934132835879,1.,2.0769044187063));
#46074=CARTESIAN_POINT('Ctrl Pts',(3.19388465568113,-1.,2.07192253497765));
#46075=CARTESIAN_POINT('Ctrl Pts',(3.19388465568113,1.,2.07192253497765));
#46076=CARTESIAN_POINT('Ctrl Pts',(3.18809755562297,-1.,2.06684062744065));
#46077=CARTESIAN_POINT('Ctrl Pts',(3.18809755562297,1.,2.06684062744065));
#46078=CARTESIAN_POINT('Ctrl Pts',(3.18197692964677,-1.,2.06166849827143));
#46079=CARTESIAN_POINT('Ctrl Pts',(3.18197692964677,1.,2.06166849827143));
#46080=CARTESIAN_POINT('Ctrl Pts',(3.17564906975592,-1.,2.05650186773279));
#46081=CARTESIAN_POINT('Ctrl Pts',(3.17564906975592,1.,2.05650186773279));
#46082=CARTESIAN_POINT('Ctrl Pts',(3.16936341689859,-1.,2.05151770247452));
#46083=CARTESIAN_POINT('Ctrl Pts',(3.16936341689859,1.,2.05151770247452));
#46084=CARTESIAN_POINT('Ctrl Pts',(3.16343165059235,-1.,2.0469333124766));
#46085=CARTESIAN_POINT('Ctrl Pts',(3.16343165059235,1.,2.0469333124766));
#46086=CARTESIAN_POINT('Ctrl Pts',(3.15817983946525,-1.,2.04297406404132));
#46087=CARTESIAN_POINT('Ctrl Pts',(3.15817983946525,1.,2.04297406404132));
#46088=CARTESIAN_POINT('Ctrl Pts',(3.1538999167466,-1.,2.03984073791432));
#46089=CARTESIAN_POINT('Ctrl Pts',(3.1538999167466,1.,2.03984073791432));
#46090=CARTESIAN_POINT('Ctrl Pts',(3.15079010635326,-1.,2.03766932526171));
#46091=CARTESIAN_POINT('Ctrl Pts',(3.15079010635326,1.,2.03766932526171));
#46092=CARTESIAN_POINT('Ctrl Pts',(3.14931281967585,-1.,2.03675273048882));
#46093=CARTESIAN_POINT('Ctrl Pts',(3.14931281967585,1.,2.03675273048882));
#46094=CARTESIAN_POINT('Ctrl Pts',(3.14878756590499,-1.,2.03653654935384));
#46095=CARTESIAN_POINT('Ctrl Pts',(3.14878756590499,1.,2.03653654935384));
#46096=CARTESIAN_POINT('Ctrl Pts',(3.14869618937138,-1.,2.036601737578));
#46097=CARTESIAN_POINT('Ctrl Pts',(3.14869618937138,1.,2.036601737578));
#46098=CARTESIAN_POINT('Ctrl Pts',(3.1487152044751,-1.,2.03668666247593));
#46099=CARTESIAN_POINT('Ctrl Pts',(3.1487152044751,1.,2.03668666247593));
#46100=CARTESIAN_POINT('',(3.44202241512147,1.,2.40675750623143));
#46101=CARTESIAN_POINT('Ctrl Pts',(3.44202241512147,1.,2.40675750623143));
#46102=CARTESIAN_POINT('Ctrl Pts',(3.44127120683402,1.,2.40537592959345));
#46103=CARTESIAN_POINT('Ctrl Pts',(3.43976627485223,1.,2.40261515590099));
#46104=CARTESIAN_POINT('Ctrl Pts',(3.43750133066036,1.,2.39848113411429));
#46105=CARTESIAN_POINT('Ctrl Pts',(3.43446630680436,1.,2.39298338805823));
#46106=CARTESIAN_POINT('Ctrl Pts',(3.43064732714472,1.,2.38613505844641));
#46107=CARTESIAN_POINT('Ctrl Pts',(3.42680309755241,1.,2.37931067029517));
#46108=CARTESIAN_POINT('Ctrl Pts',(3.42293356216595,1.,2.37251035954351));
#46109=CARTESIAN_POINT('Ctrl Pts',(3.41903866635384,1.,2.36573431470314));
#46110=CARTESIAN_POINT('Ctrl Pts',(3.4151183675076,1.,2.35898278606449));
#46111=CARTESIAN_POINT('Ctrl Pts',(3.41117262313464,1.,2.35225606823649));
#46112=CARTESIAN_POINT('Ctrl Pts',(3.40720137403888,1.,2.34555447648901));
#46113=CARTESIAN_POINT('Ctrl Pts',(3.40320452776646,1.,2.33887832342715));
#46114=CARTESIAN_POINT('Ctrl Pts',(3.39918194578115,1.,2.33222789882601));
#46115=CARTESIAN_POINT('Ctrl Pts',(3.39513342020045,1.,2.32560343902683));
#46116=CARTESIAN_POINT('Ctrl Pts',(3.39105869475112,1.,2.31900513925627));
#46117=CARTESIAN_POINT('Ctrl Pts',(3.38695751492659,1.,2.31243319489505));
#46118=CARTESIAN_POINT('Ctrl Pts',(3.38282967336676,1.,2.30588783640389));
#46119=CARTESIAN_POINT('Ctrl Pts',(3.37867504959382,1.,2.29936936127588));
#46120=CARTESIAN_POINT('Ctrl Pts',(3.37449367172707,1.,2.2928781800731));
#46121=CARTESIAN_POINT('Ctrl Pts',(3.37028570206357,1.,2.28641481081045));
#46122=CARTESIAN_POINT('Ctrl Pts',(3.36605130712978,1.,2.27997979457968));
#46123=CARTESIAN_POINT('Ctrl Pts',(3.36179055004369,1.,2.27357362620902));
#46124=CARTESIAN_POINT('Ctrl Pts',(3.35750328523077,1.,2.26719668579921));
#46125=CARTESIAN_POINT('Ctrl Pts',(3.35318902552676,1.,2.26084915222484));
#46126=CARTESIAN_POINT('Ctrl Pts',(3.34884690292342,1.,2.25453097693524));
#46127=CARTESIAN_POINT('Ctrl Pts',(3.34447596770768,1.,2.24824207678288));
#46128=CARTESIAN_POINT('Ctrl Pts',(3.34007543738044,1.,2.24198249391437));
#46129=CARTESIAN_POINT('Ctrl Pts',(3.33564495756478,1.,2.2357525632881));
#46130=CARTESIAN_POINT('Ctrl Pts',(3.33118487773593,1.,2.22955308907221));
#46131=CARTESIAN_POINT('Ctrl Pts',(3.32669646722871,1.,2.22338548312759));
#46132=CARTESIAN_POINT('Ctrl Pts',(3.32218125618955,1.,2.21725135110889));
#46133=CARTESIAN_POINT('Ctrl Pts',(3.31764044024231,1.,2.21115211847872));
#46134=CARTESIAN_POINT('Ctrl Pts',(3.3130742460895,1.,2.20508863150608));
#46135=CARTESIAN_POINT('Ctrl Pts',(3.30848134694596,1.,2.19906078949925));
#46136=CARTESIAN_POINT('Ctrl Pts',(3.30385816281831,1.,2.19306710376112));
#46137=CARTESIAN_POINT('Ctrl Pts',(3.29920022557635,1.,2.18710556500325));
#46138=CARTESIAN_POINT('Ctrl Pts',(3.29450361500484,1.,2.18117455557062));
#46139=CARTESIAN_POINT('Ctrl Pts',(3.28976645712566,1.,2.17527380048422));
#46140=CARTESIAN_POINT('Ctrl Pts',(3.2849901997973,1.,2.16940517773459));
#46141=CARTESIAN_POINT('Ctrl Pts',(3.28018150841414,1.,2.16357391934434));
#46142=CARTESIAN_POINT('Ctrl Pts',(3.27534954469206,1.,2.15778690038359));
#46143=CARTESIAN_POINT('Ctrl Pts',(3.27050245897244,1.,2.15205043199818));
#46144=CARTESIAN_POINT('Ctrl Pts',(3.26564388189764,1.,2.14636805295663));
#46145=CARTESIAN_POINT('Ctrl Pts',(3.26077002641868,1.,2.14073870754258));
#46146=CARTESIAN_POINT('Ctrl Pts',(3.25586495065027,1.,2.13515375878786));
#46147=CARTESIAN_POINT('Ctrl Pts',(3.25090574493994,1.,2.1296002839681));
#46148=CARTESIAN_POINT('Ctrl Pts',(3.24587102613347,1.,2.12406646410943));
#46149=CARTESIAN_POINT('Ctrl Pts',(3.24074905517282,1.,2.11854673326972));
#46150=CARTESIAN_POINT('Ctrl Pts',(3.23554444767115,1.,2.11304604021784));
#46151=CARTESIAN_POINT('Ctrl Pts',(3.23028945793334,1.,2.1075869964248));
#46152=CARTESIAN_POINT('Ctrl Pts',(3.22503437553496,1.,2.10220384298534));
#46153=CARTESIAN_POINT('Ctrl Pts',(3.21982707347067,1.,2.09692958434933));
#46154=CARTESIAN_POINT('Ctrl Pts',(3.2146942960168,1.,2.0917841946046));
#46155=CARTESIAN_POINT('Ctrl Pts',(3.20962575845433,1.,2.08676465517435));
#46156=CARTESIAN_POINT('Ctrl Pts',(3.20454818630635,1.,2.08182850370816));
#46157=CARTESIAN_POINT('Ctrl Pts',(3.19934132835879,1.,2.0769044187063));
#46158=CARTESIAN_POINT('Ctrl Pts',(3.19388465568113,1.,2.07192253497765));
#46159=CARTESIAN_POINT('Ctrl Pts',(3.18809755562297,1.,2.06684062744065));
#46160=CARTESIAN_POINT('Ctrl Pts',(3.18197692964677,1.,2.06166849827143));
#46161=CARTESIAN_POINT('Ctrl Pts',(3.17564906975592,1.,2.05650186773279));
#46162=CARTESIAN_POINT('Ctrl Pts',(3.16936341689859,1.,2.05151770247452));
#46163=CARTESIAN_POINT('Ctrl Pts',(3.16343165059235,1.,2.0469333124766));
#46164=CARTESIAN_POINT('Ctrl Pts',(3.15817983946525,1.,2.04297406404132));
#46165=CARTESIAN_POINT('Ctrl Pts',(3.1538999167466,1.,2.03984073791432));
#46166=CARTESIAN_POINT('Ctrl Pts',(3.15102344775396,1.,2.03783225496023));
#46167=CARTESIAN_POINT('Ctrl Pts',(3.14959882629936,1.,2.03693188810614));
#46168=CARTESIAN_POINT('Ctrl Pts',(3.14901193669147,1.,2.03663974554941));
#46169=CARTESIAN_POINT('Ctrl Pts',(3.1488193908823,1.,2.03659701539175));
#46170=CARTESIAN_POINT('Ctrl Pts',(3.14877060440425,1.,2.03660101169564));
#46171=CARTESIAN_POINT('',(3.44202241512147,0.,2.40675750623143));
#46172=CARTESIAN_POINT('Ctrl Pts',(2.91001063062876,-1.,2.36523532225181));
#46173=CARTESIAN_POINT('Ctrl Pts',(2.91001063062876,1.,2.36523532225181));
#46174=CARTESIAN_POINT('Ctrl Pts',(2.90992398626211,-1.,2.36524348105112));
#46175=CARTESIAN_POINT('Ctrl Pts',(2.90992398626211,1.,2.36524348105112));
#46176=CARTESIAN_POINT('Ctrl Pts',(2.90989022548032,-1.,2.36535052956938));
#46177=CARTESIAN_POINT('Ctrl Pts',(2.90989022548032,1.,2.36535052956938));
#46178=CARTESIAN_POINT('Ctrl Pts',(2.91025813830041,-1.,2.36578327194741));
#46179=CARTESIAN_POINT('Ctrl Pts',(2.91025813830041,1.,2.36578327194741));
#46180=CARTESIAN_POINT('Ctrl Pts',(2.9115863784204,-1.,2.36690501170627));
#46181=CARTESIAN_POINT('Ctrl Pts',(2.9115863784204,1.,2.36690501170627));
#46182=CARTESIAN_POINT('Ctrl Pts',(2.9146124988314,-1.,2.36919161373173));
#46183=CARTESIAN_POINT('Ctrl Pts',(2.9146124988314,1.,2.36919161373173));
#46184=CARTESIAN_POINT('Ctrl Pts',(2.91891503791411,-1.,2.37229381109821));
#46185=CARTESIAN_POINT('Ctrl Pts',(2.91891503791411,1.,2.37229381109821));
#46186=CARTESIAN_POINT('Ctrl Pts',(2.92430340582608,-1.,2.3760651052403));
#46187=CARTESIAN_POINT('Ctrl Pts',(2.92430340582608,1.,2.3760651052403));
#46188=CARTESIAN_POINT('Ctrl Pts',(2.93049643640206,-1.,2.38028989582073));
#46189=CARTESIAN_POINT('Ctrl Pts',(2.93049643640206,1.,2.38028989582073));
#46190=CARTESIAN_POINT('Ctrl Pts',(2.93717903280391,-1.,2.38472771516311));
#46191=CARTESIAN_POINT('Ctrl Pts',(2.93717903280391,1.,2.38472771516311));
#46192=CARTESIAN_POINT('Ctrl Pts',(2.94404820669076,-1.,2.38914929090759));
#46193=CARTESIAN_POINT('Ctrl Pts',(2.94404820669076,1.,2.38914929090759));
#46194=CARTESIAN_POINT('Ctrl Pts',(2.95085857128439,-1.,2.39337207631667));
#46195=CARTESIAN_POINT('Ctrl Pts',(2.95085857128439,1.,2.39337207631667));
#46196=CARTESIAN_POINT('Ctrl Pts',(2.95748006482942,-1.,2.39730553974517));
#46197=CARTESIAN_POINT('Ctrl Pts',(2.95748006482942,1.,2.39730553974517));
#46198=CARTESIAN_POINT('Ctrl Pts',(2.96390432240312,-1.,2.4009556571164));
#46199=CARTESIAN_POINT('Ctrl Pts',(2.96390432240312,1.,2.4009556571164));
#46200=CARTESIAN_POINT('Ctrl Pts',(2.9701964131236,-1.,2.40438604734919));
#46201=CARTESIAN_POINT('Ctrl Pts',(2.9701964131236,1.,2.40438604734919));
#46202=CARTESIAN_POINT('Ctrl Pts',(2.97646002822422,-1.,2.40768975073713));
#46203=CARTESIAN_POINT('Ctrl Pts',(2.97646002822422,1.,2.40768975073713));
#46204=CARTESIAN_POINT('Ctrl Pts',(2.98280015815107,-1.,2.41095909342571));
#46205=CARTESIAN_POINT('Ctrl Pts',(2.98280015815107,1.,2.41095909342571));
#46206=CARTESIAN_POINT('Ctrl Pts',(2.98927983005796,-1.,2.41425064199586));
#46207=CARTESIAN_POINT('Ctrl Pts',(2.98927983005796,1.,2.41425064199586));
#46208=CARTESIAN_POINT('Ctrl Pts',(2.99590509293503,-1.,2.41757324500514));
#46209=CARTESIAN_POINT('Ctrl Pts',(2.99590509293503,1.,2.41757324500514));
#46210=CARTESIAN_POINT('Ctrl Pts',(3.00264868585996,-1.,2.42090763946779));
#46211=CARTESIAN_POINT('Ctrl Pts',(3.00264868585996,1.,2.42090763946779));
#46212=CARTESIAN_POINT('Ctrl Pts',(3.00946442616658,-1.,2.42421849439613));
#46213=CARTESIAN_POINT('Ctrl Pts',(3.00946442616658,1.,2.42421849439613));
#46214=CARTESIAN_POINT('Ctrl Pts',(3.01630420830504,-1.,2.42746856264168));
#46215=CARTESIAN_POINT('Ctrl Pts',(3.01630420830504,1.,2.42746856264168));
#46216=CARTESIAN_POINT('Ctrl Pts',(3.02313656036004,-1.,2.43063415586637));
#46217=CARTESIAN_POINT('Ctrl Pts',(3.02313656036004,1.,2.43063415586637));
#46218=CARTESIAN_POINT('Ctrl Pts',(3.02995534946978,-1.,2.43371241361488));
#46219=CARTESIAN_POINT('Ctrl Pts',(3.02995534946978,1.,2.43371241361488));
#46220=CARTESIAN_POINT('Ctrl Pts',(3.03676949672821,-1.,2.43671278042414));
#46221=CARTESIAN_POINT('Ctrl Pts',(3.03676949672821,1.,2.43671278042414));
#46222=CARTESIAN_POINT('Ctrl Pts',(3.04359685040555,-1.,2.43965194061857));
#46223=CARTESIAN_POINT('Ctrl Pts',(3.04359685040555,1.,2.43965194061857));
#46224=CARTESIAN_POINT('Ctrl Pts',(3.05045678021504,-1.,2.44254768923105));
#46225=CARTESIAN_POINT('Ctrl Pts',(3.05045678021504,1.,2.44254768923105));
#46226=CARTESIAN_POINT('Ctrl Pts',(3.05736242671506,-1.,2.44541251892556));
#46227=CARTESIAN_POINT('Ctrl Pts',(3.05736242671506,1.,2.44541251892556));
#46228=CARTESIAN_POINT('Ctrl Pts',(3.06431596421405,-1.,2.44824970516544));
#46229=CARTESIAN_POINT('Ctrl Pts',(3.06431596421405,1.,2.44824970516544));
#46230=CARTESIAN_POINT('Ctrl Pts',(3.07131290521297,-1.,2.45105688854422));
#46231=CARTESIAN_POINT('Ctrl Pts',(3.07131290521297,1.,2.45105688854422));
#46232=CARTESIAN_POINT('Ctrl Pts',(3.07834472886139,-1.,2.4538282678779));
#46233=CARTESIAN_POINT('Ctrl Pts',(3.07834472886139,1.,2.4538282678779));
#46234=CARTESIAN_POINT('Ctrl Pts',(3.08540206545315,-1.,2.45655725437039));
#46235=CARTESIAN_POINT('Ctrl Pts',(3.08540206545315,1.,2.45655725437039));
#46236=CARTESIAN_POINT('Ctrl Pts',(3.09247787931887,-1.,2.4592391256388));
#46237=CARTESIAN_POINT('Ctrl Pts',(3.09247787931887,1.,2.4592391256388));
#46238=CARTESIAN_POINT('Ctrl Pts',(3.09956993697052,-1.,2.46187308501884));
#46239=CARTESIAN_POINT('Ctrl Pts',(3.09956993697052,1.,2.46187308501884));
#46240=CARTESIAN_POINT('Ctrl Pts',(3.1066790790198,-1.,2.46446082979646));
#46241=CARTESIAN_POINT('Ctrl Pts',(3.1066790790198,1.,2.46446082979646));
#46242=CARTESIAN_POINT('Ctrl Pts',(3.11380805536122,-1.,2.46700558843506));
#46243=CARTESIAN_POINT('Ctrl Pts',(3.11380805536122,1.,2.46700558843506));
#46244=CARTESIAN_POINT('Ctrl Pts',(3.12096015766983,-1.,2.46951098947469));
#46245=CARTESIAN_POINT('Ctrl Pts',(3.12096015766983,1.,2.46951098947469));
#46246=CARTESIAN_POINT('Ctrl Pts',(3.12813790805952,-1.,2.47197997765871));
#46247=CARTESIAN_POINT('Ctrl Pts',(3.12813790805952,1.,2.47197997765871));
#46248=CARTESIAN_POINT('Ctrl Pts',(3.13534181229295,-1.,2.47441378371932));
#46249=CARTESIAN_POINT('Ctrl Pts',(3.13534181229295,1.,2.47441378371932));
#46250=CARTESIAN_POINT('Ctrl Pts',(3.1425709954655,-1.,2.47681245356109));
#46251=CARTESIAN_POINT('Ctrl Pts',(3.1425709954655,1.,2.47681245356109));
#46252=CARTESIAN_POINT('Ctrl Pts',(3.14982373241352,-1.,2.47917529057029));
#46253=CARTESIAN_POINT('Ctrl Pts',(3.14982373241352,1.,2.47917529057029));
#46254=CARTESIAN_POINT('Ctrl Pts',(3.15709802322739,-1.,2.48150133566571));
#46255=CARTESIAN_POINT('Ctrl Pts',(3.15709802322739,1.,2.48150133566571));
#46256=CARTESIAN_POINT('Ctrl Pts',(3.16439213290161,-1.,2.48378981792725));
#46257=CARTESIAN_POINT('Ctrl Pts',(3.16439213290161,1.,2.48378981792725));
#46258=CARTESIAN_POINT('Ctrl Pts',(3.17170518863313,-1.,2.48604065348587));
#46259=CARTESIAN_POINT('Ctrl Pts',(3.17170518863313,1.,2.48604065348587));
#46260=CARTESIAN_POINT('Ctrl Pts',(3.17903698136622,-1.,2.48825428288201));
#46261=CARTESIAN_POINT('Ctrl Pts',(3.17903698136622,1.,2.48825428288201));
#46262=CARTESIAN_POINT('Ctrl Pts',(3.18638771282266,-1.,2.49043146334059));
#46263=CARTESIAN_POINT('Ctrl Pts',(3.18638771282266,1.,2.49043146334059));
#46264=CARTESIAN_POINT('Ctrl Pts',(3.19375775555798,-1.,2.49257307239848));
#46265=CARTESIAN_POINT('Ctrl Pts',(3.19375775555798,1.,2.49257307239848));
#46266=CARTESIAN_POINT('Ctrl Pts',(3.20114742397588,-1.,2.49467992057755));
#46267=CARTESIAN_POINT('Ctrl Pts',(3.20114742397588,1.,2.49467992057755));
#46268=CARTESIAN_POINT('Ctrl Pts',(3.20855669849836,-1.,2.4967525264737));
#46269=CARTESIAN_POINT('Ctrl Pts',(3.20855669849836,1.,2.4967525264737));
#46270=CARTESIAN_POINT('Ctrl Pts',(3.21598526261286,-1.,2.4987911459939));
#46271=CARTESIAN_POINT('Ctrl Pts',(3.21598526261286,1.,2.4987911459939));
#46272=CARTESIAN_POINT('Ctrl Pts',(3.22343262620503,-1.,2.50079587201958));
#46273=CARTESIAN_POINT('Ctrl Pts',(3.22343262620503,1.,2.50079587201958));
#46274=CARTESIAN_POINT('Ctrl Pts',(3.23089822320646,-1.,2.50276671338111));
#46275=CARTESIAN_POINT('Ctrl Pts',(3.23089822320646,1.,2.50276671338111));
#46276=CARTESIAN_POINT('Ctrl Pts',(3.23838151080319,-1.,2.5047036758003));
#46277=CARTESIAN_POINT('Ctrl Pts',(3.23838151080319,1.,2.5047036758003));
#46278=CARTESIAN_POINT('Ctrl Pts',(3.24588208983849,-1.,2.506606859405));
#46279=CARTESIAN_POINT('Ctrl Pts',(3.24588208983849,1.,2.506606859405));
#46280=CARTESIAN_POINT('Ctrl Pts',(3.25339971460982,-1.,2.50847647070723));
#46281=CARTESIAN_POINT('Ctrl Pts',(3.25339971460982,1.,2.50847647070723));
#46282=CARTESIAN_POINT('Ctrl Pts',(3.26093423001434,-1.,2.51031277813486));
#46283=CARTESIAN_POINT('Ctrl Pts',(3.26093423001434,1.,2.51031277813486));
#46284=CARTESIAN_POINT('Ctrl Pts',(3.26848552888115,-1.,2.51211608411423));
#46285=CARTESIAN_POINT('Ctrl Pts',(3.26848552888115,1.,2.51211608411423));
#46286=CARTESIAN_POINT('Ctrl Pts',(3.27605350473142,-1.,2.513886692704));
#46287=CARTESIAN_POINT('Ctrl Pts',(3.27605350473142,1.,2.513886692704));
#46288=CARTESIAN_POINT('Ctrl Pts',(3.28363799702982,-1.,2.51562487464514));
#46289=CARTESIAN_POINT('Ctrl Pts',(3.28363799702982,1.,2.51562487464514));
#46290=CARTESIAN_POINT('Ctrl Pts',(3.2912387729927,-1.,2.51733085123797));
#46291=CARTESIAN_POINT('Ctrl Pts',(3.2912387729927,1.,2.51733085123797));
#46292=CARTESIAN_POINT('Ctrl Pts',(3.29885556388352,-1.,2.51900480701069));
#46293=CARTESIAN_POINT('Ctrl Pts',(3.29885556388352,1.,2.51900480701069));
#46294=CARTESIAN_POINT('Ctrl Pts',(3.30648808815442,-1.,2.52064689568511));
#46295=CARTESIAN_POINT('Ctrl Pts',(3.30648808815442,1.,2.52064689568511));
#46296=CARTESIAN_POINT('Ctrl Pts',(3.31413607874645,-1.,2.52225724871313));
#46297=CARTESIAN_POINT('Ctrl Pts',(3.31413607874645,1.,2.52225724871313));
#46298=CARTESIAN_POINT('Ctrl Pts',(3.32179931078699,-1.,2.5238359839626));
#46299=CARTESIAN_POINT('Ctrl Pts',(3.32179931078699,1.,2.5238359839626));
#46300=CARTESIAN_POINT('Ctrl Pts',(3.32947762187533,-1.,2.52538321164634));
#46301=CARTESIAN_POINT('Ctrl Pts',(3.32947762187533,1.,2.52538321164634));
#46302=CARTESIAN_POINT('Ctrl Pts',(3.33717089999103,-1.,2.52689902690158));
#46303=CARTESIAN_POINT('Ctrl Pts',(3.33717089999103,1.,2.52689902690158));
#46304=CARTESIAN_POINT('Ctrl Pts',(3.34333744115511,-1.,2.52808660915689));
#46305=CARTESIAN_POINT('Ctrl Pts',(3.34333744115511,1.,2.52808660915689));
#46306=CARTESIAN_POINT('Ctrl Pts',(3.34796903576663,-1.,2.52896321610703));
#46307=CARTESIAN_POINT('Ctrl Pts',(3.34796903576663,1.,2.52896321610703));
#46308=CARTESIAN_POINT('Ctrl Pts',(3.35105973714071,-1.,2.5295413654909));
#46309=CARTESIAN_POINT('Ctrl Pts',(3.35105973714071,1.,2.5295413654909));
#46310=CARTESIAN_POINT('Ctrl Pts',(3.35260583073571,-1.,2.52982887637028));
#46311=CARTESIAN_POINT('Ctrl Pts',(3.35260583073571,1.,2.52982887637028));
#46312=CARTESIAN_POINT('',(2.90994629141676,1.,2.36531447826073));
#46313=CARTESIAN_POINT('Ctrl Pts',(2.90994629141676,-1.,2.36531447826073));
#46314=CARTESIAN_POINT('Ctrl Pts',(2.90994629141676,-0.666666666666667,
2.36531447826073));
#46315=CARTESIAN_POINT('Ctrl Pts',(2.90994629141676,-0.333333333333333,
2.36531447826073));
#46316=CARTESIAN_POINT('Ctrl Pts',(2.90994629141676,0.333333333333333,2.36531447826073));
#46317=CARTESIAN_POINT('Ctrl Pts',(2.90994629141676,0.666666666666667,2.36531447826073));
#46318=CARTESIAN_POINT('Ctrl Pts',(2.90994629141676,1.,2.36531447826073));
#46319=CARTESIAN_POINT('',(3.35260583073571,1.,2.52982887637028));
#46320=CARTESIAN_POINT('',(3.35260583073571,0.,2.52982887637028));
#46321=CARTESIAN_POINT('Ctrl Pts',(2.90994629141676,1.,2.36531447826073));
#46322=CARTESIAN_POINT('Ctrl Pts',(2.90995756655606,1.,2.36536211188453));
#46323=CARTESIAN_POINT('Ctrl Pts',(2.91005770527719,1.,2.36553202948613));
#46324=CARTESIAN_POINT('Ctrl Pts',(2.91051690822156,1.,2.36599991765749));
#46325=CARTESIAN_POINT('Ctrl Pts',(2.91181344022548,1.,2.36707658451664));
#46326=CARTESIAN_POINT('Ctrl Pts',(2.9146124988314,1.,2.36919161373173));
#46327=CARTESIAN_POINT('Ctrl Pts',(2.91891503791411,1.,2.37229381109821));
#46328=CARTESIAN_POINT('Ctrl Pts',(2.92430340582608,1.,2.3760651052403));
#46329=CARTESIAN_POINT('Ctrl Pts',(2.93049643640206,1.,2.38028989582073));
#46330=CARTESIAN_POINT('Ctrl Pts',(2.93717903280391,1.,2.38472771516311));
#46331=CARTESIAN_POINT('Ctrl Pts',(2.94404820669076,1.,2.38914929090759));
#46332=CARTESIAN_POINT('Ctrl Pts',(2.95085857128439,1.,2.39337207631667));
#46333=CARTESIAN_POINT('Ctrl Pts',(2.95748006482942,1.,2.39730553974517));
#46334=CARTESIAN_POINT('Ctrl Pts',(2.96390432240312,1.,2.4009556571164));
#46335=CARTESIAN_POINT('Ctrl Pts',(2.9701964131236,1.,2.40438604734919));
#46336=CARTESIAN_POINT('Ctrl Pts',(2.97646002822422,1.,2.40768975073713));
#46337=CARTESIAN_POINT('Ctrl Pts',(2.98280015815107,1.,2.41095909342571));
#46338=CARTESIAN_POINT('Ctrl Pts',(2.98927983005796,1.,2.41425064199586));
#46339=CARTESIAN_POINT('Ctrl Pts',(2.99590509293503,1.,2.41757324500514));
#46340=CARTESIAN_POINT('Ctrl Pts',(3.00264868585996,1.,2.42090763946779));
#46341=CARTESIAN_POINT('Ctrl Pts',(3.00946442616658,1.,2.42421849439613));
#46342=CARTESIAN_POINT('Ctrl Pts',(3.01630420830504,1.,2.42746856264168));
#46343=CARTESIAN_POINT('Ctrl Pts',(3.02313656036004,1.,2.43063415586637));
#46344=CARTESIAN_POINT('Ctrl Pts',(3.02995534946978,1.,2.43371241361488));
#46345=CARTESIAN_POINT('Ctrl Pts',(3.03676949672821,1.,2.43671278042414));
#46346=CARTESIAN_POINT('Ctrl Pts',(3.04359685040555,1.,2.43965194061857));
#46347=CARTESIAN_POINT('Ctrl Pts',(3.05045678021504,1.,2.44254768923105));
#46348=CARTESIAN_POINT('Ctrl Pts',(3.05736242671506,1.,2.44541251892556));
#46349=CARTESIAN_POINT('Ctrl Pts',(3.06431596421405,1.,2.44824970516544));
#46350=CARTESIAN_POINT('Ctrl Pts',(3.07131290521297,1.,2.45105688854422));
#46351=CARTESIAN_POINT('Ctrl Pts',(3.07834472886139,1.,2.4538282678779));
#46352=CARTESIAN_POINT('Ctrl Pts',(3.08540206545315,1.,2.45655725437039));
#46353=CARTESIAN_POINT('Ctrl Pts',(3.09247787931887,1.,2.4592391256388));
#46354=CARTESIAN_POINT('Ctrl Pts',(3.09956993697052,1.,2.46187308501884));
#46355=CARTESIAN_POINT('Ctrl Pts',(3.1066790790198,1.,2.46446082979646));
#46356=CARTESIAN_POINT('Ctrl Pts',(3.11380805536122,1.,2.46700558843506));
#46357=CARTESIAN_POINT('Ctrl Pts',(3.12096015766983,1.,2.46951098947469));
#46358=CARTESIAN_POINT('Ctrl Pts',(3.12813790805952,1.,2.47197997765871));
#46359=CARTESIAN_POINT('Ctrl Pts',(3.13534181229295,1.,2.47441378371932));
#46360=CARTESIAN_POINT('Ctrl Pts',(3.1425709954655,1.,2.47681245356109));
#46361=CARTESIAN_POINT('Ctrl Pts',(3.14982373241352,1.,2.47917529057029));
#46362=CARTESIAN_POINT('Ctrl Pts',(3.15709802322739,1.,2.48150133566571));
#46363=CARTESIAN_POINT('Ctrl Pts',(3.16439213290161,1.,2.48378981792725));
#46364=CARTESIAN_POINT('Ctrl Pts',(3.17170518863313,1.,2.48604065348587));
#46365=CARTESIAN_POINT('Ctrl Pts',(3.17903698136622,1.,2.48825428288201));
#46366=CARTESIAN_POINT('Ctrl Pts',(3.18638771282266,1.,2.49043146334059));
#46367=CARTESIAN_POINT('Ctrl Pts',(3.19375775555798,1.,2.49257307239848));
#46368=CARTESIAN_POINT('Ctrl Pts',(3.20114742397588,1.,2.49467992057755));
#46369=CARTESIAN_POINT('Ctrl Pts',(3.20855669849836,1.,2.4967525264737));
#46370=CARTESIAN_POINT('Ctrl Pts',(3.21598526261286,1.,2.4987911459939));
#46371=CARTESIAN_POINT('Ctrl Pts',(3.22343262620503,1.,2.50079587201958));
#46372=CARTESIAN_POINT('Ctrl Pts',(3.23089822320646,1.,2.50276671338111));
#46373=CARTESIAN_POINT('Ctrl Pts',(3.23838151080319,1.,2.5047036758003));
#46374=CARTESIAN_POINT('Ctrl Pts',(3.24588208983849,1.,2.506606859405));
#46375=CARTESIAN_POINT('Ctrl Pts',(3.25339971460982,1.,2.50847647070723));
#46376=CARTESIAN_POINT('Ctrl Pts',(3.26093423001434,1.,2.51031277813486));
#46377=CARTESIAN_POINT('Ctrl Pts',(3.26848552888115,1.,2.51211608411423));
#46378=CARTESIAN_POINT('Ctrl Pts',(3.27605350473142,1.,2.513886692704));
#46379=CARTESIAN_POINT('Ctrl Pts',(3.28363799702982,1.,2.51562487464514));
#46380=CARTESIAN_POINT('Ctrl Pts',(3.2912387729927,1.,2.51733085123797));
#46381=CARTESIAN_POINT('Ctrl Pts',(3.29885556388352,1.,2.51900480701069));
#46382=CARTESIAN_POINT('Ctrl Pts',(3.30648808815442,1.,2.52064689568511));
#46383=CARTESIAN_POINT('Ctrl Pts',(3.31413607874645,1.,2.52225724871313));
#46384=CARTESIAN_POINT('Ctrl Pts',(3.32179931078699,1.,2.5238359839626));
#46385=CARTESIAN_POINT('Ctrl Pts',(3.32947762187533,1.,2.52538321164634));
#46386=CARTESIAN_POINT('Ctrl Pts',(3.33717089999103,1.,2.52689902690158));
#46387=CARTESIAN_POINT('Ctrl Pts',(3.34333744115511,1.,2.52808660915689));
#46388=CARTESIAN_POINT('Ctrl Pts',(3.34796903576663,1.,2.52896321610703));
#46389=CARTESIAN_POINT('Ctrl Pts',(3.35105973714071,1.,2.5295413654909));
#46390=CARTESIAN_POINT('Ctrl Pts',(3.35260583073571,1.,2.52982887637028));
#46391=CARTESIAN_POINT('Origin',(3.35260583073571,0.,2.52982887637028));
#46392=CARTESIAN_POINT('',(3.44202241512147,1.,2.40675750623143));
#46393=CARTESIAN_POINT('Origin',(0.,0.,0.));
#46394=CARTESIAN_POINT('',(2.79140942341378,1.,2.50410331873042));
#46395=CARTESIAN_POINT('Origin',(0.,1.,0.));
#46396=CARTESIAN_POINT('Ctrl Pts',(2.79140942341378,1.,2.50410331873043));
#46397=CARTESIAN_POINT('Ctrl Pts',(2.79140942341378,0.666666666666667,2.50410331873043));
#46398=CARTESIAN_POINT('Ctrl Pts',(2.79140942341378,0.333333333333333,2.50410331873042));
#46399=CARTESIAN_POINT('Ctrl Pts',(2.79140942341378,-0.333333333333333,
2.50410331873042));
#46400=CARTESIAN_POINT('Ctrl Pts',(2.79140942341378,-0.666666666666667,
2.50410331873042));
#46401=CARTESIAN_POINT('Ctrl Pts',(2.79140942341378,-1.,2.50410331873042));
#46402=CARTESIAN_POINT('Ctrl Pts',(3.02314558451372,-1.,2.91557726271063));
#46403=CARTESIAN_POINT('Ctrl Pts',(3.02314558451372,1.,2.91557726271063));
#46404=CARTESIAN_POINT('Ctrl Pts',(3.02261975104912,-1.,2.91409518070707));
#46405=CARTESIAN_POINT('Ctrl Pts',(3.02261975104912,1.,2.91409518070707));
#46406=CARTESIAN_POINT('Ctrl Pts',(3.02156522743299,-1.,2.91113297349052));
#46407=CARTESIAN_POINT('Ctrl Pts',(3.02156522743299,1.,2.91113297349052));
#46408=CARTESIAN_POINT('Ctrl Pts',(3.01997487194926,-1.,2.90669553303902));
#46409=CARTESIAN_POINT('Ctrl Pts',(3.01997487194926,1.,2.90669553303902));
#46410=CARTESIAN_POINT('Ctrl Pts',(3.01783725123646,-1.,2.90079069102661));
#46411=CARTESIAN_POINT('Ctrl Pts',(3.01783725123646,1.,2.90079069102661));
#46412=CARTESIAN_POINT('Ctrl Pts',(3.01513660433291,-1.,2.8934292556764));
#46413=CARTESIAN_POINT('Ctrl Pts',(3.01513660433291,1.,2.8934292556764));
#46414=CARTESIAN_POINT('Ctrl Pts',(3.01240727309568,-1.,2.88608751706796));
#46415=CARTESIAN_POINT('Ctrl Pts',(3.01240727309568,1.,2.88608751706796));
#46416=CARTESIAN_POINT('Ctrl Pts',(3.0096491810855,-1.,2.87876560072799));
#46417=CARTESIAN_POINT('Ctrl Pts',(3.0096491810855,1.,2.87876560072799));
#46418=CARTESIAN_POINT('Ctrl Pts',(3.00686224485374,-1.,2.87146368430104));
#46419=CARTESIAN_POINT('Ctrl Pts',(3.00686224485374,1.,2.87146368430104));
#46420=CARTESIAN_POINT('Ctrl Pts',(3.00404638316245,-1.,2.86418200833065));
#46421=CARTESIAN_POINT('Ctrl Pts',(3.00404638316245,1.,2.86418200833065));
#46422=CARTESIAN_POINT('Ctrl Pts',(3.0012015079552,-1.,2.85692085715129));
#46423=CARTESIAN_POINT('Ctrl Pts',(3.0012015079552,1.,2.85692085715129));
#46424=CARTESIAN_POINT('Ctrl Pts',(2.99832751144566,-1.,2.84968053289104));
#46425=CARTESIAN_POINT('Ctrl Pts',(2.99832751144566,1.,2.84968053289104));
#46426=CARTESIAN_POINT('Ctrl Pts',(2.995424253416,-1.,2.84246132984334));
#46427=CARTESIAN_POINT('Ctrl Pts',(2.995424253416,1.,2.84246132984334));
#46428=CARTESIAN_POINT('Ctrl Pts',(2.99249155170479,-1.,2.83526351254383));
#46429=CARTESIAN_POINT('Ctrl Pts',(2.99249155170479,1.,2.83526351254383));
#46430=CARTESIAN_POINT('Ctrl Pts',(2.98952916401699,-1.,2.82808728190402));
#46431=CARTESIAN_POINT('Ctrl Pts',(2.98952916401699,1.,2.82808728190402));
#46432=CARTESIAN_POINT('Ctrl Pts',(2.98653680669434,-1.,2.82093279065704));
#46433=CARTESIAN_POINT('Ctrl Pts',(2.98653680669434,1.,2.82093279065704));
#46434=CARTESIAN_POINT('Ctrl Pts',(2.9835141977994,-1.,2.81380019196454));
#46435=CARTESIAN_POINT('Ctrl Pts',(2.9835141977994,1.,2.81380019196454));
#46436=CARTESIAN_POINT('Ctrl Pts',(2.98046109647299,-1.,2.80668968101162));
#46437=CARTESIAN_POINT('Ctrl Pts',(2.98046109647299,1.,2.80668968101162));
#46438=CARTESIAN_POINT('Ctrl Pts',(2.97737733718242,-1.,2.79960153278186));
#46439=CARTESIAN_POINT('Ctrl Pts',(2.97737733718242,1.,2.79960153278186));
#46440=CARTESIAN_POINT('Ctrl Pts',(2.97426288347475,-1.,2.79253615718147));
#46441=CARTESIAN_POINT('Ctrl Pts',(2.97426288347475,1.,2.79253615718147));
#46442=CARTESIAN_POINT('Ctrl Pts',(2.97111781461349,-1.,2.78549409123657));
#46443=CARTESIAN_POINT('Ctrl Pts',(2.97111781461349,1.,2.78549409123657));
#46444=CARTESIAN_POINT('Ctrl Pts',(2.9679422104295,-1.,2.77847589542767));
#46445=CARTESIAN_POINT('Ctrl Pts',(2.9679422104295,1.,2.77847589542767));
#46446=CARTESIAN_POINT('Ctrl Pts',(2.96473605585548,-1.,2.77148206836464));
#46447=CARTESIAN_POINT('Ctrl Pts',(2.96473605585548,1.,2.77148206836464));
#46448=CARTESIAN_POINT('Ctrl Pts',(2.96149914764832,-1.,2.76451296269571));
#46449=CARTESIAN_POINT('Ctrl Pts',(2.96149914764832,1.,2.76451296269571));
#46450=CARTESIAN_POINT('Ctrl Pts',(2.9582309766594,-1.,2.75756867888393));
#46451=CARTESIAN_POINT('Ctrl Pts',(2.9582309766594,1.,2.75756867888393));
#46452=CARTESIAN_POINT('Ctrl Pts',(2.95493069316211,-1.,2.75064903318996));
#46453=CARTESIAN_POINT('Ctrl Pts',(2.95493069316211,1.,2.75064903318996));
#46454=CARTESIAN_POINT('Ctrl Pts',(2.95159737214304,-1.,2.7437537949221));
#46455=CARTESIAN_POINT('Ctrl Pts',(2.95159737214304,1.,2.7437537949221));
#46456=CARTESIAN_POINT('Ctrl Pts',(2.94823023414381,-1.,2.73688288329825));
#46457=CARTESIAN_POINT('Ctrl Pts',(2.94823023414381,1.,2.73688288329825));
#46458=CARTESIAN_POINT('Ctrl Pts',(2.94482887675139,-1.,2.73003657371613));
#46459=CARTESIAN_POINT('Ctrl Pts',(2.94482887675139,1.,2.73003657371613));
#46460=CARTESIAN_POINT('Ctrl Pts',(2.94139351933882,-1.,2.72321571511322));
#46461=CARTESIAN_POINT('Ctrl Pts',(2.94139351933882,1.,2.72321571511322));
#46462=CARTESIAN_POINT('Ctrl Pts',(2.93792519474955,-1.,2.71642190053575));
#46463=CARTESIAN_POINT('Ctrl Pts',(2.93792519474955,1.,2.71642190053575));
#46464=CARTESIAN_POINT('Ctrl Pts',(2.93442516311167,-1.,2.70965695523776));
#46465=CARTESIAN_POINT('Ctrl Pts',(2.93442516311167,1.,2.70965695523776));
#46466=CARTESIAN_POINT('Ctrl Pts',(2.93089438233746,-1.,2.70292247416881));
#46467=CARTESIAN_POINT('Ctrl Pts',(2.93089438233746,1.,2.70292247416881));
#46468=CARTESIAN_POINT('Ctrl Pts',(2.92733294395268,-1.,2.69621932864302));
#46469=CARTESIAN_POINT('Ctrl Pts',(2.92733294395268,1.,2.69621932864302));
#46470=CARTESIAN_POINT('Ctrl Pts',(2.92373955325876,-1.,2.68954721165342));
#46471=CARTESIAN_POINT('Ctrl Pts',(2.92373955325876,1.,2.68954721165342));
#46472=CARTESIAN_POINT('Ctrl Pts',(2.92011090722152,-1.,2.68290409279689));
#46473=CARTESIAN_POINT('Ctrl Pts',(2.92011090722152,1.,2.68290409279689));
#46474=CARTESIAN_POINT('Ctrl Pts',(2.91644290704281,-1.,2.67628728855309));
#46475=CARTESIAN_POINT('Ctrl Pts',(2.91644290704281,1.,2.67628728855309));
#46476=CARTESIAN_POINT('Ctrl Pts',(2.91273193382876,-1.,2.66969458792627));
#46477=CARTESIAN_POINT('Ctrl Pts',(2.91273193382876,1.,2.66969458792627));
#46478=CARTESIAN_POINT('Ctrl Pts',(2.90897617968921,-1.,2.66312542616809));
#46479=CARTESIAN_POINT('Ctrl Pts',(2.90897617968921,1.,2.66312542616809));
#46480=CARTESIAN_POINT('Ctrl Pts',(2.90517678087467,-1.,2.65658188464287));
#46481=CARTESIAN_POINT('Ctrl Pts',(2.90517678087467,1.,2.65658188464287));
#46482=CARTESIAN_POINT('Ctrl Pts',(2.90133950224879,-1.,2.65007017365576));
#46483=CARTESIAN_POINT('Ctrl Pts',(2.90133950224879,1.,2.65007017365576));
#46484=CARTESIAN_POINT('Ctrl Pts',(2.89747231723361,-1.,2.64359851684146));
#46485=CARTESIAN_POINT('Ctrl Pts',(2.89747231723361,1.,2.64359851684146));
#46486=CARTESIAN_POINT('Ctrl Pts',(2.89358228854557,-1.,2.63717442263944));
#46487=CARTESIAN_POINT('Ctrl Pts',(2.89358228854557,1.,2.63717442263944));
#46488=CARTESIAN_POINT('Ctrl Pts',(2.88967244854243,-1.,2.63080195420771));
#46489=CARTESIAN_POINT('Ctrl Pts',(2.88967244854243,1.,2.63080195420771));
#46490=CARTESIAN_POINT('Ctrl Pts',(2.88573922195049,-1.,2.62447947640253));
#46491=CARTESIAN_POINT('Ctrl Pts',(2.88573922195049,1.,2.62447947640253));
#46492=CARTESIAN_POINT('Ctrl Pts',(2.88176821427502,-1.,2.61819596473087));
#46493=CARTESIAN_POINT('Ctrl Pts',(2.88176821427502,1.,2.61819596473087));
#46494=CARTESIAN_POINT('Ctrl Pts',(2.87773881947885,-1.,2.61193507170928));
#46495=CARTESIAN_POINT('Ctrl Pts',(2.87773881947885,1.,2.61193507170928));
#46496=CARTESIAN_POINT('Ctrl Pts',(2.87363176656475,-1.,2.6056817788128));
#46497=CARTESIAN_POINT('Ctrl Pts',(2.87363176656475,1.,2.6056817788128));
#46498=CARTESIAN_POINT('Ctrl Pts',(2.86943633170712,-1.,2.59942875223202));
#46499=CARTESIAN_POINT('Ctrl Pts',(2.86943633170712,1.,2.59942875223202));
#46500=CARTESIAN_POINT('Ctrl Pts',(2.86515629953528,-1.,2.59318160184921));
#46501=CARTESIAN_POINT('Ctrl Pts',(2.86515629953528,1.,2.59318160184921));
#46502=CARTESIAN_POINT('Ctrl Pts',(2.86081999003668,-1.,2.5869677064356));
#46503=CARTESIAN_POINT('Ctrl Pts',(2.86081999003668,1.,2.5869677064356));
#46504=CARTESIAN_POINT('Ctrl Pts',(2.85647171715147,-1.,2.58082875254407));
#46505=CARTESIAN_POINT('Ctrl Pts',(2.85647171715147,1.,2.58082875254407));
#46506=CARTESIAN_POINT('Ctrl Pts',(2.85215360144482,-1.,2.57480482727128));
#46507=CARTESIAN_POINT('Ctrl Pts',(2.85215360144482,1.,2.57480482727128));
#46508=CARTESIAN_POINT('Ctrl Pts',(2.84788893329091,-1.,2.56891984251743));
#46509=CARTESIAN_POINT('Ctrl Pts',(2.84788893329091,1.,2.56891984251743));
#46510=CARTESIAN_POINT('Ctrl Pts',(2.84366802680211,-1.,2.56316920798489));
#46511=CARTESIAN_POINT('Ctrl Pts',(2.84366802680211,1.,2.56316920798489));
#46512=CARTESIAN_POINT('Ctrl Pts',(2.83942515220699,-1.,2.55749952145165));
#46513=CARTESIAN_POINT('Ctrl Pts',(2.83942515220699,1.,2.55749952145165));
#46514=CARTESIAN_POINT('Ctrl Pts',(2.83505269592412,-1.,2.55182152806964));
#46515=CARTESIAN_POINT('Ctrl Pts',(2.83505269592412,1.,2.55182152806964));
#46516=CARTESIAN_POINT('Ctrl Pts',(2.83044254225794,-1.,2.54604736792542));
#46517=CARTESIAN_POINT('Ctrl Pts',(2.83044254225794,1.,2.54604736792542));
#46518=CARTESIAN_POINT('Ctrl Pts',(2.82552167649157,-1.,2.54012272520141));
#46519=CARTESIAN_POINT('Ctrl Pts',(2.82552167649157,1.,2.54012272520141));
#46520=CARTESIAN_POINT('Ctrl Pts',(2.82028550483744,-1.,2.53405679667463));
#46521=CARTESIAN_POINT('Ctrl Pts',(2.82028550483744,1.,2.53405679667463));
#46522=CARTESIAN_POINT('Ctrl Pts',(2.8148437904867,-1.,2.52796388055457));
#46523=CARTESIAN_POINT('Ctrl Pts',(2.8148437904867,1.,2.52796388055457));
#46524=CARTESIAN_POINT('Ctrl Pts',(2.80941521967234,-1.,2.52205778589922));
#46525=CARTESIAN_POINT('Ctrl Pts',(2.80941521967234,1.,2.52205778589922));
#46526=CARTESIAN_POINT('Ctrl Pts',(2.80427363984939,-1.,2.51660190466067));
#46527=CARTESIAN_POINT('Ctrl Pts',(2.80427363984939,1.,2.51660190466067));
#46528=CARTESIAN_POINT('Ctrl Pts',(2.79970585014308,-1.,2.51186983687947));
#46529=CARTESIAN_POINT('Ctrl Pts',(2.79970585014308,1.,2.51186983687947));
#46530=CARTESIAN_POINT('Ctrl Pts',(2.7959687805717,-1.,2.50810555977564));
#46531=CARTESIAN_POINT('Ctrl Pts',(2.7959687805717,1.,2.50810555977564));
#46532=CARTESIAN_POINT('Ctrl Pts',(2.79323694088143,-1.,2.50547439929077));
#46533=CARTESIAN_POINT('Ctrl Pts',(2.79323694088143,1.,2.50547439929077));
#46534=CARTESIAN_POINT('Ctrl Pts',(2.79192122906739,-1.,2.50433799076945));
#46535=CARTESIAN_POINT('Ctrl Pts',(2.79192122906739,1.,2.50433799076945));
#46536=CARTESIAN_POINT('Ctrl Pts',(2.79143626022225,-1.,2.50404230339032));
#46537=CARTESIAN_POINT('Ctrl Pts',(2.79143626022225,1.,2.50404230339032));
#46538=CARTESIAN_POINT('Ctrl Pts',(2.79133581100044,-1.,2.50409239460011));
#46539=CARTESIAN_POINT('Ctrl Pts',(2.79133581100044,1.,2.50409239460011));
#46540=CARTESIAN_POINT('Ctrl Pts',(2.79134130681569,-1.,2.50417924854921));
#46541=CARTESIAN_POINT('Ctrl Pts',(2.79134130681569,1.,2.50417924854921));
#46542=CARTESIAN_POINT('',(3.02314558451372,1.,2.91557726271063));
#46543=CARTESIAN_POINT('Ctrl Pts',(3.02314558451372,1.,2.91557726271063));
#46544=CARTESIAN_POINT('Ctrl Pts',(3.02261975104912,1.,2.91409518070707));
#46545=CARTESIAN_POINT('Ctrl Pts',(3.02156522743299,1.,2.91113297349052));
#46546=CARTESIAN_POINT('Ctrl Pts',(3.01997487194926,1.,2.90669553303902));
#46547=CARTESIAN_POINT('Ctrl Pts',(3.01783725123646,1.,2.90079069102661));
#46548=CARTESIAN_POINT('Ctrl Pts',(3.01513660433291,1.,2.8934292556764));
#46549=CARTESIAN_POINT('Ctrl Pts',(3.01240727309568,1.,2.88608751706796));
#46550=CARTESIAN_POINT('Ctrl Pts',(3.0096491810855,1.,2.87876560072799));
#46551=CARTESIAN_POINT('Ctrl Pts',(3.00686224485374,1.,2.87146368430104));
#46552=CARTESIAN_POINT('Ctrl Pts',(3.00404638316245,1.,2.86418200833065));
#46553=CARTESIAN_POINT('Ctrl Pts',(3.0012015079552,1.,2.85692085715129));
#46554=CARTESIAN_POINT('Ctrl Pts',(2.99832751144566,1.,2.84968053289104));
#46555=CARTESIAN_POINT('Ctrl Pts',(2.995424253416,1.,2.84246132984334));
#46556=CARTESIAN_POINT('Ctrl Pts',(2.99249155170479,1.,2.83526351254383));
#46557=CARTESIAN_POINT('Ctrl Pts',(2.98952916401699,1.,2.82808728190402));
#46558=CARTESIAN_POINT('Ctrl Pts',(2.98653680669434,1.,2.82093279065704));
#46559=CARTESIAN_POINT('Ctrl Pts',(2.9835141977994,1.,2.81380019196454));
#46560=CARTESIAN_POINT('Ctrl Pts',(2.98046109647299,1.,2.80668968101162));
#46561=CARTESIAN_POINT('Ctrl Pts',(2.97737733718242,1.,2.79960153278186));
#46562=CARTESIAN_POINT('Ctrl Pts',(2.97426288347475,1.,2.79253615718147));
#46563=CARTESIAN_POINT('Ctrl Pts',(2.97111781461349,1.,2.78549409123657));
#46564=CARTESIAN_POINT('Ctrl Pts',(2.9679422104295,1.,2.77847589542767));
#46565=CARTESIAN_POINT('Ctrl Pts',(2.96473605585548,1.,2.77148206836464));
#46566=CARTESIAN_POINT('Ctrl Pts',(2.96149914764832,1.,2.76451296269571));
#46567=CARTESIAN_POINT('Ctrl Pts',(2.9582309766594,1.,2.75756867888393));
#46568=CARTESIAN_POINT('Ctrl Pts',(2.95493069316211,1.,2.75064903318996));
#46569=CARTESIAN_POINT('Ctrl Pts',(2.95159737214304,1.,2.7437537949221));
#46570=CARTESIAN_POINT('Ctrl Pts',(2.94823023414381,1.,2.73688288329825));
#46571=CARTESIAN_POINT('Ctrl Pts',(2.94482887675139,1.,2.73003657371613));
#46572=CARTESIAN_POINT('Ctrl Pts',(2.94139351933882,1.,2.72321571511322));
#46573=CARTESIAN_POINT('Ctrl Pts',(2.93792519474955,1.,2.71642190053575));
#46574=CARTESIAN_POINT('Ctrl Pts',(2.93442516311167,1.,2.70965695523776));
#46575=CARTESIAN_POINT('Ctrl Pts',(2.93089438233746,1.,2.70292247416881));
#46576=CARTESIAN_POINT('Ctrl Pts',(2.92733294395268,1.,2.69621932864302));
#46577=CARTESIAN_POINT('Ctrl Pts',(2.92373955325876,1.,2.68954721165342));
#46578=CARTESIAN_POINT('Ctrl Pts',(2.92011090722152,1.,2.68290409279689));
#46579=CARTESIAN_POINT('Ctrl Pts',(2.91644290704281,1.,2.67628728855309));
#46580=CARTESIAN_POINT('Ctrl Pts',(2.91273193382876,1.,2.66969458792627));
#46581=CARTESIAN_POINT('Ctrl Pts',(2.90897617968921,1.,2.66312542616809));
#46582=CARTESIAN_POINT('Ctrl Pts',(2.90517678087467,1.,2.65658188464287));
#46583=CARTESIAN_POINT('Ctrl Pts',(2.90133950224879,1.,2.65007017365576));
#46584=CARTESIAN_POINT('Ctrl Pts',(2.89747231723361,1.,2.64359851684146));
#46585=CARTESIAN_POINT('Ctrl Pts',(2.89358228854557,1.,2.63717442263944));
#46586=CARTESIAN_POINT('Ctrl Pts',(2.88967244854243,1.,2.63080195420771));
#46587=CARTESIAN_POINT('Ctrl Pts',(2.88573922195049,1.,2.62447947640253));
#46588=CARTESIAN_POINT('Ctrl Pts',(2.88176821427502,1.,2.61819596473087));
#46589=CARTESIAN_POINT('Ctrl Pts',(2.87773881947885,1.,2.61193507170928));
#46590=CARTESIAN_POINT('Ctrl Pts',(2.87363176656475,1.,2.6056817788128));
#46591=CARTESIAN_POINT('Ctrl Pts',(2.86943633170712,1.,2.59942875223202));
#46592=CARTESIAN_POINT('Ctrl Pts',(2.86515629953528,1.,2.59318160184921));
#46593=CARTESIAN_POINT('Ctrl Pts',(2.86081999003668,1.,2.5869677064356));
#46594=CARTESIAN_POINT('Ctrl Pts',(2.85647171715147,1.,2.58082875254407));
#46595=CARTESIAN_POINT('Ctrl Pts',(2.85215360144482,1.,2.57480482727128));
#46596=CARTESIAN_POINT('Ctrl Pts',(2.84788893329091,1.,2.56891984251743));
#46597=CARTESIAN_POINT('Ctrl Pts',(2.84366802680211,1.,2.56316920798489));
#46598=CARTESIAN_POINT('Ctrl Pts',(2.83942515220699,1.,2.55749952145165));
#46599=CARTESIAN_POINT('Ctrl Pts',(2.83505269592412,1.,2.55182152806964));
#46600=CARTESIAN_POINT('Ctrl Pts',(2.83044254225794,1.,2.54604736792542));
#46601=CARTESIAN_POINT('Ctrl Pts',(2.82552167649157,1.,2.54012272520141));
#46602=CARTESIAN_POINT('Ctrl Pts',(2.82028550483744,1.,2.53405679667463));
#46603=CARTESIAN_POINT('Ctrl Pts',(2.8148437904867,1.,2.52796388055457));
#46604=CARTESIAN_POINT('Ctrl Pts',(2.80941521967234,1.,2.52205778589922));
#46605=CARTESIAN_POINT('Ctrl Pts',(2.80427363984939,1.,2.51660190466067));
#46606=CARTESIAN_POINT('Ctrl Pts',(2.79970585014308,1.,2.51186983687947));
#46607=CARTESIAN_POINT('Ctrl Pts',(2.7959687805717,1.,2.50810555977564));
#46608=CARTESIAN_POINT('Ctrl Pts',(2.79344192164204,1.,2.50567182569153));
#46609=CARTESIAN_POINT('Ctrl Pts',(2.79217568804874,1.,2.50455968395235));
#46610=CARTESIAN_POINT('Ctrl Pts',(2.79164172519039,1.,2.50417932839344));
#46611=CARTESIAN_POINT('Ctrl Pts',(2.79145823440899,1.,2.50410700351426));
#46612=CARTESIAN_POINT('Ctrl Pts',(2.79140942341378,1.,2.50410331873042));
#46613=CARTESIAN_POINT('',(3.02314558451372,0.,2.91557726271063));
#46614=CARTESIAN_POINT('Ctrl Pts',(2.5041792485492,-1.,2.79134130681569));
#46615=CARTESIAN_POINT('Ctrl Pts',(2.5041792485492,1.,2.79134130681569));
#46616=CARTESIAN_POINT('Ctrl Pts',(2.50409239460108,-1.,2.7913358110015));
#46617=CARTESIAN_POINT('Ctrl Pts',(2.50409239460108,1.,2.7913358110015));
#46618=CARTESIAN_POINT('Ctrl Pts',(2.50404230339286,-1.,2.79143626022503));
#46619=CARTESIAN_POINT('Ctrl Pts',(2.50404230339286,1.,2.79143626022503));
#46620=CARTESIAN_POINT('Ctrl Pts',(2.5043379907732,-1.,2.79192122907148));
#46621=CARTESIAN_POINT('Ctrl Pts',(2.5043379907732,1.,2.79192122907148));
#46622=CARTESIAN_POINT('Ctrl Pts',(2.50547439929414,-1.,2.7932369408851));
#46623=CARTESIAN_POINT('Ctrl Pts',(2.50547439929414,1.,2.7932369408851));
#46624=CARTESIAN_POINT('Ctrl Pts',(2.5081055597767,-1.,2.79596878057287));
#46625=CARTESIAN_POINT('Ctrl Pts',(2.5081055597767,1.,2.79596878057287));
#46626=CARTESIAN_POINT('Ctrl Pts',(2.51186983687818,-1.,2.79970585014168));
#46627=CARTESIAN_POINT('Ctrl Pts',(2.51186983687818,1.,2.79970585014168));
#46628=CARTESIAN_POINT('Ctrl Pts',(2.51660190465805,-1.,2.80427363984653));
#46629=CARTESIAN_POINT('Ctrl Pts',(2.51660190465805,1.,2.80427363984653));
#46630=CARTESIAN_POINT('Ctrl Pts',(2.52205778589653,-1.,2.80941521966941));
#46631=CARTESIAN_POINT('Ctrl Pts',(2.52205778589653,1.,2.80941521966941));
#46632=CARTESIAN_POINT('Ctrl Pts',(2.52796388055278,-1.,2.81484379048475));
#46633=CARTESIAN_POINT('Ctrl Pts',(2.52796388055278,1.,2.81484379048475));
#46634=CARTESIAN_POINT('Ctrl Pts',(2.53405679667412,-1.,2.82028550483689));
#46635=CARTESIAN_POINT('Ctrl Pts',(2.53405679667412,1.,2.82028550483689));
#46636=CARTESIAN_POINT('Ctrl Pts',(2.54012272520199,-1.,2.8255216764922));
#46637=CARTESIAN_POINT('Ctrl Pts',(2.54012272520199,1.,2.8255216764922));
#46638=CARTESIAN_POINT('Ctrl Pts',(2.54604736792655,-1.,2.83044254225917));
#46639=CARTESIAN_POINT('Ctrl Pts',(2.54604736792655,1.,2.83044254225917));
#46640=CARTESIAN_POINT('Ctrl Pts',(2.55182152807077,-1.,2.83505269592536));
#46641=CARTESIAN_POINT('Ctrl Pts',(2.55182152807077,1.,2.83505269592536));
#46642=CARTESIAN_POINT('Ctrl Pts',(2.55749952145241,-1.,2.83942515220782));
#46643=CARTESIAN_POINT('Ctrl Pts',(2.55749952145241,1.,2.83942515220782));
#46644=CARTESIAN_POINT('Ctrl Pts',(2.56316920798513,-1.,2.84366802680237));
#46645=CARTESIAN_POINT('Ctrl Pts',(2.56316920798513,1.,2.84366802680237));
#46646=CARTESIAN_POINT('Ctrl Pts',(2.56891984251721,-1.,2.84788893329067));
#46647=CARTESIAN_POINT('Ctrl Pts',(2.56891984251721,1.,2.84788893329067));
#46648=CARTESIAN_POINT('Ctrl Pts',(2.57480482727081,-1.,2.85215360144431));
#46649=CARTESIAN_POINT('Ctrl Pts',(2.57480482727081,1.,2.85215360144431));
#46650=CARTESIAN_POINT('Ctrl Pts',(2.58082875254357,-1.,2.85647171715092));
#46651=CARTESIAN_POINT('Ctrl Pts',(2.58082875254357,1.,2.85647171715092));
#46652=CARTESIAN_POINT('Ctrl Pts',(2.58696770643524,-1.,2.86081999003629));
#46653=CARTESIAN_POINT('Ctrl Pts',(2.58696770643524,1.,2.86081999003629));
#46654=CARTESIAN_POINT('Ctrl Pts',(2.59318160184908,-1.,2.86515629953513));
#46655=CARTESIAN_POINT('Ctrl Pts',(2.59318160184908,1.,2.86515629953513));
#46656=CARTESIAN_POINT('Ctrl Pts',(2.5994287522321,-1.,2.86943633170722));
#46657=CARTESIAN_POINT('Ctrl Pts',(2.5994287522321,1.,2.86943633170722));
#46658=CARTESIAN_POINT('Ctrl Pts',(2.60568177881303,-1.,2.87363176656501));
#46659=CARTESIAN_POINT('Ctrl Pts',(2.60568177881303,1.,2.87363176656501));
#46660=CARTESIAN_POINT('Ctrl Pts',(2.61193507170955,-1.,2.87773881947916));
#46661=CARTESIAN_POINT('Ctrl Pts',(2.61193507170955,1.,2.87773881947916));
#46662=CARTESIAN_POINT('Ctrl Pts',(2.61819596473108,-1.,2.88176821427525));
#46663=CARTESIAN_POINT('Ctrl Pts',(2.61819596473108,1.,2.88176821427525));
#46664=CARTESIAN_POINT('Ctrl Pts',(2.62447947640262,-1.,2.88573922195059));
#46665=CARTESIAN_POINT('Ctrl Pts',(2.62447947640262,1.,2.88573922195059));
#46666=CARTESIAN_POINT('Ctrl Pts',(2.63080195420767,-1.,2.88967244854239));
#46667=CARTESIAN_POINT('Ctrl Pts',(2.63080195420767,1.,2.88967244854239));
#46668=CARTESIAN_POINT('Ctrl Pts',(2.63717442263932,-1.,2.89358228854544));
#46669=CARTESIAN_POINT('Ctrl Pts',(2.63717442263932,1.,2.89358228854544));
#46670=CARTESIAN_POINT('Ctrl Pts',(2.64359851684131,-1.,2.89747231723345));
#46671=CARTESIAN_POINT('Ctrl Pts',(2.64359851684131,1.,2.89747231723345));
#46672=CARTESIAN_POINT('Ctrl Pts',(2.65007017365564,-1.,2.90133950224867));
#46673=CARTESIAN_POINT('Ctrl Pts',(2.65007017365564,1.,2.90133950224867));
#46674=CARTESIAN_POINT('Ctrl Pts',(2.65658188464282,-1.,2.90517678087461));
#46675=CARTESIAN_POINT('Ctrl Pts',(2.65658188464282,1.,2.90517678087461));
#46676=CARTESIAN_POINT('Ctrl Pts',(2.6631254261681,-1.,2.90897617968923));
#46677=CARTESIAN_POINT('Ctrl Pts',(2.6631254261681,1.,2.90897617968923));
#46678=CARTESIAN_POINT('Ctrl Pts',(2.66969458792631,-1.,2.91273193382882));
#46679=CARTESIAN_POINT('Ctrl Pts',(2.66969458792631,1.,2.91273193382882));
#46680=CARTESIAN_POINT('Ctrl Pts',(2.67628728855312,-1.,2.91644290704285));
#46681=CARTESIAN_POINT('Ctrl Pts',(2.67628728855312,1.,2.91644290704285));
#46682=CARTESIAN_POINT('Ctrl Pts',(2.68290409279688,-1.,2.92011090722152));
#46683=CARTESIAN_POINT('Ctrl Pts',(2.68290409279688,1.,2.92011090722152));
#46684=CARTESIAN_POINT('Ctrl Pts',(2.68954721165339,-1.,2.92373955325875));
#46685=CARTESIAN_POINT('Ctrl Pts',(2.68954721165339,1.,2.92373955325875));
#46686=CARTESIAN_POINT('Ctrl Pts',(2.69621932864301,-1.,2.92733294395267));
#46687=CARTESIAN_POINT('Ctrl Pts',(2.69621932864301,1.,2.92733294395267));
#46688=CARTESIAN_POINT('Ctrl Pts',(2.70292247416885,-1.,2.9308943823375));
#46689=CARTESIAN_POINT('Ctrl Pts',(2.70292247416885,1.,2.9308943823375));
#46690=CARTESIAN_POINT('Ctrl Pts',(2.70965695523787,-1.,2.93442516311179));
#46691=CARTESIAN_POINT('Ctrl Pts',(2.70965695523787,1.,2.93442516311179));
#46692=CARTESIAN_POINT('Ctrl Pts',(2.71642190053592,-1.,2.93792519474972));
#46693=CARTESIAN_POINT('Ctrl Pts',(2.71642190053592,1.,2.93792519474972));
#46694=CARTESIAN_POINT('Ctrl Pts',(2.72321571511337,-1.,2.94139351933897));
#46695=CARTESIAN_POINT('Ctrl Pts',(2.72321571511337,1.,2.94139351933897));
#46696=CARTESIAN_POINT('Ctrl Pts',(2.73003657371616,-1.,2.94482887675143));
#46697=CARTESIAN_POINT('Ctrl Pts',(2.73003657371616,1.,2.94482887675143));
#46698=CARTESIAN_POINT('Ctrl Pts',(2.73688288329808,-1.,2.94823023414364));
#46699=CARTESIAN_POINT('Ctrl Pts',(2.73688288329808,1.,2.94823023414364));
#46700=CARTESIAN_POINT('Ctrl Pts',(2.74375379492172,-1.,2.95159737214266));
#46701=CARTESIAN_POINT('Ctrl Pts',(2.74375379492172,1.,2.95159737214266));
#46702=CARTESIAN_POINT('Ctrl Pts',(2.75064903318947,-1.,2.95493069316161));
#46703=CARTESIAN_POINT('Ctrl Pts',(2.75064903318947,1.,2.95493069316161));
#46704=CARTESIAN_POINT('Ctrl Pts',(2.7575686788835,-1.,2.95823097665896));
#46705=CARTESIAN_POINT('Ctrl Pts',(2.7575686788835,1.,2.95823097665896));
#46706=CARTESIAN_POINT('Ctrl Pts',(2.76451296269557,-1.,2.96149914764818));
#46707=CARTESIAN_POINT('Ctrl Pts',(2.76451296269557,1.,2.96149914764818));
#46708=CARTESIAN_POINT('Ctrl Pts',(2.77148206836498,-1.,2.96473605585583));
#46709=CARTESIAN_POINT('Ctrl Pts',(2.77148206836498,1.,2.96473605585583));
#46710=CARTESIAN_POINT('Ctrl Pts',(2.7784758954285,-1.,2.96794221043036));
#46711=CARTESIAN_POINT('Ctrl Pts',(2.7784758954285,1.,2.96794221043036));
#46712=CARTESIAN_POINT('Ctrl Pts',(2.78549409123769,-1.,2.97111781461465));
#46713=CARTESIAN_POINT('Ctrl Pts',(2.78549409123769,1.,2.97111781461465));
#46714=CARTESIAN_POINT('Ctrl Pts',(2.79253615718248,-1.,2.9742628834758));
#46715=CARTESIAN_POINT('Ctrl Pts',(2.79253615718248,1.,2.9742628834758));
#46716=CARTESIAN_POINT('Ctrl Pts',(2.7996015327823,-1.,2.97737733718287));
#46717=CARTESIAN_POINT('Ctrl Pts',(2.7996015327823,1.,2.97737733718287));
#46718=CARTESIAN_POINT('Ctrl Pts',(2.80668968101106,-1.,2.98046109647241));
#46719=CARTESIAN_POINT('Ctrl Pts',(2.80668968101106,1.,2.98046109647241));
#46720=CARTESIAN_POINT('Ctrl Pts',(2.81380019196286,-1.,2.98351419779767));
#46721=CARTESIAN_POINT('Ctrl Pts',(2.81380019196286,1.,2.98351419779767));
#46722=CARTESIAN_POINT('Ctrl Pts',(2.82093279065457,-1.,2.9865368066918));
#46723=CARTESIAN_POINT('Ctrl Pts',(2.82093279065457,1.,2.9865368066918));
#46724=CARTESIAN_POINT('Ctrl Pts',(2.82808728190157,-1.,2.98952916401446));
#46725=CARTESIAN_POINT('Ctrl Pts',(2.82808728190157,1.,2.98952916401446));
#46726=CARTESIAN_POINT('Ctrl Pts',(2.83526351254248,-1.,2.9924915517034));
#46727=CARTESIAN_POINT('Ctrl Pts',(2.83526351254248,1.,2.9924915517034));
#46728=CARTESIAN_POINT('Ctrl Pts',(2.84246132984415,-1.,2.99542425341685));
#46729=CARTESIAN_POINT('Ctrl Pts',(2.84246132984415,1.,2.99542425341685));
#46730=CARTESIAN_POINT('Ctrl Pts',(2.84968053289451,-1.,2.99832751144925));
#46731=CARTESIAN_POINT('Ctrl Pts',(2.84968053289451,1.,2.99832751144925));
#46732=CARTESIAN_POINT('Ctrl Pts',(2.85692085715685,-1.,3.00120150796095));
#46733=CARTESIAN_POINT('Ctrl Pts',(2.85692085715685,1.,3.00120150796095));
#46734=CARTESIAN_POINT('Ctrl Pts',(2.86418200833667,-1.,3.00404638316867));
#46735=CARTESIAN_POINT('Ctrl Pts',(2.86418200833667,1.,3.00404638316867));
#46736=CARTESIAN_POINT('Ctrl Pts',(2.87146368430501,-1.,3.00686224485784));
#46737=CARTESIAN_POINT('Ctrl Pts',(2.87146368430501,1.,3.00686224485784));
#46738=CARTESIAN_POINT('Ctrl Pts',(2.87876560072727,-1.,3.00964918108476));
#46739=CARTESIAN_POINT('Ctrl Pts',(2.87876560072727,1.,3.00964918108476));
#46740=CARTESIAN_POINT('Ctrl Pts',(2.8860875170608,-1.,3.01240727308829));
#46741=CARTESIAN_POINT('Ctrl Pts',(2.8860875170608,1.,3.01240727308829));
#46742=CARTESIAN_POINT('Ctrl Pts',(2.89342925566321,-1.,3.01513660431928));
#46743=CARTESIAN_POINT('Ctrl Pts',(2.89342925566321,1.,3.01513660431928));
#46744=CARTESIAN_POINT('Ctrl Pts',(2.9007906910105,-1.,3.01783725121981));
#46745=CARTESIAN_POINT('Ctrl Pts',(2.9007906910105,1.,3.01783725121981));
#46746=CARTESIAN_POINT('Ctrl Pts',(2.90669553302526,-1.,3.01997487193503));
#46747=CARTESIAN_POINT('Ctrl Pts',(2.90669553302526,1.,3.01997487193503));
#46748=CARTESIAN_POINT('Ctrl Pts',(2.91113297348212,-1.,3.02156522742431));
#46749=CARTESIAN_POINT('Ctrl Pts',(2.91113297348212,1.,3.02156522742431));
#46750=CARTESIAN_POINT('Ctrl Pts',(2.91409518070399,-1.,3.02261975104593));
#46751=CARTESIAN_POINT('Ctrl Pts',(2.91409518070399,1.,3.02261975104593));
#46752=CARTESIAN_POINT('Ctrl Pts',(2.91557726271063,-1.,3.02314558451372));
#46753=CARTESIAN_POINT('Ctrl Pts',(2.91557726271063,1.,3.02314558451372));
#46754=CARTESIAN_POINT('',(2.50410331873176,1.,2.79140942341258));
#46755=CARTESIAN_POINT('Ctrl Pts',(2.50410331873176,-1.,2.79140942341258));
#46756=CARTESIAN_POINT('Ctrl Pts',(2.50410331873176,-0.666666666666667,
2.79140942341258));
#46757=CARTESIAN_POINT('Ctrl Pts',(2.50410331873176,-0.333333333333333,
2.79140942341258));
#46758=CARTESIAN_POINT('Ctrl Pts',(2.50410331873176,0.333333333333333,2.79140942341258));
#46759=CARTESIAN_POINT('Ctrl Pts',(2.50410331873176,0.666666666666667,2.79140942341258));
#46760=CARTESIAN_POINT('Ctrl Pts',(2.50410331873176,1.,2.79140942341258));
#46761=CARTESIAN_POINT('',(2.91557726271063,1.,3.02314558451372));
#46762=CARTESIAN_POINT('',(2.91557726271063,0.,3.02314558451372));
#46763=CARTESIAN_POINT('Ctrl Pts',(2.50410331873176,1.,2.79140942341258));
#46764=CARTESIAN_POINT('Ctrl Pts',(2.50410700351493,1.,2.79145823440781));
#46765=CARTESIAN_POINT('Ctrl Pts',(2.50417932839313,1.,2.79164172518905));
#46766=CARTESIAN_POINT('Ctrl Pts',(2.50455968395146,1.,2.79217568804755));
#46767=CARTESIAN_POINT('Ctrl Pts',(2.50567182569081,1.,2.79344192164147));
#46768=CARTESIAN_POINT('Ctrl Pts',(2.5081055597767,1.,2.79596878057287));
#46769=CARTESIAN_POINT('Ctrl Pts',(2.51186983687818,1.,2.79970585014168));
#46770=CARTESIAN_POINT('Ctrl Pts',(2.51660190465805,1.,2.80427363984653));
#46771=CARTESIAN_POINT('Ctrl Pts',(2.52205778589653,1.,2.80941521966941));
#46772=CARTESIAN_POINT('Ctrl Pts',(2.52796388055278,1.,2.81484379048475));
#46773=CARTESIAN_POINT('Ctrl Pts',(2.53405679667412,1.,2.82028550483689));
#46774=CARTESIAN_POINT('Ctrl Pts',(2.54012272520199,1.,2.8255216764922));
#46775=CARTESIAN_POINT('Ctrl Pts',(2.54604736792655,1.,2.83044254225917));
#46776=CARTESIAN_POINT('Ctrl Pts',(2.55182152807077,1.,2.83505269592536));
#46777=CARTESIAN_POINT('Ctrl Pts',(2.55749952145241,1.,2.83942515220782));
#46778=CARTESIAN_POINT('Ctrl Pts',(2.56316920798513,1.,2.84366802680237));
#46779=CARTESIAN_POINT('Ctrl Pts',(2.56891984251721,1.,2.84788893329067));
#46780=CARTESIAN_POINT('Ctrl Pts',(2.57480482727081,1.,2.85215360144431));
#46781=CARTESIAN_POINT('Ctrl Pts',(2.58082875254357,1.,2.85647171715092));
#46782=CARTESIAN_POINT('Ctrl Pts',(2.58696770643524,1.,2.86081999003629));
#46783=CARTESIAN_POINT('Ctrl Pts',(2.59318160184908,1.,2.86515629953513));
#46784=CARTESIAN_POINT('Ctrl Pts',(2.5994287522321,1.,2.86943633170722));
#46785=CARTESIAN_POINT('Ctrl Pts',(2.60568177881303,1.,2.87363176656501));
#46786=CARTESIAN_POINT('Ctrl Pts',(2.61193507170955,1.,2.87773881947916));
#46787=CARTESIAN_POINT('Ctrl Pts',(2.61819596473108,1.,2.88176821427525));
#46788=CARTESIAN_POINT('Ctrl Pts',(2.62447947640262,1.,2.88573922195059));
#46789=CARTESIAN_POINT('Ctrl Pts',(2.63080195420767,1.,2.88967244854239));
#46790=CARTESIAN_POINT('Ctrl Pts',(2.63717442263932,1.,2.89358228854544));
#46791=CARTESIAN_POINT('Ctrl Pts',(2.64359851684131,1.,2.89747231723345));
#46792=CARTESIAN_POINT('Ctrl Pts',(2.65007017365564,1.,2.90133950224867));
#46793=CARTESIAN_POINT('Ctrl Pts',(2.65658188464282,1.,2.90517678087461));
#46794=CARTESIAN_POINT('Ctrl Pts',(2.6631254261681,1.,2.90897617968923));
#46795=CARTESIAN_POINT('Ctrl Pts',(2.66969458792631,1.,2.91273193382882));
#46796=CARTESIAN_POINT('Ctrl Pts',(2.67628728855312,1.,2.91644290704285));
#46797=CARTESIAN_POINT('Ctrl Pts',(2.68290409279688,1.,2.92011090722152));
#46798=CARTESIAN_POINT('Ctrl Pts',(2.68954721165339,1.,2.92373955325875));
#46799=CARTESIAN_POINT('Ctrl Pts',(2.69621932864301,1.,2.92733294395267));
#46800=CARTESIAN_POINT('Ctrl Pts',(2.70292247416885,1.,2.9308943823375));
#46801=CARTESIAN_POINT('Ctrl Pts',(2.70965695523787,1.,2.93442516311179));
#46802=CARTESIAN_POINT('Ctrl Pts',(2.71642190053592,1.,2.93792519474972));
#46803=CARTESIAN_POINT('Ctrl Pts',(2.72321571511337,1.,2.94139351933897));
#46804=CARTESIAN_POINT('Ctrl Pts',(2.73003657371616,1.,2.94482887675143));
#46805=CARTESIAN_POINT('Ctrl Pts',(2.73688288329808,1.,2.94823023414364));
#46806=CARTESIAN_POINT('Ctrl Pts',(2.74375379492172,1.,2.95159737214266));
#46807=CARTESIAN_POINT('Ctrl Pts',(2.75064903318947,1.,2.95493069316161));
#46808=CARTESIAN_POINT('Ctrl Pts',(2.7575686788835,1.,2.95823097665896));
#46809=CARTESIAN_POINT('Ctrl Pts',(2.76451296269557,1.,2.96149914764818));
#46810=CARTESIAN_POINT('Ctrl Pts',(2.77148206836498,1.,2.96473605585583));
#46811=CARTESIAN_POINT('Ctrl Pts',(2.7784758954285,1.,2.96794221043036));
#46812=CARTESIAN_POINT('Ctrl Pts',(2.78549409123769,1.,2.97111781461465));
#46813=CARTESIAN_POINT('Ctrl Pts',(2.79253615718248,1.,2.9742628834758));
#46814=CARTESIAN_POINT('Ctrl Pts',(2.7996015327823,1.,2.97737733718287));
#46815=CARTESIAN_POINT('Ctrl Pts',(2.80668968101106,1.,2.98046109647241));
#46816=CARTESIAN_POINT('Ctrl Pts',(2.81380019196286,1.,2.98351419779767));
#46817=CARTESIAN_POINT('Ctrl Pts',(2.82093279065457,1.,2.9865368066918));
#46818=CARTESIAN_POINT('Ctrl Pts',(2.82808728190157,1.,2.98952916401446));
#46819=CARTESIAN_POINT('Ctrl Pts',(2.83526351254248,1.,2.9924915517034));
#46820=CARTESIAN_POINT('Ctrl Pts',(2.84246132984415,1.,2.99542425341685));
#46821=CARTESIAN_POINT('Ctrl Pts',(2.84968053289451,1.,2.99832751144925));
#46822=CARTESIAN_POINT('Ctrl Pts',(2.85692085715685,1.,3.00120150796095));
#46823=CARTESIAN_POINT('Ctrl Pts',(2.86418200833667,1.,3.00404638316867));
#46824=CARTESIAN_POINT('Ctrl Pts',(2.87146368430501,1.,3.00686224485784));
#46825=CARTESIAN_POINT('Ctrl Pts',(2.87876560072727,1.,3.00964918108476));
#46826=CARTESIAN_POINT('Ctrl Pts',(2.8860875170608,1.,3.01240727308829));
#46827=CARTESIAN_POINT('Ctrl Pts',(2.89342925566321,1.,3.01513660431928));
#46828=CARTESIAN_POINT('Ctrl Pts',(2.9007906910105,1.,3.01783725121981));
#46829=CARTESIAN_POINT('Ctrl Pts',(2.90669553302526,1.,3.01997487193503));
#46830=CARTESIAN_POINT('Ctrl Pts',(2.91113297348212,1.,3.02156522742431));
#46831=CARTESIAN_POINT('Ctrl Pts',(2.91409518070399,1.,3.02261975104593));
#46832=CARTESIAN_POINT('Ctrl Pts',(2.91557726271063,1.,3.02314558451372));
#46833=CARTESIAN_POINT('Origin',(2.91557726271063,0.,3.02314558451372));
#46834=CARTESIAN_POINT('',(3.02314558451372,1.,2.91557726271063));
#46835=CARTESIAN_POINT('Origin',(0.,0.,0.));
#46836=CARTESIAN_POINT('',(2.36531447826213,1.,2.90994629141562));
#46837=CARTESIAN_POINT('Origin',(0.,1.,0.));
#46838=CARTESIAN_POINT('Ctrl Pts',(2.36531447826213,1.,2.90994629141563));
#46839=CARTESIAN_POINT('Ctrl Pts',(2.36531447826213,0.666666666666667,2.90994629141563));
#46840=CARTESIAN_POINT('Ctrl Pts',(2.36531447826213,0.333333333333333,2.90994629141563));
#46841=CARTESIAN_POINT('Ctrl Pts',(2.36531447826213,-0.333333333333333,
2.90994629141563));
#46842=CARTESIAN_POINT('Ctrl Pts',(2.36531447826213,-0.666666666666667,
2.90994629141563));
#46843=CARTESIAN_POINT('Ctrl Pts',(2.36531447826213,-1.,2.90994629141563));
#46844=CARTESIAN_POINT('Ctrl Pts',(2.52982887637028,-1.,3.35260583073571));
#46845=CARTESIAN_POINT('Ctrl Pts',(2.52982887637028,1.,3.35260583073571));
#46846=CARTESIAN_POINT('Ctrl Pts',(2.52954136549357,-1.,3.35105973714426));
#46847=CARTESIAN_POINT('Ctrl Pts',(2.52954136549357,1.,3.35105973714426));
#46848=CARTESIAN_POINT('Ctrl Pts',(2.5289632161143,-1.,3.34796903577628));
#46849=CARTESIAN_POINT('Ctrl Pts',(2.5289632161143,1.,3.34796903577628));
#46850=CARTESIAN_POINT('Ctrl Pts',(2.52808660916879,-1.,3.34333744117093));
#46851=CARTESIAN_POINT('Ctrl Pts',(2.52808660916879,1.,3.34333744117093));
#46852=CARTESIAN_POINT('Ctrl Pts',(2.52689902691551,-1.,3.33717090000955));
#46853=CARTESIAN_POINT('Ctrl Pts',(2.52689902691551,1.,3.33717090000955));
#46854=CARTESIAN_POINT('Ctrl Pts',(2.52538321165774,-1.,3.32947762189049));
#46855=CARTESIAN_POINT('Ctrl Pts',(2.52538321165774,1.,3.32947762189049));
#46856=CARTESIAN_POINT('Ctrl Pts',(2.52383598396878,-1.,3.32179931079521));
#46857=CARTESIAN_POINT('Ctrl Pts',(2.52383598396878,1.,3.32179931079521));
#46858=CARTESIAN_POINT('Ctrl Pts',(2.52225724871375,-1.,3.31413607874727));
#46859=CARTESIAN_POINT('Ctrl Pts',(2.52225724871375,1.,3.31413607874727));
#46860=CARTESIAN_POINT('Ctrl Pts',(2.52064689568167,-1.,3.30648808814986));
#46861=CARTESIAN_POINT('Ctrl Pts',(2.52064689568167,1.,3.30648808814986));
#46862=CARTESIAN_POINT('Ctrl Pts',(2.51900480700548,-1.,3.29885556387661));
#46863=CARTESIAN_POINT('Ctrl Pts',(2.51900480700548,1.,3.29885556387661));
#46864=CARTESIAN_POINT('Ctrl Pts',(2.51733085123316,-1.,3.2912387729863));
#46865=CARTESIAN_POINT('Ctrl Pts',(2.51733085123316,1.,3.2912387729863));
#46866=CARTESIAN_POINT('Ctrl Pts',(2.51562487464214,-1.,3.28363799702583));
#46867=CARTESIAN_POINT('Ctrl Pts',(2.51562487464214,1.,3.28363799702583));
#46868=CARTESIAN_POINT('Ctrl Pts',(2.51388669270329,-1.,3.27605350473048));
#46869=CARTESIAN_POINT('Ctrl Pts',(2.51388669270329,1.,3.27605350473048));
#46870=CARTESIAN_POINT('Ctrl Pts',(2.51211608411539,-1.,3.26848552888271));
#46871=CARTESIAN_POINT('Ctrl Pts',(2.51211608411539,1.,3.26848552888271));
#46872=CARTESIAN_POINT('Ctrl Pts',(2.51031277813697,-1.,3.26093423001716));
#46873=CARTESIAN_POINT('Ctrl Pts',(2.51031277813697,1.,3.26093423001716));
#46874=CARTESIAN_POINT('Ctrl Pts',(2.50847647070936,-1.,3.25339971461265));
#46875=CARTESIAN_POINT('Ctrl Pts',(2.50847647070936,1.,3.25339971461265));
#46876=CARTESIAN_POINT('Ctrl Pts',(2.50660685940645,-1.,3.24588208984042));
#46877=CARTESIAN_POINT('Ctrl Pts',(2.50660685940645,1.,3.24588208984042));
#46878=CARTESIAN_POINT('Ctrl Pts',(2.50470367580078,-1.,3.23838151080383));
#46879=CARTESIAN_POINT('Ctrl Pts',(2.50470367580078,1.,3.23838151080383));
#46880=CARTESIAN_POINT('Ctrl Pts',(2.50276671338074,-1.,3.23089822320596));
#46881=CARTESIAN_POINT('Ctrl Pts',(2.50276671338074,1.,3.23089822320596));
#46882=CARTESIAN_POINT('Ctrl Pts',(2.5007958720187,-1.,3.22343262620387));
#46883=CARTESIAN_POINT('Ctrl Pts',(2.5007958720187,1.,3.22343262620387));
#46884=CARTESIAN_POINT('Ctrl Pts',(2.49879114599293,-1.,3.21598526261157));
#46885=CARTESIAN_POINT('Ctrl Pts',(2.49879114599293,1.,3.21598526261157));
#46886=CARTESIAN_POINT('Ctrl Pts',(2.49675252647298,-1.,3.2085566984974));
#46887=CARTESIAN_POINT('Ctrl Pts',(2.49675252647298,1.,3.2085566984974));
#46888=CARTESIAN_POINT('Ctrl Pts',(2.49467992057726,-1.,3.20114742397549));
#46889=CARTESIAN_POINT('Ctrl Pts',(2.49467992057726,1.,3.20114742397549));
#46890=CARTESIAN_POINT('Ctrl Pts',(2.4925730723986,-1.,3.19375775555814));
#46891=CARTESIAN_POINT('Ctrl Pts',(2.4925730723986,1.,3.19375775555814));
#46892=CARTESIAN_POINT('Ctrl Pts',(2.49043146334095,-1.,3.18638771282315));
#46893=CARTESIAN_POINT('Ctrl Pts',(2.49043146334095,1.,3.18638771282315));
#46894=CARTESIAN_POINT('Ctrl Pts',(2.48825428288242,-1.,3.17903698136679));
#46895=CARTESIAN_POINT('Ctrl Pts',(2.48825428288242,1.,3.17903698136679));
#46896=CARTESIAN_POINT('Ctrl Pts',(2.48604065348619,-1.,3.17170518863357));
#46897=CARTESIAN_POINT('Ctrl Pts',(2.48604065348619,1.,3.17170518863357));
#46898=CARTESIAN_POINT('Ctrl Pts',(2.48378981792739,-1.,3.16439213290181));
#46899=CARTESIAN_POINT('Ctrl Pts',(2.48378981792739,1.,3.16439213290181));
#46900=CARTESIAN_POINT('Ctrl Pts',(2.48150133566568,-1.,3.15709802322735));
#46901=CARTESIAN_POINT('Ctrl Pts',(2.48150133566568,1.,3.15709802322735));
#46902=CARTESIAN_POINT('Ctrl Pts',(2.47917529057016,-1.,3.14982373241335));
#46903=CARTESIAN_POINT('Ctrl Pts',(2.47917529057016,1.,3.14982373241335));
#46904=CARTESIAN_POINT('Ctrl Pts',(2.47681245356095,-1.,3.14257099546531));
#46905=CARTESIAN_POINT('Ctrl Pts',(2.47681245356095,1.,3.14257099546531));
#46906=CARTESIAN_POINT('Ctrl Pts',(2.47441378371923,-1.,3.13534181229282));
#46907=CARTESIAN_POINT('Ctrl Pts',(2.47441378371923,1.,3.13534181229282));
#46908=CARTESIAN_POINT('Ctrl Pts',(2.47197997765868,-1.,3.12813790805948));
#46909=CARTESIAN_POINT('Ctrl Pts',(2.47197997765868,1.,3.12813790805948));
#46910=CARTESIAN_POINT('Ctrl Pts',(2.4695109894747,-1.,3.12096015766984));
#46911=CARTESIAN_POINT('Ctrl Pts',(2.4695109894747,1.,3.12096015766984));
#46912=CARTESIAN_POINT('Ctrl Pts',(2.46700558843507,-1.,3.11380805536124));
#46913=CARTESIAN_POINT('Ctrl Pts',(2.46700558843507,1.,3.11380805536124));
#46914=CARTESIAN_POINT('Ctrl Pts',(2.46446082979645,-1.,3.10667907901981));
#46915=CARTESIAN_POINT('Ctrl Pts',(2.46446082979645,1.,3.10667907901981));
#46916=CARTESIAN_POINT('Ctrl Pts',(2.4618730850188,-1.,3.09956993697048));
#46917=CARTESIAN_POINT('Ctrl Pts',(2.4618730850188,1.,3.09956993697048));
#46918=CARTESIAN_POINT('Ctrl Pts',(2.45923912563875,-1.,3.09247787931881));
#46919=CARTESIAN_POINT('Ctrl Pts',(2.45923912563875,1.,3.09247787931881));
#46920=CARTESIAN_POINT('Ctrl Pts',(2.45655725437037,-1.,3.08540206545313));
#46921=CARTESIAN_POINT('Ctrl Pts',(2.45655725437037,1.,3.08540206545313));
#46922=CARTESIAN_POINT('Ctrl Pts',(2.45382826787795,-1.,3.07834472886145));
#46923=CARTESIAN_POINT('Ctrl Pts',(2.45382826787795,1.,3.07834472886145));
#46924=CARTESIAN_POINT('Ctrl Pts',(2.45105688854432,-1.,3.0713129052131));
#46925=CARTESIAN_POINT('Ctrl Pts',(2.45105688854432,1.,3.0713129052131));
#46926=CARTESIAN_POINT('Ctrl Pts',(2.44824970516557,-1.,3.06431596421422));
#46927=CARTESIAN_POINT('Ctrl Pts',(2.44824970516557,1.,3.06431596421422));
#46928=CARTESIAN_POINT('Ctrl Pts',(2.44541251892568,-1.,3.05736242671521));
#46929=CARTESIAN_POINT('Ctrl Pts',(2.44541251892568,1.,3.05736242671521));
#46930=CARTESIAN_POINT('Ctrl Pts',(2.44254768923109,-1.,3.05045678021509));
#46931=CARTESIAN_POINT('Ctrl Pts',(2.44254768923109,1.,3.05045678021509));
#46932=CARTESIAN_POINT('Ctrl Pts',(2.43965194061849,-1.,3.04359685040545));
#46933=CARTESIAN_POINT('Ctrl Pts',(2.43965194061849,1.,3.04359685040545));
#46934=CARTESIAN_POINT('Ctrl Pts',(2.43671278042394,-1.,3.03676949672797));
#46935=CARTESIAN_POINT('Ctrl Pts',(2.43671278042394,1.,3.03676949672797));
#46936=CARTESIAN_POINT('Ctrl Pts',(2.43371241361462,-1.,3.02995534946946));
#46937=CARTESIAN_POINT('Ctrl Pts',(2.43371241361462,1.,3.02995534946946));
#46938=CARTESIAN_POINT('Ctrl Pts',(2.43063415586615,-1.,3.02313656035977));
#46939=CARTESIAN_POINT('Ctrl Pts',(2.43063415586615,1.,3.02313656035977));
#46940=CARTESIAN_POINT('Ctrl Pts',(2.4274685626416,-1.,3.01630420830494));
#46941=CARTESIAN_POINT('Ctrl Pts',(2.4274685626416,1.,3.01630420830494));
#46942=CARTESIAN_POINT('Ctrl Pts',(2.42421849439625,-1.,3.00946442616674));
#46943=CARTESIAN_POINT('Ctrl Pts',(2.42421849439625,1.,3.00946442616674));
#46944=CARTESIAN_POINT('Ctrl Pts',(2.42090763946812,-1.,3.00264868586038));
#46945=CARTESIAN_POINT('Ctrl Pts',(2.42090763946812,1.,3.00264868586038));
#46946=CARTESIAN_POINT('Ctrl Pts',(2.4175732450056,-1.,2.99590509293561));
#46947=CARTESIAN_POINT('Ctrl Pts',(2.4175732450056,1.,2.99590509293561));
#46948=CARTESIAN_POINT('Ctrl Pts',(2.4142506419963,-1.,2.98927983005851));
#46949=CARTESIAN_POINT('Ctrl Pts',(2.4142506419963,1.,2.98927983005851));
#46950=CARTESIAN_POINT('Ctrl Pts',(2.41095909342591,-1.,2.98280015815132));
#46951=CARTESIAN_POINT('Ctrl Pts',(2.41095909342591,1.,2.98280015815132));
#46952=CARTESIAN_POINT('Ctrl Pts',(2.40768975073691,-1.,2.97646002822395));
#46953=CARTESIAN_POINT('Ctrl Pts',(2.40768975073691,1.,2.97646002822395));
#46954=CARTESIAN_POINT('Ctrl Pts',(2.40438604734848,-1.,2.97019641312272));
#46955=CARTESIAN_POINT('Ctrl Pts',(2.40438604734848,1.,2.97019641312272));
#46956=CARTESIAN_POINT('Ctrl Pts',(2.40095565711535,-1.,2.96390432240181));
#46957=CARTESIAN_POINT('Ctrl Pts',(2.40095565711535,1.,2.96390432240181));
#46958=CARTESIAN_POINT('Ctrl Pts',(2.39730553974412,-1.,2.95748006482811));
#46959=CARTESIAN_POINT('Ctrl Pts',(2.39730553974412,1.,2.95748006482811));
#46960=CARTESIAN_POINT('Ctrl Pts',(2.39337207631613,-1.,2.95085857128372));
#46961=CARTESIAN_POINT('Ctrl Pts',(2.39337207631613,1.,2.95085857128372));
#46962=CARTESIAN_POINT('Ctrl Pts',(2.38914929090806,-1.,2.94404820669135));
#46963=CARTESIAN_POINT('Ctrl Pts',(2.38914929090806,1.,2.94404820669135));
#46964=CARTESIAN_POINT('Ctrl Pts',(2.38472771516476,-1.,2.93717903280599));
#46965=CARTESIAN_POINT('Ctrl Pts',(2.38472771516476,1.,2.93717903280599));
#46966=CARTESIAN_POINT('Ctrl Pts',(2.3802898958232,-1.,2.93049643640517));
#46967=CARTESIAN_POINT('Ctrl Pts',(2.3802898958232,1.,2.93049643640517));
#46968=CARTESIAN_POINT('Ctrl Pts',(2.37606510524271,-1.,2.92430340582912));
#46969=CARTESIAN_POINT('Ctrl Pts',(2.37606510524271,1.,2.92430340582912));
#46970=CARTESIAN_POINT('Ctrl Pts',(2.37229381109939,-1.,2.9189150379156));
#46971=CARTESIAN_POINT('Ctrl Pts',(2.37229381109939,1.,2.9189150379156));
#46972=CARTESIAN_POINT('Ctrl Pts',(2.36919161373074,-1.,2.91461249883016));
#46973=CARTESIAN_POINT('Ctrl Pts',(2.36919161373074,1.,2.91461249883016));
#46974=CARTESIAN_POINT('Ctrl Pts',(2.36690501170317,-1.,2.9115863784165));
#46975=CARTESIAN_POINT('Ctrl Pts',(2.36690501170317,1.,2.9115863784165));
#46976=CARTESIAN_POINT('Ctrl Pts',(2.36578327194396,-1.,2.91025813829606));
#46977=CARTESIAN_POINT('Ctrl Pts',(2.36578327194396,1.,2.91025813829606));
#46978=CARTESIAN_POINT('Ctrl Pts',(2.36535052956704,-1.,2.90989022547738));
#46979=CARTESIAN_POINT('Ctrl Pts',(2.36535052956704,1.,2.90989022547738));
#46980=CARTESIAN_POINT('Ctrl Pts',(2.36524348105023,-1.,2.90992398626098));
#46981=CARTESIAN_POINT('Ctrl Pts',(2.36524348105023,1.,2.90992398626098));
#46982=CARTESIAN_POINT('Ctrl Pts',(2.36523532225181,-1.,2.91001063062876));
#46983=CARTESIAN_POINT('Ctrl Pts',(2.36523532225181,1.,2.91001063062876));
#46984=CARTESIAN_POINT('',(2.52982887637028,1.,3.35260583073571));
#46985=CARTESIAN_POINT('Ctrl Pts',(2.52982887637028,1.,3.35260583073571));
#46986=CARTESIAN_POINT('Ctrl Pts',(2.52954136549357,1.,3.35105973714426));
#46987=CARTESIAN_POINT('Ctrl Pts',(2.5289632161143,1.,3.34796903577628));
#46988=CARTESIAN_POINT('Ctrl Pts',(2.52808660916879,1.,3.34333744117093));
#46989=CARTESIAN_POINT('Ctrl Pts',(2.52689902691551,1.,3.33717090000955));
#46990=CARTESIAN_POINT('Ctrl Pts',(2.52538321165774,1.,3.32947762189049));
#46991=CARTESIAN_POINT('Ctrl Pts',(2.52383598396878,1.,3.32179931079521));
#46992=CARTESIAN_POINT('Ctrl Pts',(2.52225724871375,1.,3.31413607874727));
#46993=CARTESIAN_POINT('Ctrl Pts',(2.52064689568167,1.,3.30648808814986));
#46994=CARTESIAN_POINT('Ctrl Pts',(2.51900480700548,1.,3.29885556387661));
#46995=CARTESIAN_POINT('Ctrl Pts',(2.51733085123316,1.,3.2912387729863));
#46996=CARTESIAN_POINT('Ctrl Pts',(2.51562487464214,1.,3.28363799702583));
#46997=CARTESIAN_POINT('Ctrl Pts',(2.51388669270329,1.,3.27605350473048));
#46998=CARTESIAN_POINT('Ctrl Pts',(2.51211608411539,1.,3.26848552888271));
#46999=CARTESIAN_POINT('Ctrl Pts',(2.51031277813697,1.,3.26093423001716));
#47000=CARTESIAN_POINT('Ctrl Pts',(2.50847647070936,1.,3.25339971461265));
#47001=CARTESIAN_POINT('Ctrl Pts',(2.50660685940645,1.,3.24588208984042));
#47002=CARTESIAN_POINT('Ctrl Pts',(2.50470367580078,1.,3.23838151080383));
#47003=CARTESIAN_POINT('Ctrl Pts',(2.50276671338074,1.,3.23089822320596));
#47004=CARTESIAN_POINT('Ctrl Pts',(2.5007958720187,1.,3.22343262620387));
#47005=CARTESIAN_POINT('Ctrl Pts',(2.49879114599293,1.,3.21598526261157));
#47006=CARTESIAN_POINT('Ctrl Pts',(2.49675252647298,1.,3.2085566984974));
#47007=CARTESIAN_POINT('Ctrl Pts',(2.49467992057726,1.,3.20114742397549));
#47008=CARTESIAN_POINT('Ctrl Pts',(2.4925730723986,1.,3.19375775555814));
#47009=CARTESIAN_POINT('Ctrl Pts',(2.49043146334095,1.,3.18638771282315));
#47010=CARTESIAN_POINT('Ctrl Pts',(2.48825428288242,1.,3.17903698136679));
#47011=CARTESIAN_POINT('Ctrl Pts',(2.48604065348619,1.,3.17170518863357));
#47012=CARTESIAN_POINT('Ctrl Pts',(2.48378981792739,1.,3.16439213290181));
#47013=CARTESIAN_POINT('Ctrl Pts',(2.48150133566568,1.,3.15709802322735));
#47014=CARTESIAN_POINT('Ctrl Pts',(2.47917529057016,1.,3.14982373241335));
#47015=CARTESIAN_POINT('Ctrl Pts',(2.47681245356095,1.,3.14257099546531));
#47016=CARTESIAN_POINT('Ctrl Pts',(2.47441378371923,1.,3.13534181229282));
#47017=CARTESIAN_POINT('Ctrl Pts',(2.47197997765868,1.,3.12813790805948));
#47018=CARTESIAN_POINT('Ctrl Pts',(2.4695109894747,1.,3.12096015766984));
#47019=CARTESIAN_POINT('Ctrl Pts',(2.46700558843507,1.,3.11380805536124));
#47020=CARTESIAN_POINT('Ctrl Pts',(2.46446082979645,1.,3.10667907901981));
#47021=CARTESIAN_POINT('Ctrl Pts',(2.4618730850188,1.,3.09956993697048));
#47022=CARTESIAN_POINT('Ctrl Pts',(2.45923912563875,1.,3.09247787931881));
#47023=CARTESIAN_POINT('Ctrl Pts',(2.45655725437037,1.,3.08540206545313));
#47024=CARTESIAN_POINT('Ctrl Pts',(2.45382826787795,1.,3.07834472886145));
#47025=CARTESIAN_POINT('Ctrl Pts',(2.45105688854432,1.,3.0713129052131));
#47026=CARTESIAN_POINT('Ctrl Pts',(2.44824970516557,1.,3.06431596421422));
#47027=CARTESIAN_POINT('Ctrl Pts',(2.44541251892568,1.,3.05736242671521));
#47028=CARTESIAN_POINT('Ctrl Pts',(2.44254768923109,1.,3.05045678021509));
#47029=CARTESIAN_POINT('Ctrl Pts',(2.43965194061849,1.,3.04359685040545));
#47030=CARTESIAN_POINT('Ctrl Pts',(2.43671278042394,1.,3.03676949672797));
#47031=CARTESIAN_POINT('Ctrl Pts',(2.43371241361462,1.,3.02995534946946));
#47032=CARTESIAN_POINT('Ctrl Pts',(2.43063415586615,1.,3.02313656035977));
#47033=CARTESIAN_POINT('Ctrl Pts',(2.4274685626416,1.,3.01630420830494));
#47034=CARTESIAN_POINT('Ctrl Pts',(2.42421849439625,1.,3.00946442616674));
#47035=CARTESIAN_POINT('Ctrl Pts',(2.42090763946812,1.,3.00264868586038));
#47036=CARTESIAN_POINT('Ctrl Pts',(2.4175732450056,1.,2.99590509293561));
#47037=CARTESIAN_POINT('Ctrl Pts',(2.4142506419963,1.,2.98927983005851));
#47038=CARTESIAN_POINT('Ctrl Pts',(2.41095909342591,1.,2.98280015815132));
#47039=CARTESIAN_POINT('Ctrl Pts',(2.40768975073691,1.,2.97646002822395));
#47040=CARTESIAN_POINT('Ctrl Pts',(2.40438604734848,1.,2.97019641312272));
#47041=CARTESIAN_POINT('Ctrl Pts',(2.40095565711535,1.,2.96390432240181));
#47042=CARTESIAN_POINT('Ctrl Pts',(2.39730553974412,1.,2.95748006482811));
#47043=CARTESIAN_POINT('Ctrl Pts',(2.39337207631613,1.,2.95085857128372));
#47044=CARTESIAN_POINT('Ctrl Pts',(2.38914929090806,1.,2.94404820669135));
#47045=CARTESIAN_POINT('Ctrl Pts',(2.38472771516476,1.,2.93717903280599));
#47046=CARTESIAN_POINT('Ctrl Pts',(2.3802898958232,1.,2.93049643640517));
#47047=CARTESIAN_POINT('Ctrl Pts',(2.37606510524271,1.,2.92430340582912));
#47048=CARTESIAN_POINT('Ctrl Pts',(2.37229381109939,1.,2.9189150379156));
#47049=CARTESIAN_POINT('Ctrl Pts',(2.36919161373074,1.,2.91461249883016));
#47050=CARTESIAN_POINT('Ctrl Pts',(2.36707658451709,1.,2.91181344022628));
#47051=CARTESIAN_POINT('Ctrl Pts',(2.36599991765853,1.,2.91051690822262));
#47052=CARTESIAN_POINT('Ctrl Pts',(2.36553202948741,1.,2.91005770527771));
#47053=CARTESIAN_POINT('Ctrl Pts',(2.3653621118858,1.,2.90995756655559));
#47054=CARTESIAN_POINT('Ctrl Pts',(2.36531447826213,1.,2.90994629141563));
#47055=CARTESIAN_POINT('',(2.52982887637028,0.,3.35260583073571));
#47056=CARTESIAN_POINT('Ctrl Pts',(2.03668666247593,-1.,3.1487152044751));
#47057=CARTESIAN_POINT('Ctrl Pts',(2.03668666247593,1.,3.1487152044751));
#47058=CARTESIAN_POINT('Ctrl Pts',(2.03660173757879,-1.,3.14869618937258));
#47059=CARTESIAN_POINT('Ctrl Pts',(2.03660173757879,1.,3.14869618937258));
#47060=CARTESIAN_POINT('Ctrl Pts',(2.03653654935591,-1.,3.14878756590812));
#47061=CARTESIAN_POINT('Ctrl Pts',(2.03653654935591,1.,3.14878756590812));
#47062=CARTESIAN_POINT('Ctrl Pts',(2.03675273049189,-1.,3.14931281968048));
#47063=CARTESIAN_POINT('Ctrl Pts',(2.03675273049189,1.,3.14931281968048));
#47064=CARTESIAN_POINT('Ctrl Pts',(2.03766932526445,-1.,3.15079010635742));
#47065=CARTESIAN_POINT('Ctrl Pts',(2.03766932526445,1.,3.15079010635742));
#47066=CARTESIAN_POINT('Ctrl Pts',(2.03984073791519,-1.,3.15389991674792));
#47067=CARTESIAN_POINT('Ctrl Pts',(2.03984073791519,1.,3.15389991674792));
#47068=CARTESIAN_POINT('Ctrl Pts',(2.04297406404027,-1.,3.15817983946367));
#47069=CARTESIAN_POINT('Ctrl Pts',(2.04297406404027,1.,3.15817983946367));
#47070=CARTESIAN_POINT('Ctrl Pts',(2.04693331247446,-1.,3.16343165058912));
#47071=CARTESIAN_POINT('Ctrl Pts',(2.04693331247446,1.,3.16343165058912));
#47072=CARTESIAN_POINT('Ctrl Pts',(2.05151770247233,-1.,3.16936341689527));
#47073=CARTESIAN_POINT('Ctrl Pts',(2.05151770247233,1.,3.16936341689527));
#47074=CARTESIAN_POINT('Ctrl Pts',(2.05650186773132,-1.,3.17564906975371));
#47075=CARTESIAN_POINT('Ctrl Pts',(2.05650186773132,1.,3.17564906975371));
#47076=CARTESIAN_POINT('Ctrl Pts',(2.06166849827101,-1.,3.18197692964614));
#47077=CARTESIAN_POINT('Ctrl Pts',(2.06166849827101,1.,3.18197692964614));
#47078=CARTESIAN_POINT('Ctrl Pts',(2.06684062744112,-1.,3.18809755562368));
#47079=CARTESIAN_POINT('Ctrl Pts',(2.06684062744112,1.,3.18809755562368));
#47080=CARTESIAN_POINT('Ctrl Pts',(2.07192253497857,-1.,3.19388465568252));
#47081=CARTESIAN_POINT('Ctrl Pts',(2.07192253497857,1.,3.19388465568252));
#47082=CARTESIAN_POINT('Ctrl Pts',(2.07690441870722,-1.,3.19934132836019));
#47083=CARTESIAN_POINT('Ctrl Pts',(2.07690441870722,1.,3.19934132836019));
#47084=CARTESIAN_POINT('Ctrl Pts',(2.08182850370878,-1.,3.2045481863073));
#47085=CARTESIAN_POINT('Ctrl Pts',(2.08182850370878,1.,3.2045481863073));
#47086=CARTESIAN_POINT('Ctrl Pts',(2.08676465517455,-1.,3.20962575845463));
#47087=CARTESIAN_POINT('Ctrl Pts',(2.08676465517455,1.,3.20962575845463));
#47088=CARTESIAN_POINT('Ctrl Pts',(2.09178419460443,-1.,3.21469429601654));
#47089=CARTESIAN_POINT('Ctrl Pts',(2.09178419460443,1.,3.21469429601654));
#47090=CARTESIAN_POINT('Ctrl Pts',(2.09692958434895,-1.,3.21982707347009));
#47091=CARTESIAN_POINT('Ctrl Pts',(2.09692958434895,1.,3.21982707347009));
#47092=CARTESIAN_POINT('Ctrl Pts',(2.10220384298492,-1.,3.22503437553434));
#47093=CARTESIAN_POINT('Ctrl Pts',(2.10220384298492,1.,3.22503437553434));
#47094=CARTESIAN_POINT('Ctrl Pts',(2.10758699642451,-1.,3.23028945793289));
#47095=CARTESIAN_POINT('Ctrl Pts',(2.10758699642451,1.,3.23028945793289));
#47096=CARTESIAN_POINT('Ctrl Pts',(2.11304604021773,-1.,3.23554444767099));
#47097=CARTESIAN_POINT('Ctrl Pts',(2.11304604021773,1.,3.23554444767099));
#47098=CARTESIAN_POINT('Ctrl Pts',(2.11854673326979,-1.,3.24074905517293));
#47099=CARTESIAN_POINT('Ctrl Pts',(2.11854673326979,1.,3.24074905517293));
#47100=CARTESIAN_POINT('Ctrl Pts',(2.12406646410962,-1.,3.24587102613376));
#47101=CARTESIAN_POINT('Ctrl Pts',(2.12406646410962,1.,3.24587102613376));
#47102=CARTESIAN_POINT('Ctrl Pts',(2.12960028396832,-1.,3.25090574494028));
#47103=CARTESIAN_POINT('Ctrl Pts',(2.12960028396832,1.,3.25090574494028));
#47104=CARTESIAN_POINT('Ctrl Pts',(2.13515375878803,-1.,3.25586495065054));
#47105=CARTESIAN_POINT('Ctrl Pts',(2.13515375878803,1.,3.25586495065054));
#47106=CARTESIAN_POINT('Ctrl Pts',(2.14073870754264,-1.,3.26077002641879));
#47107=CARTESIAN_POINT('Ctrl Pts',(2.14073870754264,1.,3.26077002641879));
#47108=CARTESIAN_POINT('Ctrl Pts',(2.1463680529566,-1.,3.26564388189759));
#47109=CARTESIAN_POINT('Ctrl Pts',(2.1463680529566,1.,3.26564388189759));
#47110=CARTESIAN_POINT('Ctrl Pts',(2.15205043199808,-1.,3.27050245897228));
#47111=CARTESIAN_POINT('Ctrl Pts',(2.15205043199808,1.,3.27050245897228));
#47112=CARTESIAN_POINT('Ctrl Pts',(2.15778690038347,-1.,3.27534954469187));
#47113=CARTESIAN_POINT('Ctrl Pts',(2.15778690038347,1.,3.27534954469187));
#47114=CARTESIAN_POINT('Ctrl Pts',(2.16357391934425,-1.,3.280181508414));
#47115=CARTESIAN_POINT('Ctrl Pts',(2.16357391934425,1.,3.280181508414));
#47116=CARTESIAN_POINT('Ctrl Pts',(2.16940517773455,-1.,3.28499019979724));
#47117=CARTESIAN_POINT('Ctrl Pts',(2.16940517773455,1.,3.28499019979724));
#47118=CARTESIAN_POINT('Ctrl Pts',(2.17527380048423,-1.,3.28976645712568));
#47119=CARTESIAN_POINT('Ctrl Pts',(2.17527380048423,1.,3.28976645712568));
#47120=CARTESIAN_POINT('Ctrl Pts',(2.18117455557065,-1.,3.2945036150049));
#47121=CARTESIAN_POINT('Ctrl Pts',(2.18117455557065,1.,3.2945036150049));
#47122=CARTESIAN_POINT('Ctrl Pts',(2.18710556500327,-1.,3.29920022557639));
#47123=CARTESIAN_POINT('Ctrl Pts',(2.18710556500327,1.,3.29920022557639));
#47124=CARTESIAN_POINT('Ctrl Pts',(2.19306710376111,-1.,3.30385816281831));
#47125=CARTESIAN_POINT('Ctrl Pts',(2.19306710376111,1.,3.30385816281831));
#47126=CARTESIAN_POINT('Ctrl Pts',(2.19906078949922,-1.,3.30848134694595));
#47127=CARTESIAN_POINT('Ctrl Pts',(2.19906078949922,1.,3.30848134694595));
#47128=CARTESIAN_POINT('Ctrl Pts',(2.20508863150607,-1.,3.31307424608949));
#47129=CARTESIAN_POINT('Ctrl Pts',(2.20508863150607,1.,3.31307424608949));
#47130=CARTESIAN_POINT('Ctrl Pts',(2.21115211847875,-1.,3.31764044024235));
#47131=CARTESIAN_POINT('Ctrl Pts',(2.21115211847875,1.,3.31764044024235));
#47132=CARTESIAN_POINT('Ctrl Pts',(2.21725135110898,-1.,3.32218125618968));
#47133=CARTESIAN_POINT('Ctrl Pts',(2.21725135110898,1.,3.32218125618968));
#47134=CARTESIAN_POINT('Ctrl Pts',(2.22338548312772,-1.,3.3266964672289));
#47135=CARTESIAN_POINT('Ctrl Pts',(2.22338548312772,1.,3.3266964672289));
#47136=CARTESIAN_POINT('Ctrl Pts',(2.22955308907233,-1.,3.33118487773611));
#47137=CARTESIAN_POINT('Ctrl Pts',(2.22955308907233,1.,3.33118487773611));
#47138=CARTESIAN_POINT('Ctrl Pts',(2.23575256328812,-1.,3.33564495756482));
#47139=CARTESIAN_POINT('Ctrl Pts',(2.23575256328812,1.,3.33564495756482));
#47140=CARTESIAN_POINT('Ctrl Pts',(2.24198249391422,-1.,3.34007543738025));
#47141=CARTESIAN_POINT('Ctrl Pts',(2.24198249391422,1.,3.34007543738025));
#47142=CARTESIAN_POINT('Ctrl Pts',(2.24824207678256,-1.,3.34447596770723));
#47143=CARTESIAN_POINT('Ctrl Pts',(2.24824207678256,1.,3.34447596770723));
#47144=CARTESIAN_POINT('Ctrl Pts',(2.25453097693483,-1.,3.34884690292285));
#47145=CARTESIAN_POINT('Ctrl Pts',(2.25453097693483,1.,3.34884690292285));
#47146=CARTESIAN_POINT('Ctrl Pts',(2.26084915222449,-1.,3.35318902552626));
#47147=CARTESIAN_POINT('Ctrl Pts',(2.26084915222449,1.,3.35318902552626));
#47148=CARTESIAN_POINT('Ctrl Pts',(2.26719668579909,-1.,3.35750328523061));
#47149=CARTESIAN_POINT('Ctrl Pts',(2.26719668579909,1.,3.35750328523061));
#47150=CARTESIAN_POINT('Ctrl Pts',(2.2735736262093,-1.,3.36179055004409));
#47151=CARTESIAN_POINT('Ctrl Pts',(2.2735736262093,1.,3.36179055004409));
#47152=CARTESIAN_POINT('Ctrl Pts',(2.27997979458037,-1.,3.36605130713076));
#47153=CARTESIAN_POINT('Ctrl Pts',(2.27997979458037,1.,3.36605130713076));
#47154=CARTESIAN_POINT('Ctrl Pts',(2.28641481081137,-1.,3.37028570206488));
#47155=CARTESIAN_POINT('Ctrl Pts',(2.28641481081137,1.,3.37028570206488));
#47156=CARTESIAN_POINT('Ctrl Pts',(2.29287818007393,-1.,3.37449367172826));
#47157=CARTESIAN_POINT('Ctrl Pts',(2.29287818007393,1.,3.37449367172826));
#47158=CARTESIAN_POINT('Ctrl Pts',(2.29936936127624,-1.,3.37867504959433));
#47159=CARTESIAN_POINT('Ctrl Pts',(2.29936936127624,1.,3.37867504959433));
#47160=CARTESIAN_POINT('Ctrl Pts',(2.30588783640343,-1.,3.3828296733661));
#47161=CARTESIAN_POINT('Ctrl Pts',(2.30588783640343,1.,3.3828296733661));
#47162=CARTESIAN_POINT('Ctrl Pts',(2.31243319489367,-1.,3.38695751492462));
#47163=CARTESIAN_POINT('Ctrl Pts',(2.31243319489367,1.,3.38695751492462));
#47164=CARTESIAN_POINT('Ctrl Pts',(2.31900513925424,-1.,3.39105869474822));
#47165=CARTESIAN_POINT('Ctrl Pts',(2.31900513925424,1.,3.39105869474822));
#47166=CARTESIAN_POINT('Ctrl Pts',(2.3256034390248,-1.,3.39513342019756));
#47167=CARTESIAN_POINT('Ctrl Pts',(2.3256034390248,1.,3.39513342019756));
#47168=CARTESIAN_POINT('Ctrl Pts',(2.33222789882489,-1.,3.39918194577956));
#47169=CARTESIAN_POINT('Ctrl Pts',(2.33222789882489,1.,3.39918194577956));
#47170=CARTESIAN_POINT('Ctrl Pts',(2.33887832342782,-1.,3.40320452776743));
#47171=CARTESIAN_POINT('Ctrl Pts',(2.33887832342782,1.,3.40320452776743));
#47172=CARTESIAN_POINT('Ctrl Pts',(2.34555447649188,-1.,3.40720137404297));
#47173=CARTESIAN_POINT('Ctrl Pts',(2.34555447649188,1.,3.40720137404297));
#47174=CARTESIAN_POINT('Ctrl Pts',(2.35225606824109,-1.,3.41117262314119));
#47175=CARTESIAN_POINT('Ctrl Pts',(2.35225606824109,1.,3.41117262314119));
#47176=CARTESIAN_POINT('Ctrl Pts',(2.35898278606946,-1.,3.41511836751469));
#47177=CARTESIAN_POINT('Ctrl Pts',(2.35898278606946,1.,3.41511836751469));
#47178=CARTESIAN_POINT('Ctrl Pts',(2.36573431470642,-1.,3.41903866635852));
#47179=CARTESIAN_POINT('Ctrl Pts',(2.36573431470642,1.,3.41903866635852));
#47180=CARTESIAN_POINT('Ctrl Pts',(2.37251035954292,-1.,3.42293356216511));
#47181=CARTESIAN_POINT('Ctrl Pts',(2.37251035954292,1.,3.42293356216511));
#47182=CARTESIAN_POINT('Ctrl Pts',(2.37931067028926,-1.,3.42680309754399));
#47183=CARTESIAN_POINT('Ctrl Pts',(2.37931067028926,1.,3.42680309754399));
#47184=CARTESIAN_POINT('Ctrl Pts',(2.38613505843552,-1.,3.4306473271292));
#47185=CARTESIAN_POINT('Ctrl Pts',(2.38613505843552,1.,3.4306473271292));
#47186=CARTESIAN_POINT('Ctrl Pts',(2.39298338804493,-1.,3.4344663067854));
#47187=CARTESIAN_POINT('Ctrl Pts',(2.39298338804493,1.,3.4344663067854));
#47188=CARTESIAN_POINT('Ctrl Pts',(2.39848113410292,-1.,3.43750133064416));
#47189=CARTESIAN_POINT('Ctrl Pts',(2.39848113410292,1.,3.43750133064416));
#47190=CARTESIAN_POINT('Ctrl Pts',(2.40261515589405,-1.,3.43976627484234));
#47191=CARTESIAN_POINT('Ctrl Pts',(2.40261515589405,1.,3.43976627484234));
#47192=CARTESIAN_POINT('Ctrl Pts',(2.4053759295909,-1.,3.44127120683039));
#47193=CARTESIAN_POINT('Ctrl Pts',(2.4053759295909,1.,3.44127120683039));
#47194=CARTESIAN_POINT('Ctrl Pts',(2.40675750623143,-1.,3.44202241512147));
#47195=CARTESIAN_POINT('Ctrl Pts',(2.40675750623143,1.,3.44202241512147));
#47196=CARTESIAN_POINT('',(2.03660101169714,1.,3.14877060440328));
#47197=CARTESIAN_POINT('Ctrl Pts',(2.03660101169714,-1.,3.14877060440327));
#47198=CARTESIAN_POINT('Ctrl Pts',(2.03660101169714,-0.666666666666667,
3.14877060440327));
#47199=CARTESIAN_POINT('Ctrl Pts',(2.03660101169714,-0.333333333333333,
3.14877060440327));
#47200=CARTESIAN_POINT('Ctrl Pts',(2.03660101169714,0.333333333333333,3.14877060440327));
#47201=CARTESIAN_POINT('Ctrl Pts',(2.03660101169714,0.666666666666667,3.14877060440327));
#47202=CARTESIAN_POINT('Ctrl Pts',(2.03660101169714,1.,3.14877060440327));
#47203=CARTESIAN_POINT('',(2.40675750623143,1.,3.44202241512147));
#47204=CARTESIAN_POINT('',(2.40675750623143,0.,3.44202241512147));
#47205=CARTESIAN_POINT('Ctrl Pts',(2.03660101169714,1.,3.14877060440328));
#47206=CARTESIAN_POINT('Ctrl Pts',(2.03659701539259,1.,3.14881939088124));
#47207=CARTESIAN_POINT('Ctrl Pts',(2.03663974554932,1.,3.1490119366901));
#47208=CARTESIAN_POINT('Ctrl Pts',(2.03693188810545,1.,3.14959882629805));
#47209=CARTESIAN_POINT('Ctrl Pts',(2.03783225495961,1.,3.15102344775328));
#47210=CARTESIAN_POINT('Ctrl Pts',(2.03984073791519,1.,3.15389991674792));
#47211=CARTESIAN_POINT('Ctrl Pts',(2.04297406404027,1.,3.15817983946367));
#47212=CARTESIAN_POINT('Ctrl Pts',(2.04693331247446,1.,3.16343165058912));
#47213=CARTESIAN_POINT('Ctrl Pts',(2.05151770247233,1.,3.16936341689527));
#47214=CARTESIAN_POINT('Ctrl Pts',(2.05650186773132,1.,3.17564906975371));
#47215=CARTESIAN_POINT('Ctrl Pts',(2.06166849827101,1.,3.18197692964614));
#47216=CARTESIAN_POINT('Ctrl Pts',(2.06684062744112,1.,3.18809755562368));
#47217=CARTESIAN_POINT('Ctrl Pts',(2.07192253497857,1.,3.19388465568252));
#47218=CARTESIAN_POINT('Ctrl Pts',(2.07690441870722,1.,3.19934132836019));
#47219=CARTESIAN_POINT('Ctrl Pts',(2.08182850370878,1.,3.2045481863073));
#47220=CARTESIAN_POINT('Ctrl Pts',(2.08676465517455,1.,3.20962575845463));
#47221=CARTESIAN_POINT('Ctrl Pts',(2.09178419460443,1.,3.21469429601654));
#47222=CARTESIAN_POINT('Ctrl Pts',(2.09692958434895,1.,3.21982707347009));
#47223=CARTESIAN_POINT('Ctrl Pts',(2.10220384298492,1.,3.22503437553434));
#47224=CARTESIAN_POINT('Ctrl Pts',(2.10758699642451,1.,3.23028945793289));
#47225=CARTESIAN_POINT('Ctrl Pts',(2.11304604021773,1.,3.23554444767099));
#47226=CARTESIAN_POINT('Ctrl Pts',(2.11854673326979,1.,3.24074905517293));
#47227=CARTESIAN_POINT('Ctrl Pts',(2.12406646410962,1.,3.24587102613376));
#47228=CARTESIAN_POINT('Ctrl Pts',(2.12960028396832,1.,3.25090574494028));
#47229=CARTESIAN_POINT('Ctrl Pts',(2.13515375878803,1.,3.25586495065054));
#47230=CARTESIAN_POINT('Ctrl Pts',(2.14073870754264,1.,3.26077002641879));
#47231=CARTESIAN_POINT('Ctrl Pts',(2.1463680529566,1.,3.26564388189759));
#47232=CARTESIAN_POINT('Ctrl Pts',(2.15205043199808,1.,3.27050245897228));
#47233=CARTESIAN_POINT('Ctrl Pts',(2.15778690038347,1.,3.27534954469187));
#47234=CARTESIAN_POINT('Ctrl Pts',(2.16357391934425,1.,3.280181508414));
#47235=CARTESIAN_POINT('Ctrl Pts',(2.16940517773455,1.,3.28499019979724));
#47236=CARTESIAN_POINT('Ctrl Pts',(2.17527380048423,1.,3.28976645712568));
#47237=CARTESIAN_POINT('Ctrl Pts',(2.18117455557065,1.,3.2945036150049));
#47238=CARTESIAN_POINT('Ctrl Pts',(2.18710556500327,1.,3.29920022557639));
#47239=CARTESIAN_POINT('Ctrl Pts',(2.19306710376111,1.,3.30385816281831));
#47240=CARTESIAN_POINT('Ctrl Pts',(2.19906078949922,1.,3.30848134694595));
#47241=CARTESIAN_POINT('Ctrl Pts',(2.20508863150607,1.,3.31307424608949));
#47242=CARTESIAN_POINT('Ctrl Pts',(2.21115211847875,1.,3.31764044024235));
#47243=CARTESIAN_POINT('Ctrl Pts',(2.21725135110898,1.,3.32218125618968));
#47244=CARTESIAN_POINT('Ctrl Pts',(2.22338548312772,1.,3.3266964672289));
#47245=CARTESIAN_POINT('Ctrl Pts',(2.22955308907233,1.,3.33118487773611));
#47246=CARTESIAN_POINT('Ctrl Pts',(2.23575256328812,1.,3.33564495756482));
#47247=CARTESIAN_POINT('Ctrl Pts',(2.24198249391422,1.,3.34007543738025));
#47248=CARTESIAN_POINT('Ctrl Pts',(2.24824207678256,1.,3.34447596770723));
#47249=CARTESIAN_POINT('Ctrl Pts',(2.25453097693483,1.,3.34884690292285));
#47250=CARTESIAN_POINT('Ctrl Pts',(2.26084915222449,1.,3.35318902552626));
#47251=CARTESIAN_POINT('Ctrl Pts',(2.26719668579909,1.,3.35750328523061));
#47252=CARTESIAN_POINT('Ctrl Pts',(2.2735736262093,1.,3.36179055004409));
#47253=CARTESIAN_POINT('Ctrl Pts',(2.27997979458037,1.,3.36605130713076));
#47254=CARTESIAN_POINT('Ctrl Pts',(2.28641481081137,1.,3.37028570206488));
#47255=CARTESIAN_POINT('Ctrl Pts',(2.29287818007393,1.,3.37449367172826));
#47256=CARTESIAN_POINT('Ctrl Pts',(2.29936936127624,1.,3.37867504959433));
#47257=CARTESIAN_POINT('Ctrl Pts',(2.30588783640343,1.,3.3828296733661));
#47258=CARTESIAN_POINT('Ctrl Pts',(2.31243319489367,1.,3.38695751492462));
#47259=CARTESIAN_POINT('Ctrl Pts',(2.31900513925424,1.,3.39105869474822));
#47260=CARTESIAN_POINT('Ctrl Pts',(2.3256034390248,1.,3.39513342019756));
#47261=CARTESIAN_POINT('Ctrl Pts',(2.33222789882489,1.,3.39918194577956));
#47262=CARTESIAN_POINT('Ctrl Pts',(2.33887832342782,1.,3.40320452776743));
#47263=CARTESIAN_POINT('Ctrl Pts',(2.34555447649188,1.,3.40720137404297));
#47264=CARTESIAN_POINT('Ctrl Pts',(2.35225606824109,1.,3.41117262314119));
#47265=CARTESIAN_POINT('Ctrl Pts',(2.35898278606946,1.,3.41511836751469));
#47266=CARTESIAN_POINT('Ctrl Pts',(2.36573431470642,1.,3.41903866635852));
#47267=CARTESIAN_POINT('Ctrl Pts',(2.37251035954292,1.,3.42293356216511));
#47268=CARTESIAN_POINT('Ctrl Pts',(2.37931067028926,1.,3.42680309754399));
#47269=CARTESIAN_POINT('Ctrl Pts',(2.38613505843552,1.,3.4306473271292));
#47270=CARTESIAN_POINT('Ctrl Pts',(2.39298338804493,1.,3.4344663067854));
#47271=CARTESIAN_POINT('Ctrl Pts',(2.39848113410292,1.,3.43750133064416));
#47272=CARTESIAN_POINT('Ctrl Pts',(2.40261515589405,1.,3.43976627484234));
#47273=CARTESIAN_POINT('Ctrl Pts',(2.4053759295909,1.,3.44127120683039));
#47274=CARTESIAN_POINT('Ctrl Pts',(2.40675750623143,1.,3.44202241512147));
#47275=CARTESIAN_POINT('Origin',(2.40675750623143,0.,3.44202241512147));
#47276=CARTESIAN_POINT('',(2.52982887637028,1.,3.35260583073571));
#47277=CARTESIAN_POINT('Origin',(0.,0.,0.));
#47278=CARTESIAN_POINT('',(1.88097764062697,1.,3.24413672884812));
#47279=CARTESIAN_POINT('Origin',(0.,1.,0.));
#47280=CARTESIAN_POINT('Ctrl Pts',(1.88097764062697,1.,3.24413672884812));
#47281=CARTESIAN_POINT('Ctrl Pts',(1.88097764062697,0.666666666666667,3.24413672884812));
#47282=CARTESIAN_POINT('Ctrl Pts',(1.88097764062697,0.333333333333333,3.24413672884812));
#47283=CARTESIAN_POINT('Ctrl Pts',(1.88097764062697,-0.333333333333333,
3.24413672884812));
#47284=CARTESIAN_POINT('Ctrl Pts',(1.88097764062697,-0.666666666666667,
3.24413672884812));
#47285=CARTESIAN_POINT('Ctrl Pts',(1.88097764062697,-1.,3.24413672884812));
#47286=CARTESIAN_POINT('Ctrl Pts',(1.97421938526992,-1.,3.70708211654725));
#47287=CARTESIAN_POINT('Ctrl Pts',(1.97421938526992,1.,3.70708211654725));
#47288=CARTESIAN_POINT('Ctrl Pts',(1.97417727645308,-1.,3.70551008132332));
#47289=CARTESIAN_POINT('Ctrl Pts',(1.97417727645308,1.,3.70551008132332));
#47290=CARTESIAN_POINT('Ctrl Pts',(1.97408973726715,-1.,3.70236698912904));
#47291=CARTESIAN_POINT('Ctrl Pts',(1.97408973726715,1.,3.70236698912904));
#47292=CARTESIAN_POINT('Ctrl Pts',(1.97394846383216,-1.,3.6976552856004));
#47293=CARTESIAN_POINT('Ctrl Pts',(1.97394846383216,1.,3.6976552856004));
#47294=CARTESIAN_POINT('Ctrl Pts',(1.97374016225483,-1.,3.69137888599902));
#47295=CARTESIAN_POINT('Ctrl Pts',(1.97374016225483,1.,3.69137888599902));
#47296=CARTESIAN_POINT('Ctrl Pts',(1.97344650304519,-1.,3.68354319915092));
#47297=CARTESIAN_POINT('Ctrl Pts',(1.97344650304519,1.,3.68354319915092));
#47298=CARTESIAN_POINT('Ctrl Pts',(1.97311947678516,-1.,3.67571738107084));
#47299=CARTESIAN_POINT('Ctrl Pts',(1.97311947678516,1.,3.67571738107084));
#47300=CARTESIAN_POINT('Ctrl Pts',(1.97275897198678,-1.,3.66790152752075));
#47301=CARTESIAN_POINT('Ctrl Pts',(1.97275897198678,1.,3.66790152752075));
#47302=CARTESIAN_POINT('Ctrl Pts',(1.9723648543905,-1.,3.6600957816636));
#47303=CARTESIAN_POINT('Ctrl Pts',(1.9723648543905,1.,3.6600957816636));
#47304=CARTESIAN_POINT('Ctrl Pts',(1.97193697240239,-1.,3.652300347166));
#47305=CARTESIAN_POINT('Ctrl Pts',(1.97193697240239,1.,3.652300347166));
#47306=CARTESIAN_POINT('Ctrl Pts',(1.97147515441164,-1.,3.64451546723514));
#47307=CARTESIAN_POINT('Ctrl Pts',(1.97147515441164,1.,3.64451546723514));
#47308=CARTESIAN_POINT('Ctrl Pts',(1.97097920454464,-1.,3.63674139590412));
#47309=CARTESIAN_POINT('Ctrl Pts',(1.97097920454464,1.,3.63674139590412));
#47310=CARTESIAN_POINT('Ctrl Pts',(1.97044889850463,-1.,3.62897836973293));
#47311=CARTESIAN_POINT('Ctrl Pts',(1.97044889850463,1.,3.62897836973293));
#47312=CARTESIAN_POINT('Ctrl Pts',(1.96988398129978,-1.,3.62122658401893));
#47313=CARTESIAN_POINT('Ctrl Pts',(1.96988398129978,1.,3.62122658401893));
#47314=CARTESIAN_POINT('Ctrl Pts',(1.96928416040877,-1.,3.61348615496704));
#47315=CARTESIAN_POINT('Ctrl Pts',(1.96928416040877,1.,3.61348615496704));
#47316=CARTESIAN_POINT('Ctrl Pts',(1.9686491188594,-1.,3.60575714017989));
#47317=CARTESIAN_POINT('Ctrl Pts',(1.9686491188594,1.,3.60575714017989));
#47318=CARTESIAN_POINT('Ctrl Pts',(1.96797854118369,-1.,3.59803959819938));
#47319=CARTESIAN_POINT('Ctrl Pts',(1.96797854118369,1.,3.59803959819938));
#47320=CARTESIAN_POINT('Ctrl Pts',(1.96727213799544,-1.,3.59033364022801));
#47321=CARTESIAN_POINT('Ctrl Pts',(1.96727213799544,1.,3.59033364022801));
#47322=CARTESIAN_POINT('Ctrl Pts',(1.96652966688911,-1.,3.58263947663829));
#47323=CARTESIAN_POINT('Ctrl Pts',(1.96652966688911,1.,3.58263947663829));
#47324=CARTESIAN_POINT('Ctrl Pts',(1.96575096652789,-1.,3.57495748600959));
#47325=CARTESIAN_POINT('Ctrl Pts',(1.96575096652789,1.,3.57495748600959));
#47326=CARTESIAN_POINT('Ctrl Pts',(1.96493594634567,-1.,3.56728820357791));
#47327=CARTESIAN_POINT('Ctrl Pts',(1.96493594634567,1.,3.56728820357791));
#47328=CARTESIAN_POINT('Ctrl Pts',(1.96408450906812,-1.,3.55963218706096));
#47329=CARTESIAN_POINT('Ctrl Pts',(1.96408450906812,1.,3.55963218706096));
#47330=CARTESIAN_POINT('Ctrl Pts',(1.96319648628644,-1.,3.55198990600886));
#47331=CARTESIAN_POINT('Ctrl Pts',(1.96319648628644,1.,3.55198990600886));
#47332=CARTESIAN_POINT('Ctrl Pts',(1.96227157573067,-1.,3.54436163300443));
#47333=CARTESIAN_POINT('Ctrl Pts',(1.96227157573067,1.,3.54436163300443));
#47334=CARTESIAN_POINT('Ctrl Pts',(1.96130926212689,-1.,3.53674730625813));
#47335=CARTESIAN_POINT('Ctrl Pts',(1.96130926212689,1.,3.53674730625813));
#47336=CARTESIAN_POINT('Ctrl Pts',(1.96030879411566,-1.,3.52914648844351));
#47337=CARTESIAN_POINT('Ctrl Pts',(1.96030879411566,1.,3.52914648844351));
#47338=CARTESIAN_POINT('Ctrl Pts',(1.95926936324461,-1.,3.52155867431486));
#47339=CARTESIAN_POINT('Ctrl Pts',(1.95926936324461,1.,3.52155867431486));
#47340=CARTESIAN_POINT('Ctrl Pts',(1.95819025316779,-1.,3.51398354617794));
#47341=CARTESIAN_POINT('Ctrl Pts',(1.95819025316779,1.,3.51398354617794));
#47342=CARTESIAN_POINT('Ctrl Pts',(1.95707099606511,-1.,3.50642124159909));
#47343=CARTESIAN_POINT('Ctrl Pts',(1.95707099606511,1.,3.50642124159909));
#47344=CARTESIAN_POINT('Ctrl Pts',(1.95591153823661,-1.,3.49887263575583));
#47345=CARTESIAN_POINT('Ctrl Pts',(1.95591153823661,1.,3.49887263575583));
#47346=CARTESIAN_POINT('Ctrl Pts',(1.95471236969643,-1.,3.49133956289133));
#47347=CARTESIAN_POINT('Ctrl Pts',(1.95471236969643,1.,3.49133956289133));
#47348=CARTESIAN_POINT('Ctrl Pts',(1.95347412486308,-1.,3.48382414832634));
#47349=CARTESIAN_POINT('Ctrl Pts',(1.95347412486308,1.,3.48382414832634));
#47350=CARTESIAN_POINT('Ctrl Pts',(1.95219722189876,-1.,3.47632820495921));
#47351=CARTESIAN_POINT('Ctrl Pts',(1.95219722189876,1.,3.47632820495921));
#47352=CARTESIAN_POINT('Ctrl Pts',(1.95088147859876,-1.,3.46885258974191));
#47353=CARTESIAN_POINT('Ctrl Pts',(1.95088147859876,1.,3.46885258974191));
#47354=CARTESIAN_POINT('Ctrl Pts',(1.94952575850197,-1.,3.46139661060962));
#47355=CARTESIAN_POINT('Ctrl Pts',(1.94952575850197,1.,3.46139661060962));
#47356=CARTESIAN_POINT('Ctrl Pts',(1.94812754766524,-1.,3.45395731584051));
#47357=CARTESIAN_POINT('Ctrl Pts',(1.94812754766524,1.,3.45395731584051));
#47358=CARTESIAN_POINT('Ctrl Pts',(1.94668377715329,-1.,3.44653088665681));
#47359=CARTESIAN_POINT('Ctrl Pts',(1.94668377715329,1.,3.44653088665681));
#47360=CARTESIAN_POINT('Ctrl Pts',(1.94519168842879,-1.,3.43911410197687));
#47361=CARTESIAN_POINT('Ctrl Pts',(1.94519168842879,1.,3.43911410197687));
#47362=CARTESIAN_POINT('Ctrl Pts',(1.94364973660284,-1.,3.43170586602434));
#47363=CARTESIAN_POINT('Ctrl Pts',(1.94364973660284,1.,3.43170586602434));
#47364=CARTESIAN_POINT('Ctrl Pts',(1.94205835913696,-1.,3.42430850941503));
#47365=CARTESIAN_POINT('Ctrl Pts',(1.94205835913696,1.,3.42430850941503));
#47366=CARTESIAN_POINT('Ctrl Pts',(1.94042111965246,-1.,3.41692971994096));
#47367=CARTESIAN_POINT('Ctrl Pts',(1.94042111965246,1.,3.41692971994096));
#47368=CARTESIAN_POINT('Ctrl Pts',(1.93874306008143,-1.,3.40957978266642));
#47369=CARTESIAN_POINT('Ctrl Pts',(1.93874306008143,1.,3.40957978266642));
#47370=CARTESIAN_POINT('Ctrl Pts',(1.93702857723098,-1.,3.40226802104109));
#47371=CARTESIAN_POINT('Ctrl Pts',(1.93702857723098,1.,3.40226802104109));
#47372=CARTESIAN_POINT('Ctrl Pts',(1.93527929945985,-1.,3.39499923640795));
#47373=CARTESIAN_POINT('Ctrl Pts',(1.93527929945985,1.,3.39499923640795));
#47374=CARTESIAN_POINT('Ctrl Pts',(1.93349233176788,-1.,3.38777076883256));
#47375=CARTESIAN_POINT('Ctrl Pts',(1.93349233176788,1.,3.38777076883256));
#47376=CARTESIAN_POINT('Ctrl Pts',(1.93165739093276,-1.,3.3805676852555));
#47377=CARTESIAN_POINT('Ctrl Pts',(1.93165739093276,1.,3.3805676852555));
#47378=CARTESIAN_POINT('Ctrl Pts',(1.92975993109877,-1.,3.37336807068043));
#47379=CARTESIAN_POINT('Ctrl Pts',(1.92975993109877,1.,3.37336807068043));
#47380=CARTESIAN_POINT('Ctrl Pts',(1.92778626543786,-1.,3.36615168657567));
#47381=CARTESIAN_POINT('Ctrl Pts',(1.92778626543786,1.,3.36615168657567));
#47382=CARTESIAN_POINT('Ctrl Pts',(1.92572846125756,-1.,3.35890824422965));
#47383=CARTESIAN_POINT('Ctrl Pts',(1.92572846125756,1.,3.35890824422965));
#47384=CARTESIAN_POINT('Ctrl Pts',(1.92358838440528,-1.,3.35164424847223));
#47385=CARTESIAN_POINT('Ctrl Pts',(1.92358838440528,1.,3.35164424847223));
#47386=CARTESIAN_POINT('Ctrl Pts',(1.92138450828404,-1.,3.34439448941961));
#47387=CARTESIAN_POINT('Ctrl Pts',(1.92138450828404,1.,3.34439448941961));
#47388=CARTESIAN_POINT('Ctrl Pts',(1.9191460961021,-1.,3.33721230710012));
#47389=CARTESIAN_POINT('Ctrl Pts',(1.9191460961021,1.,3.33721230710012));
#47390=CARTESIAN_POINT('Ctrl Pts',(1.91690081930331,-1.,3.33014884257873));
#47391=CARTESIAN_POINT('Ctrl Pts',(1.91690081930331,1.,3.33014884257873));
#47392=CARTESIAN_POINT('Ctrl Pts',(1.91466343916627,-1.,3.32323403454535));
#47393=CARTESIAN_POINT('Ctrl Pts',(1.91466343916627,1.,3.32323403454535));
#47394=CARTESIAN_POINT('Ctrl Pts',(1.91242616234442,-1.,3.31646052426364));
#47395=CARTESIAN_POINT('Ctrl Pts',(1.91242616234442,1.,3.31646052426364));
#47396=CARTESIAN_POINT('Ctrl Pts',(1.91014297830446,-1.,3.30975721158596));
#47397=CARTESIAN_POINT('Ctrl Pts',(1.91014297830446,1.,3.30975721158596));
#47398=CARTESIAN_POINT('Ctrl Pts',(1.90773912171341,-1.,3.30300595568195));
#47399=CARTESIAN_POINT('Ctrl Pts',(1.90773912171341,1.,3.30300595568195));
#47400=CARTESIAN_POINT('Ctrl Pts',(1.90513891864087,-1.,3.29608978722113));
#47401=CARTESIAN_POINT('Ctrl Pts',(1.90513891864087,1.,3.29608978722113));
#47402=CARTESIAN_POINT('Ctrl Pts',(1.90228971247527,-1.,3.2889344860029));
#47403=CARTESIAN_POINT('Ctrl Pts',(1.90228971247527,1.,3.2889344860029));
#47404=CARTESIAN_POINT('Ctrl Pts',(1.89918429230462,-1.,3.28154737912352));
#47405=CARTESIAN_POINT('Ctrl Pts',(1.89918429230462,1.,3.28154737912352));
#47406=CARTESIAN_POINT('Ctrl Pts',(1.89589172903793,-1.,3.27407108933139));
#47407=CARTESIAN_POINT('Ctrl Pts',(1.89589172903793,1.,3.27407108933139));
#47408=CARTESIAN_POINT('Ctrl Pts',(1.89255393500965,-1.,3.26677653888676));
#47409=CARTESIAN_POINT('Ctrl Pts',(1.89255393500965,1.,3.26677653888676));
#47410=CARTESIAN_POINT('Ctrl Pts',(1.88934996203698,-1.,3.25999885193947));
#47411=CARTESIAN_POINT('Ctrl Pts',(1.88934996203698,1.,3.25999885193947));
#47412=CARTESIAN_POINT('Ctrl Pts',(1.88646802523466,-1.,3.25408686339463));
#47413=CARTESIAN_POINT('Ctrl Pts',(1.88646802523466,1.,3.25408686339463));
#47414=CARTESIAN_POINT('Ctrl Pts',(1.88407708646357,-1.,3.24935200511918));
#47415=CARTESIAN_POINT('Ctrl Pts',(1.88407708646357,1.,3.24935200511918));
#47416=CARTESIAN_POINT('Ctrl Pts',(1.88229202582941,-1.,3.24600543790443));
#47417=CARTESIAN_POINT('Ctrl Pts',(1.88229202582941,1.,3.24600543790443));
#47418=CARTESIAN_POINT('Ctrl Pts',(1.88139187908074,-1.,3.24451807186481));
#47419=CARTESIAN_POINT('Ctrl Pts',(1.88139187908074,1.,3.24451807186481));
#47420=CARTESIAN_POINT('Ctrl Pts',(1.88102201872555,-1.,3.24408699284121));
#47421=CARTESIAN_POINT('Ctrl Pts',(1.88102201872555,1.,3.24408699284121));
#47422=CARTESIAN_POINT('Ctrl Pts',(1.88091100680349,-1.,3.24410359189609));
#47423=CARTESIAN_POINT('Ctrl Pts',(1.88091100680349,1.,3.24410359189609));
#47424=CARTESIAN_POINT('Ctrl Pts',(1.8808893942881,-1.,3.24418789321065));
#47425=CARTESIAN_POINT('Ctrl Pts',(1.8808893942881,1.,3.24418789321065));
#47426=CARTESIAN_POINT('',(1.97421938526992,1.,3.70708211654725));
#47427=CARTESIAN_POINT('Ctrl Pts',(1.97421938526992,1.,3.70708211654725));
#47428=CARTESIAN_POINT('Ctrl Pts',(1.97417727645308,1.,3.70551008132332));
#47429=CARTESIAN_POINT('Ctrl Pts',(1.97408973726715,1.,3.70236698912904));
#47430=CARTESIAN_POINT('Ctrl Pts',(1.97394846383216,1.,3.6976552856004));
#47431=CARTESIAN_POINT('Ctrl Pts',(1.97374016225483,1.,3.69137888599902));
#47432=CARTESIAN_POINT('Ctrl Pts',(1.97344650304519,1.,3.68354319915092));
#47433=CARTESIAN_POINT('Ctrl Pts',(1.97311947678516,1.,3.67571738107084));
#47434=CARTESIAN_POINT('Ctrl Pts',(1.97275897198678,1.,3.66790152752075));
#47435=CARTESIAN_POINT('Ctrl Pts',(1.9723648543905,1.,3.6600957816636));
#47436=CARTESIAN_POINT('Ctrl Pts',(1.97193697240239,1.,3.652300347166));
#47437=CARTESIAN_POINT('Ctrl Pts',(1.97147515441164,1.,3.64451546723514));
#47438=CARTESIAN_POINT('Ctrl Pts',(1.97097920454464,1.,3.63674139590412));
#47439=CARTESIAN_POINT('Ctrl Pts',(1.97044889850463,1.,3.62897836973293));
#47440=CARTESIAN_POINT('Ctrl Pts',(1.96988398129978,1.,3.62122658401893));
#47441=CARTESIAN_POINT('Ctrl Pts',(1.96928416040877,1.,3.61348615496704));
#47442=CARTESIAN_POINT('Ctrl Pts',(1.9686491188594,1.,3.60575714017989));
#47443=CARTESIAN_POINT('Ctrl Pts',(1.96797854118369,1.,3.59803959819938));
#47444=CARTESIAN_POINT('Ctrl Pts',(1.96727213799544,1.,3.59033364022801));
#47445=CARTESIAN_POINT('Ctrl Pts',(1.96652966688911,1.,3.58263947663829));
#47446=CARTESIAN_POINT('Ctrl Pts',(1.96575096652789,1.,3.57495748600959));
#47447=CARTESIAN_POINT('Ctrl Pts',(1.96493594634567,1.,3.56728820357791));
#47448=CARTESIAN_POINT('Ctrl Pts',(1.96408450906812,1.,3.55963218706096));
#47449=CARTESIAN_POINT('Ctrl Pts',(1.96319648628644,1.,3.55198990600886));
#47450=CARTESIAN_POINT('Ctrl Pts',(1.96227157573067,1.,3.54436163300443));
#47451=CARTESIAN_POINT('Ctrl Pts',(1.96130926212689,1.,3.53674730625813));
#47452=CARTESIAN_POINT('Ctrl Pts',(1.96030879411566,1.,3.52914648844351));
#47453=CARTESIAN_POINT('Ctrl Pts',(1.95926936324461,1.,3.52155867431486));
#47454=CARTESIAN_POINT('Ctrl Pts',(1.95819025316779,1.,3.51398354617794));
#47455=CARTESIAN_POINT('Ctrl Pts',(1.95707099606511,1.,3.50642124159909));
#47456=CARTESIAN_POINT('Ctrl Pts',(1.95591153823661,1.,3.49887263575583));
#47457=CARTESIAN_POINT('Ctrl Pts',(1.95471236969643,1.,3.49133956289133));
#47458=CARTESIAN_POINT('Ctrl Pts',(1.95347412486308,1.,3.48382414832634));
#47459=CARTESIAN_POINT('Ctrl Pts',(1.95219722189876,1.,3.47632820495921));
#47460=CARTESIAN_POINT('Ctrl Pts',(1.95088147859876,1.,3.46885258974191));
#47461=CARTESIAN_POINT('Ctrl Pts',(1.94952575850197,1.,3.46139661060962));
#47462=CARTESIAN_POINT('Ctrl Pts',(1.94812754766524,1.,3.45395731584051));
#47463=CARTESIAN_POINT('Ctrl Pts',(1.94668377715329,1.,3.44653088665681));
#47464=CARTESIAN_POINT('Ctrl Pts',(1.94519168842879,1.,3.43911410197687));
#47465=CARTESIAN_POINT('Ctrl Pts',(1.94364973660284,1.,3.43170586602434));
#47466=CARTESIAN_POINT('Ctrl Pts',(1.94205835913696,1.,3.42430850941503));
#47467=CARTESIAN_POINT('Ctrl Pts',(1.94042111965246,1.,3.41692971994096));
#47468=CARTESIAN_POINT('Ctrl Pts',(1.93874306008143,1.,3.40957978266642));
#47469=CARTESIAN_POINT('Ctrl Pts',(1.93702857723098,1.,3.40226802104109));
#47470=CARTESIAN_POINT('Ctrl Pts',(1.93527929945985,1.,3.39499923640795));
#47471=CARTESIAN_POINT('Ctrl Pts',(1.93349233176788,1.,3.38777076883256));
#47472=CARTESIAN_POINT('Ctrl Pts',(1.93165739093276,1.,3.3805676852555));
#47473=CARTESIAN_POINT('Ctrl Pts',(1.92975993109877,1.,3.37336807068043));
#47474=CARTESIAN_POINT('Ctrl Pts',(1.92778626543786,1.,3.36615168657567));
#47475=CARTESIAN_POINT('Ctrl Pts',(1.92572846125756,1.,3.35890824422965));
#47476=CARTESIAN_POINT('Ctrl Pts',(1.92358838440528,1.,3.35164424847223));
#47477=CARTESIAN_POINT('Ctrl Pts',(1.92138450828404,1.,3.34439448941961));
#47478=CARTESIAN_POINT('Ctrl Pts',(1.9191460961021,1.,3.33721230710012));
#47479=CARTESIAN_POINT('Ctrl Pts',(1.91690081930331,1.,3.33014884257873));
#47480=CARTESIAN_POINT('Ctrl Pts',(1.91466343916627,1.,3.32323403454535));
#47481=CARTESIAN_POINT('Ctrl Pts',(1.91242616234442,1.,3.31646052426364));
#47482=CARTESIAN_POINT('Ctrl Pts',(1.91014297830446,1.,3.30975721158596));
#47483=CARTESIAN_POINT('Ctrl Pts',(1.90773912171341,1.,3.30300595568195));
#47484=CARTESIAN_POINT('Ctrl Pts',(1.90513891864087,1.,3.29608978722113));
#47485=CARTESIAN_POINT('Ctrl Pts',(1.90228971247527,1.,3.2889344860029));
#47486=CARTESIAN_POINT('Ctrl Pts',(1.89918429230462,1.,3.28154737912352));
#47487=CARTESIAN_POINT('Ctrl Pts',(1.89589172903793,1.,3.27407108933139));
#47488=CARTESIAN_POINT('Ctrl Pts',(1.89255393500965,1.,3.26677653888676));
#47489=CARTESIAN_POINT('Ctrl Pts',(1.88934996203698,1.,3.25999885193947));
#47490=CARTESIAN_POINT('Ctrl Pts',(1.88646802523466,1.,3.25408686339463));
#47491=CARTESIAN_POINT('Ctrl Pts',(1.88407708646357,1.,3.24935200511918));
#47492=CARTESIAN_POINT('Ctrl Pts',(1.88242596600454,1.,3.2462565441079));
#47493=CARTESIAN_POINT('Ctrl Pts',(1.88156537699203,1.,3.24480754676064));
#47494=CARTESIAN_POINT('Ctrl Pts',(1.88117508446775,1.,3.24428080353022));
#47495=CARTESIAN_POINT('Ctrl Pts',(1.8810229239812,1.,3.24415531671284));
#47496=CARTESIAN_POINT('Ctrl Pts',(1.88097764062697,1.,3.24413672884812));
#47497=CARTESIAN_POINT('',(1.97421938526992,0.,3.70708211654725));
#47498=CARTESIAN_POINT('Ctrl Pts',(1.519044091397,-1.,3.42855728381368));
#47499=CARTESIAN_POINT('Ctrl Pts',(1.519044091397,1.,3.42855728381368));
#47500=CARTESIAN_POINT('Ctrl Pts',(1.51896318668366,-1.,3.42852521763778));
#47501=CARTESIAN_POINT('Ctrl Pts',(1.51896318668366,1.,3.42852521763778));
#47502=CARTESIAN_POINT('Ctrl Pts',(1.51888450659652,-1.,3.42860527149177));
#47503=CARTESIAN_POINT('Ctrl Pts',(1.51888450659652,1.,3.42860527149177));
#47504=CARTESIAN_POINT('Ctrl Pts',(1.51901585839109,-1.,3.42915787669893));
#47505=CARTESIAN_POINT('Ctrl Pts',(1.51901585839109,1.,3.42915787669893));
#47506=CARTESIAN_POINT('Ctrl Pts',(1.51969006980999,-1.,3.43076036253837));
#47507=CARTESIAN_POINT('Ctrl Pts',(1.51969006980999,1.,3.43076036253837));
#47508=CARTESIAN_POINT('Ctrl Pts',(1.52134826724292,-1.,3.43417156977893));
#47509=CARTESIAN_POINT('Ctrl Pts',(1.52134826724292,1.,3.43417156977893));
#47510=CARTESIAN_POINT('Ctrl Pts',(1.5237734895035,-1.,3.4388889597401));
#47511=CARTESIAN_POINT('Ctrl Pts',(1.5237734895035,1.,3.4388889597401));
#47512=CARTESIAN_POINT('Ctrl Pts',(1.52686242875556,-1.,3.44469547526647));
#47513=CARTESIAN_POINT('Ctrl Pts',(1.52686242875556,1.,3.44469547526647));
#47514=CARTESIAN_POINT('Ctrl Pts',(1.53046244461635,-1.,3.45127136828305));
#47515=CARTESIAN_POINT('Ctrl Pts',(1.53046244461635,1.,3.45127136828305));
#47516=CARTESIAN_POINT('Ctrl Pts',(1.53440195378792,-1.,3.45825932955032));
#47517=CARTESIAN_POINT('Ctrl Pts',(1.53440195378792,1.,3.45825932955032));
#47518=CARTESIAN_POINT('Ctrl Pts',(1.53851507915502,-1.,3.46531752207153));
#47519=CARTESIAN_POINT('Ctrl Pts',(1.53851507915502,1.,3.46531752207153));
#47520=CARTESIAN_POINT('Ctrl Pts',(1.54266605398187,-1.,3.47217189224653));
#47521=CARTESIAN_POINT('Ctrl Pts',(1.54266605398187,1.,3.47217189224653));
#47522=CARTESIAN_POINT('Ctrl Pts',(1.54678009290276,-1.,3.47868272898751));
#47523=CARTESIAN_POINT('Ctrl Pts',(1.54678009290276,1.,3.47868272898751));
#47524=CARTESIAN_POINT('Ctrl Pts',(1.55084702970452,-1.,3.48485155928567));
#47525=CARTESIAN_POINT('Ctrl Pts',(1.55084702970452,1.,3.48485155928567));
#47526=CARTESIAN_POINT('Ctrl Pts',(1.55489595901116,-1.,3.4907646087742));
#47527=CARTESIAN_POINT('Ctrl Pts',(1.55489595901116,1.,3.4907646087742));
#47528=CARTESIAN_POINT('Ctrl Pts',(1.55897703097874,-1.,3.49655185179655));
#47529=CARTESIAN_POINT('Ctrl Pts',(1.55897703097874,1.,3.49655185179655));
#47530=CARTESIAN_POINT('Ctrl Pts',(1.56314187758675,-1.,3.50234321621578));
#47531=CARTESIAN_POINT('Ctrl Pts',(1.56314187758675,1.,3.50234321621578));
#47532=CARTESIAN_POINT('Ctrl Pts',(1.56742097575012,-1.,3.50821771695363));
#47533=CARTESIAN_POINT('Ctrl Pts',(1.56742097575012,1.,3.50821771695363));
#47534=CARTESIAN_POINT('Ctrl Pts',(1.57181569799743,-1.,3.51418598431665));
#47535=CARTESIAN_POINT('Ctrl Pts',(1.57181569799743,1.,3.51418598431665));
#47536=CARTESIAN_POINT('Ctrl Pts',(1.57631049988158,-1.,3.52021847865912));
#47537=CARTESIAN_POINT('Ctrl Pts',(1.57631049988158,1.,3.52021847865912));
#47538=CARTESIAN_POINT('Ctrl Pts',(1.58088027227848,-1.,3.52626275334881));
#47539=CARTESIAN_POINT('Ctrl Pts',(1.58088027227848,1.,3.52626275334881));
#47540=CARTESIAN_POINT('Ctrl Pts',(1.58549906268088,-1.,3.5322637814708));
#47541=CARTESIAN_POINT('Ctrl Pts',(1.58549906268088,1.,3.5322637814708));
#47542=CARTESIAN_POINT('Ctrl Pts',(1.59014958368739,-1.,3.53818616861077));
#47543=CARTESIAN_POINT('Ctrl Pts',(1.59014958368739,1.,3.53818616861077));
#47544=CARTESIAN_POINT('Ctrl Pts',(1.59482766949766,-1.,3.54402458182337));
#47545=CARTESIAN_POINT('Ctrl Pts',(1.59482766949766,1.,3.54402458182337));
#47546=CARTESIAN_POINT('Ctrl Pts',(1.59953698113457,-1.,3.54979148634454));
#47547=CARTESIAN_POINT('Ctrl Pts',(1.59953698113457,1.,3.54979148634454));
#47548=CARTESIAN_POINT('Ctrl Pts',(1.60428584699853,-1.,3.55550985096129));
#47549=CARTESIAN_POINT('Ctrl Pts',(1.60428584699853,1.,3.55550985096129));
#47550=CARTESIAN_POINT('Ctrl Pts',(1.60908344685457,-1.,3.5612043248298));
#47551=CARTESIAN_POINT('Ctrl Pts',(1.60908344685457,1.,3.5612043248298));
#47552=CARTESIAN_POINT('Ctrl Pts',(1.61393581747514,-1.,3.56689200468387));
#47553=CARTESIAN_POINT('Ctrl Pts',(1.61393581747514,1.,3.56689200468387));
#47554=CARTESIAN_POINT('Ctrl Pts',(1.61884340915404,-1.,3.57257679609806));
#47555=CARTESIAN_POINT('Ctrl Pts',(1.61884340915404,1.,3.57257679609806));
#47556=CARTESIAN_POINT('Ctrl Pts',(1.62380329464844,-1.,3.5782545595439));
#47557=CARTESIAN_POINT('Ctrl Pts',(1.62380329464844,1.,3.5782545595439));
#47558=CARTESIAN_POINT('Ctrl Pts',(1.62881051550745,-1.,3.58391625774343));
#47559=CARTESIAN_POINT('Ctrl Pts',(1.62881051550745,1.,3.58391625774343));
#47560=CARTESIAN_POINT('Ctrl Pts',(1.6338597145126,-1.,3.58955176627879));
#47561=CARTESIAN_POINT('Ctrl Pts',(1.6338597145126,1.,3.58955176627879));
#47562=CARTESIAN_POINT('Ctrl Pts',(1.63894676675352,-1.,3.59515368334893));
#47563=CARTESIAN_POINT('Ctrl Pts',(1.63894676675352,1.,3.59515368334893));
#47564=CARTESIAN_POINT('Ctrl Pts',(1.64407004385582,-1.,3.60072028513845));
#47565=CARTESIAN_POINT('Ctrl Pts',(1.64407004385582,1.,3.60072028513845));
#47566=CARTESIAN_POINT('Ctrl Pts',(1.64922952425832,-1.,3.60625346556992));
#47567=CARTESIAN_POINT('Ctrl Pts',(1.64922952425832,1.,3.60625346556992));
#47568=CARTESIAN_POINT('Ctrl Pts',(1.65442619244325,-1.,3.61175734965127));
#47569=CARTESIAN_POINT('Ctrl Pts',(1.65442619244325,1.,3.61175734965127));
#47570=CARTESIAN_POINT('Ctrl Pts',(1.65966133399186,-1.,3.61723666482456));
#47571=CARTESIAN_POINT('Ctrl Pts',(1.65966133399186,1.,3.61723666482456));
#47572=CARTESIAN_POINT('Ctrl Pts',(1.66493585923855,-1.,3.62269517989109));
#47573=CARTESIAN_POINT('Ctrl Pts',(1.66493585923855,1.,3.62269517989109));
#47574=CARTESIAN_POINT('Ctrl Pts',(1.67024966008044,-1.,3.62813422105271));
#47575=CARTESIAN_POINT('Ctrl Pts',(1.67024966008044,1.,3.62813422105271));
#47576=CARTESIAN_POINT('Ctrl Pts',(1.67560193613156,-1.,3.63355343201232));
#47577=CARTESIAN_POINT('Ctrl Pts',(1.67560193613156,1.,3.63355343201232));
#47578=CARTESIAN_POINT('Ctrl Pts',(1.68099146651586,-1.,3.63895140887462));
#47579=CARTESIAN_POINT('Ctrl Pts',(1.68099146651586,1.,3.63895140887462));
#47580=CARTESIAN_POINT('Ctrl Pts',(1.68641690471457,-1.,3.64432638915203));
#47581=CARTESIAN_POINT('Ctrl Pts',(1.68641690471457,1.,3.64432638915203));
#47582=CARTESIAN_POINT('Ctrl Pts',(1.69187705481689,-1.,3.64967689827371));
#47583=CARTESIAN_POINT('Ctrl Pts',(1.69187705481689,1.,3.64967689827371));
#47584=CARTESIAN_POINT('Ctrl Pts',(1.69737117722534,-1.,3.65500246526749));
#47585=CARTESIAN_POINT('Ctrl Pts',(1.69737117722534,1.,3.65500246526749));
#47586=CARTESIAN_POINT('Ctrl Pts',(1.70289888566873,-1.,3.66030338774847));
#47587=CARTESIAN_POINT('Ctrl Pts',(1.70289888566873,1.,3.66030338774847));
#47588=CARTESIAN_POINT('Ctrl Pts',(1.70846001610956,-1.,3.66558043198876));
#47589=CARTESIAN_POINT('Ctrl Pts',(1.70846001610956,1.,3.66558043198876));
#47590=CARTESIAN_POINT('Ctrl Pts',(1.71405450210383,-1.,3.67083454901611));
#47591=CARTESIAN_POINT('Ctrl Pts',(1.71405450210383,1.,3.67083454901611));
#47592=CARTESIAN_POINT('Ctrl Pts',(1.71968225581808,-1.,3.67606660374709));
#47593=CARTESIAN_POINT('Ctrl Pts',(1.71968225581808,1.,3.67606660374709));
#47594=CARTESIAN_POINT('Ctrl Pts',(1.72534302437056,-1.,3.68127704936579));
#47595=CARTESIAN_POINT('Ctrl Pts',(1.72534302437056,1.,3.68127704936579));
#47596=CARTESIAN_POINT('Ctrl Pts',(1.73103640956717,-1.,3.68646597019332));
#47597=CARTESIAN_POINT('Ctrl Pts',(1.73103640956717,1.,3.68646597019332));
#47598=CARTESIAN_POINT('Ctrl Pts',(1.73676193254557,-1.,3.69163322648036));
#47599=CARTESIAN_POINT('Ctrl Pts',(1.73676193254557,1.,3.69163322648036));
#47600=CARTESIAN_POINT('Ctrl Pts',(1.74251908492617,-1.,3.69677856910517));
#47601=CARTESIAN_POINT('Ctrl Pts',(1.74251908492617,1.,3.69677856910517));
#47602=CARTESIAN_POINT('Ctrl Pts',(1.74830738046057,-1.,3.7019017567335));
#47603=CARTESIAN_POINT('Ctrl Pts',(1.74830738046057,1.,3.7019017567335));
#47604=CARTESIAN_POINT('Ctrl Pts',(1.75412641804042,-1.,3.70700269736659));
#47605=CARTESIAN_POINT('Ctrl Pts',(1.75412641804042,1.,3.70700269736659));
#47606=CARTESIAN_POINT('Ctrl Pts',(1.75997588498865,-1.,3.71208146346136));
#47607=CARTESIAN_POINT('Ctrl Pts',(1.75997588498865,1.,3.71208146346136));
#47608=CARTESIAN_POINT('Ctrl Pts',(1.76585552124394,-1.,3.71713822377359));
#47609=CARTESIAN_POINT('Ctrl Pts',(1.76585552124394,1.,3.71713822377359));
#47610=CARTESIAN_POINT('Ctrl Pts',(1.77176509401761,-1.,3.72217319911254));
#47611=CARTESIAN_POINT('Ctrl Pts',(1.77176509401761,1.,3.72217319911254));
#47612=CARTESIAN_POINT('Ctrl Pts',(1.77770437039658,-1.,3.72718661205609));
#47613=CARTESIAN_POINT('Ctrl Pts',(1.77770437039658,1.,3.72718661205609));
#47614=CARTESIAN_POINT('Ctrl Pts',(1.78367308442901,-1.,3.7321786309547));
#47615=CARTESIAN_POINT('Ctrl Pts',(1.78367308442901,1.,3.7321786309547));
#47616=CARTESIAN_POINT('Ctrl Pts',(1.78967092823491,-1.,3.73714934730681));
#47617=CARTESIAN_POINT('Ctrl Pts',(1.78967092823491,1.,3.73714934730681));
#47618=CARTESIAN_POINT('Ctrl Pts',(1.79569757859422,-1.,3.74209880352445));
#47619=CARTESIAN_POINT('Ctrl Pts',(1.79569757859422,1.,3.74209880352445));
#47620=CARTESIAN_POINT('Ctrl Pts',(1.8017527148577,-1.,3.74702700875467));
#47621=CARTESIAN_POINT('Ctrl Pts',(1.8017527148577,1.,3.74702700875467));
#47622=CARTESIAN_POINT('Ctrl Pts',(1.80783603939617,-1.,3.75193395887977));
#47623=CARTESIAN_POINT('Ctrl Pts',(1.80783603939617,1.,3.75193395887977));
#47624=CARTESIAN_POINT('Ctrl Pts',(1.8139472983358,-1.,3.75681965683071));
#47625=CARTESIAN_POINT('Ctrl Pts',(1.8139472983358,1.,3.75681965683071));
#47626=CARTESIAN_POINT('Ctrl Pts',(1.82008629694091,-1.,3.76168412707948));
#47627=CARTESIAN_POINT('Ctrl Pts',(1.82008629694091,1.,3.76168412707948));
#47628=CARTESIAN_POINT('Ctrl Pts',(1.82625289220915,-1.,3.76652740353775));
#47629=CARTESIAN_POINT('Ctrl Pts',(1.82625289220915,1.,3.76652740353775));
#47630=CARTESIAN_POINT('Ctrl Pts',(1.83120816955645,-1.,3.77038509817999));
#47631=CARTESIAN_POINT('Ctrl Pts',(1.83120816955645,1.,3.77038509817999));
#47632=CARTESIAN_POINT('Ctrl Pts',(1.83493697934534,-1.,3.77326886064398));
#47633=CARTESIAN_POINT('Ctrl Pts',(1.83493697934534,1.,3.77326886064398));
#47634=CARTESIAN_POINT('Ctrl Pts',(1.83742834010626,-1.,3.77518714457833));
#47635=CARTESIAN_POINT('Ctrl Pts',(1.83742834010626,1.,3.77518714457833));
#47636=CARTESIAN_POINT('Ctrl Pts',(1.8386753923786,-1.,3.77614523045147));
#47637=CARTESIAN_POINT('Ctrl Pts',(1.8386753923786,1.,3.77614523045147));
#47638=CARTESIAN_POINT('',(1.5189508286633,1.,3.42859860294306));
#47639=CARTESIAN_POINT('Ctrl Pts',(1.5189508286633,-1.,3.42859860294306));
#47640=CARTESIAN_POINT('Ctrl Pts',(1.5189508286633,-0.666666666666667,3.42859860294306));
#47641=CARTESIAN_POINT('Ctrl Pts',(1.5189508286633,-0.333333333333333,3.42859860294306));
#47642=CARTESIAN_POINT('Ctrl Pts',(1.5189508286633,0.333333333333333,3.42859860294306));
#47643=CARTESIAN_POINT('Ctrl Pts',(1.5189508286633,0.666666666666667,3.42859860294306));
#47644=CARTESIAN_POINT('Ctrl Pts',(1.5189508286633,1.,3.42859860294306));
#47645=CARTESIAN_POINT('',(1.8386753923786,1.,3.77614523045147));
#47646=CARTESIAN_POINT('',(1.8386753923786,0.,3.77614523045147));
#47647=CARTESIAN_POINT('Ctrl Pts',(1.5189508286633,1.,3.42859860294306));
#47648=CARTESIAN_POINT('Ctrl Pts',(1.51893924967331,1.,3.42864616361875));
#47649=CARTESIAN_POINT('Ctrl Pts',(1.5189513329503,1.,3.42884302333841));
#47650=CARTESIAN_POINT('Ctrl Pts',(1.51914806898491,1.,3.42946838852587));
#47651=CARTESIAN_POINT('Ctrl Pts',(1.5198144909338,1.,3.43101631893414));
#47652=CARTESIAN_POINT('Ctrl Pts',(1.52134826724292,1.,3.43417156977893));
#47653=CARTESIAN_POINT('Ctrl Pts',(1.5237734895035,1.,3.4388889597401));
#47654=CARTESIAN_POINT('Ctrl Pts',(1.52686242875556,1.,3.44469547526647));
#47655=CARTESIAN_POINT('Ctrl Pts',(1.53046244461635,1.,3.45127136828305));
#47656=CARTESIAN_POINT('Ctrl Pts',(1.53440195378792,1.,3.45825932955032));
#47657=CARTESIAN_POINT('Ctrl Pts',(1.53851507915502,1.,3.46531752207153));
#47658=CARTESIAN_POINT('Ctrl Pts',(1.54266605398187,1.,3.47217189224653));
#47659=CARTESIAN_POINT('Ctrl Pts',(1.54678009290276,1.,3.47868272898751));
#47660=CARTESIAN_POINT('Ctrl Pts',(1.55084702970452,1.,3.48485155928567));
#47661=CARTESIAN_POINT('Ctrl Pts',(1.55489595901116,1.,3.4907646087742));
#47662=CARTESIAN_POINT('Ctrl Pts',(1.55897703097874,1.,3.49655185179655));
#47663=CARTESIAN_POINT('Ctrl Pts',(1.56314187758675,1.,3.50234321621578));
#47664=CARTESIAN_POINT('Ctrl Pts',(1.56742097575012,1.,3.50821771695363));
#47665=CARTESIAN_POINT('Ctrl Pts',(1.57181569799743,1.,3.51418598431665));
#47666=CARTESIAN_POINT('Ctrl Pts',(1.57631049988158,1.,3.52021847865912));
#47667=CARTESIAN_POINT('Ctrl Pts',(1.58088027227848,1.,3.52626275334881));
#47668=CARTESIAN_POINT('Ctrl Pts',(1.58549906268088,1.,3.5322637814708));
#47669=CARTESIAN_POINT('Ctrl Pts',(1.59014958368739,1.,3.53818616861077));
#47670=CARTESIAN_POINT('Ctrl Pts',(1.59482766949766,1.,3.54402458182337));
#47671=CARTESIAN_POINT('Ctrl Pts',(1.59953698113457,1.,3.54979148634454));
#47672=CARTESIAN_POINT('Ctrl Pts',(1.60428584699853,1.,3.55550985096129));
#47673=CARTESIAN_POINT('Ctrl Pts',(1.60908344685457,1.,3.5612043248298));
#47674=CARTESIAN_POINT('Ctrl Pts',(1.61393581747514,1.,3.56689200468387));
#47675=CARTESIAN_POINT('Ctrl Pts',(1.61884340915404,1.,3.57257679609806));
#47676=CARTESIAN_POINT('Ctrl Pts',(1.62380329464844,1.,3.5782545595439));
#47677=CARTESIAN_POINT('Ctrl Pts',(1.62881051550745,1.,3.58391625774343));
#47678=CARTESIAN_POINT('Ctrl Pts',(1.6338597145126,1.,3.58955176627879));
#47679=CARTESIAN_POINT('Ctrl Pts',(1.63894676675352,1.,3.59515368334893));
#47680=CARTESIAN_POINT('Ctrl Pts',(1.64407004385582,1.,3.60072028513845));
#47681=CARTESIAN_POINT('Ctrl Pts',(1.64922952425832,1.,3.60625346556992));
#47682=CARTESIAN_POINT('Ctrl Pts',(1.65442619244325,1.,3.61175734965127));
#47683=CARTESIAN_POINT('Ctrl Pts',(1.65966133399186,1.,3.61723666482456));
#47684=CARTESIAN_POINT('Ctrl Pts',(1.66493585923855,1.,3.62269517989109));
#47685=CARTESIAN_POINT('Ctrl Pts',(1.67024966008044,1.,3.62813422105271));
#47686=CARTESIAN_POINT('Ctrl Pts',(1.67560193613156,1.,3.63355343201232));
#47687=CARTESIAN_POINT('Ctrl Pts',(1.68099146651586,1.,3.63895140887462));
#47688=CARTESIAN_POINT('Ctrl Pts',(1.68641690471457,1.,3.64432638915203));
#47689=CARTESIAN_POINT('Ctrl Pts',(1.69187705481689,1.,3.64967689827371));
#47690=CARTESIAN_POINT('Ctrl Pts',(1.69737117722534,1.,3.65500246526749));
#47691=CARTESIAN_POINT('Ctrl Pts',(1.70289888566873,1.,3.66030338774847));
#47692=CARTESIAN_POINT('Ctrl Pts',(1.70846001610956,1.,3.66558043198876));
#47693=CARTESIAN_POINT('Ctrl Pts',(1.71405450210383,1.,3.67083454901611));
#47694=CARTESIAN_POINT('Ctrl Pts',(1.71968225581808,1.,3.67606660374709));
#47695=CARTESIAN_POINT('Ctrl Pts',(1.72534302437056,1.,3.68127704936579));
#47696=CARTESIAN_POINT('Ctrl Pts',(1.73103640956717,1.,3.68646597019332));
#47697=CARTESIAN_POINT('Ctrl Pts',(1.73676193254557,1.,3.69163322648036));
#47698=CARTESIAN_POINT('Ctrl Pts',(1.74251908492617,1.,3.69677856910517));
#47699=CARTESIAN_POINT('Ctrl Pts',(1.74830738046057,1.,3.7019017567335));
#47700=CARTESIAN_POINT('Ctrl Pts',(1.75412641804042,1.,3.70700269736659));
#47701=CARTESIAN_POINT('Ctrl Pts',(1.75997588498865,1.,3.71208146346136));
#47702=CARTESIAN_POINT('Ctrl Pts',(1.76585552124394,1.,3.71713822377359));
#47703=CARTESIAN_POINT('Ctrl Pts',(1.77176509401761,1.,3.72217319911254));
#47704=CARTESIAN_POINT('Ctrl Pts',(1.77770437039658,1.,3.72718661205609));
#47705=CARTESIAN_POINT('Ctrl Pts',(1.78367308442901,1.,3.7321786309547));
#47706=CARTESIAN_POINT('Ctrl Pts',(1.78967092823491,1.,3.73714934730681));
#47707=CARTESIAN_POINT('Ctrl Pts',(1.79569757859422,1.,3.74209880352445));
#47708=CARTESIAN_POINT('Ctrl Pts',(1.8017527148577,1.,3.74702700875467));
#47709=CARTESIAN_POINT('Ctrl Pts',(1.80783603939617,1.,3.75193395887977));
#47710=CARTESIAN_POINT('Ctrl Pts',(1.8139472983358,1.,3.75681965683071));
#47711=CARTESIAN_POINT('Ctrl Pts',(1.82008629694091,1.,3.76168412707948));
#47712=CARTESIAN_POINT('Ctrl Pts',(1.82625289220915,1.,3.76652740353775));
#47713=CARTESIAN_POINT('Ctrl Pts',(1.83120816955645,1.,3.77038509817999));
#47714=CARTESIAN_POINT('Ctrl Pts',(1.83493697934534,1.,3.77326886064398));
#47715=CARTESIAN_POINT('Ctrl Pts',(1.83742834010626,1.,3.77518714457833));
#47716=CARTESIAN_POINT('Ctrl Pts',(1.8386753923786,1.,3.77614523045147));
#47717=CARTESIAN_POINT('Origin',(1.8386753923786,0.,3.77614523045147));
#47718=CARTESIAN_POINT('',(1.97421938526992,1.,3.70708211654725));
#47719=CARTESIAN_POINT('Origin',(0.,0.,0.));
#47720=CARTESIAN_POINT('',(1.35032489087269,1.,3.49844575334386));
#47721=CARTESIAN_POINT('Origin',(0.,1.,0.));
#47722=CARTESIAN_POINT('Ctrl Pts',(1.35032489087269,1.,3.49844575334386));
#47723=CARTESIAN_POINT('Ctrl Pts',(1.35032489087269,0.666666666666667,3.49844575334386));
#47724=CARTESIAN_POINT('Ctrl Pts',(1.35032489087269,0.333333333333333,3.49844575334386));
#47725=CARTESIAN_POINT('Ctrl Pts',(1.35032489087269,-0.333333333333333,
3.49844575334386));
#47726=CARTESIAN_POINT('Ctrl Pts',(1.35032489087269,-0.666666666666667,
3.49844575334386));
#47727=CARTESIAN_POINT('Ctrl Pts',(1.35032489087269,-1.,3.49844575334386));
#47728=CARTESIAN_POINT('Ctrl Pts',(1.36999806084572,-1.,3.97027773754922));
#47729=CARTESIAN_POINT('Ctrl Pts',(1.36999806084572,1.,3.97027773754922));
#47730=CARTESIAN_POINT('Ctrl Pts',(1.37020239094758,-1.,3.9687184694173));
#47731=CARTESIAN_POINT('Ctrl Pts',(1.37020239094758,1.,3.9687184694173));
#47732=CARTESIAN_POINT('Ctrl Pts',(1.37060761746027,-1.,3.96560037975788));
#47733=CARTESIAN_POINT('Ctrl Pts',(1.37060761746027,1.,3.96560037975788));
#47734=CARTESIAN_POINT('Ctrl Pts',(1.37120515615663,-1.,3.96092458508407));
#47735=CARTESIAN_POINT('Ctrl Pts',(1.37120515615663,1.,3.96092458508407));
#47736=CARTESIAN_POINT('Ctrl Pts',(1.37198126433139,-1.,3.95469287283105));
#47737=CARTESIAN_POINT('Ctrl Pts',(1.37198126433139,1.,3.95469287283105));
#47738=CARTESIAN_POINT('Ctrl Pts',(1.37291699203423,-1.,3.94690771786926));
#47739=CARTESIAN_POINT('Ctrl Pts',(1.37291699203423,1.,3.94690771786926));
#47740=CARTESIAN_POINT('Ctrl Pts',(1.37381821967499,-1.,3.93912709041791));
#47741=CARTESIAN_POINT('Ctrl Pts',(1.37381821967499,1.,3.93912709041791));
#47742=CARTESIAN_POINT('Ctrl Pts',(1.37468482215784,-1.,3.93135106761941));
#47743=CARTESIAN_POINT('Ctrl Pts',(1.37468482215784,1.,3.93135106761941));
#47744=CARTESIAN_POINT('Ctrl Pts',(1.37551664448057,-1.,3.92357976987132));
#47745=CARTESIAN_POINT('Ctrl Pts',(1.37551664448057,1.,3.92357976987132));
#47746=CARTESIAN_POINT('Ctrl Pts',(1.37631350505516,-1.,3.91581337461825));
#47747=CARTESIAN_POINT('Ctrl Pts',(1.37631350505516,1.,3.91581337461825));
#47748=CARTESIAN_POINT('Ctrl Pts',(1.3770751963376,-1.,3.90805209522729));
#47749=CARTESIAN_POINT('Ctrl Pts',(1.3770751963376,1.,3.90805209522729));
#47750=CARTESIAN_POINT('Ctrl Pts',(1.3778014851263,-1.,3.90029615196255));
#47751=CARTESIAN_POINT('Ctrl Pts',(1.3778014851263,1.,3.90029615196255));
#47752=CARTESIAN_POINT('Ctrl Pts',(1.37849211287981,-1.,3.89254574338385));
#47753=CARTESIAN_POINT('Ctrl Pts',(1.37849211287981,1.,3.89254574338385));
#47754=CARTESIAN_POINT('Ctrl Pts',(1.37914679719446,-1.,3.88480102249461));
#47755=CARTESIAN_POINT('Ctrl Pts',(1.37914679719446,1.,3.88480102249461));
#47756=CARTESIAN_POINT('Ctrl Pts',(1.37976523097187,-1.,3.87706205830865));
#47757=CARTESIAN_POINT('Ctrl Pts',(1.37976523097187,1.,3.87706205830865));
#47758=CARTESIAN_POINT('Ctrl Pts',(1.38034709213129,-1.,3.86932885813403));
#47759=CARTESIAN_POINT('Ctrl Pts',(1.38034709213129,1.,3.86932885813403));
#47760=CARTESIAN_POINT('Ctrl Pts',(1.38089205993067,-1.,3.86160143044187));
#47761=CARTESIAN_POINT('Ctrl Pts',(1.38089205993067,1.,3.86160143044187));
#47762=CARTESIAN_POINT('Ctrl Pts',(1.38139983115075,-1.,3.85387983979557));
#47763=CARTESIAN_POINT('Ctrl Pts',(1.38139983115075,1.,3.85387983979557));
#47764=CARTESIAN_POINT('Ctrl Pts',(1.38187013346089,-1.,3.84616425605705));
#47765=CARTESIAN_POINT('Ctrl Pts',(1.38187013346089,1.,3.84616425605705));
#47766=CARTESIAN_POINT('Ctrl Pts',(1.38230274828774,-1.,3.83845502790609));
#47767=CARTESIAN_POINT('Ctrl Pts',(1.38230274828774,1.,3.83845502790609));
#47768=CARTESIAN_POINT('Ctrl Pts',(1.38269750245086,-1.,3.83075266982138));
#47769=CARTESIAN_POINT('Ctrl Pts',(1.38269750245086,1.,3.83075266982138));
#47770=CARTESIAN_POINT('Ctrl Pts',(1.38305421262724,-1.,3.82305771743715));
#47771=CARTESIAN_POINT('Ctrl Pts',(1.38305421262724,1.,3.82305771743715));
#47772=CARTESIAN_POINT('Ctrl Pts',(1.38337263902766,-1.,3.81537060817765));
#47773=CARTESIAN_POINT('Ctrl Pts',(1.38337263902766,1.,3.81537060817765));
#47774=CARTESIAN_POINT('Ctrl Pts',(1.38365244046226,-1.,3.80769156398429));
#47775=CARTESIAN_POINT('Ctrl Pts',(1.38365244046226,1.,3.80769156398429));
#47776=CARTESIAN_POINT('Ctrl Pts',(1.38389311766701,-1.,3.80002044322169));
#47777=CARTESIAN_POINT('Ctrl Pts',(1.38389311766701,1.,3.80002044322169));
#47778=CARTESIAN_POINT('Ctrl Pts',(1.38409399694588,-1.,3.79235669640907));
#47779=CARTESIAN_POINT('Ctrl Pts',(1.38409399694588,1.,3.79235669640907));
#47780=CARTESIAN_POINT('Ctrl Pts',(1.38425435883773,-1.,3.78469969805134));
#47781=CARTESIAN_POINT('Ctrl Pts',(1.38425435883773,1.,3.78469969805134));
#47782=CARTESIAN_POINT('Ctrl Pts',(1.38437354551435,-1.,3.77704902230441));
#47783=CARTESIAN_POINT('Ctrl Pts',(1.38437354551435,1.,3.77704902230441));
#47784=CARTESIAN_POINT('Ctrl Pts',(1.38445107339517,-1.,3.76940473185775));
#47785=CARTESIAN_POINT('Ctrl Pts',(1.38445107339517,1.,3.76940473185775));
#47786=CARTESIAN_POINT('Ctrl Pts',(1.38448675253343,-1.,3.76176768271347));
#47787=CARTESIAN_POINT('Ctrl Pts',(1.38448675253343,1.,3.76176768271347));
#47788=CARTESIAN_POINT('Ctrl Pts',(1.38448077997155,-1.,3.75413976318727));
#47789=CARTESIAN_POINT('Ctrl Pts',(1.38448077997155,1.,3.75413976318727));
#47790=CARTESIAN_POINT('Ctrl Pts',(1.38443344984389,-1.,3.7465231716786));
#47791=CARTESIAN_POINT('Ctrl Pts',(1.38443344984389,1.,3.7465231716786));
#47792=CARTESIAN_POINT('Ctrl Pts',(1.38434489156456,-1.,3.73891976418099));
#47793=CARTESIAN_POINT('Ctrl Pts',(1.38434489156456,1.,3.73891976418099));
#47794=CARTESIAN_POINT('Ctrl Pts',(1.38421479111531,-1.,3.73133035859283));
#47795=CARTESIAN_POINT('Ctrl Pts',(1.38421479111531,1.,3.73133035859283));
#47796=CARTESIAN_POINT('Ctrl Pts',(1.3840421342895,-1.,3.72375409358805));
#47797=CARTESIAN_POINT('Ctrl Pts',(1.3840421342895,1.,3.72375409358805));
#47798=CARTESIAN_POINT('Ctrl Pts',(1.38382489984585,-1.,3.7161876605181));
#47799=CARTESIAN_POINT('Ctrl Pts',(1.38382489984585,1.,3.7161876605181));
#47800=CARTESIAN_POINT('Ctrl Pts',(1.38356065402122,-1.,3.70862680753343));
#47801=CARTESIAN_POINT('Ctrl Pts',(1.38356065402122,1.,3.70862680753343));
#47802=CARTESIAN_POINT('Ctrl Pts',(1.38324717612862,-1.,3.70106792167894));
#47803=CARTESIAN_POINT('Ctrl Pts',(1.38324717612862,1.,3.70106792167894));
#47804=CARTESIAN_POINT('Ctrl Pts',(1.38288311171649,-1.,3.69350967899523));
#47805=CARTESIAN_POINT('Ctrl Pts',(1.38288311171649,1.,3.69350967899523));
#47806=CARTESIAN_POINT('Ctrl Pts',(1.38246852827185,-1.,3.68595444983844));
#47807=CARTESIAN_POINT('Ctrl Pts',(1.38246852827185,1.,3.68595444983844));
#47808=CARTESIAN_POINT('Ctrl Pts',(1.38200574290626,-1.,3.6784103848243));
#47809=CARTESIAN_POINT('Ctrl Pts',(1.38200574290626,1.,3.6784103848243));
#47810=CARTESIAN_POINT('Ctrl Pts',(1.38149812653876,-1.,3.67088843112282));
#47811=CARTESIAN_POINT('Ctrl Pts',(1.38149812653876,1.,3.67088843112282));
#47812=CARTESIAN_POINT('Ctrl Pts',(1.38094856333558,-1.,3.66339848520874));
#47813=CARTESIAN_POINT('Ctrl Pts',(1.38094856333558,1.,3.66339848520874));
#47814=CARTESIAN_POINT('Ctrl Pts',(1.38035791051215,-1.,3.65594554404396));
#47815=CARTESIAN_POINT('Ctrl Pts',(1.38035791051215,1.,3.65594554404396));
#47816=CARTESIAN_POINT('Ctrl Pts',(1.37972372481598,-1.,3.64852652756444));
#47817=CARTESIAN_POINT('Ctrl Pts',(1.37972372481598,1.,3.64852652756444));
#47818=CARTESIAN_POINT('Ctrl Pts',(1.37903818567347,-1.,3.64112507791112));
#47819=CARTESIAN_POINT('Ctrl Pts',(1.37903818567347,1.,3.64112507791112));
#47820=CARTESIAN_POINT('Ctrl Pts',(1.37829035457324,-1.,3.63371727442448));
#47821=CARTESIAN_POINT('Ctrl Pts',(1.37829035457324,1.,3.63371727442448));
#47822=CARTESIAN_POINT('Ctrl Pts',(1.37746987919868,-1.,3.62628098665112));
#47823=CARTESIAN_POINT('Ctrl Pts',(1.37746987919868,1.,3.62628098665112));
#47824=CARTESIAN_POINT('Ctrl Pts',(1.37657053403102,-1.,3.61880481160408));
#47825=CARTESIAN_POINT('Ctrl Pts',(1.37657053403102,1.,3.61880481160408));
#47826=CARTESIAN_POINT('Ctrl Pts',(1.37559314436641,-1.,3.61129546591082));
#47827=CARTESIAN_POINT('Ctrl Pts',(1.37559314436641,1.,3.61129546591082));
#47828=CARTESIAN_POINT('Ctrl Pts',(1.37455051379642,-1.,3.60379020124038));
#47829=CARTESIAN_POINT('Ctrl Pts',(1.37455051379642,1.,3.60379020124038));
#47830=CARTESIAN_POINT('Ctrl Pts',(1.37346320103184,-1.,3.59634627869117));
#47831=CARTESIAN_POINT('Ctrl Pts',(1.37346320103184,1.,3.59634627869117));
#47832=CARTESIAN_POINT('Ctrl Pts',(1.37235053661,-1.,3.5890185384643));
#47833=CARTESIAN_POINT('Ctrl Pts',(1.37235053661,1.,3.5890185384643));
#47834=CARTESIAN_POINT('Ctrl Pts',(1.37122241663073,-1.,3.58183885982745));
#47835=CARTESIAN_POINT('Ctrl Pts',(1.37122241663073,1.,3.58183885982745));
#47836=CARTESIAN_POINT('Ctrl Pts',(1.37007229485646,-1.,3.57479875549453));
#47837=CARTESIAN_POINT('Ctrl Pts',(1.37007229485646,1.,3.57479875549453));
#47838=CARTESIAN_POINT('Ctrl Pts',(1.36886584973349,-1.,3.56782080304554));
#47839=CARTESIAN_POINT('Ctrl Pts',(1.36886584973349,1.,3.56782080304554));
#47840=CARTESIAN_POINT('Ctrl Pts',(1.36754771771174,-1.,3.56077662028492));
#47841=CARTESIAN_POINT('Ctrl Pts',(1.36754771771174,1.,3.56077662028492));
#47842=CARTESIAN_POINT('Ctrl Pts',(1.36606145456711,-1.,3.55353883995793));
#47843=CARTESIAN_POINT('Ctrl Pts',(1.36606145456711,1.,3.55353883995793));
#47844=CARTESIAN_POINT('Ctrl Pts',(1.36436666257567,-1.,3.54602591832893));
#47845=CARTESIAN_POINT('Ctrl Pts',(1.36436666257567,1.,3.54602591832893));
#47846=CARTESIAN_POINT('Ctrl Pts',(1.36245507339334,-1.,3.53824396425032));
#47847=CARTESIAN_POINT('Ctrl Pts',(1.36245507339334,1.,3.53824396425032));
#47848=CARTESIAN_POINT('Ctrl Pts',(1.36037259643827,-1.,3.53034464961849));
#47849=CARTESIAN_POINT('Ctrl Pts',(1.36037259643827,1.,3.53034464961849));
#47850=CARTESIAN_POINT('Ctrl Pts',(1.35821701528975,-1.,3.52261776117121));
#47851=CARTESIAN_POINT('Ctrl Pts',(1.35821701528975,1.,3.52261776117121));
#47852=CARTESIAN_POINT('Ctrl Pts',(1.35611275237288,-1.,3.51542230699919));
#47853=CARTESIAN_POINT('Ctrl Pts',(1.35611275237288,1.,3.51542230699919));
#47854=CARTESIAN_POINT('Ctrl Pts',(1.35419113576022,-1.,3.50913227060177));
#47855=CARTESIAN_POINT('Ctrl Pts',(1.35419113576022,1.,3.50913227060177));
#47856=CARTESIAN_POINT('Ctrl Pts',(1.3525703284343,-1.,3.50408168106113));
#47857=CARTESIAN_POINT('Ctrl Pts',(1.3525703284343,1.,3.50408168106113));
#47858=CARTESIAN_POINT('Ctrl Pts',(1.35133076331065,-1.,3.50049707063673));
#47859=CARTESIAN_POINT('Ctrl Pts',(1.35133076331065,1.,3.50049707063673));
#47860=CARTESIAN_POINT('Ctrl Pts',(1.35067437417289,-1.,3.49888720256612));
#47861=CARTESIAN_POINT('Ctrl Pts',(1.35067437417289,1.,3.49888720256612));
#47862=CARTESIAN_POINT('Ctrl Pts',(1.35037650302887,-1.,3.49840357193384));
#47863=CARTESIAN_POINT('Ctrl Pts',(1.35037650302887,1.,3.49840357193384));
#47864=CARTESIAN_POINT('Ctrl Pts',(1.35026426118351,-1.,3.49840260053616));
#47865=CARTESIAN_POINT('Ctrl Pts',(1.35026426118351,1.,3.49840260053616));
#47866=CARTESIAN_POINT('Ctrl Pts',(1.35022972712301,-1.,3.49848248301936));
#47867=CARTESIAN_POINT('Ctrl Pts',(1.35022972712301,1.,3.49848248301936));
#47868=CARTESIAN_POINT('',(1.36999806084572,1.,3.97027773754922));
#47869=CARTESIAN_POINT('Ctrl Pts',(1.36999806084572,1.,3.97027773754922));
#47870=CARTESIAN_POINT('Ctrl Pts',(1.37020239094758,1.,3.9687184694173));
#47871=CARTESIAN_POINT('Ctrl Pts',(1.37060761746027,1.,3.96560037975788));
#47872=CARTESIAN_POINT('Ctrl Pts',(1.37120515615663,1.,3.96092458508407));
#47873=CARTESIAN_POINT('Ctrl Pts',(1.37198126433139,1.,3.95469287283105));
#47874=CARTESIAN_POINT('Ctrl Pts',(1.37291699203423,1.,3.94690771786926));
#47875=CARTESIAN_POINT('Ctrl Pts',(1.37381821967499,1.,3.93912709041791));
#47876=CARTESIAN_POINT('Ctrl Pts',(1.37468482215784,1.,3.93135106761941));
#47877=CARTESIAN_POINT('Ctrl Pts',(1.37551664448057,1.,3.92357976987132));
#47878=CARTESIAN_POINT('Ctrl Pts',(1.37631350505516,1.,3.91581337461825));
#47879=CARTESIAN_POINT('Ctrl Pts',(1.3770751963376,1.,3.90805209522729));
#47880=CARTESIAN_POINT('Ctrl Pts',(1.3778014851263,1.,3.90029615196255));
#47881=CARTESIAN_POINT('Ctrl Pts',(1.37849211287981,1.,3.89254574338385));
#47882=CARTESIAN_POINT('Ctrl Pts',(1.37914679719446,1.,3.88480102249461));
#47883=CARTESIAN_POINT('Ctrl Pts',(1.37976523097187,1.,3.87706205830865));
#47884=CARTESIAN_POINT('Ctrl Pts',(1.38034709213129,1.,3.86932885813403));
#47885=CARTESIAN_POINT('Ctrl Pts',(1.38089205993067,1.,3.86160143044187));
#47886=CARTESIAN_POINT('Ctrl Pts',(1.38139983115075,1.,3.85387983979557));
#47887=CARTESIAN_POINT('Ctrl Pts',(1.38187013346089,1.,3.84616425605705));
#47888=CARTESIAN_POINT('Ctrl Pts',(1.38230274828774,1.,3.83845502790609));
#47889=CARTESIAN_POINT('Ctrl Pts',(1.38269750245086,1.,3.83075266982138));
#47890=CARTESIAN_POINT('Ctrl Pts',(1.38305421262724,1.,3.82305771743715));
#47891=CARTESIAN_POINT('Ctrl Pts',(1.38337263902766,1.,3.81537060817765));
#47892=CARTESIAN_POINT('Ctrl Pts',(1.38365244046226,1.,3.80769156398429));
#47893=CARTESIAN_POINT('Ctrl Pts',(1.38389311766701,1.,3.80002044322169));
#47894=CARTESIAN_POINT('Ctrl Pts',(1.38409399694588,1.,3.79235669640907));
#47895=CARTESIAN_POINT('Ctrl Pts',(1.38425435883773,1.,3.78469969805134));
#47896=CARTESIAN_POINT('Ctrl Pts',(1.38437354551435,1.,3.77704902230441));
#47897=CARTESIAN_POINT('Ctrl Pts',(1.38445107339517,1.,3.76940473185775));
#47898=CARTESIAN_POINT('Ctrl Pts',(1.38448675253343,1.,3.76176768271347));
#47899=CARTESIAN_POINT('Ctrl Pts',(1.38448077997155,1.,3.75413976318727));
#47900=CARTESIAN_POINT('Ctrl Pts',(1.38443344984389,1.,3.7465231716786));
#47901=CARTESIAN_POINT('Ctrl Pts',(1.38434489156456,1.,3.73891976418099));
#47902=CARTESIAN_POINT('Ctrl Pts',(1.38421479111531,1.,3.73133035859283));
#47903=CARTESIAN_POINT('Ctrl Pts',(1.3840421342895,1.,3.72375409358805));
#47904=CARTESIAN_POINT('Ctrl Pts',(1.38382489984585,1.,3.7161876605181));
#47905=CARTESIAN_POINT('Ctrl Pts',(1.38356065402122,1.,3.70862680753343));
#47906=CARTESIAN_POINT('Ctrl Pts',(1.38324717612862,1.,3.70106792167894));
#47907=CARTESIAN_POINT('Ctrl Pts',(1.38288311171649,1.,3.69350967899523));
#47908=CARTESIAN_POINT('Ctrl Pts',(1.38246852827185,1.,3.68595444983844));
#47909=CARTESIAN_POINT('Ctrl Pts',(1.38200574290626,1.,3.6784103848243));
#47910=CARTESIAN_POINT('Ctrl Pts',(1.38149812653876,1.,3.67088843112282));
#47911=CARTESIAN_POINT('Ctrl Pts',(1.38094856333558,1.,3.66339848520874));
#47912=CARTESIAN_POINT('Ctrl Pts',(1.38035791051215,1.,3.65594554404396));
#47913=CARTESIAN_POINT('Ctrl Pts',(1.37972372481598,1.,3.64852652756444));
#47914=CARTESIAN_POINT('Ctrl Pts',(1.37903818567347,1.,3.64112507791112));
#47915=CARTESIAN_POINT('Ctrl Pts',(1.37829035457324,1.,3.63371727442448));
#47916=CARTESIAN_POINT('Ctrl Pts',(1.37746987919868,1.,3.62628098665112));
#47917=CARTESIAN_POINT('Ctrl Pts',(1.37657053403102,1.,3.61880481160408));
#47918=CARTESIAN_POINT('Ctrl Pts',(1.37559314436641,1.,3.61129546591082));
#47919=CARTESIAN_POINT('Ctrl Pts',(1.37455051379642,1.,3.60379020124038));
#47920=CARTESIAN_POINT('Ctrl Pts',(1.37346320103184,1.,3.59634627869117));
#47921=CARTESIAN_POINT('Ctrl Pts',(1.37235053661,1.,3.5890185384643));
#47922=CARTESIAN_POINT('Ctrl Pts',(1.37122241663073,1.,3.58183885982745));
#47923=CARTESIAN_POINT('Ctrl Pts',(1.37007229485646,1.,3.57479875549453));
#47924=CARTESIAN_POINT('Ctrl Pts',(1.36886584973349,1.,3.56782080304554));
#47925=CARTESIAN_POINT('Ctrl Pts',(1.36754771771174,1.,3.56077662028492));
#47926=CARTESIAN_POINT('Ctrl Pts',(1.36606145456711,1.,3.55353883995793));
#47927=CARTESIAN_POINT('Ctrl Pts',(1.36436666257567,1.,3.54602591832893));
#47928=CARTESIAN_POINT('Ctrl Pts',(1.36245507339334,1.,3.53824396425032));
#47929=CARTESIAN_POINT('Ctrl Pts',(1.36037259643827,1.,3.53034464961849));
#47930=CARTESIAN_POINT('Ctrl Pts',(1.35821701528975,1.,3.52261776117121));
#47931=CARTESIAN_POINT('Ctrl Pts',(1.35611275237288,1.,3.51542230699919));
#47932=CARTESIAN_POINT('Ctrl Pts',(1.35419113576022,1.,3.50913227060177));
#47933=CARTESIAN_POINT('Ctrl Pts',(1.3525703284343,1.,3.50408168106113));
#47934=CARTESIAN_POINT('Ctrl Pts',(1.35142377279535,1.,3.5007660381658));
#47935=CARTESIAN_POINT('Ctrl Pts',(1.35080045218652,1.,3.49920025459856));
#47936=CARTESIAN_POINT('Ctrl Pts',(1.35049736560633,1.,3.49861894124915));
#47937=CARTESIAN_POINT('Ctrl Pts',(1.35036670893102,1.,3.49847119623841));
#47938=CARTESIAN_POINT('Ctrl Pts',(1.35032489087269,1.,3.49844575334386));
#47939=CARTESIAN_POINT('',(1.36999806084572,0.,3.97027773754922));
#47940=CARTESIAN_POINT('Ctrl Pts',(0.96399761336957,-1.,3.62397690409552));
#47941=CARTESIAN_POINT('Ctrl Pts',(0.96399761336957,1.,3.62397690409552));
#47942=CARTESIAN_POINT('Ctrl Pts',(0.963922720982576,-1.,3.62393257642191));
#47943=CARTESIAN_POINT('Ctrl Pts',(0.963922720982576,1.,3.62393257642191));
#47944=CARTESIAN_POINT('Ctrl Pts',(0.963832486396055,-1.,3.62399933640277));
#47945=CARTESIAN_POINT('Ctrl Pts',(0.963832486396055,1.,3.62399933640277));
#47946=CARTESIAN_POINT('Ctrl Pts',(0.963875774532102,-1.,3.62456568607055));
#47947=CARTESIAN_POINT('Ctrl Pts',(0.963875774532102,1.,3.62456568607055));
#47948=CARTESIAN_POINT('Ctrl Pts',(0.964291001274618,-1.,3.62625391255277));
#47949=CARTESIAN_POINT('Ctrl Pts',(0.964291001274618,1.,3.62625391255277));
#47950=CARTESIAN_POINT('Ctrl Pts',(0.965395153165715,-1.,3.62988252139998));
#47951=CARTESIAN_POINT('Ctrl Pts',(0.965395153165715,1.,3.62988252139998));
#47952=CARTESIAN_POINT('Ctrl Pts',(0.967052554540877,-1.,3.6349212208096));
#47953=CARTESIAN_POINT('Ctrl Pts',(0.967052554540877,1.,3.6349212208096));
#47954=CARTESIAN_POINT('Ctrl Pts',(0.969195124674828,-1.,3.64113946505393));
#47955=CARTESIAN_POINT('Ctrl Pts',(0.969195124674828,1.,3.64113946505393));
#47956=CARTESIAN_POINT('Ctrl Pts',(0.971722122060277,-1.,3.64819756447072));
#47957=CARTESIAN_POINT('Ctrl Pts',(0.971722122060277,1.,3.64819756447072));
#47958=CARTESIAN_POINT('Ctrl Pts',(0.974519971354138,-1.,3.6557157673487));
#47959=CARTESIAN_POINT('Ctrl Pts',(0.974519971354138,1.,3.6557157673487));
#47960=CARTESIAN_POINT('Ctrl Pts',(0.977478312751416,-1.,3.66333049637403));
#47961=CARTESIAN_POINT('Ctrl Pts',(0.977478312751416,1.,3.66333049637403));
#47962=CARTESIAN_POINT('Ctrl Pts',(0.980505922458494,-1.,3.67074983340444));
#47963=CARTESIAN_POINT('Ctrl Pts',(0.980505922458494,1.,3.67074983340444));
#47964=CARTESIAN_POINT('Ctrl Pts',(0.983550791470864,-1.,3.67782408841876));
#47965=CARTESIAN_POINT('Ctrl Pts',(0.983550791470864,1.,3.67782408841876));
#47966=CARTESIAN_POINT('Ctrl Pts',(0.986602639864285,-1.,3.6845531792623));
#47967=CARTESIAN_POINT('Ctrl Pts',(0.986602639864285,1.,3.6845531792623));
#47968=CARTESIAN_POINT('Ctrl Pts',(0.989676715398858,-1.,3.69102682138955));
#47969=CARTESIAN_POINT('Ctrl Pts',(0.989676715398858,1.,3.69102682138955));
#47970=CARTESIAN_POINT('Ctrl Pts',(0.992802218332103,-1.,3.69738123415696));
#47971=CARTESIAN_POINT('Ctrl Pts',(0.992802218332103,1.,3.69738123415696));
#47972=CARTESIAN_POINT('Ctrl Pts',(0.996009819772431,-1.,3.70375282282107));
#47973=CARTESIAN_POINT('Ctrl Pts',(0.996009819772431,1.,3.70375282282107));
#47974=CARTESIAN_POINT('Ctrl Pts',(0.999317260756344,-1.,3.7102243971387));
#47975=CARTESIAN_POINT('Ctrl Pts',(0.999317260756344,1.,3.7102243971387));
#47976=CARTESIAN_POINT('Ctrl Pts',(1.00272423396802,-1.,3.71680667125047));
#47977=CARTESIAN_POINT('Ctrl Pts',(1.00272423396802,1.,3.71680667125047));
#47978=CARTESIAN_POINT('Ctrl Pts',(1.00622000735696,-1.,3.72346803750544));
#47979=CARTESIAN_POINT('Ctrl Pts',(1.00622000735696,1.,3.72346803750544));
#47980=CARTESIAN_POINT('Ctrl Pts',(1.00978798539491,-1.,3.73015276704407));
#47981=CARTESIAN_POINT('Ctrl Pts',(1.00978798539491,1.,3.73015276704407));
#47982=CARTESIAN_POINT('Ctrl Pts',(1.01341114319906,-1.,3.73680245055747));
#47983=CARTESIAN_POINT('Ctrl Pts',(1.01341114319906,1.,3.73680245055747));
#47984=CARTESIAN_POINT('Ctrl Pts',(1.01707794311088,-1.,3.74337942504993));
#47985=CARTESIAN_POINT('Ctrl Pts',(1.01707794311088,1.,3.74337942504993));
#47986=CARTESIAN_POINT('Ctrl Pts',(1.02078510487439,-1.,3.74987777155873));
#47987=CARTESIAN_POINT('Ctrl Pts',(1.02078510487439,1.,3.74987777155873));
#47988=CARTESIAN_POINT('Ctrl Pts',(1.02453429444668,-1.,3.75631037456224));
#47989=CARTESIAN_POINT('Ctrl Pts',(1.02453429444668,1.,3.75631037456224));
#47990=CARTESIAN_POINT('Ctrl Pts',(1.02833014458184,-1.,3.76270122291245));
#47991=CARTESIAN_POINT('Ctrl Pts',(1.02833014458184,1.,3.76270122291245));
#47992=CARTESIAN_POINT('Ctrl Pts',(1.03217786604919,-1.,3.76907609832516));
#47993=CARTESIAN_POINT('Ctrl Pts',(1.03217786604919,1.,3.76907609832516));
#47994=CARTESIAN_POINT('Ctrl Pts',(1.03608074678008,-1.,3.77545283140427));
#47995=CARTESIAN_POINT('Ctrl Pts',(1.03608074678008,1.,3.77545283140427));
#47996=CARTESIAN_POINT('Ctrl Pts',(1.04003862055798,-1.,3.7818353500817));
#47997=CARTESIAN_POINT('Ctrl Pts',(1.04003862055798,1.,3.7818353500817));
#47998=CARTESIAN_POINT('Ctrl Pts',(1.04404924374422,-1.,3.78821910787179));
#47999=CARTESIAN_POINT('Ctrl Pts',(1.04404924374422,1.,3.78821910787179));
#48000=CARTESIAN_POINT('Ctrl Pts',(1.04810913267639,-1.,3.79459440308786));
#48001=CARTESIAN_POINT('Ctrl Pts',(1.04810913267639,1.,3.79459440308786));
#48002=CARTESIAN_POINT('Ctrl Pts',(1.05221457990016,-1.,3.80095039790681));
#48003=CARTESIAN_POINT('Ctrl Pts',(1.05221457990016,1.,3.80095039790681));
#48004=CARTESIAN_POINT('Ctrl Pts',(1.05636266918644,-1.,3.80727913637791));
#48005=CARTESIAN_POINT('Ctrl Pts',(1.05636266918644,1.,3.80727913637791));
#48006=CARTESIAN_POINT('Ctrl Pts',(1.06055206187299,-1.,3.8135786611749));
#48007=CARTESIAN_POINT('Ctrl Pts',(1.06055206187299,1.,3.8135786611749));
#48008=CARTESIAN_POINT('Ctrl Pts',(1.0647824403893,-1.,3.81985083953012));
#48009=CARTESIAN_POINT('Ctrl Pts',(1.0647824403893,1.,3.81985083953012));
#48010=CARTESIAN_POINT('Ctrl Pts',(1.06905413180359,-1.,3.82609989967276));
#48011=CARTESIAN_POINT('Ctrl Pts',(1.06905413180359,1.,3.82609989967276));
#48012=CARTESIAN_POINT('Ctrl Pts',(1.07336766633459,-1.,3.83233071195144));
#48013=CARTESIAN_POINT('Ctrl Pts',(1.07336766633459,1.,3.83233071195144));
#48014=CARTESIAN_POINT('Ctrl Pts',(1.07772335353858,-1.,3.83854714117491));
#48015=CARTESIAN_POINT('Ctrl Pts',(1.07772335353858,1.,3.83854714117491));
#48016=CARTESIAN_POINT('Ctrl Pts',(1.08212087917991,-1.,3.8447504803063));
#48017=CARTESIAN_POINT('Ctrl Pts',(1.08212087917991,1.,3.8447504803063));
#48018=CARTESIAN_POINT('Ctrl Pts',(1.08655950846384,-1.,3.85094025222713));
#48019=CARTESIAN_POINT('Ctrl Pts',(1.08655950846384,1.,3.85094025222713));
#48020=CARTESIAN_POINT('Ctrl Pts',(1.09103825516294,-1.,3.85711487933931));
#48021=CARTESIAN_POINT('Ctrl Pts',(1.09103825516294,1.,3.85711487933931));
#48022=CARTESIAN_POINT('Ctrl Pts',(1.09555606505013,-1.,3.86327241021247));
#48023=CARTESIAN_POINT('Ctrl Pts',(1.09555606505013,1.,3.86327241021247));
#48024=CARTESIAN_POINT('Ctrl Pts',(1.10011198761195,-1.,3.86941120134849));
#48025=CARTESIAN_POINT('Ctrl Pts',(1.10011198761195,1.,3.86941120134849));
#48026=CARTESIAN_POINT('Ctrl Pts',(1.10470536603287,-1.,3.87553067187514));
#48027=CARTESIAN_POINT('Ctrl Pts',(1.10470536603287,1.,3.87553067187514));
#48028=CARTESIAN_POINT('Ctrl Pts',(1.10933577224008,-1.,3.88163105531724));
#48029=CARTESIAN_POINT('Ctrl Pts',(1.10933577224008,1.,3.88163105531724));
#48030=CARTESIAN_POINT('Ctrl Pts',(1.11400292434429,-1.,3.88771308285171));
#48031=CARTESIAN_POINT('Ctrl Pts',(1.11400292434429,1.,3.88771308285171));
#48032=CARTESIAN_POINT('Ctrl Pts',(1.11870660794603,-1.,3.89377768340344));
#48033=CARTESIAN_POINT('Ctrl Pts',(1.11870660794603,1.,3.89377768340344));
#48034=CARTESIAN_POINT('Ctrl Pts',(1.12344660099043,-1.,3.89982569750025));
#48035=CARTESIAN_POINT('Ctrl Pts',(1.12344660099043,1.,3.89982569750025));
#48036=CARTESIAN_POINT('Ctrl Pts',(1.12822258281553,-1.,3.90585753318737));
#48037=CARTESIAN_POINT('Ctrl Pts',(1.12822258281553,1.,3.90585753318737));
#48038=CARTESIAN_POINT('Ctrl Pts',(1.13303414693896,-1.,3.91187321145649));
#48039=CARTESIAN_POINT('Ctrl Pts',(1.13303414693896,1.,3.91187321145649));
#48040=CARTESIAN_POINT('Ctrl Pts',(1.13788084225554,-1.,3.91787251936827));
#48041=CARTESIAN_POINT('Ctrl Pts',(1.13788084225554,1.,3.91787251936827));
#48042=CARTESIAN_POINT('Ctrl Pts',(1.14276220561593,-1.,3.92385513133997));
#48043=CARTESIAN_POINT('Ctrl Pts',(1.14276220561593,1.,3.92385513133997));
#48044=CARTESIAN_POINT('Ctrl Pts',(1.14767779451123,-1.,3.92982073294257));
#48045=CARTESIAN_POINT('Ctrl Pts',(1.14767779451123,1.,3.92982073294257));
#48046=CARTESIAN_POINT('Ctrl Pts',(1.1526272271632,-1.,3.9357691705628));
#48047=CARTESIAN_POINT('Ctrl Pts',(1.1526272271632,1.,3.9357691705628));
#48048=CARTESIAN_POINT('Ctrl Pts',(1.15761018340956,-1.,3.94170046685203));
#48049=CARTESIAN_POINT('Ctrl Pts',(1.15761018340956,1.,3.94170046685203));
#48050=CARTESIAN_POINT('Ctrl Pts',(1.16262637999157,-1.,3.94761474780583));
#48051=CARTESIAN_POINT('Ctrl Pts',(1.16262637999157,1.,3.94761474780583));
#48052=CARTESIAN_POINT('Ctrl Pts',(1.16767555244438,-1.,3.95351219509876));
#48053=CARTESIAN_POINT('Ctrl Pts',(1.16767555244438,1.,3.95351219509876));
#48054=CARTESIAN_POINT('Ctrl Pts',(1.17275743590361,-1.,3.95939299213276));
#48055=CARTESIAN_POINT('Ctrl Pts',(1.17275743590361,1.,3.95939299213276));
#48056=CARTESIAN_POINT('Ctrl Pts',(1.17787174135592,-1.,3.96525726358159));
#48057=CARTESIAN_POINT('Ctrl Pts',(1.17787174135592,1.,3.96525726358159));
#48058=CARTESIAN_POINT('Ctrl Pts',(1.18301815039831,-1.,3.97110505165415));
#48059=CARTESIAN_POINT('Ctrl Pts',(1.18301815039831,1.,3.97110505165415));
#48060=CARTESIAN_POINT('Ctrl Pts',(1.18819633715539,-1.,3.97693634767754));
#48061=CARTESIAN_POINT('Ctrl Pts',(1.18819633715539,1.,3.97693634767754));
#48062=CARTESIAN_POINT('Ctrl Pts',(1.19340598349475,-1.,3.98275111052561));
#48063=CARTESIAN_POINT('Ctrl Pts',(1.19340598349475,1.,3.98275111052561));
#48064=CARTESIAN_POINT('Ctrl Pts',(1.19864679609566,-1.,3.98854928957189));
#48065=CARTESIAN_POINT('Ctrl Pts',(1.19864679609566,1.,3.98854928957189));
#48066=CARTESIAN_POINT('Ctrl Pts',(1.20391852375138,-1.,3.99433084799666));
#48067=CARTESIAN_POINT('Ctrl Pts',(1.20391852375138,1.,3.99433084799666));
#48068=CARTESIAN_POINT('Ctrl Pts',(1.20922097029551,-1.,4.00009577950721));
#48069=CARTESIAN_POINT('Ctrl Pts',(1.20922097029551,1.,4.00009577950721));
#48070=CARTESIAN_POINT('Ctrl Pts',(1.21455398918133,-1.,4.00584409522722));
#48071=CARTESIAN_POINT('Ctrl Pts',(1.21455398918133,1.,4.00584409522722));
#48072=CARTESIAN_POINT('Ctrl Pts',(1.21884478244403,-1.,4.01042947140789));
#48073=CARTESIAN_POINT('Ctrl Pts',(1.21884478244403,1.,4.01042947140789));
#48074=CARTESIAN_POINT('Ctrl Pts',(1.22207656455845,-1.,4.01386104433519));
#48075=CARTESIAN_POINT('Ctrl Pts',(1.22207656455845,1.,4.01386104433519));
#48076=CARTESIAN_POINT('Ctrl Pts',(1.22423716681317,-1.,4.01614544569895));
#48077=CARTESIAN_POINT('Ctrl Pts',(1.22423716681317,1.,4.01614544569895));
#48078=CARTESIAN_POINT('Ctrl Pts',(1.22531898815164,-1.,4.01728681790024));
#48079=CARTESIAN_POINT('Ctrl Pts',(1.22531898815164,1.,4.01728681790024));
#48080=CARTESIAN_POINT('',(0.963899035118985,1.,3.62400312501199));
#48081=CARTESIAN_POINT('Ctrl Pts',(0.963899035118985,-1.,3.62400312501199));
#48082=CARTESIAN_POINT('Ctrl Pts',(0.963899035118985,-0.666666666666667,
3.62400312501199));
#48083=CARTESIAN_POINT('Ctrl Pts',(0.963899035118985,-0.333333333333333,
3.62400312501199));
#48084=CARTESIAN_POINT('Ctrl Pts',(0.963899035118985,0.333333333333333,
3.62400312501199));
#48085=CARTESIAN_POINT('Ctrl Pts',(0.963899035118985,0.666666666666667,
3.62400312501199));
#48086=CARTESIAN_POINT('Ctrl Pts',(0.963899035118985,1.,3.62400312501199));
#48087=CARTESIAN_POINT('',(1.22531898815164,1.,4.01728681790024));
#48088=CARTESIAN_POINT('',(1.22531898815164,0.,4.01728681790024));
#48089=CARTESIAN_POINT('Ctrl Pts',(0.963899035118985,1.,3.62400312501199));
#48090=CARTESIAN_POINT('Ctrl Pts',(0.963880158556712,1.,3.62404828878375));
#48091=CARTESIAN_POINT('Ctrl Pts',(0.963861297423578,1.,3.62424461507455));
#48092=CARTESIAN_POINT('Ctrl Pts',(0.963957782642589,1.,3.62489305727516));
#48093=CARTESIAN_POINT('Ctrl Pts',(0.964373850166081,1.,3.62652618145252));
#48094=CARTESIAN_POINT('Ctrl Pts',(0.965395153165715,1.,3.62988252139998));
#48095=CARTESIAN_POINT('Ctrl Pts',(0.967052554540877,1.,3.6349212208096));
#48096=CARTESIAN_POINT('Ctrl Pts',(0.969195124674828,1.,3.64113946505393));
#48097=CARTESIAN_POINT('Ctrl Pts',(0.971722122060277,1.,3.64819756447072));
#48098=CARTESIAN_POINT('Ctrl Pts',(0.974519971354138,1.,3.6557157673487));
#48099=CARTESIAN_POINT('Ctrl Pts',(0.977478312751416,1.,3.66333049637403));
#48100=CARTESIAN_POINT('Ctrl Pts',(0.980505922458494,1.,3.67074983340444));
#48101=CARTESIAN_POINT('Ctrl Pts',(0.983550791470864,1.,3.67782408841876));
#48102=CARTESIAN_POINT('Ctrl Pts',(0.986602639864285,1.,3.6845531792623));
#48103=CARTESIAN_POINT('Ctrl Pts',(0.989676715398858,1.,3.69102682138955));
#48104=CARTESIAN_POINT('Ctrl Pts',(0.992802218332103,1.,3.69738123415696));
#48105=CARTESIAN_POINT('Ctrl Pts',(0.996009819772431,1.,3.70375282282107));
#48106=CARTESIAN_POINT('Ctrl Pts',(0.999317260756344,1.,3.7102243971387));
#48107=CARTESIAN_POINT('Ctrl Pts',(1.00272423396802,1.,3.71680667125047));
#48108=CARTESIAN_POINT('Ctrl Pts',(1.00622000735696,1.,3.72346803750544));
#48109=CARTESIAN_POINT('Ctrl Pts',(1.00978798539491,1.,3.73015276704407));
#48110=CARTESIAN_POINT('Ctrl Pts',(1.01341114319906,1.,3.73680245055747));
#48111=CARTESIAN_POINT('Ctrl Pts',(1.01707794311088,1.,3.74337942504993));
#48112=CARTESIAN_POINT('Ctrl Pts',(1.02078510487439,1.,3.74987777155873));
#48113=CARTESIAN_POINT('Ctrl Pts',(1.02453429444668,1.,3.75631037456224));
#48114=CARTESIAN_POINT('Ctrl Pts',(1.02833014458184,1.,3.76270122291245));
#48115=CARTESIAN_POINT('Ctrl Pts',(1.03217786604919,1.,3.76907609832516));
#48116=CARTESIAN_POINT('Ctrl Pts',(1.03608074678008,1.,3.77545283140427));
#48117=CARTESIAN_POINT('Ctrl Pts',(1.04003862055798,1.,3.7818353500817));
#48118=CARTESIAN_POINT('Ctrl Pts',(1.04404924374422,1.,3.78821910787179));
#48119=CARTESIAN_POINT('Ctrl Pts',(1.04810913267639,1.,3.79459440308786));
#48120=CARTESIAN_POINT('Ctrl Pts',(1.05221457990016,1.,3.80095039790681));
#48121=CARTESIAN_POINT('Ctrl Pts',(1.05636266918644,1.,3.80727913637791));
#48122=CARTESIAN_POINT('Ctrl Pts',(1.06055206187299,1.,3.8135786611749));
#48123=CARTESIAN_POINT('Ctrl Pts',(1.0647824403893,1.,3.81985083953012));
#48124=CARTESIAN_POINT('Ctrl Pts',(1.06905413180359,1.,3.82609989967276));
#48125=CARTESIAN_POINT('Ctrl Pts',(1.07336766633459,1.,3.83233071195144));
#48126=CARTESIAN_POINT('Ctrl Pts',(1.07772335353858,1.,3.83854714117491));
#48127=CARTESIAN_POINT('Ctrl Pts',(1.08212087917991,1.,3.8447504803063));
#48128=CARTESIAN_POINT('Ctrl Pts',(1.08655950846384,1.,3.85094025222713));
#48129=CARTESIAN_POINT('Ctrl Pts',(1.09103825516294,1.,3.85711487933931));
#48130=CARTESIAN_POINT('Ctrl Pts',(1.09555606505013,1.,3.86327241021247));
#48131=CARTESIAN_POINT('Ctrl Pts',(1.10011198761195,1.,3.86941120134849));
#48132=CARTESIAN_POINT('Ctrl Pts',(1.10470536603287,1.,3.87553067187514));
#48133=CARTESIAN_POINT('Ctrl Pts',(1.10933577224008,1.,3.88163105531724));
#48134=CARTESIAN_POINT('Ctrl Pts',(1.11400292434429,1.,3.88771308285171));
#48135=CARTESIAN_POINT('Ctrl Pts',(1.11870660794603,1.,3.89377768340344));
#48136=CARTESIAN_POINT('Ctrl Pts',(1.12344660099043,1.,3.89982569750025));
#48137=CARTESIAN_POINT('Ctrl Pts',(1.12822258281553,1.,3.90585753318737));
#48138=CARTESIAN_POINT('Ctrl Pts',(1.13303414693896,1.,3.91187321145649));
#48139=CARTESIAN_POINT('Ctrl Pts',(1.13788084225554,1.,3.91787251936827));
#48140=CARTESIAN_POINT('Ctrl Pts',(1.14276220561593,1.,3.92385513133997));
#48141=CARTESIAN_POINT('Ctrl Pts',(1.14767779451123,1.,3.92982073294257));
#48142=CARTESIAN_POINT('Ctrl Pts',(1.1526272271632,1.,3.9357691705628));
#48143=CARTESIAN_POINT('Ctrl Pts',(1.15761018340956,1.,3.94170046685203));
#48144=CARTESIAN_POINT('Ctrl Pts',(1.16262637999157,1.,3.94761474780583));
#48145=CARTESIAN_POINT('Ctrl Pts',(1.16767555244438,1.,3.95351219509876));
#48146=CARTESIAN_POINT('Ctrl Pts',(1.17275743590361,1.,3.95939299213276));
#48147=CARTESIAN_POINT('Ctrl Pts',(1.17787174135592,1.,3.96525726358159));
#48148=CARTESIAN_POINT('Ctrl Pts',(1.18301815039831,1.,3.97110505165415));
#48149=CARTESIAN_POINT('Ctrl Pts',(1.18819633715539,1.,3.97693634767754));
#48150=CARTESIAN_POINT('Ctrl Pts',(1.19340598349475,1.,3.98275111052561));
#48151=CARTESIAN_POINT('Ctrl Pts',(1.19864679609566,1.,3.98854928957189));
#48152=CARTESIAN_POINT('Ctrl Pts',(1.20391852375138,1.,3.99433084799666));
#48153=CARTESIAN_POINT('Ctrl Pts',(1.20922097029551,1.,4.00009577950721));
#48154=CARTESIAN_POINT('Ctrl Pts',(1.21455398918133,1.,4.00584409522722));
#48155=CARTESIAN_POINT('Ctrl Pts',(1.21884478244403,1.,4.01042947140789));
#48156=CARTESIAN_POINT('Ctrl Pts',(1.22207656455845,1.,4.01386104433519));
#48157=CARTESIAN_POINT('Ctrl Pts',(1.22423716681317,1.,4.01614544569895));
#48158=CARTESIAN_POINT('Ctrl Pts',(1.22531898815164,1.,4.01728681790024));
#48159=CARTESIAN_POINT('Origin',(1.22531898815164,0.,4.01728681790024));
#48160=CARTESIAN_POINT('',(1.36999806084572,1.,3.97027773754922));
#48161=CARTESIAN_POINT('Origin',(0.,0.,0.));
#48162=CARTESIAN_POINT('',(0.786422660833742,1.,3.66661143271648));
#48163=CARTESIAN_POINT('Origin',(0.,1.,0.));
#48164=CARTESIAN_POINT('Ctrl Pts',(0.786422660833742,1.,3.66661143271648));
#48165=CARTESIAN_POINT('Ctrl Pts',(0.786422660833742,0.666666666666667,
3.66661143271648));
#48166=CARTESIAN_POINT('Ctrl Pts',(0.786422660833742,0.333333333333333,
3.66661143271648));
#48167=CARTESIAN_POINT('Ctrl Pts',(0.786422660833742,-0.333333333333333,
3.66661143271648));
#48168=CARTESIAN_POINT('Ctrl Pts',(0.786422660833742,-0.666666666666667,
3.66661143271648));
#48169=CARTESIAN_POINT('Ctrl Pts',(0.786422660833742,-1.,3.66661143271648));
#48170=CARTESIAN_POINT('Ctrl Pts',(0.732042837400619,-1.,4.13571194405636));
#48171=CARTESIAN_POINT('Ctrl Pts',(0.732042837400619,1.,4.13571194405636));
#48172=CARTESIAN_POINT('Ctrl Pts',(0.732488575135925,-1.,4.13420383737278));
#48173=CARTESIAN_POINT('Ctrl Pts',(0.732488575135925,1.,4.13420383737278));
#48174=CARTESIAN_POINT('Ctrl Pts',(0.733376589325634,-1.,4.13118752796397));
#48175=CARTESIAN_POINT('Ctrl Pts',(0.733376589325634,1.,4.13118752796397));
#48176=CARTESIAN_POINT('Ctrl Pts',(0.734698226767512,-1.,4.12666277572794));
#48177=CARTESIAN_POINT('Ctrl Pts',(0.734698226767512,1.,4.12666277572794));
#48178=CARTESIAN_POINT('Ctrl Pts',(0.736439634335347,-1.,4.12062919626082));
#48179=CARTESIAN_POINT('Ctrl Pts',(0.736439634335347,1.,4.12062919626082));
#48180=CARTESIAN_POINT('Ctrl Pts',(0.738581708229118,-1.,4.11308626953795));
#48181=CARTESIAN_POINT('Ctrl Pts',(0.738581708229118,1.,4.11308626953795));
#48182=CARTESIAN_POINT('Ctrl Pts',(0.740688998555151,-1.,4.1055424175856));
#48183=CARTESIAN_POINT('Ctrl Pts',(0.740688998555151,1.,4.1055424175856));
#48184=CARTESIAN_POINT('Ctrl Pts',(0.742761369690017,-1.,4.09799769702712));
#48185=CARTESIAN_POINT('Ctrl Pts',(0.742761369690017,1.,4.09799769702712));
#48186=CARTESIAN_POINT('Ctrl Pts',(0.744798649705513,-1.,4.09045220253011));
#48187=CARTESIAN_POINT('Ctrl Pts',(0.744798649705513,1.,4.09045220253011));
#48188=CARTESIAN_POINT('Ctrl Pts',(0.746800631490821,-1.,4.08290608094789));
#48189=CARTESIAN_POINT('Ctrl Pts',(0.746800631490821,1.,4.08290608094789));
#48190=CARTESIAN_POINT('Ctrl Pts',(0.748767076679176,-1.,4.07535951055363));
#48191=CARTESIAN_POINT('Ctrl Pts',(0.748767076679176,1.,4.07535951055363));
#48192=CARTESIAN_POINT('Ctrl Pts',(0.750697720483175,-1.,4.06781267241886));
#48193=CARTESIAN_POINT('Ctrl Pts',(0.750697720483175,1.,4.06781267241886));
#48194=CARTESIAN_POINT('Ctrl Pts',(0.752592276482868,-1.,4.06026572221399));
#48195=CARTESIAN_POINT('Ctrl Pts',(0.752592276482868,1.,4.06026572221399));
#48196=CARTESIAN_POINT('Ctrl Pts',(0.754450441816411,-1.,4.05271876688106));
#48197=CARTESIAN_POINT('Ctrl Pts',(0.754450441816411,1.,4.05271876688106));
#48198=CARTESIAN_POINT('Ctrl Pts',(0.756271902370186,-1.,4.04517182654344));
#48199=CARTESIAN_POINT('Ctrl Pts',(0.756271902370186,1.,4.04517182654344));
#48200=CARTESIAN_POINT('Ctrl Pts',(0.758056338885553,-1.,4.03762485803468));
#48201=CARTESIAN_POINT('Ctrl Pts',(0.758056338885553,1.,4.03762485803468));
#48202=CARTESIAN_POINT('Ctrl Pts',(0.759803433244165,-1.,4.0300778195465));
#48203=CARTESIAN_POINT('Ctrl Pts',(0.759803433244165,1.,4.0300778195465));
#48204=CARTESIAN_POINT('Ctrl Pts',(0.761512875859941,-1.,4.02253072741347));
#48205=CARTESIAN_POINT('Ctrl Pts',(0.761512875859941,1.,4.02253072741347));
#48206=CARTESIAN_POINT('Ctrl Pts',(0.763184371182826,-1.,4.01498370680434));
#48207=CARTESIAN_POINT('Ctrl Pts',(0.763184371182826,1.,4.01498370680434));
#48208=CARTESIAN_POINT('Ctrl Pts',(0.764817648784946,-1.,4.00743706791366));
#48209=CARTESIAN_POINT('Ctrl Pts',(0.764817648784946,1.,4.00743706791366));
#48210=CARTESIAN_POINT('Ctrl Pts',(0.766412457135785,-1.,3.99989129179464));
#48211=CARTESIAN_POINT('Ctrl Pts',(0.766412457135785,1.,3.99989129179464));
#48212=CARTESIAN_POINT('Ctrl Pts',(0.767968531377707,-1.,3.99234687880892));
#48213=CARTESIAN_POINT('Ctrl Pts',(0.767968531377707,1.,3.99234687880892));
#48214=CARTESIAN_POINT('Ctrl Pts',(0.769485566245459,-1.,3.98480422348403));
#48215=CARTESIAN_POINT('Ctrl Pts',(0.769485566245459,1.,3.98480422348403));
#48216=CARTESIAN_POINT('Ctrl Pts',(0.770963190030503,-1.,3.97726349165507));
#48217=CARTESIAN_POINT('Ctrl Pts',(0.770963190030503,1.,3.97726349165507));
#48218=CARTESIAN_POINT('Ctrl Pts',(0.772400931772238,-1.,3.96972446532832));
#48219=CARTESIAN_POINT('Ctrl Pts',(0.772400931772238,1.,3.96972446532832));
#48220=CARTESIAN_POINT('Ctrl Pts',(0.773798212026682,-1.,3.96218649639876));
#48221=CARTESIAN_POINT('Ctrl Pts',(0.773798212026682,1.,3.96218649639876));
#48222=CARTESIAN_POINT('Ctrl Pts',(0.775154418039441,-1.,3.95464885452364));
#48223=CARTESIAN_POINT('Ctrl Pts',(0.775154418039441,1.,3.95464885452364));
#48224=CARTESIAN_POINT('Ctrl Pts',(0.776468966697959,-1.,3.94711101619471));
#48225=CARTESIAN_POINT('Ctrl Pts',(0.776468966697959,1.,3.94711101619471));
#48226=CARTESIAN_POINT('Ctrl Pts',(0.777741370568549,-1.,3.93957296768098));
#48227=CARTESIAN_POINT('Ctrl Pts',(0.777741370568549,1.,3.93957296768098));
#48228=CARTESIAN_POINT('Ctrl Pts',(0.778971308134786,-1.,3.93203552473153));
#48229=CARTESIAN_POINT('Ctrl Pts',(0.778971308134786,1.,3.93203552473153));
#48230=CARTESIAN_POINT('Ctrl Pts',(0.780158678615506,-1.,3.92450058323799));
#48231=CARTESIAN_POINT('Ctrl Pts',(0.780158678615506,1.,3.92450058323799));
#48232=CARTESIAN_POINT('Ctrl Pts',(0.781303428618343,-1.,3.9169703605466));
#48233=CARTESIAN_POINT('Ctrl Pts',(0.781303428618343,1.,3.9169703605466));
#48234=CARTESIAN_POINT('Ctrl Pts',(0.782405395622758,-1.,3.90944671004536));
#48235=CARTESIAN_POINT('Ctrl Pts',(0.782405395622758,1.,3.90944671004536));
#48236=CARTESIAN_POINT('Ctrl Pts',(0.783464141529082,-1.,3.90193039043971));
#48237=CARTESIAN_POINT('Ctrl Pts',(0.783464141529082,1.,3.90193039043971));
#48238=CARTESIAN_POINT('Ctrl Pts',(0.784478799358335,-1.,3.89442039235105));
#48239=CARTESIAN_POINT('Ctrl Pts',(0.784478799358335,1.,3.89442039235105));
#48240=CARTESIAN_POINT('Ctrl Pts',(0.785447890340723,-1.,3.88691313167399));
#48241=CARTESIAN_POINT('Ctrl Pts',(0.785447890340723,1.,3.88691313167399));
#48242=CARTESIAN_POINT('Ctrl Pts',(0.786369675812591,-1.,3.87940402818186));
#48243=CARTESIAN_POINT('Ctrl Pts',(0.786369675812591,1.,3.87940402818186));
#48244=CARTESIAN_POINT('Ctrl Pts',(0.78724252761798,-1.,3.87188916600905));
#48245=CARTESIAN_POINT('Ctrl Pts',(0.78724252761798,1.,3.87188916600905));
#48246=CARTESIAN_POINT('Ctrl Pts',(0.78806531509377,-1.,3.86436702561342));
#48247=CARTESIAN_POINT('Ctrl Pts',(0.78806531509377,1.,3.86436702561342));
#48248=CARTESIAN_POINT('Ctrl Pts',(0.788837734090688,-1.,3.85683995872536));
#48249=CARTESIAN_POINT('Ctrl Pts',(0.788837734090688,1.,3.85683995872536));
#48250=CARTESIAN_POINT('Ctrl Pts',(0.789560798155618,-1.,3.8493163780891));
#48251=CARTESIAN_POINT('Ctrl Pts',(0.789560798155618,1.,3.8493163780891));
#48252=CARTESIAN_POINT('Ctrl Pts',(0.790236124191289,-1.,3.84180762342476));
#48253=CARTESIAN_POINT('Ctrl Pts',(0.790236124191289,1.,3.84180762342476));
#48254=CARTESIAN_POINT('Ctrl Pts',(0.790865012705339,-1.,3.83432392054804));
#48255=CARTESIAN_POINT('Ctrl Pts',(0.790865012705339,1.,3.83432392054804));
#48256=CARTESIAN_POINT('Ctrl Pts',(0.791447528662381,-1.,3.82687033899799));
#48257=CARTESIAN_POINT('Ctrl Pts',(0.791447528662381,1.,3.82687033899799));
#48258=CARTESIAN_POINT('Ctrl Pts',(0.791981740718606,-1.,3.81944345442237));
#48259=CARTESIAN_POINT('Ctrl Pts',(0.791981740718606,1.,3.81944345442237));
#48260=CARTESIAN_POINT('Ctrl Pts',(0.792462483517568,-1.,3.81202588694726));
#48261=CARTESIAN_POINT('Ctrl Pts',(0.792462483517568,1.,3.81202588694726));
#48262=CARTESIAN_POINT('Ctrl Pts',(0.792882695234692,-1.,3.80459229925598));
#48263=CARTESIAN_POINT('Ctrl Pts',(0.792882695234692,1.,3.80459229925598));
#48264=CARTESIAN_POINT('Ctrl Pts',(0.7932356129732,-1.,3.79711921389862));
#48265=CARTESIAN_POINT('Ctrl Pts',(0.7932356129732,1.,3.79711921389862));
#48266=CARTESIAN_POINT('Ctrl Pts',(0.793516871680965,-1.,3.78959439439222));
#48267=CARTESIAN_POINT('Ctrl Pts',(0.793516871680965,1.,3.78959439439222));
#48268=CARTESIAN_POINT('Ctrl Pts',(0.793726235781339,-1.,3.78202460377617));
#48269=CARTESIAN_POINT('Ctrl Pts',(0.793726235781339,1.,3.78202460377617));
#48270=CARTESIAN_POINT('Ctrl Pts',(0.793870523787515,-1.,3.77444863801264));
#48271=CARTESIAN_POINT('Ctrl Pts',(0.793870523787515,1.,3.77444863801264));
#48272=CARTESIAN_POINT('Ctrl Pts',(0.793961083689141,-1.,3.76692626931184));
#48273=CARTESIAN_POINT('Ctrl Pts',(0.793961083689141,1.,3.76692626931184));
#48274=CARTESIAN_POINT('Ctrl Pts',(0.794008429135046,-1.,3.75951468666325));
#48275=CARTESIAN_POINT('Ctrl Pts',(0.794008429135046,1.,3.75951468666325));
#48276=CARTESIAN_POINT('Ctrl Pts',(0.79401734737144,-1.,3.75224692493895));
#48277=CARTESIAN_POINT('Ctrl Pts',(0.79401734737144,1.,3.75224692493895));
#48278=CARTESIAN_POINT('Ctrl Pts',(0.79398270045988,-1.,3.74511357728827));
#48279=CARTESIAN_POINT('Ctrl Pts',(0.79398270045988,1.,3.74511357728827));
#48280=CARTESIAN_POINT('Ctrl Pts',(0.79388270093679,-1.,3.73803280541576));
#48281=CARTESIAN_POINT('Ctrl Pts',(0.79388270093679,1.,3.73803280541576));
#48282=CARTESIAN_POINT('Ctrl Pts',(0.793682750269347,-1.,3.7308691469564));
#48283=CARTESIAN_POINT('Ctrl Pts',(0.793682750269347,1.,3.7308691469564));
#48284=CARTESIAN_POINT('Ctrl Pts',(0.79334702378387,-1.,3.7234879729357));
#48285=CARTESIAN_POINT('Ctrl Pts',(0.79334702378387,1.,3.7234879729357));
#48286=CARTESIAN_POINT('Ctrl Pts',(0.792848377370115,-1.,3.7158024239604));
#48287=CARTESIAN_POINT('Ctrl Pts',(0.792848377370115,1.,3.7158024239604));
#48288=CARTESIAN_POINT('Ctrl Pts',(0.792177688845967,-1.,3.70781724021879));
#48289=CARTESIAN_POINT('Ctrl Pts',(0.792177688845967,1.,3.70781724021879));
#48290=CARTESIAN_POINT('Ctrl Pts',(0.791356575696508,-1.,3.69968940808982));
#48291=CARTESIAN_POINT('Ctrl Pts',(0.791356575696508,1.,3.69968940808982));
#48292=CARTESIAN_POINT('Ctrl Pts',(0.790436284989579,-1.,3.69172044327754));
#48293=CARTESIAN_POINT('Ctrl Pts',(0.790436284989579,1.,3.69172044327754));
#48294=CARTESIAN_POINT('Ctrl Pts',(0.789483546065158,-1.,3.68428439784285));
#48295=CARTESIAN_POINT('Ctrl Pts',(0.789483546065158,1.,3.68428439784285));
#48296=CARTESIAN_POINT('Ctrl Pts',(0.788569566220662,-1.,3.67777119516438));
#48297=CARTESIAN_POINT('Ctrl Pts',(0.788569566220662,1.,3.67777119516438));
#48298=CARTESIAN_POINT('Ctrl Pts',(0.787758799995426,-1.,3.672529236635));
#48299=CARTESIAN_POINT('Ctrl Pts',(0.787758799995426,1.,3.672529236635));
#48300=CARTESIAN_POINT('Ctrl Pts',(0.787095252589507,-1.,3.66879484800625));
#48301=CARTESIAN_POINT('Ctrl Pts',(0.787095252589507,1.,3.66879484800625));
#48302=CARTESIAN_POINT('Ctrl Pts',(0.786698783541657,-1.,3.66710211819938));
#48303=CARTESIAN_POINT('Ctrl Pts',(0.786698783541657,1.,3.66710211819938));
#48304=CARTESIAN_POINT('Ctrl Pts',(0.786480236184947,-1.,3.66657784454965));
#48305=CARTESIAN_POINT('Ctrl Pts',(0.786480236184947,1.,3.66657784454965));
#48306=CARTESIAN_POINT('Ctrl Pts',(0.786369528183039,-1.,3.66655932661846));
#48307=CARTESIAN_POINT('Ctrl Pts',(0.786369528183039,1.,3.66655932661846));
#48308=CARTESIAN_POINT('Ctrl Pts',(0.786322922920599,-1.,3.66663282329846));
#48309=CARTESIAN_POINT('Ctrl Pts',(0.786322922920599,1.,3.66663282329846));
#48310=CARTESIAN_POINT('',(0.732042837400619,1.,4.13571194405636));
#48311=CARTESIAN_POINT('Ctrl Pts',(0.732042837400619,1.,4.13571194405636));
#48312=CARTESIAN_POINT('Ctrl Pts',(0.732488575135925,1.,4.13420383737278));
#48313=CARTESIAN_POINT('Ctrl Pts',(0.733376589325634,1.,4.13118752796397));
#48314=CARTESIAN_POINT('Ctrl Pts',(0.734698226767512,1.,4.12666277572794));
#48315=CARTESIAN_POINT('Ctrl Pts',(0.736439634335347,1.,4.12062919626082));
#48316=CARTESIAN_POINT('Ctrl Pts',(0.738581708229118,1.,4.11308626953795));
#48317=CARTESIAN_POINT('Ctrl Pts',(0.740688998555151,1.,4.1055424175856));
#48318=CARTESIAN_POINT('Ctrl Pts',(0.742761369690017,1.,4.09799769702712));
#48319=CARTESIAN_POINT('Ctrl Pts',(0.744798649705513,1.,4.09045220253011));
#48320=CARTESIAN_POINT('Ctrl Pts',(0.746800631490821,1.,4.08290608094789));
#48321=CARTESIAN_POINT('Ctrl Pts',(0.748767076679176,1.,4.07535951055363));
#48322=CARTESIAN_POINT('Ctrl Pts',(0.750697720483175,1.,4.06781267241886));
#48323=CARTESIAN_POINT('Ctrl Pts',(0.752592276482868,1.,4.06026572221399));
#48324=CARTESIAN_POINT('Ctrl Pts',(0.754450441816411,1.,4.05271876688106));
#48325=CARTESIAN_POINT('Ctrl Pts',(0.756271902370186,1.,4.04517182654344));
#48326=CARTESIAN_POINT('Ctrl Pts',(0.758056338885553,1.,4.03762485803468));
#48327=CARTESIAN_POINT('Ctrl Pts',(0.759803433244165,1.,4.0300778195465));
#48328=CARTESIAN_POINT('Ctrl Pts',(0.761512875859941,1.,4.02253072741347));
#48329=CARTESIAN_POINT('Ctrl Pts',(0.763184371182826,1.,4.01498370680434));
#48330=CARTESIAN_POINT('Ctrl Pts',(0.764817648784946,1.,4.00743706791366));
#48331=CARTESIAN_POINT('Ctrl Pts',(0.766412457135785,1.,3.99989129179464));
#48332=CARTESIAN_POINT('Ctrl Pts',(0.767968531377707,1.,3.99234687880892));
#48333=CARTESIAN_POINT('Ctrl Pts',(0.769485566245459,1.,3.98480422348403));
#48334=CARTESIAN_POINT('Ctrl Pts',(0.770963190030503,1.,3.97726349165507));
#48335=CARTESIAN_POINT('Ctrl Pts',(0.772400931772238,1.,3.96972446532832));
#48336=CARTESIAN_POINT('Ctrl Pts',(0.773798212026682,1.,3.96218649639876));
#48337=CARTESIAN_POINT('Ctrl Pts',(0.775154418039441,1.,3.95464885452364));
#48338=CARTESIAN_POINT('Ctrl Pts',(0.776468966697959,1.,3.94711101619471));
#48339=CARTESIAN_POINT('Ctrl Pts',(0.777741370568549,1.,3.93957296768098));
#48340=CARTESIAN_POINT('Ctrl Pts',(0.778971308134786,1.,3.93203552473153));
#48341=CARTESIAN_POINT('Ctrl Pts',(0.780158678615506,1.,3.92450058323799));
#48342=CARTESIAN_POINT('Ctrl Pts',(0.781303428618343,1.,3.9169703605466));
#48343=CARTESIAN_POINT('Ctrl Pts',(0.782405395622758,1.,3.90944671004536));
#48344=CARTESIAN_POINT('Ctrl Pts',(0.783464141529082,1.,3.90193039043971));
#48345=CARTESIAN_POINT('Ctrl Pts',(0.784478799358335,1.,3.89442039235105));
#48346=CARTESIAN_POINT('Ctrl Pts',(0.785447890340723,1.,3.88691313167399));
#48347=CARTESIAN_POINT('Ctrl Pts',(0.786369675812591,1.,3.87940402818186));
#48348=CARTESIAN_POINT('Ctrl Pts',(0.78724252761798,1.,3.87188916600905));
#48349=CARTESIAN_POINT('Ctrl Pts',(0.78806531509377,1.,3.86436702561342));
#48350=CARTESIAN_POINT('Ctrl Pts',(0.788837734090688,1.,3.85683995872536));
#48351=CARTESIAN_POINT('Ctrl Pts',(0.789560798155618,1.,3.8493163780891));
#48352=CARTESIAN_POINT('Ctrl Pts',(0.790236124191289,1.,3.84180762342476));
#48353=CARTESIAN_POINT('Ctrl Pts',(0.790865012705339,1.,3.83432392054804));
#48354=CARTESIAN_POINT('Ctrl Pts',(0.791447528662381,1.,3.82687033899799));
#48355=CARTESIAN_POINT('Ctrl Pts',(0.791981740718606,1.,3.81944345442237));
#48356=CARTESIAN_POINT('Ctrl Pts',(0.792462483517568,1.,3.81202588694726));
#48357=CARTESIAN_POINT('Ctrl Pts',(0.792882695234692,1.,3.80459229925598));
#48358=CARTESIAN_POINT('Ctrl Pts',(0.7932356129732,1.,3.79711921389862));
#48359=CARTESIAN_POINT('Ctrl Pts',(0.793516871680965,1.,3.78959439439222));
#48360=CARTESIAN_POINT('Ctrl Pts',(0.793726235781339,1.,3.78202460377617));
#48361=CARTESIAN_POINT('Ctrl Pts',(0.793870523787515,1.,3.77444863801264));
#48362=CARTESIAN_POINT('Ctrl Pts',(0.793961083689141,1.,3.76692626931184));
#48363=CARTESIAN_POINT('Ctrl Pts',(0.794008429135046,1.,3.75951468666325));
#48364=CARTESIAN_POINT('Ctrl Pts',(0.79401734737144,1.,3.75224692493895));
#48365=CARTESIAN_POINT('Ctrl Pts',(0.79398270045988,1.,3.74511357728827));
#48366=CARTESIAN_POINT('Ctrl Pts',(0.79388270093679,1.,3.73803280541576));
#48367=CARTESIAN_POINT('Ctrl Pts',(0.793682750269347,1.,3.7308691469564));
#48368=CARTESIAN_POINT('Ctrl Pts',(0.79334702378387,1.,3.7234879729357));
#48369=CARTESIAN_POINT('Ctrl Pts',(0.792848377370115,1.,3.7158024239604));
#48370=CARTESIAN_POINT('Ctrl Pts',(0.792177688845967,1.,3.70781724021879));
#48371=CARTESIAN_POINT('Ctrl Pts',(0.791356575696508,1.,3.69968940808982));
#48372=CARTESIAN_POINT('Ctrl Pts',(0.790436284989579,1.,3.69172044327754));
#48373=CARTESIAN_POINT('Ctrl Pts',(0.789483546065158,1.,3.68428439784285));
#48374=CARTESIAN_POINT('Ctrl Pts',(0.788569566220662,1.,3.67777119516438));
#48375=CARTESIAN_POINT('Ctrl Pts',(0.787758799995426,1.,3.672529236635));
#48376=CARTESIAN_POINT('Ctrl Pts',(0.787145041181588,1.,3.66907505398769));
#48377=CARTESIAN_POINT('Ctrl Pts',(0.786774337198499,1.,3.66743103898844));
#48378=CARTESIAN_POINT('Ctrl Pts',(0.786565919559889,1.,3.66680946938396));
#48379=CARTESIAN_POINT('Ctrl Pts',(0.786459983896781,1.,3.66664310415236));
#48380=CARTESIAN_POINT('Ctrl Pts',(0.786422660833743,1.,3.66661143271648));
#48381=CARTESIAN_POINT('',(0.732042837400619,0.,4.13571194405636));
#48382=CARTESIAN_POINT('Ctrl Pts',(0.385214314776328,-1.,3.73016218570874));
#48383=CARTESIAN_POINT('Ctrl Pts',(0.385214314776328,1.,3.73016218570874));
#48384=CARTESIAN_POINT('Ctrl Pts',(0.385147278814803,-1.,3.73010668803185));
#48385=CARTESIAN_POINT('Ctrl Pts',(0.385147278814803,1.,3.73010668803185));
#48386=CARTESIAN_POINT('Ctrl Pts',(0.385047711603887,-1.,3.73015851028729));
#48387=CARTESIAN_POINT('Ctrl Pts',(0.385047711603887,1.,3.73015851028729));
#48388=CARTESIAN_POINT('Ctrl Pts',(0.385001870183841,-1.,3.73072465900727));
#48389=CARTESIAN_POINT('Ctrl Pts',(0.385001870183841,1.,3.73072465900727));
#48390=CARTESIAN_POINT('Ctrl Pts',(0.385147887989514,-1.,3.73245705639337));
#48391=CARTESIAN_POINT('Ctrl Pts',(0.385147887989514,1.,3.73245705639337));
#48392=CARTESIAN_POINT('Ctrl Pts',(0.385670806454744,-1.,3.73621371845475));
#48393=CARTESIAN_POINT('Ctrl Pts',(0.385670806454744,1.,3.73621371845475));
#48394=CARTESIAN_POINT('Ctrl Pts',(0.386519576222035,-1.,3.74144965781088));
#48395=CARTESIAN_POINT('Ctrl Pts',(0.386519576222035,1.,3.74144965781088));
#48396=CARTESIAN_POINT('Ctrl Pts',(0.387663020050396,-1.,3.74792651696269));
#48397=CARTESIAN_POINT('Ctrl Pts',(0.387663020050396,1.,3.74792651696269));
#48398=CARTESIAN_POINT('Ctrl Pts',(0.38905477589825,-1.,3.75529302894757));
#48399=CARTESIAN_POINT('Ctrl Pts',(0.38905477589825,1.,3.75529302894757));
#48400=CARTESIAN_POINT('Ctrl Pts',(0.390642072979258,-1.,3.76315635032993));
#48401=CARTESIAN_POINT('Ctrl Pts',(0.390642072979258,1.,3.76315635032993));
#48402=CARTESIAN_POINT('Ctrl Pts',(0.392372786223346,-1.,3.77114011595892));
#48403=CARTESIAN_POINT('Ctrl Pts',(0.392372786223346,1.,3.77114011595892));
#48404=CARTESIAN_POINT('Ctrl Pts',(0.394202481011595,-1.,3.77894173114368));
#48405=CARTESIAN_POINT('Ctrl Pts',(0.394202481011595,1.,3.77894173114368));
#48406=CARTESIAN_POINT('Ctrl Pts',(0.396103205335028,-1.,3.78640521279479));
#48407=CARTESIAN_POINT('Ctrl Pts',(0.396103205335028,1.,3.78640521279479));
#48408=CARTESIAN_POINT('Ctrl Pts',(0.398064818684158,-1.,3.79352887163457));
#48409=CARTESIAN_POINT('Ctrl Pts',(0.398064818684158,1.,3.79352887163457));
#48410=CARTESIAN_POINT('Ctrl Pts',(0.400088346504726,-1.,3.80040370384659));
#48411=CARTESIAN_POINT('Ctrl Pts',(0.400088346504726,1.,3.80040370384659));
#48412=CARTESIAN_POINT('Ctrl Pts',(0.402181320148474,-1.,3.80716881962763));
#48413=CARTESIAN_POINT('Ctrl Pts',(0.402181320148474,1.,3.80716881962763));
#48414=CARTESIAN_POINT('Ctrl Pts',(0.404352694628236,-1.,3.81396374287762));
#48415=CARTESIAN_POINT('Ctrl Pts',(0.404352694628236,1.,3.81396374287762));
#48416=CARTESIAN_POINT('Ctrl Pts',(0.406607038258906,-1.,3.82087303913741));
#48417=CARTESIAN_POINT('Ctrl Pts',(0.406607038258906,1.,3.82087303913741));
#48418=CARTESIAN_POINT('Ctrl Pts',(0.408942371447376,-1.,3.82790724256397));
#48419=CARTESIAN_POINT('Ctrl Pts',(0.408942371447376,1.,3.82790724256397));
#48420=CARTESIAN_POINT('Ctrl Pts',(0.411353038798459,-1.,3.83503345578645));
#48421=CARTESIAN_POINT('Ctrl Pts',(0.411353038798459,1.,3.83503345578645));
#48422=CARTESIAN_POINT('Ctrl Pts',(0.413831367016726,-1.,3.84219403994742));
#48423=CARTESIAN_POINT('Ctrl Pts',(0.413831367016726,1.,3.84219403994742));
#48424=CARTESIAN_POINT('Ctrl Pts',(0.41636967805292,-1.,3.8493286415751));
#48425=CARTESIAN_POINT('Ctrl Pts',(0.41636967805292,1.,3.8493286415751));
#48426=CARTESIAN_POINT('Ctrl Pts',(0.418962468086809,-1.,3.85639825648031));
#48427=CARTESIAN_POINT('Ctrl Pts',(0.418962468086809,1.,3.85639825648031));
#48428=CARTESIAN_POINT('Ctrl Pts',(0.421607423177575,-1.,3.86339652542749));
#48429=CARTESIAN_POINT('Ctrl Pts',(0.421607423177575,1.,3.86339652542749));
#48430=CARTESIAN_POINT('Ctrl Pts',(0.424304173195142,-1.,3.87033643487882));
#48431=CARTESIAN_POINT('Ctrl Pts',(0.424304173195142,1.,3.87033643487882));
#48432=CARTESIAN_POINT('Ctrl Pts',(0.427053541173469,-1.,3.87724240306609));
#48433=CARTESIAN_POINT('Ctrl Pts',(0.427053541173469,1.,3.87724240306609));
#48434=CARTESIAN_POINT('Ctrl Pts',(0.429856640579733,-1.,3.88414070943334));
#48435=CARTESIAN_POINT('Ctrl Pts',(0.429856640579733,1.,3.88414070943334));
#48436=CARTESIAN_POINT('Ctrl Pts',(0.432713929544439,-1.,3.89104947940592));
#48437=CARTESIAN_POINT('Ctrl Pts',(0.432713929544439,1.,3.89104947940592));
#48438=CARTESIAN_POINT('Ctrl Pts',(0.435624629433505,-1.,3.8979725665544));
#48439=CARTESIAN_POINT('Ctrl Pts',(0.435624629433505,1.,3.8979725665544));
#48440=CARTESIAN_POINT('Ctrl Pts',(0.438587235458233,-1.,3.90490512938546));
#48441=CARTESIAN_POINT('Ctrl Pts',(0.438587235458233,1.,3.90490512938546));
#48442=CARTESIAN_POINT('Ctrl Pts',(0.441599824524047,-1.,3.91183704069146));
#48443=CARTESIAN_POINT('Ctrl Pts',(0.441599824524047,1.,3.91183704069146));
#48444=CARTESIAN_POINT('Ctrl Pts',(0.444660430230592,-1.,3.91875701610721));
#48445=CARTESIAN_POINT('Ctrl Pts',(0.444660430230592,1.,3.91875701610721));
#48446=CARTESIAN_POINT('Ctrl Pts',(0.447767416837296,-1.,3.92565674143424));
#48447=CARTESIAN_POINT('Ctrl Pts',(0.447767416837296,1.,3.92565674143424));
#48448=CARTESIAN_POINT('Ctrl Pts',(0.450919768356346,-1.,3.93253407403128));
#48449=CARTESIAN_POINT('Ctrl Pts',(0.450919768356346,1.,3.93253407403128));
#48450=CARTESIAN_POINT('Ctrl Pts',(0.454116879027575,-1.,3.93939080846298));
#48451=CARTESIAN_POINT('Ctrl Pts',(0.454116879027575,1.,3.93939080846298));
#48452=CARTESIAN_POINT('Ctrl Pts',(0.457358410451673,-1.,3.94623117206675));
#48453=CARTESIAN_POINT('Ctrl Pts',(0.457358410451673,1.,3.94623117206675));
#48454=CARTESIAN_POINT('Ctrl Pts',(0.460644124429119,-1.,3.95306005817363));
#48455=CARTESIAN_POINT('Ctrl Pts',(0.460644124429119,1.,3.95306005817363));
#48456=CARTESIAN_POINT('Ctrl Pts',(0.463973722115744,-1.,3.95988133243543));
#48457=CARTESIAN_POINT('Ctrl Pts',(0.463973722115744,1.,3.95988133243543));
#48458=CARTESIAN_POINT('Ctrl Pts',(0.467346690880671,-1.,3.96669622273946));
#48459=CARTESIAN_POINT('Ctrl Pts',(0.467346690880671,1.,3.96669622273946));
#48460=CARTESIAN_POINT('Ctrl Pts',(0.470762379613477,-1.,3.97350414289415));
#48461=CARTESIAN_POINT('Ctrl Pts',(0.470762379613477,1.,3.97350414289415));
#48462=CARTESIAN_POINT('Ctrl Pts',(0.474220061019542,-1.,3.9803033804443));
#48463=CARTESIAN_POINT('Ctrl Pts',(0.474220061019542,1.,3.9803033804443));
#48464=CARTESIAN_POINT('Ctrl Pts',(0.477718999122033,-1.,3.98709184306743));
#48465=CARTESIAN_POINT('Ctrl Pts',(0.477718999122033,1.,3.98709184306743));
#48466=CARTESIAN_POINT('Ctrl Pts',(0.481258512209637,-1.,3.99386775880655));
#48467=CARTESIAN_POINT('Ctrl Pts',(0.481258512209637,1.,3.99386775880655));
#48468=CARTESIAN_POINT('Ctrl Pts',(0.484838042421754,-1.,4.00063045119234));
#48469=CARTESIAN_POINT('Ctrl Pts',(0.484838042421754,1.,4.00063045119234));
#48470=CARTESIAN_POINT('Ctrl Pts',(0.48845713042453,-1.,4.0073800839092));
#48471=CARTESIAN_POINT('Ctrl Pts',(0.48845713042453,1.,4.0073800839092));
#48472=CARTESIAN_POINT('Ctrl Pts',(0.49211538341793,-1.,4.01411733503486));
#48473=CARTESIAN_POINT('Ctrl Pts',(0.49211538341793,1.,4.01411733503486));
#48474=CARTESIAN_POINT('Ctrl Pts',(0.495812444326222,-1.,4.02084308851813));
#48475=CARTESIAN_POINT('Ctrl Pts',(0.495812444326222,1.,4.02084308851813));
#48476=CARTESIAN_POINT('Ctrl Pts',(0.499547962340889,-1.,4.0275581398015));
#48477=CARTESIAN_POINT('Ctrl Pts',(0.499547962340889,1.,4.0275581398015));
#48478=CARTESIAN_POINT('Ctrl Pts',(0.503321556915513,-1.,4.0342628417439));
#48479=CARTESIAN_POINT('Ctrl Pts',(0.503321556915513,1.,4.0342628417439));
#48480=CARTESIAN_POINT('Ctrl Pts',(0.507132823288361,-1.,4.04095715149074));
#48481=CARTESIAN_POINT('Ctrl Pts',(0.507132823288361,1.,4.04095715149074));
#48482=CARTESIAN_POINT('Ctrl Pts',(0.510981349219173,-1.,4.04764078815591));
#48483=CARTESIAN_POINT('Ctrl Pts',(0.510981349219173,1.,4.04764078815591));
#48484=CARTESIAN_POINT('Ctrl Pts',(0.514866728193103,-1.,4.05431335771261));
#48485=CARTESIAN_POINT('Ctrl Pts',(0.514866728193103,1.,4.05431335771261));
#48486=CARTESIAN_POINT('Ctrl Pts',(0.518788572336809,-1.,4.06097448037934));
#48487=CARTESIAN_POINT('Ctrl Pts',(0.518788572336809,1.,4.06097448037934));
#48488=CARTESIAN_POINT('Ctrl Pts',(0.522746528602767,-1.,4.06762394471075));
#48489=CARTESIAN_POINT('Ctrl Pts',(0.522746528602767,1.,4.06762394471075));
#48490=CARTESIAN_POINT('Ctrl Pts',(0.526740277226999,-1.,4.07426172299496));
#48491=CARTESIAN_POINT('Ctrl Pts',(0.526740277226999,1.,4.07426172299496));
#48492=CARTESIAN_POINT('Ctrl Pts',(0.530769518728075,-1.,4.08088789536488));
#48493=CARTESIAN_POINT('Ctrl Pts',(0.530769518728075,1.,4.08088789536488));
#48494=CARTESIAN_POINT('Ctrl Pts',(0.534833963476999,-1.,4.08750259988693));
#48495=CARTESIAN_POINT('Ctrl Pts',(0.534833963476999,1.,4.08750259988693));
#48496=CARTESIAN_POINT('Ctrl Pts',(0.53893332117992,-1.,4.09410597627116));
#48497=CARTESIAN_POINT('Ctrl Pts',(0.53893332117992,1.,4.09410597627116));
#48498=CARTESIAN_POINT('Ctrl Pts',(0.543067286878457,-1.,4.10069810244473));
#48499=CARTESIAN_POINT('Ctrl Pts',(0.543067286878457,1.,4.10069810244473));
#48500=CARTESIAN_POINT('Ctrl Pts',(0.547235539486759,-1.,4.1072789702877));
#48501=CARTESIAN_POINT('Ctrl Pts',(0.547235539486759,1.,4.1072789702877));
#48502=CARTESIAN_POINT('Ctrl Pts',(0.551437758498246,-1.,4.11384852025578));
#48503=CARTESIAN_POINT('Ctrl Pts',(0.551437758498246,1.,4.11384852025578));
#48504=CARTESIAN_POINT('Ctrl Pts',(0.555673636130778,-1.,4.1204066619623));
#48505=CARTESIAN_POINT('Ctrl Pts',(0.555673636130778,1.,4.1204066619623));
#48506=CARTESIAN_POINT('Ctrl Pts',(0.559942890594628,-1.,4.12695329951859));
#48507=CARTESIAN_POINT('Ctrl Pts',(0.559942890594628,1.,4.12695329951859));
#48508=CARTESIAN_POINT('Ctrl Pts',(0.564245279535705,-1.,4.13348835726086));
#48509=CARTESIAN_POINT('Ctrl Pts',(0.564245279535705,1.,4.13348835726086));
#48510=CARTESIAN_POINT('Ctrl Pts',(0.568580610187115,-1.,4.14001179828669));
#48511=CARTESIAN_POINT('Ctrl Pts',(0.568580610187115,1.,4.14001179828669));
#48512=CARTESIAN_POINT('Ctrl Pts',(0.572948736066276,-1.,4.14652361065787));
#48513=CARTESIAN_POINT('Ctrl Pts',(0.572948736066276,1.,4.14652361065787));
#48514=CARTESIAN_POINT('Ctrl Pts',(0.576469391673916,-1.,4.1517237611974));
#48515=CARTESIAN_POINT('Ctrl Pts',(0.576469391673916,1.,4.1517237611974));
#48516=CARTESIAN_POINT('Ctrl Pts',(0.579124568912543,-1.,4.15561864787379));
#48517=CARTESIAN_POINT('Ctrl Pts',(0.579124568912543,1.,4.15561864787379));
#48518=CARTESIAN_POINT('Ctrl Pts',(0.580901211462913,-1.,4.15821291712391));
#48519=CARTESIAN_POINT('Ctrl Pts',(0.580901211462913,1.,4.15821291712391));
#48520=CARTESIAN_POINT('Ctrl Pts',(0.581791163835814,-1.,4.15950947128175));
#48521=CARTESIAN_POINT('Ctrl Pts',(0.581791163835814,1.,4.15950947128175));
#48522=CARTESIAN_POINT('',(0.385112848332548,1.,3.73017266276632));
#48523=CARTESIAN_POINT('Ctrl Pts',(0.385112848332548,-1.,3.73017266276632));
#48524=CARTESIAN_POINT('Ctrl Pts',(0.385112848332548,-0.666666666666667,
3.73017266276632));
#48525=CARTESIAN_POINT('Ctrl Pts',(0.385112848332548,-0.333333333333333,
3.73017266276632));
#48526=CARTESIAN_POINT('Ctrl Pts',(0.385112848332548,0.333333333333333,
3.73017266276632));
#48527=CARTESIAN_POINT('Ctrl Pts',(0.385112848332548,0.666666666666667,
3.73017266276632));
#48528=CARTESIAN_POINT('Ctrl Pts',(0.385112848332548,1.,3.73017266276632));
#48529=CARTESIAN_POINT('',(0.581791163835814,1.,4.15950947128175));
#48530=CARTESIAN_POINT('',(0.581791163835814,0.,4.15950947128175));
#48531=CARTESIAN_POINT('Ctrl Pts',(0.385112848332549,1.,3.73017266276632));
#48532=CARTESIAN_POINT('Ctrl Pts',(0.385087139001608,1.,3.73021431755218));
#48533=CARTESIAN_POINT('Ctrl Pts',(0.385037797882046,1.,3.73040527620929));
#48534=CARTESIAN_POINT('Ctrl Pts',(0.385031656499141,1.,3.731060828624));
#48535=CARTESIAN_POINT('Ctrl Pts',(0.385187124633964,1.,3.73273893363318));
#48536=CARTESIAN_POINT('Ctrl Pts',(0.385670806454744,1.,3.73621371845475));
#48537=CARTESIAN_POINT('Ctrl Pts',(0.386519576222035,1.,3.74144965781088));
#48538=CARTESIAN_POINT('Ctrl Pts',(0.387663020050396,1.,3.74792651696269));
#48539=CARTESIAN_POINT('Ctrl Pts',(0.38905477589825,1.,3.75529302894757));
#48540=CARTESIAN_POINT('Ctrl Pts',(0.390642072979258,1.,3.76315635032993));
#48541=CARTESIAN_POINT('Ctrl Pts',(0.392372786223346,1.,3.77114011595892));
#48542=CARTESIAN_POINT('Ctrl Pts',(0.394202481011595,1.,3.77894173114368));
#48543=CARTESIAN_POINT('Ctrl Pts',(0.396103205335028,1.,3.78640521279479));
#48544=CARTESIAN_POINT('Ctrl Pts',(0.398064818684158,1.,3.79352887163457));
#48545=CARTESIAN_POINT('Ctrl Pts',(0.400088346504726,1.,3.80040370384659));
#48546=CARTESIAN_POINT('Ctrl Pts',(0.402181320148474,1.,3.80716881962763));
#48547=CARTESIAN_POINT('Ctrl Pts',(0.404352694628236,1.,3.81396374287762));
#48548=CARTESIAN_POINT('Ctrl Pts',(0.406607038258906,1.,3.82087303913741));
#48549=CARTESIAN_POINT('Ctrl Pts',(0.408942371447376,1.,3.82790724256397));
#48550=CARTESIAN_POINT('Ctrl Pts',(0.411353038798459,1.,3.83503345578645));
#48551=CARTESIAN_POINT('Ctrl Pts',(0.413831367016726,1.,3.84219403994742));
#48552=CARTESIAN_POINT('Ctrl Pts',(0.41636967805292,1.,3.8493286415751));
#48553=CARTESIAN_POINT('Ctrl Pts',(0.418962468086809,1.,3.85639825648031));
#48554=CARTESIAN_POINT('Ctrl Pts',(0.421607423177575,1.,3.86339652542749));
#48555=CARTESIAN_POINT('Ctrl Pts',(0.424304173195142,1.,3.87033643487882));
#48556=CARTESIAN_POINT('Ctrl Pts',(0.427053541173469,1.,3.87724240306609));
#48557=CARTESIAN_POINT('Ctrl Pts',(0.429856640579733,1.,3.88414070943334));
#48558=CARTESIAN_POINT('Ctrl Pts',(0.432713929544439,1.,3.89104947940592));
#48559=CARTESIAN_POINT('Ctrl Pts',(0.435624629433505,1.,3.8979725665544));
#48560=CARTESIAN_POINT('Ctrl Pts',(0.438587235458233,1.,3.90490512938546));
#48561=CARTESIAN_POINT('Ctrl Pts',(0.441599824524047,1.,3.91183704069146));
#48562=CARTESIAN_POINT('Ctrl Pts',(0.444660430230592,1.,3.91875701610721));
#48563=CARTESIAN_POINT('Ctrl Pts',(0.447767416837296,1.,3.92565674143424));
#48564=CARTESIAN_POINT('Ctrl Pts',(0.450919768356346,1.,3.93253407403128));
#48565=CARTESIAN_POINT('Ctrl Pts',(0.454116879027575,1.,3.93939080846298));
#48566=CARTESIAN_POINT('Ctrl Pts',(0.457358410451673,1.,3.94623117206675));
#48567=CARTESIAN_POINT('Ctrl Pts',(0.460644124429119,1.,3.95306005817363));
#48568=CARTESIAN_POINT('Ctrl Pts',(0.463973722115744,1.,3.95988133243543));
#48569=CARTESIAN_POINT('Ctrl Pts',(0.467346690880671,1.,3.96669622273946));
#48570=CARTESIAN_POINT('Ctrl Pts',(0.470762379613477,1.,3.97350414289415));
#48571=CARTESIAN_POINT('Ctrl Pts',(0.474220061019542,1.,3.9803033804443));
#48572=CARTESIAN_POINT('Ctrl Pts',(0.477718999122033,1.,3.98709184306743));
#48573=CARTESIAN_POINT('Ctrl Pts',(0.481258512209637,1.,3.99386775880655));
#48574=CARTESIAN_POINT('Ctrl Pts',(0.484838042421754,1.,4.00063045119234));
#48575=CARTESIAN_POINT('Ctrl Pts',(0.48845713042453,1.,4.0073800839092));
#48576=CARTESIAN_POINT('Ctrl Pts',(0.49211538341793,1.,4.01411733503486));
#48577=CARTESIAN_POINT('Ctrl Pts',(0.495812444326222,1.,4.02084308851813));
#48578=CARTESIAN_POINT('Ctrl Pts',(0.499547962340889,1.,4.0275581398015));
#48579=CARTESIAN_POINT('Ctrl Pts',(0.503321556915513,1.,4.0342628417439));
#48580=CARTESIAN_POINT('Ctrl Pts',(0.507132823288361,1.,4.04095715149074));
#48581=CARTESIAN_POINT('Ctrl Pts',(0.510981349219173,1.,4.04764078815591));
#48582=CARTESIAN_POINT('Ctrl Pts',(0.514866728193103,1.,4.05431335771261));
#48583=CARTESIAN_POINT('Ctrl Pts',(0.518788572336809,1.,4.06097448037934));
#48584=CARTESIAN_POINT('Ctrl Pts',(0.522746528602767,1.,4.06762394471075));
#48585=CARTESIAN_POINT('Ctrl Pts',(0.526740277226999,1.,4.07426172299496));
#48586=CARTESIAN_POINT('Ctrl Pts',(0.530769518728075,1.,4.08088789536488));
#48587=CARTESIAN_POINT('Ctrl Pts',(0.534833963476999,1.,4.08750259988693));
#48588=CARTESIAN_POINT('Ctrl Pts',(0.53893332117992,1.,4.09410597627116));
#48589=CARTESIAN_POINT('Ctrl Pts',(0.543067286878457,1.,4.10069810244473));
#48590=CARTESIAN_POINT('Ctrl Pts',(0.547235539486759,1.,4.1072789702877));
#48591=CARTESIAN_POINT('Ctrl Pts',(0.551437758498246,1.,4.11384852025578));
#48592=CARTESIAN_POINT('Ctrl Pts',(0.555673636130778,1.,4.1204066619623));
#48593=CARTESIAN_POINT('Ctrl Pts',(0.559942890594628,1.,4.12695329951859));
#48594=CARTESIAN_POINT('Ctrl Pts',(0.564245279535705,1.,4.13348835726086));
#48595=CARTESIAN_POINT('Ctrl Pts',(0.568580610187115,1.,4.14001179828669));
#48596=CARTESIAN_POINT('Ctrl Pts',(0.572948736066276,1.,4.14652361065787));
#48597=CARTESIAN_POINT('Ctrl Pts',(0.576469391673916,1.,4.1517237611974));
#48598=CARTESIAN_POINT('Ctrl Pts',(0.579124568912543,1.,4.15561864787379));
#48599=CARTESIAN_POINT('Ctrl Pts',(0.580901211462913,1.,4.15821291712391));
#48600=CARTESIAN_POINT('Ctrl Pts',(0.581791163835814,1.,4.15950947128175));
#48601=CARTESIAN_POINT('Origin',(0.581791163835814,0.,4.15950947128175));
#48602=CARTESIAN_POINT('',(0.732042837400619,1.,4.13571194405636));
#48603=CARTESIAN_POINT('Origin',(0.,0.,0.));
#48604=CARTESIAN_POINT('',(0.203156094897895,1.,3.74449296982994));
#48605=CARTESIAN_POINT('Origin',(0.,1.,0.));
#48606=CARTESIAN_POINT('Ctrl Pts',(0.203156094897895,1.,3.74449296982994));
#48607=CARTESIAN_POINT('Ctrl Pts',(0.203156094897895,0.666666666666667,
3.74449296982994));
#48608=CARTESIAN_POINT('Ctrl Pts',(0.203156094897895,0.333333333333333,
3.74449296982994));
#48609=CARTESIAN_POINT('Ctrl Pts',(0.203156094897895,-0.333333333333333,
3.74449296982994));
#48610=CARTESIAN_POINT('Ctrl Pts',(0.203156094897895,-0.666666666666667,
3.74449296982994));
#48611=CARTESIAN_POINT('Ctrl Pts',(0.203156094897895,-1.,3.74449296982994));
#48612=CARTESIAN_POINT('Ctrl Pts',(0.0760622897878233,-1.,4.19931119685982));
#48613=CARTESIAN_POINT('Ctrl Pts',(0.0760622897878233,1.,4.19931119685982));
#48614=CARTESIAN_POINT('Ctrl Pts',(0.0767384596142192,-1.,4.19789138621624));
#48615=CARTESIAN_POINT('Ctrl Pts',(0.0767384596142192,1.,4.19789138621624));
#48616=CARTESIAN_POINT('Ctrl Pts',(0.0780873956244399,-1.,4.19505112860624));
#48617=CARTESIAN_POINT('Ctrl Pts',(0.0780873956244399,1.,4.19505112860624));
#48618=CARTESIAN_POINT('Ctrl Pts',(0.08010058871176,-1.,4.19078883322483));
#48619=CARTESIAN_POINT('Ctrl Pts',(0.08010058871176,1.,4.19078883322483));
#48620=CARTESIAN_POINT('Ctrl Pts',(0.0827644164389507,-1.,4.1851019532944));
#48621=CARTESIAN_POINT('Ctrl Pts',(0.0827644164389507,1.,4.1851019532944));
#48622=CARTESIAN_POINT('Ctrl Pts',(0.0860600915552512,-1.,4.17798698669991));
#48623=CARTESIAN_POINT('Ctrl Pts',(0.0860600915552512,1.,4.17798698669991));
#48624=CARTESIAN_POINT('Ctrl Pts',(0.0893215560850325,-1.,4.17086566491823));
#48625=CARTESIAN_POINT('Ctrl Pts',(0.0893215560850325,1.,4.17086566491823));
#48626=CARTESIAN_POINT('Ctrl Pts',(0.0925486672167687,-1.,4.16373802265942));
#48627=CARTESIAN_POINT('Ctrl Pts',(0.0925486672167687,1.,4.16373802265942));
#48628=CARTESIAN_POINT('Ctrl Pts',(0.0957412403297065,-1.,4.15660412653006));
#48629=CARTESIAN_POINT('Ctrl Pts',(0.0957412403297065,1.,4.15660412653006));
#48630=CARTESIAN_POINT('Ctrl Pts',(0.0988990478899809,-1.,4.1494640891762));
#48631=CARTESIAN_POINT('Ctrl Pts',(0.0988990478899809,1.,4.1494640891762));
#48632=CARTESIAN_POINT('Ctrl Pts',(0.102021826577453,-1.,4.14231804938737));
#48633=CARTESIAN_POINT('Ctrl Pts',(0.102021826577453,1.,4.14231804938737));
#48634=CARTESIAN_POINT('Ctrl Pts',(0.105109286538864,-1.,4.13516614458396));
#48635=CARTESIAN_POINT('Ctrl Pts',(0.105109286538864,1.,4.13516614458396));
#48636=CARTESIAN_POINT('Ctrl Pts',(0.10816112052835,-1.,4.12800848371386));
#48637=CARTESIAN_POINT('Ctrl Pts',(0.10816112052835,1.,4.12800848371386));
#48638=CARTESIAN_POINT('Ctrl Pts',(0.111177012683377,-1.,4.12084512502444));
#48639=CARTESIAN_POINT('Ctrl Pts',(0.111177012683377,1.,4.12084512502444));
#48640=CARTESIAN_POINT('Ctrl Pts',(0.114156649609601,-1.,4.11367603925313));
#48641=CARTESIAN_POINT('Ctrl Pts',(0.114156649609601,1.,4.11367603925313));
#48642=CARTESIAN_POINT('Ctrl Pts',(0.117099722731704,-1.,4.10650113382187));
#48643=CARTESIAN_POINT('Ctrl Pts',(0.117099722731704,1.,4.10650113382187));
#48644=CARTESIAN_POINT('Ctrl Pts',(0.120005924388162,-1.,4.09932031767243));
#48645=CARTESIAN_POINT('Ctrl Pts',(0.120005924388162,1.,4.09932031767243));
#48646=CARTESIAN_POINT('Ctrl Pts',(0.122874946249119,-1.,4.09213355850836));
#48647=CARTESIAN_POINT('Ctrl Pts',(0.122874946249119,1.,4.09213355850836));
#48648=CARTESIAN_POINT('Ctrl Pts',(0.125706476822529,-1.,4.08494093372315));
#48649=CARTESIAN_POINT('Ctrl Pts',(0.125706476822529,1.,4.08494093372315));
#48650=CARTESIAN_POINT('Ctrl Pts',(0.128500200484813,-1.,4.07774270738809));
#48651=CARTESIAN_POINT('Ctrl Pts',(0.128500200484813,1.,4.07774270738809));
#48652=CARTESIAN_POINT('Ctrl Pts',(0.131255793548914,-1.,4.07053931528579));
#48653=CARTESIAN_POINT('Ctrl Pts',(0.131255793548914,1.,4.07053931528579));
#48654=CARTESIAN_POINT('Ctrl Pts',(0.133972916144225,-1.,4.06333121018476));
#48655=CARTESIAN_POINT('Ctrl Pts',(0.133972916144225,1.,4.06333121018476));
#48656=CARTESIAN_POINT('Ctrl Pts',(0.136651205046111,-1.,4.05611873400122));
#48657=CARTESIAN_POINT('Ctrl Pts',(0.136651205046111,1.,4.05611873400122));
#48658=CARTESIAN_POINT('Ctrl Pts',(0.139290267180059,-1.,4.04890199238056));
#48659=CARTESIAN_POINT('Ctrl Pts',(0.139290267180059,1.,4.04890199238056));
#48660=CARTESIAN_POINT('Ctrl Pts',(0.141889671485507,-1.,4.04168069633842));
#48661=CARTESIAN_POINT('Ctrl Pts',(0.141889671485507,1.,4.04168069633842));
#48662=CARTESIAN_POINT('Ctrl Pts',(0.144448947038352,-1.,4.03445411510403));
#48663=CARTESIAN_POINT('Ctrl Pts',(0.144448947038352,1.,4.03445411510403));
#48664=CARTESIAN_POINT('Ctrl Pts',(0.146967602878998,-1.,4.02722143147048));
#48665=CARTESIAN_POINT('Ctrl Pts',(0.146967602878998,1.,4.02722143147048));
#48666=CARTESIAN_POINT('Ctrl Pts',(0.149445144968707,-1.,4.01998203715588));
#48667=CARTESIAN_POINT('Ctrl Pts',(0.149445144968707,1.,4.01998203715588));
#48668=CARTESIAN_POINT('Ctrl Pts',(0.151881094022909,-1.,4.01273584234684));
#48669=CARTESIAN_POINT('Ctrl Pts',(0.151881094022909,1.,4.01273584234684));
#48670=CARTESIAN_POINT('Ctrl Pts',(0.154275004872309,-1.,4.00548360245297));
#48671=CARTESIAN_POINT('Ctrl Pts',(0.154275004872309,1.,4.00548360245297));
#48672=CARTESIAN_POINT('Ctrl Pts',(0.156626481393735,-1.,3.99822717425869));
#48673=CARTESIAN_POINT('Ctrl Pts',(0.156626481393735,1.,3.99822717425869));
#48674=CARTESIAN_POINT('Ctrl Pts',(0.158935123982796,-1.,3.99096873945862));
#48675=CARTESIAN_POINT('Ctrl Pts',(0.158935123982796,1.,3.99096873945862));
#48676=CARTESIAN_POINT('Ctrl Pts',(0.161200482186087,-1.,3.98371010319866));
#48677=CARTESIAN_POINT('Ctrl Pts',(0.161200482186087,1.,3.98371010319866));
#48678=CARTESIAN_POINT('Ctrl Pts',(0.163422004609998,-1.,3.97645194630944));
#48679=CARTESIAN_POINT('Ctrl Pts',(0.163422004609998,1.,3.97645194630944));
#48680=CARTESIAN_POINT('Ctrl Pts',(0.165598992851097,-1.,3.9691931362141));
#48681=CARTESIAN_POINT('Ctrl Pts',(0.165598992851097,1.,3.9691931362141));
#48682=CARTESIAN_POINT('Ctrl Pts',(0.167730547023312,-1.,3.96192990160296));
#48683=CARTESIAN_POINT('Ctrl Pts',(0.167730547023312,1.,3.96192990160296));
#48684=CARTESIAN_POINT('Ctrl Pts',(0.16981566637413,-1.,3.95465744665263));
#48685=CARTESIAN_POINT('Ctrl Pts',(0.16981566637413,1.,3.95465744665263));
#48686=CARTESIAN_POINT('Ctrl Pts',(0.171853355369232,-1.,3.94737164900861));
#48687=CARTESIAN_POINT('Ctrl Pts',(0.171853355369232,1.,3.94737164900861));
#48688=CARTESIAN_POINT('Ctrl Pts',(0.173842734974607,-1.,3.94007083096214));
#48689=CARTESIAN_POINT('Ctrl Pts',(0.173842734974607,1.,3.94007083096214));
#48690=CARTESIAN_POINT('Ctrl Pts',(0.175783136893872,-1.,3.93275726771049));
#48691=CARTESIAN_POINT('Ctrl Pts',(0.175783136893872,1.,3.93275726771049));
#48692=CARTESIAN_POINT('Ctrl Pts',(0.177674246152328,-1.,3.92543942697672));
#48693=CARTESIAN_POINT('Ctrl Pts',(0.177674246152328,1.,3.92543942697672));
#48694=CARTESIAN_POINT('Ctrl Pts',(0.179515885822894,-1.,3.91812876180948));
#48695=CARTESIAN_POINT('Ctrl Pts',(0.179515885822894,1.,3.91812876180948));
#48696=CARTESIAN_POINT('Ctrl Pts',(0.181307740731795,-1.,3.91083557557193));
#48697=CARTESIAN_POINT('Ctrl Pts',(0.181307740731795,1.,3.91083557557193));
#48698=CARTESIAN_POINT('Ctrl Pts',(0.183049081993193,-1.,3.90356488555138));
#48699=CARTESIAN_POINT('Ctrl Pts',(0.183049081993193,1.,3.90356488555138));
#48700=CARTESIAN_POINT('Ctrl Pts',(0.184738537728034,-1.,3.89631300742633));
#48701=CARTESIAN_POINT('Ctrl Pts',(0.184738537728034,1.,3.89631300742633));
#48702=CARTESIAN_POINT('Ctrl Pts',(0.186373724985263,-1.,3.88906196725817));
#48703=CARTESIAN_POINT('Ctrl Pts',(0.186373724985263,1.,3.88906196725817));
#48704=CARTESIAN_POINT('Ctrl Pts',(0.187951632512663,-1.,3.88178563496187));
#48705=CARTESIAN_POINT('Ctrl Pts',(0.187951632512663,1.,3.88178563496187));
#48706=CARTESIAN_POINT('Ctrl Pts',(0.189469253358254,-1.,3.87445976418377));
#48707=CARTESIAN_POINT('Ctrl Pts',(0.189469253358254,1.,3.87445976418377));
#48708=CARTESIAN_POINT('Ctrl Pts',(0.190924190418612,-1.,3.8670715862477));
#48709=CARTESIAN_POINT('Ctrl Pts',(0.190924190418612,1.,3.8670715862477));
#48710=CARTESIAN_POINT('Ctrl Pts',(0.192315153044979,-1.,3.85962774407652));
#48711=CARTESIAN_POINT('Ctrl Pts',(0.192315153044979,1.,3.85962774407652));
#48712=CARTESIAN_POINT('Ctrl Pts',(0.193642806777747,-1.,3.85216762264019));
#48713=CARTESIAN_POINT('Ctrl Pts',(0.193642806777747,1.,3.85216762264019));
#48714=CARTESIAN_POINT('Ctrl Pts',(0.194909009460254,-1.,3.84475203347052));
#48715=CARTESIAN_POINT('Ctrl Pts',(0.194909009460254,1.,3.84475203347052));
#48716=CARTESIAN_POINT('Ctrl Pts',(0.196115198971889,-1.,3.83743910616265));
#48717=CARTESIAN_POINT('Ctrl Pts',(0.196115198971889,1.,3.83743910616265));
#48718=CARTESIAN_POINT('Ctrl Pts',(0.197260935827375,-1.,3.83026221776488));
#48719=CARTESIAN_POINT('Ctrl Pts',(0.197260935827375,1.,3.83026221776488));
#48720=CARTESIAN_POINT('Ctrl Pts',(0.198342616900469,-1.,3.82321127348981));
#48721=CARTESIAN_POINT('Ctrl Pts',(0.198342616900469,1.,3.82321127348981));
#48722=CARTESIAN_POINT('Ctrl Pts',(0.199351525297396,-1.,3.81620203429702));
#48723=CARTESIAN_POINT('Ctrl Pts',(0.199351525297396,1.,3.81620203429702));
#48724=CARTESIAN_POINT('Ctrl Pts',(0.200274679433289,-1.,3.80909529318501));
#48725=CARTESIAN_POINT('Ctrl Pts',(0.200274679433289,1.,3.80909529318501));
#48726=CARTESIAN_POINT('Ctrl Pts',(0.201097756307251,-1.,3.80175247447171));
#48727=CARTESIAN_POINT('Ctrl Pts',(0.201097756307251,1.,3.80175247447171));
#48728=CARTESIAN_POINT('Ctrl Pts',(0.201807533800798,-1.,3.79408354187274));
#48729=CARTESIAN_POINT('Ctrl Pts',(0.201807533800798,1.,3.79408354187274));
#48730=CARTESIAN_POINT('Ctrl Pts',(0.202394260512192,-1.,3.78609175019317));
#48731=CARTESIAN_POINT('Ctrl Pts',(0.202394260512192,1.,3.78609175019317));
#48732=CARTESIAN_POINT('Ctrl Pts',(0.202854729699196,-1.,3.77793553476879));
#48733=CARTESIAN_POINT('Ctrl Pts',(0.202854729699196,1.,3.77793553476879));
#48734=CARTESIAN_POINT('Ctrl Pts',(0.203192390045337,-1.,3.76992071595267));
#48735=CARTESIAN_POINT('Ctrl Pts',(0.203192390045337,1.,3.76992071595267));
#48736=CARTESIAN_POINT('Ctrl Pts',(0.203414634707646,-1.,3.76242717937273));
#48737=CARTESIAN_POINT('Ctrl Pts',(0.203414634707646,1.,3.76242717937273));
#48738=CARTESIAN_POINT('Ctrl Pts',(0.203530796848403,-1.,3.75585118707924));
#48739=CARTESIAN_POINT('Ctrl Pts',(0.203530796848403,1.,3.75585118707924));
#48740=CARTESIAN_POINT('Ctrl Pts',(0.203550035479096,-1.,3.75054693397716));
#48741=CARTESIAN_POINT('Ctrl Pts',(0.203550035479096,1.,3.75054693397716));
#48742=CARTESIAN_POINT('Ctrl Pts',(0.203478844530229,-1.,3.74675472018582));
#48743=CARTESIAN_POINT('Ctrl Pts',(0.203478844530229,1.,3.74675472018582));
#48744=CARTESIAN_POINT('Ctrl Pts',(0.203352057956055,-1.,3.7450208092684));
#48745=CARTESIAN_POINT('Ctrl Pts',(0.203352057956055,1.,3.7450208092684));
#48746=CARTESIAN_POINT('Ctrl Pts',(0.203218215747894,-1.,3.74446880195845));
#48747=CARTESIAN_POINT('Ctrl Pts',(0.203218215747894,1.,3.74446880195845));
#48748=CARTESIAN_POINT('Ctrl Pts',(0.20311176758786,-1.,3.74443319346666));
#48749=CARTESIAN_POINT('Ctrl Pts',(0.20311176758786,1.,3.74443319346666));
#48750=CARTESIAN_POINT('Ctrl Pts',(0.203054238699719,-1.,3.74449849461127));
#48751=CARTESIAN_POINT('Ctrl Pts',(0.203054238699719,1.,3.74449849461127));
#48752=CARTESIAN_POINT('',(0.0760622897878233,1.,4.19931119685982));
#48753=CARTESIAN_POINT('Ctrl Pts',(0.0760622897878233,1.,4.19931119685982));
#48754=CARTESIAN_POINT('Ctrl Pts',(0.0767384596142192,1.,4.19789138621624));
#48755=CARTESIAN_POINT('Ctrl Pts',(0.0780873956244399,1.,4.19505112860624));
#48756=CARTESIAN_POINT('Ctrl Pts',(0.08010058871176,1.,4.19078883322483));
#48757=CARTESIAN_POINT('Ctrl Pts',(0.0827644164389507,1.,4.1851019532944));
#48758=CARTESIAN_POINT('Ctrl Pts',(0.0860600915552512,1.,4.17798698669991));
#48759=CARTESIAN_POINT('Ctrl Pts',(0.0893215560850325,1.,4.17086566491823));
#48760=CARTESIAN_POINT('Ctrl Pts',(0.0925486672167687,1.,4.16373802265942));
#48761=CARTESIAN_POINT('Ctrl Pts',(0.0957412403297065,1.,4.15660412653006));
#48762=CARTESIAN_POINT('Ctrl Pts',(0.0988990478899809,1.,4.1494640891762));
#48763=CARTESIAN_POINT('Ctrl Pts',(0.102021826577453,1.,4.14231804938737));
#48764=CARTESIAN_POINT('Ctrl Pts',(0.105109286538864,1.,4.13516614458396));
#48765=CARTESIAN_POINT('Ctrl Pts',(0.10816112052835,1.,4.12800848371386));
#48766=CARTESIAN_POINT('Ctrl Pts',(0.111177012683377,1.,4.12084512502444));
#48767=CARTESIAN_POINT('Ctrl Pts',(0.114156649609601,1.,4.11367603925313));
#48768=CARTESIAN_POINT('Ctrl Pts',(0.117099722731704,1.,4.10650113382187));
#48769=CARTESIAN_POINT('Ctrl Pts',(0.120005924388162,1.,4.09932031767243));
#48770=CARTESIAN_POINT('Ctrl Pts',(0.122874946249119,1.,4.09213355850836));
#48771=CARTESIAN_POINT('Ctrl Pts',(0.125706476822529,1.,4.08494093372315));
#48772=CARTESIAN_POINT('Ctrl Pts',(0.128500200484813,1.,4.07774270738809));
#48773=CARTESIAN_POINT('Ctrl Pts',(0.131255793548914,1.,4.07053931528579));
#48774=CARTESIAN_POINT('Ctrl Pts',(0.133972916144225,1.,4.06333121018476));
#48775=CARTESIAN_POINT('Ctrl Pts',(0.136651205046111,1.,4.05611873400122));
#48776=CARTESIAN_POINT('Ctrl Pts',(0.139290267180059,1.,4.04890199238056));
#48777=CARTESIAN_POINT('Ctrl Pts',(0.141889671485507,1.,4.04168069633842));
#48778=CARTESIAN_POINT('Ctrl Pts',(0.144448947038352,1.,4.03445411510403));
#48779=CARTESIAN_POINT('Ctrl Pts',(0.146967602878998,1.,4.02722143147048));
#48780=CARTESIAN_POINT('Ctrl Pts',(0.149445144968707,1.,4.01998203715588));
#48781=CARTESIAN_POINT('Ctrl Pts',(0.151881094022909,1.,4.01273584234684));
#48782=CARTESIAN_POINT('Ctrl Pts',(0.154275004872309,1.,4.00548360245297));
#48783=CARTESIAN_POINT('Ctrl Pts',(0.156626481393735,1.,3.99822717425869));
#48784=CARTESIAN_POINT('Ctrl Pts',(0.158935123982796,1.,3.99096873945862));
#48785=CARTESIAN_POINT('Ctrl Pts',(0.161200482186087,1.,3.98371010319866));
#48786=CARTESIAN_POINT('Ctrl Pts',(0.163422004609998,1.,3.97645194630944));
#48787=CARTESIAN_POINT('Ctrl Pts',(0.165598992851097,1.,3.9691931362141));
#48788=CARTESIAN_POINT('Ctrl Pts',(0.167730547023312,1.,3.96192990160296));
#48789=CARTESIAN_POINT('Ctrl Pts',(0.16981566637413,1.,3.95465744665263));
#48790=CARTESIAN_POINT('Ctrl Pts',(0.171853355369232,1.,3.94737164900861));
#48791=CARTESIAN_POINT('Ctrl Pts',(0.173842734974607,1.,3.94007083096214));
#48792=CARTESIAN_POINT('Ctrl Pts',(0.175783136893872,1.,3.93275726771049));
#48793=CARTESIAN_POINT('Ctrl Pts',(0.177674246152328,1.,3.92543942697672));
#48794=CARTESIAN_POINT('Ctrl Pts',(0.179515885822894,1.,3.91812876180948));
#48795=CARTESIAN_POINT('Ctrl Pts',(0.181307740731795,1.,3.91083557557193));
#48796=CARTESIAN_POINT('Ctrl Pts',(0.183049081993193,1.,3.90356488555138));
#48797=CARTESIAN_POINT('Ctrl Pts',(0.184738537728034,1.,3.89631300742633));
#48798=CARTESIAN_POINT('Ctrl Pts',(0.186373724985263,1.,3.88906196725817));
#48799=CARTESIAN_POINT('Ctrl Pts',(0.187951632512663,1.,3.88178563496187));
#48800=CARTESIAN_POINT('Ctrl Pts',(0.189469253358254,1.,3.87445976418377));
#48801=CARTESIAN_POINT('Ctrl Pts',(0.190924190418612,1.,3.8670715862477));
#48802=CARTESIAN_POINT('Ctrl Pts',(0.192315153044979,1.,3.85962774407652));
#48803=CARTESIAN_POINT('Ctrl Pts',(0.193642806777747,1.,3.85216762264019));
#48804=CARTESIAN_POINT('Ctrl Pts',(0.194909009460254,1.,3.84475203347052));
#48805=CARTESIAN_POINT('Ctrl Pts',(0.196115198971889,1.,3.83743910616265));
#48806=CARTESIAN_POINT('Ctrl Pts',(0.197260935827375,1.,3.83026221776488));
#48807=CARTESIAN_POINT('Ctrl Pts',(0.198342616900469,1.,3.82321127348981));
#48808=CARTESIAN_POINT('Ctrl Pts',(0.199351525297396,1.,3.81620203429702));
#48809=CARTESIAN_POINT('Ctrl Pts',(0.200274679433289,1.,3.80909529318501));
#48810=CARTESIAN_POINT('Ctrl Pts',(0.201097756307251,1.,3.80175247447171));
#48811=CARTESIAN_POINT('Ctrl Pts',(0.201807533800798,1.,3.79408354187274));
#48812=CARTESIAN_POINT('Ctrl Pts',(0.202394260512192,1.,3.78609175019317));
#48813=CARTESIAN_POINT('Ctrl Pts',(0.202854729699196,1.,3.77793553476879));
#48814=CARTESIAN_POINT('Ctrl Pts',(0.203192390045337,1.,3.76992071595267));
#48815=CARTESIAN_POINT('Ctrl Pts',(0.203414634707646,1.,3.76242717937273));
#48816=CARTESIAN_POINT('Ctrl Pts',(0.203530796848403,1.,3.75585118707924));
#48817=CARTESIAN_POINT('Ctrl Pts',(0.203550035479096,1.,3.75054693397716));
#48818=CARTESIAN_POINT('Ctrl Pts',(0.203484186269314,1.,3.74703926501843));
#48819=CARTESIAN_POINT('Ctrl Pts',(0.203375226874331,1.,3.74535749969262));
#48820=CARTESIAN_POINT('Ctrl Pts',(0.203266610111263,1.,3.74471097893961));
#48821=CARTESIAN_POINT('Ctrl Pts',(0.203188003947964,1.,3.74453008995129));
#48822=CARTESIAN_POINT('Ctrl Pts',(0.203156094897895,1.,3.74449296982994));
#48823=CARTESIAN_POINT('',(0.0760622897878233,0.,4.19931119685982));
#48824=CARTESIAN_POINT('Ctrl Pts',(-0.20305423869972,-1.,3.74449849461127));
#48825=CARTESIAN_POINT('Ctrl Pts',(-0.20305423869972,1.,3.74449849461127));
#48826=CARTESIAN_POINT('Ctrl Pts',(-0.203111767587923,-1.,3.7444331934681));
#48827=CARTESIAN_POINT('Ctrl Pts',(-0.203111767587923,1.,3.7444331934681));
#48828=CARTESIAN_POINT('Ctrl Pts',(-0.203218215748059,-1.,3.7444688019622));
#48829=CARTESIAN_POINT('Ctrl Pts',(-0.203218215748059,1.,3.7444688019622));
#48830=CARTESIAN_POINT('Ctrl Pts',(-0.203352057956297,-1.,3.74502080927395));
#48831=CARTESIAN_POINT('Ctrl Pts',(-0.203352057956297,1.,3.74502080927395));
#48832=CARTESIAN_POINT('Ctrl Pts',(-0.203478844530447,-1.,3.7467547201908));
#48833=CARTESIAN_POINT('Ctrl Pts',(-0.203478844530447,1.,3.7467547201908));
#48834=CARTESIAN_POINT('Ctrl Pts',(-0.203550035479166,-1.,3.75054693397875));
#48835=CARTESIAN_POINT('Ctrl Pts',(-0.203550035479166,1.,3.75054693397875));
#48836=CARTESIAN_POINT('Ctrl Pts',(-0.203530796848322,-1.,3.75585118707734));
#48837=CARTESIAN_POINT('Ctrl Pts',(-0.203530796848322,1.,3.75585118707734));
#48838=CARTESIAN_POINT('Ctrl Pts',(-0.203414634707479,-1.,3.76242717936885));
#48839=CARTESIAN_POINT('Ctrl Pts',(-0.203414634707479,1.,3.76242717936885));
#48840=CARTESIAN_POINT('Ctrl Pts',(-0.203192390045165,-1.,3.7699207159487));
#48841=CARTESIAN_POINT('Ctrl Pts',(-0.203192390045165,1.,3.7699207159487));
#48842=CARTESIAN_POINT('Ctrl Pts',(-0.202854729699081,-1.,3.77793553476614));
#48843=CARTESIAN_POINT('Ctrl Pts',(-0.202854729699081,1.,3.77793553476614));
#48844=CARTESIAN_POINT('Ctrl Pts',(-0.20239426051216,-1.,3.78609175019242));
#48845=CARTESIAN_POINT('Ctrl Pts',(-0.20239426051216,1.,3.78609175019242));
#48846=CARTESIAN_POINT('Ctrl Pts',(-0.201807533800837,-1.,3.7940835418736));
#48847=CARTESIAN_POINT('Ctrl Pts',(-0.201807533800837,1.,3.7940835418736));
#48848=CARTESIAN_POINT('Ctrl Pts',(-0.201097756307326,-1.,3.80175247447337));
#48849=CARTESIAN_POINT('Ctrl Pts',(-0.201097756307326,1.,3.80175247447337));
#48850=CARTESIAN_POINT('Ctrl Pts',(-0.200274679433365,-1.,3.80909529318669));
#48851=CARTESIAN_POINT('Ctrl Pts',(-0.200274679433365,1.,3.80909529318669));
#48852=CARTESIAN_POINT('Ctrl Pts',(-0.199351525297447,-1.,3.81620203429815));
#48853=CARTESIAN_POINT('Ctrl Pts',(-0.199351525297447,1.,3.81620203429815));
#48854=CARTESIAN_POINT('Ctrl Pts',(-0.198342616900487,-1.,3.82321127349016));
#48855=CARTESIAN_POINT('Ctrl Pts',(-0.198342616900487,1.,3.82321127349016));
#48856=CARTESIAN_POINT('Ctrl Pts',(-0.197260935827362,-1.,3.83026221776456));
#48857=CARTESIAN_POINT('Ctrl Pts',(-0.197260935827362,1.,3.83026221776456));
#48858=CARTESIAN_POINT('Ctrl Pts',(-0.196115198971859,-1.,3.83743910616195));
#48859=CARTESIAN_POINT('Ctrl Pts',(-0.196115198971859,1.,3.83743910616195));
#48860=CARTESIAN_POINT('Ctrl Pts',(-0.194909009460221,-1.,3.84475203346977));
#48861=CARTESIAN_POINT('Ctrl Pts',(-0.194909009460221,1.,3.84475203346977));
#48862=CARTESIAN_POINT('Ctrl Pts',(-0.193642806777723,-1.,3.85216762263966));
#48863=CARTESIAN_POINT('Ctrl Pts',(-0.193642806777723,1.,3.85216762263966));
#48864=CARTESIAN_POINT('Ctrl Pts',(-0.192315153044971,-1.,3.85962774407633));
#48865=CARTESIAN_POINT('Ctrl Pts',(-0.192315153044971,1.,3.85962774407633));
#48866=CARTESIAN_POINT('Ctrl Pts',(-0.19092419041862,-1.,3.86707158624783));
#48867=CARTESIAN_POINT('Ctrl Pts',(-0.19092419041862,1.,3.86707158624783));
#48868=CARTESIAN_POINT('Ctrl Pts',(-0.189469253358273,-1.,3.87445976418412));
#48869=CARTESIAN_POINT('Ctrl Pts',(-0.189469253358273,1.,3.87445976418412));
#48870=CARTESIAN_POINT('Ctrl Pts',(-0.187951632512685,-1.,3.88178563496228));
#48871=CARTESIAN_POINT('Ctrl Pts',(-0.187951632512685,1.,3.88178563496228));
#48872=CARTESIAN_POINT('Ctrl Pts',(-0.186373724985281,-1.,3.88906196725848));
#48873=CARTESIAN_POINT('Ctrl Pts',(-0.186373724985281,1.,3.88906196725848));
#48874=CARTESIAN_POINT('Ctrl Pts',(-0.184738537728043,-1.,3.89631300742646));
#48875=CARTESIAN_POINT('Ctrl Pts',(-0.184738537728043,1.,3.89631300742646));
#48876=CARTESIAN_POINT('Ctrl Pts',(-0.183049081993191,-1.,3.90356488555132));
#48877=CARTESIAN_POINT('Ctrl Pts',(-0.183049081993191,1.,3.90356488555132));
#48878=CARTESIAN_POINT('Ctrl Pts',(-0.181307740731786,-1.,3.91083557557175));
#48879=CARTESIAN_POINT('Ctrl Pts',(-0.181307740731786,1.,3.91083557557175));
#48880=CARTESIAN_POINT('Ctrl Pts',(-0.179515885822882,-1.,3.91812876180926));
#48881=CARTESIAN_POINT('Ctrl Pts',(-0.179515885822882,1.,3.91812876180926));
#48882=CARTESIAN_POINT('Ctrl Pts',(-0.177674246152318,-1.,3.92543942697655));
#48883=CARTESIAN_POINT('Ctrl Pts',(-0.177674246152318,1.,3.92543942697655));
#48884=CARTESIAN_POINT('Ctrl Pts',(-0.175783136893868,-1.,3.93275726771042));
#48885=CARTESIAN_POINT('Ctrl Pts',(-0.175783136893868,1.,3.93275726771042));
#48886=CARTESIAN_POINT('Ctrl Pts',(-0.17384273497461,-1.,3.94007083096217));
#48887=CARTESIAN_POINT('Ctrl Pts',(-0.17384273497461,1.,3.94007083096217));
#48888=CARTESIAN_POINT('Ctrl Pts',(-0.17185335536924,-1.,3.94737164900868));
#48889=CARTESIAN_POINT('Ctrl Pts',(-0.17185335536924,1.,3.94737164900868));
#48890=CARTESIAN_POINT('Ctrl Pts',(-0.169815666374139,-1.,3.95465744665268));
#48891=CARTESIAN_POINT('Ctrl Pts',(-0.169815666374139,1.,3.95465744665268));
#48892=CARTESIAN_POINT('Ctrl Pts',(-0.16773054702332,-1.,3.96192990160296));
#48893=CARTESIAN_POINT('Ctrl Pts',(-0.16773054702332,1.,3.96192990160296));
#48894=CARTESIAN_POINT('Ctrl Pts',(-0.165598992851102,-1.,3.96919313621407));
#48895=CARTESIAN_POINT('Ctrl Pts',(-0.165598992851102,1.,3.96919313621407));
#48896=CARTESIAN_POINT('Ctrl Pts',(-0.163422004609999,-1.,3.97645194630943));
#48897=CARTESIAN_POINT('Ctrl Pts',(-0.163422004609999,1.,3.97645194630943));
#48898=CARTESIAN_POINT('Ctrl Pts',(-0.161200482186085,-1.,3.98371010319872));
#48899=CARTESIAN_POINT('Ctrl Pts',(-0.161200482186085,1.,3.98371010319872));
#48900=CARTESIAN_POINT('Ctrl Pts',(-0.158935123982793,-1.,3.99096873945878));
#48901=CARTESIAN_POINT('Ctrl Pts',(-0.158935123982793,1.,3.99096873945878));
#48902=CARTESIAN_POINT('Ctrl Pts',(-0.156626481393734,-1.,3.99822717425893));
#48903=CARTESIAN_POINT('Ctrl Pts',(-0.156626481393734,1.,3.99822717425893));
#48904=CARTESIAN_POINT('Ctrl Pts',(-0.154275004872311,-1.,4.00548360245319));
#48905=CARTESIAN_POINT('Ctrl Pts',(-0.154275004872311,1.,4.00548360245319));
#48906=CARTESIAN_POINT('Ctrl Pts',(-0.151881094022911,-1.,4.01273584234689));
#48907=CARTESIAN_POINT('Ctrl Pts',(-0.151881094022911,1.,4.01273584234689));
#48908=CARTESIAN_POINT('Ctrl Pts',(-0.149445144968707,-1.,4.01998203715564));
#48909=CARTESIAN_POINT('Ctrl Pts',(-0.149445144968707,1.,4.01998203715564));
#48910=CARTESIAN_POINT('Ctrl Pts',(-0.146967602878994,-1.,4.02722143146994));
#48911=CARTESIAN_POINT('Ctrl Pts',(-0.146967602878994,1.,4.02722143146994));
#48912=CARTESIAN_POINT('Ctrl Pts',(-0.144448947038345,-1.,4.03445411510333));
#48913=CARTESIAN_POINT('Ctrl Pts',(-0.144448947038345,1.,4.03445411510333));
#48914=CARTESIAN_POINT('Ctrl Pts',(-0.1418896714855,-1.,4.04168069633781));
#48915=CARTESIAN_POINT('Ctrl Pts',(-0.1418896714855,1.,4.04168069633781));
#48916=CARTESIAN_POINT('Ctrl Pts',(-0.139290267180057,-1.,4.04890199238036));
#48917=CARTESIAN_POINT('Ctrl Pts',(-0.139290267180057,1.,4.04890199238036));
#48918=CARTESIAN_POINT('Ctrl Pts',(-0.136651205046119,-1.,4.05611873400172));
#48919=CARTESIAN_POINT('Ctrl Pts',(-0.136651205046119,1.,4.05611873400172));
#48920=CARTESIAN_POINT('Ctrl Pts',(-0.133972916144245,-1.,4.06333121018596));
#48921=CARTESIAN_POINT('Ctrl Pts',(-0.133972916144245,1.,4.06333121018596));
#48922=CARTESIAN_POINT('Ctrl Pts',(-0.131255793548941,-1.,4.0705393152874));
#48923=CARTESIAN_POINT('Ctrl Pts',(-0.131255793548941,1.,4.0705393152874));
#48924=CARTESIAN_POINT('Ctrl Pts',(-0.128500200484838,-1.,4.07774270738954));
#48925=CARTESIAN_POINT('Ctrl Pts',(-0.128500200484838,1.,4.07774270738954));
#48926=CARTESIAN_POINT('Ctrl Pts',(-0.12570647682254,-1.,4.08494093372377));
#48927=CARTESIAN_POINT('Ctrl Pts',(-0.12570647682254,1.,4.08494093372377));
#48928=CARTESIAN_POINT('Ctrl Pts',(-0.122874946249107,-1.,4.09213355850756));
#48929=CARTESIAN_POINT('Ctrl Pts',(-0.122874946249107,1.,4.09213355850756));
#48930=CARTESIAN_POINT('Ctrl Pts',(-0.120005924388124,-1.,4.09932031767002));
#48931=CARTESIAN_POINT('Ctrl Pts',(-0.120005924388124,1.,4.09932031767002));
#48932=CARTESIAN_POINT('Ctrl Pts',(-0.117099722731648,-1.,4.10650113381833));
#48933=CARTESIAN_POINT('Ctrl Pts',(-0.117099722731648,1.,4.10650113381833));
#48934=CARTESIAN_POINT('Ctrl Pts',(-0.114156649609546,-1.,4.11367603924961));
#48935=CARTESIAN_POINT('Ctrl Pts',(-0.114156649609546,1.,4.11367603924961));
#48936=CARTESIAN_POINT('Ctrl Pts',(-0.111177012683347,-1.,4.1208451250225));
#48937=CARTESIAN_POINT('Ctrl Pts',(-0.111177012683347,1.,4.1208451250225));
#48938=CARTESIAN_POINT('Ctrl Pts',(-0.10816112052837,-1.,4.12800848371504));
#48939=CARTESIAN_POINT('Ctrl Pts',(-0.10816112052837,1.,4.12800848371504));
#48940=CARTESIAN_POINT('Ctrl Pts',(-0.105109286538945,-1.,4.13516614458895));
#48941=CARTESIAN_POINT('Ctrl Pts',(-0.105109286538945,1.,4.13516614458895));
#48942=CARTESIAN_POINT('Ctrl Pts',(-0.102021826577584,-1.,4.14231804939538));
#48943=CARTESIAN_POINT('Ctrl Pts',(-0.102021826577584,1.,4.14231804939538));
#48944=CARTESIAN_POINT('Ctrl Pts',(-0.0988990478901228,-1.,4.14946408918485));
#48945=CARTESIAN_POINT('Ctrl Pts',(-0.0988990478901228,1.,4.14946408918485));
#48946=CARTESIAN_POINT('Ctrl Pts',(-0.0957412403298009,-1.,4.15660412653577));
#48947=CARTESIAN_POINT('Ctrl Pts',(-0.0957412403298009,1.,4.15660412653577));
#48948=CARTESIAN_POINT('Ctrl Pts',(-0.0925486672167534,-1.,4.16373802265839));
#48949=CARTESIAN_POINT('Ctrl Pts',(-0.0925486672167534,1.,4.16373802265839));
#48950=CARTESIAN_POINT('Ctrl Pts',(-0.0893215560848652,-1.,4.17086566490794));
#48951=CARTESIAN_POINT('Ctrl Pts',(-0.0893215560848652,1.,4.17086566490794));
#48952=CARTESIAN_POINT('Ctrl Pts',(-0.0860600915549399,-1.,4.17798698668094));
#48953=CARTESIAN_POINT('Ctrl Pts',(-0.0860600915549399,1.,4.17798698668094));
#48954=CARTESIAN_POINT('Ctrl Pts',(-0.0827644164385681,-1.,4.18510195327123));
#48955=CARTESIAN_POINT('Ctrl Pts',(-0.0827644164385681,1.,4.18510195327123));
#48956=CARTESIAN_POINT('Ctrl Pts',(-0.0801005887114322,-1.,4.19078883320504));
#48957=CARTESIAN_POINT('Ctrl Pts',(-0.0801005887114322,1.,4.19078883320504));
#48958=CARTESIAN_POINT('Ctrl Pts',(-0.07808739562424,-1.,4.19505112859416));
#48959=CARTESIAN_POINT('Ctrl Pts',(-0.07808739562424,1.,4.19505112859416));
#48960=CARTESIAN_POINT('Ctrl Pts',(-0.0767384596141467,-1.,4.1978913862118));
#48961=CARTESIAN_POINT('Ctrl Pts',(-0.0767384596141467,1.,4.1978913862118));
#48962=CARTESIAN_POINT('Ctrl Pts',(-0.0760622897878249,-1.,4.19931119685982));
#48963=CARTESIAN_POINT('Ctrl Pts',(-0.0760622897878249,1.,4.19931119685982));
#48964=CARTESIAN_POINT('',(-0.203156094896102,1.,3.74449296983004));
#48965=CARTESIAN_POINT('Ctrl Pts',(-0.203156094896101,-1.,3.74449296983004));
#48966=CARTESIAN_POINT('Ctrl Pts',(-0.203156094896101,-0.666666666666667,
3.74449296983004));
#48967=CARTESIAN_POINT('Ctrl Pts',(-0.203156094896101,-0.333333333333333,
3.74449296983004));
#48968=CARTESIAN_POINT('Ctrl Pts',(-0.203156094896101,0.333333333333333,
3.74449296983004));
#48969=CARTESIAN_POINT('Ctrl Pts',(-0.203156094896101,0.666666666666667,
3.74449296983004));
#48970=CARTESIAN_POINT('Ctrl Pts',(-0.203156094896101,1.,3.74449296983004));
#48971=CARTESIAN_POINT('',(-0.0760622897878249,1.,4.19931119685982));
#48972=CARTESIAN_POINT('',(-0.0760622897878249,0.,4.19931119685982));
#48973=CARTESIAN_POINT('Ctrl Pts',(-0.203156094896101,1.,3.74449296983004));
#48974=CARTESIAN_POINT('Ctrl Pts',(-0.203188003946657,1.,3.74453008995092));
#48975=CARTESIAN_POINT('Ctrl Pts',(-0.203266610110531,1.,3.74471097893845));
#48976=CARTESIAN_POINT('Ctrl Pts',(-0.203375226874122,1.,3.74535749969115));
#48977=CARTESIAN_POINT('Ctrl Pts',(-0.203484186269415,1.,3.74703926501752));
#48978=CARTESIAN_POINT('Ctrl Pts',(-0.203550035479166,1.,3.75054693397875));
#48979=CARTESIAN_POINT('Ctrl Pts',(-0.203530796848322,1.,3.75585118707734));
#48980=CARTESIAN_POINT('Ctrl Pts',(-0.203414634707479,1.,3.76242717936885));
#48981=CARTESIAN_POINT('Ctrl Pts',(-0.203192390045165,1.,3.7699207159487));
#48982=CARTESIAN_POINT('Ctrl Pts',(-0.202854729699081,1.,3.77793553476614));
#48983=CARTESIAN_POINT('Ctrl Pts',(-0.20239426051216,1.,3.78609175019242));
#48984=CARTESIAN_POINT('Ctrl Pts',(-0.201807533800837,1.,3.7940835418736));
#48985=CARTESIAN_POINT('Ctrl Pts',(-0.201097756307326,1.,3.80175247447337));
#48986=CARTESIAN_POINT('Ctrl Pts',(-0.200274679433365,1.,3.80909529318669));
#48987=CARTESIAN_POINT('Ctrl Pts',(-0.199351525297447,1.,3.81620203429815));
#48988=CARTESIAN_POINT('Ctrl Pts',(-0.198342616900487,1.,3.82321127349016));
#48989=CARTESIAN_POINT('Ctrl Pts',(-0.197260935827362,1.,3.83026221776456));
#48990=CARTESIAN_POINT('Ctrl Pts',(-0.196115198971859,1.,3.83743910616195));
#48991=CARTESIAN_POINT('Ctrl Pts',(-0.194909009460221,1.,3.84475203346977));
#48992=CARTESIAN_POINT('Ctrl Pts',(-0.193642806777723,1.,3.85216762263966));
#48993=CARTESIAN_POINT('Ctrl Pts',(-0.192315153044971,1.,3.85962774407633));
#48994=CARTESIAN_POINT('Ctrl Pts',(-0.19092419041862,1.,3.86707158624783));
#48995=CARTESIAN_POINT('Ctrl Pts',(-0.189469253358273,1.,3.87445976418412));
#48996=CARTESIAN_POINT('Ctrl Pts',(-0.187951632512685,1.,3.88178563496228));
#48997=CARTESIAN_POINT('Ctrl Pts',(-0.186373724985281,1.,3.88906196725848));
#48998=CARTESIAN_POINT('Ctrl Pts',(-0.184738537728043,1.,3.89631300742646));
#48999=CARTESIAN_POINT('Ctrl Pts',(-0.183049081993191,1.,3.90356488555132));
#49000=CARTESIAN_POINT('Ctrl Pts',(-0.181307740731786,1.,3.91083557557175));
#49001=CARTESIAN_POINT('Ctrl Pts',(-0.179515885822882,1.,3.91812876180926));
#49002=CARTESIAN_POINT('Ctrl Pts',(-0.177674246152318,1.,3.92543942697655));
#49003=CARTESIAN_POINT('Ctrl Pts',(-0.175783136893868,1.,3.93275726771042));
#49004=CARTESIAN_POINT('Ctrl Pts',(-0.17384273497461,1.,3.94007083096217));
#49005=CARTESIAN_POINT('Ctrl Pts',(-0.17185335536924,1.,3.94737164900868));
#49006=CARTESIAN_POINT('Ctrl Pts',(-0.169815666374139,1.,3.95465744665268));
#49007=CARTESIAN_POINT('Ctrl Pts',(-0.16773054702332,1.,3.96192990160296));
#49008=CARTESIAN_POINT('Ctrl Pts',(-0.165598992851102,1.,3.96919313621407));
#49009=CARTESIAN_POINT('Ctrl Pts',(-0.163422004609999,1.,3.97645194630943));
#49010=CARTESIAN_POINT('Ctrl Pts',(-0.161200482186085,1.,3.98371010319872));
#49011=CARTESIAN_POINT('Ctrl Pts',(-0.158935123982793,1.,3.99096873945878));
#49012=CARTESIAN_POINT('Ctrl Pts',(-0.156626481393734,1.,3.99822717425893));
#49013=CARTESIAN_POINT('Ctrl Pts',(-0.154275004872311,1.,4.00548360245319));
#49014=CARTESIAN_POINT('Ctrl Pts',(-0.151881094022911,1.,4.01273584234689));
#49015=CARTESIAN_POINT('Ctrl Pts',(-0.149445144968707,1.,4.01998203715564));
#49016=CARTESIAN_POINT('Ctrl Pts',(-0.146967602878994,1.,4.02722143146994));
#49017=CARTESIAN_POINT('Ctrl Pts',(-0.144448947038345,1.,4.03445411510333));
#49018=CARTESIAN_POINT('Ctrl Pts',(-0.1418896714855,1.,4.04168069633781));
#49019=CARTESIAN_POINT('Ctrl Pts',(-0.139290267180057,1.,4.04890199238036));
#49020=CARTESIAN_POINT('Ctrl Pts',(-0.136651205046119,1.,4.05611873400172));
#49021=CARTESIAN_POINT('Ctrl Pts',(-0.133972916144245,1.,4.06333121018596));
#49022=CARTESIAN_POINT('Ctrl Pts',(-0.131255793548941,1.,4.0705393152874));
#49023=CARTESIAN_POINT('Ctrl Pts',(-0.128500200484838,1.,4.07774270738954));
#49024=CARTESIAN_POINT('Ctrl Pts',(-0.12570647682254,1.,4.08494093372377));
#49025=CARTESIAN_POINT('Ctrl Pts',(-0.122874946249107,1.,4.09213355850756));
#49026=CARTESIAN_POINT('Ctrl Pts',(-0.120005924388124,1.,4.09932031767002));
#49027=CARTESIAN_POINT('Ctrl Pts',(-0.117099722731648,1.,4.10650113381833));
#49028=CARTESIAN_POINT('Ctrl Pts',(-0.114156649609546,1.,4.11367603924961));
#49029=CARTESIAN_POINT('Ctrl Pts',(-0.111177012683347,1.,4.1208451250225));
#49030=CARTESIAN_POINT('Ctrl Pts',(-0.10816112052837,1.,4.12800848371504));
#49031=CARTESIAN_POINT('Ctrl Pts',(-0.105109286538945,1.,4.13516614458895));
#49032=CARTESIAN_POINT('Ctrl Pts',(-0.102021826577584,1.,4.14231804939538));
#49033=CARTESIAN_POINT('Ctrl Pts',(-0.0988990478901228,1.,4.14946408918485));
#49034=CARTESIAN_POINT('Ctrl Pts',(-0.0957412403298009,1.,4.15660412653577));
#49035=CARTESIAN_POINT('Ctrl Pts',(-0.0925486672167534,1.,4.16373802265839));
#49036=CARTESIAN_POINT('Ctrl Pts',(-0.0893215560848652,1.,4.17086566490794));
#49037=CARTESIAN_POINT('Ctrl Pts',(-0.0860600915549399,1.,4.17798698668094));
#49038=CARTESIAN_POINT('Ctrl Pts',(-0.0827644164385681,1.,4.18510195327123));
#49039=CARTESIAN_POINT('Ctrl Pts',(-0.0801005887114322,1.,4.19078883320504));
#49040=CARTESIAN_POINT('Ctrl Pts',(-0.07808739562424,1.,4.19505112859416));
#49041=CARTESIAN_POINT('Ctrl Pts',(-0.0767384596141467,1.,4.1978913862118));
#49042=CARTESIAN_POINT('Ctrl Pts',(-0.0760622897878249,1.,4.19931119685982));
#49043=CARTESIAN_POINT('Origin',(-0.0760622897878249,0.,4.19931119685982));
#49044=CARTESIAN_POINT('',(0.0760622897878233,1.,4.19931119685982));
#49045=CARTESIAN_POINT('Origin',(0.,0.,0.));
#49046=CARTESIAN_POINT('',(-0.385112848330762,1.,3.73017266276651));
#49047=CARTESIAN_POINT('Origin',(0.,1.,0.));
#49048=CARTESIAN_POINT('Ctrl Pts',(-0.385112848330762,1.,3.73017266276651));
#49049=CARTESIAN_POINT('Ctrl Pts',(-0.385112848330762,0.666666666666667,
3.73017266276651));
#49050=CARTESIAN_POINT('Ctrl Pts',(-0.385112848330762,0.333333333333333,
3.73017266276651));
#49051=CARTESIAN_POINT('Ctrl Pts',(-0.385112848330762,-0.333333333333333,
3.73017266276651));
#49052=CARTESIAN_POINT('Ctrl Pts',(-0.385112848330762,-0.666666666666667,
3.73017266276651));
#49053=CARTESIAN_POINT('Ctrl Pts',(-0.385112848330762,-1.,3.73017266276651));
#49054=CARTESIAN_POINT('Ctrl Pts',(-0.581791163835815,-1.,4.15950947128175));
#49055=CARTESIAN_POINT('Ctrl Pts',(-0.581791163835815,1.,4.15950947128175));
#49056=CARTESIAN_POINT('Ctrl Pts',(-0.580901211463535,-1.,4.1582129171283));
#49057=CARTESIAN_POINT('Ctrl Pts',(-0.580901211463535,1.,4.1582129171283));
#49058=CARTESIAN_POINT('Ctrl Pts',(-0.579124568914235,-1.,4.15561864788576));
#49059=CARTESIAN_POINT('Ctrl Pts',(-0.579124568914235,1.,4.15561864788576));
#49060=CARTESIAN_POINT('Ctrl Pts',(-0.576469391676688,-1.,4.151723761217));
#49061=CARTESIAN_POINT('Ctrl Pts',(-0.576469391676688,1.,4.151723761217));
#49062=CARTESIAN_POINT('Ctrl Pts',(-0.572948736069522,-1.,4.14652361068081));
#49063=CARTESIAN_POINT('Ctrl Pts',(-0.572948736069522,1.,4.14652361068081));
#49064=CARTESIAN_POINT('Ctrl Pts',(-0.568580610189775,-1.,4.14001179830547));
#49065=CARTESIAN_POINT('Ctrl Pts',(-0.568580610189775,1.,4.14001179830547));
#49066=CARTESIAN_POINT('Ctrl Pts',(-0.564245279537149,-1.,4.13348835727104));
#49067=CARTESIAN_POINT('Ctrl Pts',(-0.564245279537149,1.,4.13348835727104));
#49068=CARTESIAN_POINT('Ctrl Pts',(-0.559942890594774,-1.,4.12695329951961));
#49069=CARTESIAN_POINT('Ctrl Pts',(-0.559942890594774,1.,4.12695329951961));
#49070=CARTESIAN_POINT('Ctrl Pts',(-0.555673636129977,-1.,4.12040666195664));
#49071=CARTESIAN_POINT('Ctrl Pts',(-0.555673636129977,1.,4.12040666195664));
#49072=CARTESIAN_POINT('Ctrl Pts',(-0.551437758497033,-1.,4.11384852024721));
#49073=CARTESIAN_POINT('Ctrl Pts',(-0.551437758497033,1.,4.11384852024721));
#49074=CARTESIAN_POINT('Ctrl Pts',(-0.547235539485637,-1.,4.10727897027977));
#49075=CARTESIAN_POINT('Ctrl Pts',(-0.547235539485637,1.,4.10727897027977));
#49076=CARTESIAN_POINT('Ctrl Pts',(-0.543067286877757,-1.,4.10069810243979));
#49077=CARTESIAN_POINT('Ctrl Pts',(-0.543067286877757,1.,4.10069810243979));
#49078=CARTESIAN_POINT('Ctrl Pts',(-0.538933321179756,-1.,4.09410597627));
#49079=CARTESIAN_POINT('Ctrl Pts',(-0.538933321179756,1.,4.09410597627));
#49080=CARTESIAN_POINT('Ctrl Pts',(-0.534833963477273,-1.,4.08750259988885));
#49081=CARTESIAN_POINT('Ctrl Pts',(-0.534833963477273,1.,4.08750259988885));
#49082=CARTESIAN_POINT('Ctrl Pts',(-0.530769518728571,-1.,4.08088789536836));
#49083=CARTESIAN_POINT('Ctrl Pts',(-0.530769518728571,1.,4.08088789536836));
#49084=CARTESIAN_POINT('Ctrl Pts',(-0.526740277227498,-1.,4.07426172299847));
#49085=CARTESIAN_POINT('Ctrl Pts',(-0.526740277227498,1.,4.07426172299847));
#49086=CARTESIAN_POINT('Ctrl Pts',(-0.522746528603107,-1.,4.06762394471314));
#49087=CARTESIAN_POINT('Ctrl Pts',(-0.522746528603107,1.,4.06762394471314));
#49088=CARTESIAN_POINT('Ctrl Pts',(-0.518788572336924,-1.,4.06097448038013));
#49089=CARTESIAN_POINT('Ctrl Pts',(-0.518788572336924,1.,4.06097448038013));
#49090=CARTESIAN_POINT('Ctrl Pts',(-0.514866728193017,-1.,4.05431335771199));
#49091=CARTESIAN_POINT('Ctrl Pts',(-0.514866728193017,1.,4.05431335771199));
#49092=CARTESIAN_POINT('Ctrl Pts',(-0.51098134921897,-1.,4.04764078815447));
#49093=CARTESIAN_POINT('Ctrl Pts',(-0.51098134921897,1.,4.04764078815447));
#49094=CARTESIAN_POINT('Ctrl Pts',(-0.507132823288136,-1.,4.04095715148915));
#49095=CARTESIAN_POINT('Ctrl Pts',(-0.507132823288136,1.,4.04095715148915));
#49096=CARTESIAN_POINT('Ctrl Pts',(-0.503321556915346,-1.,4.03426284174272));
#49097=CARTESIAN_POINT('Ctrl Pts',(-0.503321556915346,1.,4.03426284174272));
#49098=CARTESIAN_POINT('Ctrl Pts',(-0.499547962340821,-1.,4.02755813980101));
#49099=CARTESIAN_POINT('Ctrl Pts',(-0.499547962340821,1.,4.02755813980101));
#49100=CARTESIAN_POINT('Ctrl Pts',(-0.495812444326251,-1.,4.02084308851832));
#49101=CARTESIAN_POINT('Ctrl Pts',(-0.495812444326251,1.,4.02084308851832));
#49102=CARTESIAN_POINT('Ctrl Pts',(-0.492115383418018,-1.,4.01411733503546));
#49103=CARTESIAN_POINT('Ctrl Pts',(-0.492115383418018,1.,4.01411733503546));
#49104=CARTESIAN_POINT('Ctrl Pts',(-0.488457130424633,-1.,4.0073800839099));
#49105=CARTESIAN_POINT('Ctrl Pts',(-0.488457130424633,1.,4.0073800839099));
#49106=CARTESIAN_POINT('Ctrl Pts',(-0.484838042421835,-1.,4.00063045119288));
#49107=CARTESIAN_POINT('Ctrl Pts',(-0.484838042421835,1.,4.00063045119288));
#49108=CARTESIAN_POINT('Ctrl Pts',(-0.481258512209675,-1.,3.99386775880679));
#49109=CARTESIAN_POINT('Ctrl Pts',(-0.481258512209675,1.,3.99386775880679));
#49110=CARTESIAN_POINT('Ctrl Pts',(-0.477718999122027,-1.,3.98709184306738));
#49111=CARTESIAN_POINT('Ctrl Pts',(-0.477718999122027,1.,3.98709184306738));
#49112=CARTESIAN_POINT('Ctrl Pts',(-0.47422006101951,-1.,3.98030338044409));
#49113=CARTESIAN_POINT('Ctrl Pts',(-0.47422006101951,1.,3.98030338044409));
#49114=CARTESIAN_POINT('Ctrl Pts',(-0.470762379613439,-1.,3.97350414289392));
#49115=CARTESIAN_POINT('Ctrl Pts',(-0.470762379613439,1.,3.97350414289392));
#49116=CARTESIAN_POINT('Ctrl Pts',(-0.467346690880643,-1.,3.9666962227393));
#49117=CARTESIAN_POINT('Ctrl Pts',(-0.467346690880643,1.,3.9666962227393));
#49118=CARTESIAN_POINT('Ctrl Pts',(-0.463973722115733,-1.,3.95988133243538));
#49119=CARTESIAN_POINT('Ctrl Pts',(-0.463973722115733,1.,3.95988133243538));
#49120=CARTESIAN_POINT('Ctrl Pts',(-0.460644124429121,-1.,3.95306005817364));
#49121=CARTESIAN_POINT('Ctrl Pts',(-0.460644124429121,1.,3.95306005817364));
#49122=CARTESIAN_POINT('Ctrl Pts',(-0.457358410451683,-1.,3.94623117206678));
#49123=CARTESIAN_POINT('Ctrl Pts',(-0.457358410451683,1.,3.94623117206678));
#49124=CARTESIAN_POINT('Ctrl Pts',(-0.454116879027584,-1.,3.93939080846298));
#49125=CARTESIAN_POINT('Ctrl Pts',(-0.454116879027584,1.,3.93939080846298));
#49126=CARTESIAN_POINT('Ctrl Pts',(-0.450919768356348,-1.,3.93253407403123));
#49127=CARTESIAN_POINT('Ctrl Pts',(-0.450919768356348,1.,3.93253407403123));
#49128=CARTESIAN_POINT('Ctrl Pts',(-0.447767416837293,-1.,3.92565674143416));
#49129=CARTESIAN_POINT('Ctrl Pts',(-0.447767416837293,1.,3.92565674143416));
#49130=CARTESIAN_POINT('Ctrl Pts',(-0.444660430230591,-1.,3.91875701610719));
#49131=CARTESIAN_POINT('Ctrl Pts',(-0.444660430230591,1.,3.91875701610719));
#49132=CARTESIAN_POINT('Ctrl Pts',(-0.441599824524054,-1.,3.91183704069153));
#49133=CARTESIAN_POINT('Ctrl Pts',(-0.441599824524054,1.,3.91183704069153));
#49134=CARTESIAN_POINT('Ctrl Pts',(-0.43858723545825,-1.,3.90490512938563));
#49135=CARTESIAN_POINT('Ctrl Pts',(-0.43858723545825,1.,3.90490512938563));
#49136=CARTESIAN_POINT('Ctrl Pts',(-0.435624629433528,-1.,3.89797256655462));
#49137=CARTESIAN_POINT('Ctrl Pts',(-0.435624629433528,1.,3.89797256655462));
#49138=CARTESIAN_POINT('Ctrl Pts',(-0.432713929544458,-1.,3.89104947940611));
#49139=CARTESIAN_POINT('Ctrl Pts',(-0.432713929544458,1.,3.89104947940611));
#49140=CARTESIAN_POINT('Ctrl Pts',(-0.429856640579741,-1.,3.88414070943341));
#49141=CARTESIAN_POINT('Ctrl Pts',(-0.429856640579741,1.,3.88414070943341));
#49142=CARTESIAN_POINT('Ctrl Pts',(-0.427053541173457,-1.,3.87724240306597));
#49143=CARTESIAN_POINT('Ctrl Pts',(-0.427053541173457,1.,3.87724240306597));
#49144=CARTESIAN_POINT('Ctrl Pts',(-0.424304173195111,-1.,3.87033643487851));
#49145=CARTESIAN_POINT('Ctrl Pts',(-0.424304173195111,1.,3.87033643487851));
#49146=CARTESIAN_POINT('Ctrl Pts',(-0.421607423177534,-1.,3.86339652542709));
#49147=CARTESIAN_POINT('Ctrl Pts',(-0.421607423177534,1.,3.86339652542709));
#49148=CARTESIAN_POINT('Ctrl Pts',(-0.418962468086773,-1.,3.85639825647996));
#49149=CARTESIAN_POINT('Ctrl Pts',(-0.418962468086773,1.,3.85639825647996));
#49150=CARTESIAN_POINT('Ctrl Pts',(-0.416369678052907,-1.,3.84932864157497));
#49151=CARTESIAN_POINT('Ctrl Pts',(-0.416369678052907,1.,3.84932864157497));
#49152=CARTESIAN_POINT('Ctrl Pts',(-0.413831367016748,-1.,3.84219403994762));
#49153=CARTESIAN_POINT('Ctrl Pts',(-0.413831367016748,1.,3.84219403994762));
#49154=CARTESIAN_POINT('Ctrl Pts',(-0.411353038798519,-1.,3.83503345578698));
#49155=CARTESIAN_POINT('Ctrl Pts',(-0.411353038798519,1.,3.83503345578698));
#49156=CARTESIAN_POINT('Ctrl Pts',(-0.40894237144746,-1.,3.82790724256471));
#49157=CARTESIAN_POINT('Ctrl Pts',(-0.40894237144746,1.,3.82790724256471));
#49158=CARTESIAN_POINT('Ctrl Pts',(-0.406607038258985,-1.,3.8208730391381));
#49159=CARTESIAN_POINT('Ctrl Pts',(-0.406607038258985,1.,3.8208730391381));
#49160=CARTESIAN_POINT('Ctrl Pts',(-0.404352694628273,-1.,3.81396374287793));
#49161=CARTESIAN_POINT('Ctrl Pts',(-0.404352694628273,1.,3.81396374287793));
#49162=CARTESIAN_POINT('Ctrl Pts',(-0.402181320148436,-1.,3.80716881962728));
#49163=CARTESIAN_POINT('Ctrl Pts',(-0.402181320148436,1.,3.80716881962728));
#49164=CARTESIAN_POINT('Ctrl Pts',(-0.4000883465046,-1.,3.80040370384546));
#49165=CARTESIAN_POINT('Ctrl Pts',(-0.4000883465046,1.,3.80040370384546));
#49166=CARTESIAN_POINT('Ctrl Pts',(-0.39806481868397,-1.,3.7935288716329));
#49167=CARTESIAN_POINT('Ctrl Pts',(-0.39806481868397,1.,3.7935288716329));
#49168=CARTESIAN_POINT('Ctrl Pts',(-0.396103205334841,-1.,3.78640521279313));
#49169=CARTESIAN_POINT('Ctrl Pts',(-0.396103205334841,1.,3.78640521279313));
#49170=CARTESIAN_POINT('Ctrl Pts',(-0.394202481011499,-1.,3.77894173114283));
#49171=CARTESIAN_POINT('Ctrl Pts',(-0.394202481011499,1.,3.77894173114283));
#49172=CARTESIAN_POINT('Ctrl Pts',(-0.392372786223433,-1.,3.77114011595967));
#49173=CARTESIAN_POINT('Ctrl Pts',(-0.392372786223433,1.,3.77114011595967));
#49174=CARTESIAN_POINT('Ctrl Pts',(-0.39064207297956,-1.,3.76315635033257));
#49175=CARTESIAN_POINT('Ctrl Pts',(-0.39064207297956,1.,3.76315635033257));
#49176=CARTESIAN_POINT('Ctrl Pts',(-0.389054775898702,-1.,3.75529302895152));
#49177=CARTESIAN_POINT('Ctrl Pts',(-0.389054775898702,1.,3.75529302895152));
#49178=CARTESIAN_POINT('Ctrl Pts',(-0.387663020050836,-1.,3.74792651696654));
#49179=CARTESIAN_POINT('Ctrl Pts',(-0.387663020050836,1.,3.74792651696654));
#49180=CARTESIAN_POINT('Ctrl Pts',(-0.386519576222251,-1.,3.74144965781276));
#49181=CARTESIAN_POINT('Ctrl Pts',(-0.386519576222251,1.,3.74144965781276));
#49182=CARTESIAN_POINT('Ctrl Pts',(-0.385670806454566,-1.,3.73621371845318));
#49183=CARTESIAN_POINT('Ctrl Pts',(-0.385670806454566,1.,3.73621371845318));
#49184=CARTESIAN_POINT('Ctrl Pts',(-0.385147887988951,-1.,3.73245705638843));
#49185=CARTESIAN_POINT('Ctrl Pts',(-0.385147887988951,1.,3.73245705638843));
#49186=CARTESIAN_POINT('Ctrl Pts',(-0.385001870183213,-1.,3.73072465900175));
#49187=CARTESIAN_POINT('Ctrl Pts',(-0.385001870183213,1.,3.73072465900175));
#49188=CARTESIAN_POINT('Ctrl Pts',(-0.385047711603462,-1.,3.73015851028356));
#49189=CARTESIAN_POINT('Ctrl Pts',(-0.385047711603462,1.,3.73015851028356));
#49190=CARTESIAN_POINT('Ctrl Pts',(-0.385147278814642,-1.,3.73010668803042));
#49191=CARTESIAN_POINT('Ctrl Pts',(-0.385147278814642,1.,3.73010668803042));
#49192=CARTESIAN_POINT('Ctrl Pts',(-0.38521431477633,-1.,3.73016218570874));
#49193=CARTESIAN_POINT('Ctrl Pts',(-0.38521431477633,1.,3.73016218570874));
#49194=CARTESIAN_POINT('',(-0.581791163835815,1.,4.15950947128175));
#49195=CARTESIAN_POINT('Ctrl Pts',(-0.581791163835815,1.,4.15950947128175));
#49196=CARTESIAN_POINT('Ctrl Pts',(-0.580901211463535,1.,4.1582129171283));
#49197=CARTESIAN_POINT('Ctrl Pts',(-0.579124568914235,1.,4.15561864788576));
#49198=CARTESIAN_POINT('Ctrl Pts',(-0.576469391676688,1.,4.151723761217));
#49199=CARTESIAN_POINT('Ctrl Pts',(-0.572948736069522,1.,4.14652361068081));
#49200=CARTESIAN_POINT('Ctrl Pts',(-0.568580610189775,1.,4.14001179830547));
#49201=CARTESIAN_POINT('Ctrl Pts',(-0.564245279537149,1.,4.13348835727104));
#49202=CARTESIAN_POINT('Ctrl Pts',(-0.559942890594774,1.,4.12695329951961));
#49203=CARTESIAN_POINT('Ctrl Pts',(-0.555673636129977,1.,4.12040666195664));
#49204=CARTESIAN_POINT('Ctrl Pts',(-0.551437758497033,1.,4.11384852024721));
#49205=CARTESIAN_POINT('Ctrl Pts',(-0.547235539485637,1.,4.10727897027977));
#49206=CARTESIAN_POINT('Ctrl Pts',(-0.543067286877757,1.,4.10069810243979));
#49207=CARTESIAN_POINT('Ctrl Pts',(-0.538933321179756,1.,4.09410597627));
#49208=CARTESIAN_POINT('Ctrl Pts',(-0.534833963477273,1.,4.08750259988885));
#49209=CARTESIAN_POINT('Ctrl Pts',(-0.530769518728571,1.,4.08088789536836));
#49210=CARTESIAN_POINT('Ctrl Pts',(-0.526740277227498,1.,4.07426172299847));
#49211=CARTESIAN_POINT('Ctrl Pts',(-0.522746528603107,1.,4.06762394471314));
#49212=CARTESIAN_POINT('Ctrl Pts',(-0.518788572336924,1.,4.06097448038013));
#49213=CARTESIAN_POINT('Ctrl Pts',(-0.514866728193017,1.,4.05431335771199));
#49214=CARTESIAN_POINT('Ctrl Pts',(-0.51098134921897,1.,4.04764078815447));
#49215=CARTESIAN_POINT('Ctrl Pts',(-0.507132823288136,1.,4.04095715148915));
#49216=CARTESIAN_POINT('Ctrl Pts',(-0.503321556915346,1.,4.03426284174272));
#49217=CARTESIAN_POINT('Ctrl Pts',(-0.499547962340821,1.,4.02755813980101));
#49218=CARTESIAN_POINT('Ctrl Pts',(-0.495812444326251,1.,4.02084308851832));
#49219=CARTESIAN_POINT('Ctrl Pts',(-0.492115383418018,1.,4.01411733503546));
#49220=CARTESIAN_POINT('Ctrl Pts',(-0.488457130424633,1.,4.0073800839099));
#49221=CARTESIAN_POINT('Ctrl Pts',(-0.484838042421835,1.,4.00063045119288));
#49222=CARTESIAN_POINT('Ctrl Pts',(-0.481258512209675,1.,3.99386775880679));
#49223=CARTESIAN_POINT('Ctrl Pts',(-0.477718999122027,1.,3.98709184306738));
#49224=CARTESIAN_POINT('Ctrl Pts',(-0.47422006101951,1.,3.98030338044409));
#49225=CARTESIAN_POINT('Ctrl Pts',(-0.470762379613439,1.,3.97350414289392));
#49226=CARTESIAN_POINT('Ctrl Pts',(-0.467346690880643,1.,3.9666962227393));
#49227=CARTESIAN_POINT('Ctrl Pts',(-0.463973722115733,1.,3.95988133243538));
#49228=CARTESIAN_POINT('Ctrl Pts',(-0.460644124429121,1.,3.95306005817364));
#49229=CARTESIAN_POINT('Ctrl Pts',(-0.457358410451683,1.,3.94623117206678));
#49230=CARTESIAN_POINT('Ctrl Pts',(-0.454116879027584,1.,3.93939080846298));
#49231=CARTESIAN_POINT('Ctrl Pts',(-0.450919768356348,1.,3.93253407403123));
#49232=CARTESIAN_POINT('Ctrl Pts',(-0.447767416837293,1.,3.92565674143416));
#49233=CARTESIAN_POINT('Ctrl Pts',(-0.444660430230591,1.,3.91875701610719));
#49234=CARTESIAN_POINT('Ctrl Pts',(-0.441599824524054,1.,3.91183704069153));
#49235=CARTESIAN_POINT('Ctrl Pts',(-0.43858723545825,1.,3.90490512938563));
#49236=CARTESIAN_POINT('Ctrl Pts',(-0.435624629433528,1.,3.89797256655462));
#49237=CARTESIAN_POINT('Ctrl Pts',(-0.432713929544458,1.,3.89104947940611));
#49238=CARTESIAN_POINT('Ctrl Pts',(-0.429856640579741,1.,3.88414070943341));
#49239=CARTESIAN_POINT('Ctrl Pts',(-0.427053541173457,1.,3.87724240306597));
#49240=CARTESIAN_POINT('Ctrl Pts',(-0.424304173195111,1.,3.87033643487851));
#49241=CARTESIAN_POINT('Ctrl Pts',(-0.421607423177534,1.,3.86339652542709));
#49242=CARTESIAN_POINT('Ctrl Pts',(-0.418962468086773,1.,3.85639825647996));
#49243=CARTESIAN_POINT('Ctrl Pts',(-0.416369678052907,1.,3.84932864157497));
#49244=CARTESIAN_POINT('Ctrl Pts',(-0.413831367016748,1.,3.84219403994762));
#49245=CARTESIAN_POINT('Ctrl Pts',(-0.411353038798519,1.,3.83503345578698));
#49246=CARTESIAN_POINT('Ctrl Pts',(-0.40894237144746,1.,3.82790724256471));
#49247=CARTESIAN_POINT('Ctrl Pts',(-0.406607038258985,1.,3.8208730391381));
#49248=CARTESIAN_POINT('Ctrl Pts',(-0.404352694628273,1.,3.81396374287793));
#49249=CARTESIAN_POINT('Ctrl Pts',(-0.402181320148436,1.,3.80716881962728));
#49250=CARTESIAN_POINT('Ctrl Pts',(-0.4000883465046,1.,3.80040370384546));
#49251=CARTESIAN_POINT('Ctrl Pts',(-0.39806481868397,1.,3.7935288716329));
#49252=CARTESIAN_POINT('Ctrl Pts',(-0.396103205334841,1.,3.78640521279313));
#49253=CARTESIAN_POINT('Ctrl Pts',(-0.394202481011499,1.,3.77894173114283));
#49254=CARTESIAN_POINT('Ctrl Pts',(-0.392372786223433,1.,3.77114011595967));
#49255=CARTESIAN_POINT('Ctrl Pts',(-0.39064207297956,1.,3.76315635033257));
#49256=CARTESIAN_POINT('Ctrl Pts',(-0.389054775898702,1.,3.75529302895152));
#49257=CARTESIAN_POINT('Ctrl Pts',(-0.387663020050836,1.,3.74792651696654));
#49258=CARTESIAN_POINT('Ctrl Pts',(-0.386519576222251,1.,3.74144965781276));
#49259=CARTESIAN_POINT('Ctrl Pts',(-0.385670806454566,1.,3.73621371845318));
#49260=CARTESIAN_POINT('Ctrl Pts',(-0.385187124634206,1.,3.73273893363406));
#49261=CARTESIAN_POINT('Ctrl Pts',(-0.385031656499164,1.,3.73106082862548));
#49262=CARTESIAN_POINT('Ctrl Pts',(-0.385037797881504,1.,3.73040527621055));
#49263=CARTESIAN_POINT('Ctrl Pts',(-0.385087139000375,1.,3.73021431755274));
#49264=CARTESIAN_POINT('Ctrl Pts',(-0.385112848330762,1.,3.73017266276651));
#49265=CARTESIAN_POINT('',(-0.581791163835815,0.,4.15950947128175));
#49266=CARTESIAN_POINT('Ctrl Pts',(-0.7863229229206,-1.,3.66663282329846));
#49267=CARTESIAN_POINT('Ctrl Pts',(-0.7863229229206,1.,3.66663282329846));
#49268=CARTESIAN_POINT('Ctrl Pts',(-0.786369528183326,-1.,3.66655932661986));
#49269=CARTESIAN_POINT('Ctrl Pts',(-0.786369528183326,1.,3.66655932661986));
#49270=CARTESIAN_POINT('Ctrl Pts',(-0.786480236185697,-1.,3.66657784455334));
#49271=CARTESIAN_POINT('Ctrl Pts',(-0.786480236185697,1.,3.66657784455334));
#49272=CARTESIAN_POINT('Ctrl Pts',(-0.786698783542764,-1.,3.66710211820482));
#49273=CARTESIAN_POINT('Ctrl Pts',(-0.786698783542764,1.,3.66710211820482));
#49274=CARTESIAN_POINT('Ctrl Pts',(-0.787095252590501,-1.,3.66879484801113));
#49275=CARTESIAN_POINT('Ctrl Pts',(-0.787095252590501,1.,3.66879484801113));
#49276=CARTESIAN_POINT('Ctrl Pts',(-0.787758799995743,-1.,3.67252923663655));
#49277=CARTESIAN_POINT('Ctrl Pts',(-0.787758799995743,1.,3.67252923663655));
#49278=CARTESIAN_POINT('Ctrl Pts',(-0.788569566220285,-1.,3.67777119516252));
#49279=CARTESIAN_POINT('Ctrl Pts',(-0.788569566220285,1.,3.67777119516252));
#49280=CARTESIAN_POINT('Ctrl Pts',(-0.789483546064387,-1.,3.68428439783905));
#49281=CARTESIAN_POINT('Ctrl Pts',(-0.789483546064387,1.,3.68428439783905));
#49282=CARTESIAN_POINT('Ctrl Pts',(-0.790436284988788,-1.,3.69172044327364));
#49283=CARTESIAN_POINT('Ctrl Pts',(-0.790436284988788,1.,3.69172044327364));
#49284=CARTESIAN_POINT('Ctrl Pts',(-0.79135657569598,-1.,3.69968940808721));
#49285=CARTESIAN_POINT('Ctrl Pts',(-0.79135657569598,1.,3.69968940808721));
#49286=CARTESIAN_POINT('Ctrl Pts',(-0.792177688845818,-1.,3.70781724021806));
#49287=CARTESIAN_POINT('Ctrl Pts',(-0.792177688845818,1.,3.70781724021806));
#49288=CARTESIAN_POINT('Ctrl Pts',(-0.792848377370287,-1.,3.71580242396124));
#49289=CARTESIAN_POINT('Ctrl Pts',(-0.792848377370287,1.,3.71580242396124));
#49290=CARTESIAN_POINT('Ctrl Pts',(-0.793347023784205,-1.,3.72348797293734));
#49291=CARTESIAN_POINT('Ctrl Pts',(-0.793347023784205,1.,3.72348797293734));
#49292=CARTESIAN_POINT('Ctrl Pts',(-0.793682750269684,-1.,3.73086914695805));
#49293=CARTESIAN_POINT('Ctrl Pts',(-0.793682750269684,1.,3.73086914695805));
#49294=CARTESIAN_POINT('Ctrl Pts',(-0.793882700937017,-1.,3.73803280541687));
#49295=CARTESIAN_POINT('Ctrl Pts',(-0.793882700937017,1.,3.73803280541687));
#49296=CARTESIAN_POINT('Ctrl Pts',(-0.793982700459952,-1.,3.74511357728861));
#49297=CARTESIAN_POINT('Ctrl Pts',(-0.793982700459952,1.,3.74511357728861));
#49298=CARTESIAN_POINT('Ctrl Pts',(-0.794017347371377,-1.,3.75224692493864));
#49299=CARTESIAN_POINT('Ctrl Pts',(-0.794017347371377,1.,3.75224692493864));
#49300=CARTESIAN_POINT('Ctrl Pts',(-0.794008429134907,-1.,3.75951468666257));
#49301=CARTESIAN_POINT('Ctrl Pts',(-0.794008429134907,1.,3.75951468666257));
#49302=CARTESIAN_POINT('Ctrl Pts',(-0.793961083688992,-1.,3.76692626931111));
#49303=CARTESIAN_POINT('Ctrl Pts',(-0.793961083688992,1.,3.76692626931111));
#49304=CARTESIAN_POINT('Ctrl Pts',(-0.793870523787408,-1.,3.77444863801212));
#49305=CARTESIAN_POINT('Ctrl Pts',(-0.793870523787408,1.,3.77444863801212));
#49306=CARTESIAN_POINT('Ctrl Pts',(-0.7937262357813,-1.,3.78202460377598));
#49307=CARTESIAN_POINT('Ctrl Pts',(-0.7937262357813,1.,3.78202460377598));
#49308=CARTESIAN_POINT('Ctrl Pts',(-0.793516871680993,-1.,3.78959439439235));
#49309=CARTESIAN_POINT('Ctrl Pts',(-0.793516871680993,1.,3.78959439439235));
#49310=CARTESIAN_POINT('Ctrl Pts',(-0.793235612973273,-1.,3.79711921389897));
#49311=CARTESIAN_POINT('Ctrl Pts',(-0.793235612973273,1.,3.79711921389897));
#49312=CARTESIAN_POINT('Ctrl Pts',(-0.792882695234778,-1.,3.80459229925637));
#49313=CARTESIAN_POINT('Ctrl Pts',(-0.792882695234778,1.,3.80459229925637));
#49314=CARTESIAN_POINT('Ctrl Pts',(-0.792462483517634,-1.,3.81202588694756));
#49315=CARTESIAN_POINT('Ctrl Pts',(-0.792462483517634,1.,3.81202588694756));
#49316=CARTESIAN_POINT('Ctrl Pts',(-0.791981740718635,-1.,3.81944345442249));
#49317=CARTESIAN_POINT('Ctrl Pts',(-0.791981740718635,1.,3.81944345442249));
#49318=CARTESIAN_POINT('Ctrl Pts',(-0.791447528662369,-1.,3.82687033899792));
#49319=CARTESIAN_POINT('Ctrl Pts',(-0.791447528662369,1.,3.82687033899792));
#49320=CARTESIAN_POINT('Ctrl Pts',(-0.790865012705301,-1.,3.83432392054786));
#49321=CARTESIAN_POINT('Ctrl Pts',(-0.790865012705301,1.,3.83432392054786));
#49322=CARTESIAN_POINT('Ctrl Pts',(-0.790236124191242,-1.,3.84180762342454));
#49323=CARTESIAN_POINT('Ctrl Pts',(-0.790236124191242,1.,3.84180762342454));
#49324=CARTESIAN_POINT('Ctrl Pts',(-0.789560798155582,-1.,3.84931637808894));
#49325=CARTESIAN_POINT('Ctrl Pts',(-0.789560798155582,1.,3.84931637808894));
#49326=CARTESIAN_POINT('Ctrl Pts',(-0.788837734090672,-1.,3.85683995872529));
#49327=CARTESIAN_POINT('Ctrl Pts',(-0.788837734090672,1.,3.85683995872529));
#49328=CARTESIAN_POINT('Ctrl Pts',(-0.788065315093778,-1.,3.86436702561345));
#49329=CARTESIAN_POINT('Ctrl Pts',(-0.788065315093778,1.,3.86436702561345));
#49330=CARTESIAN_POINT('Ctrl Pts',(-0.787242527617999,-1.,3.87188916600912));
#49331=CARTESIAN_POINT('Ctrl Pts',(-0.787242527617999,1.,3.87188916600912));
#49332=CARTESIAN_POINT('Ctrl Pts',(-0.786369675812609,-1.,3.8794040281819));
#49333=CARTESIAN_POINT('Ctrl Pts',(-0.786369675812609,1.,3.8794040281819));
#49334=CARTESIAN_POINT('Ctrl Pts',(-0.78544789034073,-1.,3.88691313167398));
#49335=CARTESIAN_POINT('Ctrl Pts',(-0.78544789034073,1.,3.88691313167398));
#49336=CARTESIAN_POINT('Ctrl Pts',(-0.784478799358336,-1.,3.89442039235103));
#49337=CARTESIAN_POINT('Ctrl Pts',(-0.784478799358336,1.,3.89442039235103));
#49338=CARTESIAN_POINT('Ctrl Pts',(-0.783464141529081,-1.,3.9019303904397));
#49339=CARTESIAN_POINT('Ctrl Pts',(-0.783464141529081,1.,3.9019303904397));
#49340=CARTESIAN_POINT('Ctrl Pts',(-0.782405395622764,-1.,3.90944671004542));
#49341=CARTESIAN_POINT('Ctrl Pts',(-0.782405395622764,1.,3.90944671004542));
#49342=CARTESIAN_POINT('Ctrl Pts',(-0.781303428618367,-1.,3.91697036054676));
#49343=CARTESIAN_POINT('Ctrl Pts',(-0.781303428618367,1.,3.91697036054676));
#49344=CARTESIAN_POINT('Ctrl Pts',(-0.780158678615543,-1.,3.92450058323823));
#49345=CARTESIAN_POINT('Ctrl Pts',(-0.780158678615543,1.,3.92450058323823));
#49346=CARTESIAN_POINT('Ctrl Pts',(-0.778971308134821,-1.,3.93203552473174));
#49347=CARTESIAN_POINT('Ctrl Pts',(-0.778971308134821,1.,3.93203552473174));
#49348=CARTESIAN_POINT('Ctrl Pts',(-0.777741370568559,-1.,3.93957296768103));
#49349=CARTESIAN_POINT('Ctrl Pts',(-0.777741370568559,1.,3.93957296768103));
#49350=CARTESIAN_POINT('Ctrl Pts',(-0.776468966697921,-1.,3.94711101619447));
#49351=CARTESIAN_POINT('Ctrl Pts',(-0.776468966697921,1.,3.94711101619447));
#49352=CARTESIAN_POINT('Ctrl Pts',(-0.775154418039352,-1.,3.9546488545231));
#49353=CARTESIAN_POINT('Ctrl Pts',(-0.775154418039352,1.,3.9546488545231));
#49354=CARTESIAN_POINT('Ctrl Pts',(-0.773798212026566,-1.,3.96218649639807));
#49355=CARTESIAN_POINT('Ctrl Pts',(-0.773798212026566,1.,3.96218649639807));
#49356=CARTESIAN_POINT('Ctrl Pts',(-0.772400931772136,-1.,3.96972446532772));
#49357=CARTESIAN_POINT('Ctrl Pts',(-0.772400931772136,1.,3.96972446532772));
#49358=CARTESIAN_POINT('Ctrl Pts',(-0.770963190030471,-1.,3.97726349165488));
#49359=CARTESIAN_POINT('Ctrl Pts',(-0.770963190030471,1.,3.97726349165488));
#49360=CARTESIAN_POINT('Ctrl Pts',(-0.769485566245544,-1.,3.98480422348451));
#49361=CARTESIAN_POINT('Ctrl Pts',(-0.769485566245544,1.,3.98480422348451));
#49362=CARTESIAN_POINT('Ctrl Pts',(-0.767968531377915,-1.,3.9923468788101));
#49363=CARTESIAN_POINT('Ctrl Pts',(-0.767968531377915,1.,3.9923468788101));
#49364=CARTESIAN_POINT('Ctrl Pts',(-0.766412457136064,-1.,3.99989129179622));
#49365=CARTESIAN_POINT('Ctrl Pts',(-0.766412457136064,1.,3.99989129179622));
#49366=CARTESIAN_POINT('Ctrl Pts',(-0.764817648785198,-1.,4.00743706791509));
#49367=CARTESIAN_POINT('Ctrl Pts',(-0.764817648785198,1.,4.00743706791509));
#49368=CARTESIAN_POINT('Ctrl Pts',(-0.763184371182935,-1.,4.01498370680496));
#49369=CARTESIAN_POINT('Ctrl Pts',(-0.763184371182935,1.,4.01498370680496));
#49370=CARTESIAN_POINT('Ctrl Pts',(-0.761512875859804,-1.,4.02253072741268));
#49371=CARTESIAN_POINT('Ctrl Pts',(-0.761512875859804,1.,4.02253072741268));
#49372=CARTESIAN_POINT('Ctrl Pts',(-0.759803433243752,-1.,4.03007781954412));
#49373=CARTESIAN_POINT('Ctrl Pts',(-0.759803433243752,1.,4.03007781954412));
#49374=CARTESIAN_POINT('Ctrl Pts',(-0.758056338884944,-1.,4.03762485803119));
#49375=CARTESIAN_POINT('Ctrl Pts',(-0.758056338884944,1.,4.03762485803119));
#49376=CARTESIAN_POINT('Ctrl Pts',(-0.756271902369581,-1.,4.04517182653997));
#49377=CARTESIAN_POINT('Ctrl Pts',(-0.756271902369581,1.,4.04517182653997));
#49378=CARTESIAN_POINT('Ctrl Pts',(-0.754450441816078,-1.,4.05271876687915));
#49379=CARTESIAN_POINT('Ctrl Pts',(-0.754450441816078,1.,4.05271876687915));
#49380=CARTESIAN_POINT('Ctrl Pts',(-0.752592276483072,-1.,4.06026572221515));
#49381=CARTESIAN_POINT('Ctrl Pts',(-0.752592276483072,1.,4.06026572221515));
#49382=CARTESIAN_POINT('Ctrl Pts',(-0.750697720484036,-1.,4.06781267242378));
#49383=CARTESIAN_POINT('Ctrl Pts',(-0.750697720484036,1.,4.06781267242378));
#49384=CARTESIAN_POINT('Ctrl Pts',(-0.748767076680557,-1.,4.07535951056152));
#49385=CARTESIAN_POINT('Ctrl Pts',(-0.748767076680557,1.,4.07535951056152));
#49386=CARTESIAN_POINT('Ctrl Pts',(-0.746800631492315,-1.,4.08290608095642));
#49387=CARTESIAN_POINT('Ctrl Pts',(-0.746800631492315,1.,4.08290608095642));
#49388=CARTESIAN_POINT('Ctrl Pts',(-0.7447986497065,-1.,4.09045220253573));
#49389=CARTESIAN_POINT('Ctrl Pts',(-0.7447986497065,1.,4.09045220253573));
#49390=CARTESIAN_POINT('Ctrl Pts',(-0.742761369689841,-1.,4.09799769702611));
#49391=CARTESIAN_POINT('Ctrl Pts',(-0.742761369689841,1.,4.09799769702611));
#49392=CARTESIAN_POINT('Ctrl Pts',(-0.740688998553377,-1.,4.10554241757547));
#49393=CARTESIAN_POINT('Ctrl Pts',(-0.740688998553377,1.,4.10554241757547));
#49394=CARTESIAN_POINT('Ctrl Pts',(-0.738581708225844,-1.,4.11308626951927));
#49395=CARTESIAN_POINT('Ctrl Pts',(-0.738581708225844,1.,4.11308626951927));
#49396=CARTESIAN_POINT('Ctrl Pts',(-0.736439634331345,-1.,4.120629196238));
#49397=CARTESIAN_POINT('Ctrl Pts',(-0.736439634331345,1.,4.120629196238));
#49398=CARTESIAN_POINT('Ctrl Pts',(-0.734698226764092,-1.,4.12666277570844));
#49399=CARTESIAN_POINT('Ctrl Pts',(-0.734698226764092,1.,4.12666277570844));
#49400=CARTESIAN_POINT('Ctrl Pts',(-0.733376589323546,-1.,4.13118752795207));
#49401=CARTESIAN_POINT('Ctrl Pts',(-0.733376589323546,1.,4.13118752795207));
#49402=CARTESIAN_POINT('Ctrl Pts',(-0.73248857513516,-1.,4.1342038373684));
#49403=CARTESIAN_POINT('Ctrl Pts',(-0.73248857513516,1.,4.1342038373684));
#49404=CARTESIAN_POINT('Ctrl Pts',(-0.73204283740062,-1.,4.13571194405636));
#49405=CARTESIAN_POINT('Ctrl Pts',(-0.73204283740062,1.,4.13571194405636));
#49406=CARTESIAN_POINT('',(-0.786422660831985,1.,3.66661143271685));
#49407=CARTESIAN_POINT('Ctrl Pts',(-0.786422660831985,-1.,3.66661143271685));
#49408=CARTESIAN_POINT('Ctrl Pts',(-0.786422660831985,-0.666666666666667,
3.66661143271685));
#49409=CARTESIAN_POINT('Ctrl Pts',(-0.786422660831985,-0.333333333333333,
3.66661143271685));
#49410=CARTESIAN_POINT('Ctrl Pts',(-0.786422660831985,0.333333333333333,
3.66661143271685));
#49411=CARTESIAN_POINT('Ctrl Pts',(-0.786422660831985,0.666666666666667,
3.66661143271685));
#49412=CARTESIAN_POINT('Ctrl Pts',(-0.786422660831985,1.,3.66661143271685));
#49413=CARTESIAN_POINT('',(-0.73204283740062,1.,4.13571194405636));
#49414=CARTESIAN_POINT('',(-0.73204283740062,0.,4.13571194405636));
#49415=CARTESIAN_POINT('Ctrl Pts',(-0.786422660831985,1.,3.66661143271685));
#49416=CARTESIAN_POINT('Ctrl Pts',(-0.786459983895432,1.,3.6666431041522));
#49417=CARTESIAN_POINT('Ctrl Pts',(-0.786565919558984,1.,3.66680946938292));
#49418=CARTESIAN_POINT('Ctrl Pts',(-0.786774337198062,1.,3.66743103898702));
#49419=CARTESIAN_POINT('Ctrl Pts',(-0.787145041181546,1.,3.66907505398677));
#49420=CARTESIAN_POINT('Ctrl Pts',(-0.787758799995743,1.,3.67252923663655));
#49421=CARTESIAN_POINT('Ctrl Pts',(-0.788569566220285,1.,3.67777119516252));
#49422=CARTESIAN_POINT('Ctrl Pts',(-0.789483546064387,1.,3.68428439783905));
#49423=CARTESIAN_POINT('Ctrl Pts',(-0.790436284988788,1.,3.69172044327364));
#49424=CARTESIAN_POINT('Ctrl Pts',(-0.79135657569598,1.,3.69968940808721));
#49425=CARTESIAN_POINT('Ctrl Pts',(-0.792177688845818,1.,3.70781724021806));
#49426=CARTESIAN_POINT('Ctrl Pts',(-0.792848377370287,1.,3.71580242396124));
#49427=CARTESIAN_POINT('Ctrl Pts',(-0.793347023784205,1.,3.72348797293734));
#49428=CARTESIAN_POINT('Ctrl Pts',(-0.793682750269684,1.,3.73086914695805));
#49429=CARTESIAN_POINT('Ctrl Pts',(-0.793882700937017,1.,3.73803280541687));
#49430=CARTESIAN_POINT('Ctrl Pts',(-0.793982700459952,1.,3.74511357728861));
#49431=CARTESIAN_POINT('Ctrl Pts',(-0.794017347371377,1.,3.75224692493864));
#49432=CARTESIAN_POINT('Ctrl Pts',(-0.794008429134907,1.,3.75951468666257));
#49433=CARTESIAN_POINT('Ctrl Pts',(-0.793961083688992,1.,3.76692626931111));
#49434=CARTESIAN_POINT('Ctrl Pts',(-0.793870523787408,1.,3.77444863801212));
#49435=CARTESIAN_POINT('Ctrl Pts',(-0.7937262357813,1.,3.78202460377598));
#49436=CARTESIAN_POINT('Ctrl Pts',(-0.793516871680993,1.,3.78959439439235));
#49437=CARTESIAN_POINT('Ctrl Pts',(-0.793235612973273,1.,3.79711921389897));
#49438=CARTESIAN_POINT('Ctrl Pts',(-0.792882695234778,1.,3.80459229925637));
#49439=CARTESIAN_POINT('Ctrl Pts',(-0.792462483517634,1.,3.81202588694756));
#49440=CARTESIAN_POINT('Ctrl Pts',(-0.791981740718635,1.,3.81944345442249));
#49441=CARTESIAN_POINT('Ctrl Pts',(-0.791447528662369,1.,3.82687033899792));
#49442=CARTESIAN_POINT('Ctrl Pts',(-0.790865012705301,1.,3.83432392054786));
#49443=CARTESIAN_POINT('Ctrl Pts',(-0.790236124191242,1.,3.84180762342454));
#49444=CARTESIAN_POINT('Ctrl Pts',(-0.789560798155582,1.,3.84931637808894));
#49445=CARTESIAN_POINT('Ctrl Pts',(-0.788837734090672,1.,3.85683995872529));
#49446=CARTESIAN_POINT('Ctrl Pts',(-0.788065315093778,1.,3.86436702561345));
#49447=CARTESIAN_POINT('Ctrl Pts',(-0.787242527617999,1.,3.87188916600912));
#49448=CARTESIAN_POINT('Ctrl Pts',(-0.786369675812609,1.,3.8794040281819));
#49449=CARTESIAN_POINT('Ctrl Pts',(-0.78544789034073,1.,3.88691313167398));
#49450=CARTESIAN_POINT('Ctrl Pts',(-0.784478799358336,1.,3.89442039235103));
#49451=CARTESIAN_POINT('Ctrl Pts',(-0.783464141529081,1.,3.9019303904397));
#49452=CARTESIAN_POINT('Ctrl Pts',(-0.782405395622764,1.,3.90944671004542));
#49453=CARTESIAN_POINT('Ctrl Pts',(-0.781303428618367,1.,3.91697036054676));
#49454=CARTESIAN_POINT('Ctrl Pts',(-0.780158678615543,1.,3.92450058323823));
#49455=CARTESIAN_POINT('Ctrl Pts',(-0.778971308134821,1.,3.93203552473174));
#49456=CARTESIAN_POINT('Ctrl Pts',(-0.777741370568559,1.,3.93957296768103));
#49457=CARTESIAN_POINT('Ctrl Pts',(-0.776468966697921,1.,3.94711101619447));
#49458=CARTESIAN_POINT('Ctrl Pts',(-0.775154418039352,1.,3.9546488545231));
#49459=CARTESIAN_POINT('Ctrl Pts',(-0.773798212026566,1.,3.96218649639807));
#49460=CARTESIAN_POINT('Ctrl Pts',(-0.772400931772136,1.,3.96972446532772));
#49461=CARTESIAN_POINT('Ctrl Pts',(-0.770963190030471,1.,3.97726349165488));
#49462=CARTESIAN_POINT('Ctrl Pts',(-0.769485566245544,1.,3.98480422348451));
#49463=CARTESIAN_POINT('Ctrl Pts',(-0.767968531377915,1.,3.9923468788101));
#49464=CARTESIAN_POINT('Ctrl Pts',(-0.766412457136064,1.,3.99989129179622));
#49465=CARTESIAN_POINT('Ctrl Pts',(-0.764817648785198,1.,4.00743706791509));
#49466=CARTESIAN_POINT('Ctrl Pts',(-0.763184371182935,1.,4.01498370680496));
#49467=CARTESIAN_POINT('Ctrl Pts',(-0.761512875859804,1.,4.02253072741268));
#49468=CARTESIAN_POINT('Ctrl Pts',(-0.759803433243752,1.,4.03007781954412));
#49469=CARTESIAN_POINT('Ctrl Pts',(-0.758056338884944,1.,4.03762485803119));
#49470=CARTESIAN_POINT('Ctrl Pts',(-0.756271902369581,1.,4.04517182653997));
#49471=CARTESIAN_POINT('Ctrl Pts',(-0.754450441816078,1.,4.05271876687915));
#49472=CARTESIAN_POINT('Ctrl Pts',(-0.752592276483072,1.,4.06026572221515));
#49473=CARTESIAN_POINT('Ctrl Pts',(-0.750697720484036,1.,4.06781267242378));
#49474=CARTESIAN_POINT('Ctrl Pts',(-0.748767076680557,1.,4.07535951056152));
#49475=CARTESIAN_POINT('Ctrl Pts',(-0.746800631492315,1.,4.08290608095642));
#49476=CARTESIAN_POINT('Ctrl Pts',(-0.7447986497065,1.,4.09045220253573));
#49477=CARTESIAN_POINT('Ctrl Pts',(-0.742761369689841,1.,4.09799769702611));
#49478=CARTESIAN_POINT('Ctrl Pts',(-0.740688998553377,1.,4.10554241757547));
#49479=CARTESIAN_POINT('Ctrl Pts',(-0.738581708225844,1.,4.11308626951927));
#49480=CARTESIAN_POINT('Ctrl Pts',(-0.736439634331345,1.,4.120629196238));
#49481=CARTESIAN_POINT('Ctrl Pts',(-0.734698226764092,1.,4.12666277570844));
#49482=CARTESIAN_POINT('Ctrl Pts',(-0.733376589323546,1.,4.13118752795207));
#49483=CARTESIAN_POINT('Ctrl Pts',(-0.73248857513516,1.,4.1342038373684));
#49484=CARTESIAN_POINT('Ctrl Pts',(-0.73204283740062,1.,4.13571194405636));
#49485=CARTESIAN_POINT('Origin',(-0.73204283740062,0.,4.13571194405636));
#49486=CARTESIAN_POINT('',(-0.581791163835815,1.,4.15950947128175));
#49487=CARTESIAN_POINT('Origin',(0.,0.,0.));
#49488=CARTESIAN_POINT('',(-0.963899035117249,1.,3.62400312501245));
#49489=CARTESIAN_POINT('Origin',(0.,1.,0.));
#49490=CARTESIAN_POINT('Ctrl Pts',(-0.963899035117249,1.,3.62400312501245));
#49491=CARTESIAN_POINT('Ctrl Pts',(-0.963899035117249,0.666666666666667,
3.62400312501245));
#49492=CARTESIAN_POINT('Ctrl Pts',(-0.963899035117249,0.333333333333333,
3.62400312501245));
#49493=CARTESIAN_POINT('Ctrl Pts',(-0.963899035117249,-0.333333333333333,
3.62400312501245));
#49494=CARTESIAN_POINT('Ctrl Pts',(-0.963899035117249,-0.666666666666667,
3.62400312501245));
#49495=CARTESIAN_POINT('Ctrl Pts',(-0.963899035117249,-1.,3.62400312501245));
#49496=CARTESIAN_POINT('Ctrl Pts',(-1.22531898815164,-1.,4.01728681790024));
#49497=CARTESIAN_POINT('Ctrl Pts',(-1.22531898815164,1.,4.01728681790024));
#49498=CARTESIAN_POINT('Ctrl Pts',(-1.22423716681447,-1.,4.0161454457032));
#49499=CARTESIAN_POINT('Ctrl Pts',(-1.22423716681447,1.,4.0161454457032));
#49500=CARTESIAN_POINT('Ctrl Pts',(-1.22207656456199,-1.,4.01386104434674));
#49501=CARTESIAN_POINT('Ctrl Pts',(-1.22207656456199,1.,4.01386104434674));
#49502=CARTESIAN_POINT('Ctrl Pts',(-1.21884478244983,-1.,4.01042947142681));
#49503=CARTESIAN_POINT('Ctrl Pts',(-1.21884478244983,1.,4.01042947142681));
#49504=CARTESIAN_POINT('Ctrl Pts',(-1.21455398918813,-1.,4.00584409524937));
#49505=CARTESIAN_POINT('Ctrl Pts',(-1.21455398918813,1.,4.00584409524937));
#49506=CARTESIAN_POINT('Ctrl Pts',(-1.20922097030107,-1.,4.00009577952534));
#49507=CARTESIAN_POINT('Ctrl Pts',(-1.20922097030107,1.,4.00009577952534));
#49508=CARTESIAN_POINT('Ctrl Pts',(-1.2039185237544,-1.,3.99433084800649));
#49509=CARTESIAN_POINT('Ctrl Pts',(-1.2039185237544,1.,3.99433084800649));
#49510=CARTESIAN_POINT('Ctrl Pts',(-1.19864679609596,-1.,3.98854928957287));
#49511=CARTESIAN_POINT('Ctrl Pts',(-1.19864679609596,1.,3.98854928957287));
#49512=CARTESIAN_POINT('Ctrl Pts',(-1.19340598349307,-1.,3.98275111052015));
#49513=CARTESIAN_POINT('Ctrl Pts',(-1.19340598349307,1.,3.98275111052015));
#49514=CARTESIAN_POINT('Ctrl Pts',(-1.18819633715285,-1.,3.97693634766926));
#49515=CARTESIAN_POINT('Ctrl Pts',(-1.18819633715285,1.,3.97693634766926));
#49516=CARTESIAN_POINT('Ctrl Pts',(-1.18301815039596,-1.,3.9711050516465));
#49517=CARTESIAN_POINT('Ctrl Pts',(-1.18301815039596,1.,3.9711050516465));
#49518=CARTESIAN_POINT('Ctrl Pts',(-1.17787174135445,-1.,3.96525726357682));
#49519=CARTESIAN_POINT('Ctrl Pts',(-1.17787174135445,1.,3.96525726357682));
#49520=CARTESIAN_POINT('Ctrl Pts',(-1.17275743590327,-1.,3.95939299213164));
#49521=CARTESIAN_POINT('Ctrl Pts',(-1.17275743590327,1.,3.95939299213164));
#49522=CARTESIAN_POINT('Ctrl Pts',(-1.16767555244495,-1.,3.95351219510062));
#49523=CARTESIAN_POINT('Ctrl Pts',(-1.16767555244495,1.,3.95351219510062));
#49524=CARTESIAN_POINT('Ctrl Pts',(-1.16262637999261,-1.,3.9476147478092));
#49525=CARTESIAN_POINT('Ctrl Pts',(-1.16262637999261,1.,3.9476147478092));
#49526=CARTESIAN_POINT('Ctrl Pts',(-1.1576101834106,-1.,3.94170046685542));
#49527=CARTESIAN_POINT('Ctrl Pts',(-1.1576101834106,1.,3.94170046685542));
#49528=CARTESIAN_POINT('Ctrl Pts',(-1.15262722716391,-1.,3.9357691705651));
#49529=CARTESIAN_POINT('Ctrl Pts',(-1.15262722716391,1.,3.9357691705651));
#49530=CARTESIAN_POINT('Ctrl Pts',(-1.14767779451147,-1.,3.92982073294334));
#49531=CARTESIAN_POINT('Ctrl Pts',(-1.14767779451147,1.,3.92982073294334));
#49532=CARTESIAN_POINT('Ctrl Pts',(-1.14276220561575,-1.,3.92385513133937));
#49533=CARTESIAN_POINT('Ctrl Pts',(-1.14276220561575,1.,3.92385513133937));
#49534=CARTESIAN_POINT('Ctrl Pts',(-1.13788084225511,-1.,3.91787251936688));
#49535=CARTESIAN_POINT('Ctrl Pts',(-1.13788084225511,1.,3.91787251936688));
#49536=CARTESIAN_POINT('Ctrl Pts',(-1.13303414693849,-1.,3.91187321145495));
#49537=CARTESIAN_POINT('Ctrl Pts',(-1.13303414693849,1.,3.91187321145495));
#49538=CARTESIAN_POINT('Ctrl Pts',(-1.12822258281518,-1.,3.90585753318622));
#49539=CARTESIAN_POINT('Ctrl Pts',(-1.12822258281518,1.,3.90585753318622));
#49540=CARTESIAN_POINT('Ctrl Pts',(-1.12344660099029,-1.,3.89982569749978));
#49541=CARTESIAN_POINT('Ctrl Pts',(-1.12344660099029,1.,3.89982569749978));
#49542=CARTESIAN_POINT('Ctrl Pts',(-1.11870660794609,-1.,3.89377768340362));
#49543=CARTESIAN_POINT('Ctrl Pts',(-1.11870660794609,1.,3.89377768340362));
#49544=CARTESIAN_POINT('Ctrl Pts',(-1.11400292434447,-1.,3.88771308285229));
#49545=CARTESIAN_POINT('Ctrl Pts',(-1.11400292434447,1.,3.88771308285229));
#49546=CARTESIAN_POINT('Ctrl Pts',(-1.10933577224029,-1.,3.88163105531791));
#49547=CARTESIAN_POINT('Ctrl Pts',(-1.10933577224029,1.,3.88163105531791));
#49548=CARTESIAN_POINT('Ctrl Pts',(-1.10470536603303,-1.,3.87553067187566));
#49549=CARTESIAN_POINT('Ctrl Pts',(-1.10470536603303,1.,3.87553067187566));
#49550=CARTESIAN_POINT('Ctrl Pts',(-1.10011198761202,-1.,3.86941120134872));
#49551=CARTESIAN_POINT('Ctrl Pts',(-1.10011198761202,1.,3.86941120134872));
#49552=CARTESIAN_POINT('Ctrl Pts',(-1.09555606505012,-1.,3.86327241021242));
#49553=CARTESIAN_POINT('Ctrl Pts',(-1.09555606505012,1.,3.86327241021242));
#49554=CARTESIAN_POINT('Ctrl Pts',(-1.09103825516288,-1.,3.85711487933911));
#49555=CARTESIAN_POINT('Ctrl Pts',(-1.09103825516288,1.,3.85711487933911));
#49556=CARTESIAN_POINT('Ctrl Pts',(-1.08655950846377,-1.,3.8509402522269));
#49557=CARTESIAN_POINT('Ctrl Pts',(-1.08655950846377,1.,3.8509402522269));
#49558=CARTESIAN_POINT('Ctrl Pts',(-1.08212087917986,-1.,3.84475048030615));
#49559=CARTESIAN_POINT('Ctrl Pts',(-1.08212087917986,1.,3.84475048030615));
#49560=CARTESIAN_POINT('Ctrl Pts',(-1.07772335353856,-1.,3.83854714117486));
#49561=CARTESIAN_POINT('Ctrl Pts',(-1.07772335353856,1.,3.83854714117486));
#49562=CARTESIAN_POINT('Ctrl Pts',(-1.0733676663346,-1.,3.83233071195145));
#49563=CARTESIAN_POINT('Ctrl Pts',(-1.0733676663346,1.,3.83233071195145));
#49564=CARTESIAN_POINT('Ctrl Pts',(-1.0690541318036,-1.,3.82609989967278));
#49565=CARTESIAN_POINT('Ctrl Pts',(-1.0690541318036,1.,3.82609989967278));
#49566=CARTESIAN_POINT('Ctrl Pts',(-1.06478244038931,-1.,3.81985083953012));
#49567=CARTESIAN_POINT('Ctrl Pts',(-1.06478244038931,1.,3.81985083953012));
#49568=CARTESIAN_POINT('Ctrl Pts',(-1.06055206187298,-1.,3.81357866117485));
#49569=CARTESIAN_POINT('Ctrl Pts',(-1.06055206187298,1.,3.81357866117485));
#49570=CARTESIAN_POINT('Ctrl Pts',(-1.05636266918643,-1.,3.80727913637784));
#49571=CARTESIAN_POINT('Ctrl Pts',(-1.05636266918643,1.,3.80727913637784));
#49572=CARTESIAN_POINT('Ctrl Pts',(-1.05221457990015,-1.,3.80095039790678));
#49573=CARTESIAN_POINT('Ctrl Pts',(-1.05221457990015,1.,3.80095039790678));
#49574=CARTESIAN_POINT('Ctrl Pts',(-1.04810913267641,-1.,3.79459440308793));
#49575=CARTESIAN_POINT('Ctrl Pts',(-1.04810913267641,1.,3.79459440308793));
#49576=CARTESIAN_POINT('Ctrl Pts',(-1.04404924374426,-1.,3.78821910787195));
#49577=CARTESIAN_POINT('Ctrl Pts',(-1.04404924374426,1.,3.78821910787195));
#49578=CARTESIAN_POINT('Ctrl Pts',(-1.04003862055804,-1.,3.78183535008192));
#49579=CARTESIAN_POINT('Ctrl Pts',(-1.04003862055804,1.,3.78183535008192));
#49580=CARTESIAN_POINT('Ctrl Pts',(-1.03608074678013,-1.,3.77545283140445));
#49581=CARTESIAN_POINT('Ctrl Pts',(-1.03608074678013,1.,3.77545283140445));
#49582=CARTESIAN_POINT('Ctrl Pts',(-1.0321778660492,-1.,3.76907609832522));
#49583=CARTESIAN_POINT('Ctrl Pts',(-1.0321778660492,1.,3.76907609832522));
#49584=CARTESIAN_POINT('Ctrl Pts',(-1.02833014458181,-1.,3.76270122291232));
#49585=CARTESIAN_POINT('Ctrl Pts',(-1.02833014458181,1.,3.76270122291232));
#49586=CARTESIAN_POINT('Ctrl Pts',(-1.0245342944466,-1.,3.75631037456194));
#49587=CARTESIAN_POINT('Ctrl Pts',(-1.0245342944466,1.,3.75631037456194));
#49588=CARTESIAN_POINT('Ctrl Pts',(-1.02078510487428,-1.,3.74987777155834));
#49589=CARTESIAN_POINT('Ctrl Pts',(-1.02078510487428,1.,3.74987777155834));
#49590=CARTESIAN_POINT('Ctrl Pts',(-1.01707794311079,-1.,3.74337942504959));
#49591=CARTESIAN_POINT('Ctrl Pts',(-1.01707794311079,1.,3.74337942504959));
#49592=CARTESIAN_POINT('Ctrl Pts',(-1.01341114319903,-1.,3.73680245055734));
#49593=CARTESIAN_POINT('Ctrl Pts',(-1.01341114319903,1.,3.73680245055734));
#49594=CARTESIAN_POINT('Ctrl Pts',(-1.00978798539496,-1.,3.73015276704426));
#49595=CARTESIAN_POINT('Ctrl Pts',(-1.00978798539496,1.,3.73015276704426));
#49596=CARTESIAN_POINT('Ctrl Pts',(-1.0062200073571,-1.,3.72346803750595));
#49597=CARTESIAN_POINT('Ctrl Pts',(-1.0062200073571,1.,3.72346803750595));
#49598=CARTESIAN_POINT('Ctrl Pts',(-1.00272423396822,-1.,3.71680667125118));
#49599=CARTESIAN_POINT('Ctrl Pts',(-1.00272423396822,1.,3.71680667125118));
#49600=CARTESIAN_POINT('Ctrl Pts',(-0.999317260756531,-1.,3.71022439713938));
#49601=CARTESIAN_POINT('Ctrl Pts',(-0.999317260756531,1.,3.71022439713938));
#49602=CARTESIAN_POINT('Ctrl Pts',(-0.996009819772518,-1.,3.70375282282138));
#49603=CARTESIAN_POINT('Ctrl Pts',(-0.996009819772518,1.,3.70375282282138));
#49604=CARTESIAN_POINT('Ctrl Pts',(-0.99280221833201,-1.,3.69738123415662));
#49605=CARTESIAN_POINT('Ctrl Pts',(-0.99280221833201,1.,3.69738123415662));
#49606=CARTESIAN_POINT('Ctrl Pts',(-0.989676715398558,-1.,3.69102682138846));
#49607=CARTESIAN_POINT('Ctrl Pts',(-0.989676715398558,1.,3.69102682138846));
#49608=CARTESIAN_POINT('Ctrl Pts',(-0.986602639863838,-1.,3.68455317926068));
#49609=CARTESIAN_POINT('Ctrl Pts',(-0.986602639863838,1.,3.68455317926068));
#49610=CARTESIAN_POINT('Ctrl Pts',(-0.983550791470419,-1.,3.67782408841715));
#49611=CARTESIAN_POINT('Ctrl Pts',(-0.983550791470419,1.,3.67782408841715));
#49612=CARTESIAN_POINT('Ctrl Pts',(-0.980505922458267,-1.,3.67074983340361));
#49613=CARTESIAN_POINT('Ctrl Pts',(-0.980505922458267,1.,3.67074983340361));
#49614=CARTESIAN_POINT('Ctrl Pts',(-0.977478312751618,-1.,3.66333049637475));
#49615=CARTESIAN_POINT('Ctrl Pts',(-0.977478312751618,1.,3.66333049637475));
#49616=CARTESIAN_POINT('Ctrl Pts',(-0.974519971354848,-1.,3.65571576735126));
#49617=CARTESIAN_POINT('Ctrl Pts',(-0.974519971354848,1.,3.65571576735126));
#49618=CARTESIAN_POINT('Ctrl Pts',(-0.971722122061341,-1.,3.64819756447455));
#49619=CARTESIAN_POINT('Ctrl Pts',(-0.971722122061341,1.,3.64819756447455));
#49620=CARTESIAN_POINT('Ctrl Pts',(-0.969195124675866,-1.,3.64113946505766));
#49621=CARTESIAN_POINT('Ctrl Pts',(-0.969195124675866,1.,3.64113946505766));
#49622=CARTESIAN_POINT('Ctrl Pts',(-0.967052554541386,-1.,3.63492122081143));
#49623=CARTESIAN_POINT('Ctrl Pts',(-0.967052554541386,1.,3.63492122081143));
#49624=CARTESIAN_POINT('Ctrl Pts',(-0.965395153165293,-1.,3.62988252139846));
#49625=CARTESIAN_POINT('Ctrl Pts',(-0.965395153165293,1.,3.62988252139846));
#49626=CARTESIAN_POINT('Ctrl Pts',(-0.964291001273288,-1.,3.62625391254797));
#49627=CARTESIAN_POINT('Ctrl Pts',(-0.964291001273288,1.,3.62625391254797));
#49628=CARTESIAN_POINT('Ctrl Pts',(-0.963875774530619,-1.,3.6245656860652));
#49629=CARTESIAN_POINT('Ctrl Pts',(-0.963875774530619,1.,3.6245656860652));
#49630=CARTESIAN_POINT('Ctrl Pts',(-0.963832486395051,-1.,3.62399933639914));
#49631=CARTESIAN_POINT('Ctrl Pts',(-0.963832486395051,1.,3.62399933639914));
#49632=CARTESIAN_POINT('Ctrl Pts',(-0.963922720982193,-1.,3.62393257642052));
#49633=CARTESIAN_POINT('Ctrl Pts',(-0.963922720982193,1.,3.62393257642052));
#49634=CARTESIAN_POINT('Ctrl Pts',(-0.963997613369571,-1.,3.62397690409552));
#49635=CARTESIAN_POINT('Ctrl Pts',(-0.963997613369571,1.,3.62397690409552));
#49636=CARTESIAN_POINT('',(-1.22531898815164,1.,4.01728681790024));
#49637=CARTESIAN_POINT('Ctrl Pts',(-1.22531898815164,1.,4.01728681790024));
#49638=CARTESIAN_POINT('Ctrl Pts',(-1.22423716681447,1.,4.0161454457032));
#49639=CARTESIAN_POINT('Ctrl Pts',(-1.22207656456199,1.,4.01386104434674));
#49640=CARTESIAN_POINT('Ctrl Pts',(-1.21884478244983,1.,4.01042947142681));
#49641=CARTESIAN_POINT('Ctrl Pts',(-1.21455398918813,1.,4.00584409524937));
#49642=CARTESIAN_POINT('Ctrl Pts',(-1.20922097030107,1.,4.00009577952534));
#49643=CARTESIAN_POINT('Ctrl Pts',(-1.2039185237544,1.,3.99433084800649));
#49644=CARTESIAN_POINT('Ctrl Pts',(-1.19864679609596,1.,3.98854928957287));
#49645=CARTESIAN_POINT('Ctrl Pts',(-1.19340598349307,1.,3.98275111052015));
#49646=CARTESIAN_POINT('Ctrl Pts',(-1.18819633715285,1.,3.97693634766926));
#49647=CARTESIAN_POINT('Ctrl Pts',(-1.18301815039596,1.,3.9711050516465));
#49648=CARTESIAN_POINT('Ctrl Pts',(-1.17787174135445,1.,3.96525726357682));
#49649=CARTESIAN_POINT('Ctrl Pts',(-1.17275743590327,1.,3.95939299213164));
#49650=CARTESIAN_POINT('Ctrl Pts',(-1.16767555244495,1.,3.95351219510062));
#49651=CARTESIAN_POINT('Ctrl Pts',(-1.16262637999261,1.,3.9476147478092));
#49652=CARTESIAN_POINT('Ctrl Pts',(-1.1576101834106,1.,3.94170046685542));
#49653=CARTESIAN_POINT('Ctrl Pts',(-1.15262722716391,1.,3.9357691705651));
#49654=CARTESIAN_POINT('Ctrl Pts',(-1.14767779451147,1.,3.92982073294334));
#49655=CARTESIAN_POINT('Ctrl Pts',(-1.14276220561575,1.,3.92385513133937));
#49656=CARTESIAN_POINT('Ctrl Pts',(-1.13788084225511,1.,3.91787251936688));
#49657=CARTESIAN_POINT('Ctrl Pts',(-1.13303414693849,1.,3.91187321145495));
#49658=CARTESIAN_POINT('Ctrl Pts',(-1.12822258281518,1.,3.90585753318622));
#49659=CARTESIAN_POINT('Ctrl Pts',(-1.12344660099029,1.,3.89982569749978));
#49660=CARTESIAN_POINT('Ctrl Pts',(-1.11870660794609,1.,3.89377768340362));
#49661=CARTESIAN_POINT('Ctrl Pts',(-1.11400292434447,1.,3.88771308285229));
#49662=CARTESIAN_POINT('Ctrl Pts',(-1.10933577224029,1.,3.88163105531791));
#49663=CARTESIAN_POINT('Ctrl Pts',(-1.10470536603303,1.,3.87553067187566));
#49664=CARTESIAN_POINT('Ctrl Pts',(-1.10011198761202,1.,3.86941120134872));
#49665=CARTESIAN_POINT('Ctrl Pts',(-1.09555606505012,1.,3.86327241021242));
#49666=CARTESIAN_POINT('Ctrl Pts',(-1.09103825516288,1.,3.85711487933911));
#49667=CARTESIAN_POINT('Ctrl Pts',(-1.08655950846377,1.,3.8509402522269));
#49668=CARTESIAN_POINT('Ctrl Pts',(-1.08212087917986,1.,3.84475048030615));
#49669=CARTESIAN_POINT('Ctrl Pts',(-1.07772335353856,1.,3.83854714117486));
#49670=CARTESIAN_POINT('Ctrl Pts',(-1.0733676663346,1.,3.83233071195145));
#49671=CARTESIAN_POINT('Ctrl Pts',(-1.0690541318036,1.,3.82609989967278));
#49672=CARTESIAN_POINT('Ctrl Pts',(-1.06478244038931,1.,3.81985083953012));
#49673=CARTESIAN_POINT('Ctrl Pts',(-1.06055206187298,1.,3.81357866117485));
#49674=CARTESIAN_POINT('Ctrl Pts',(-1.05636266918643,1.,3.80727913637784));
#49675=CARTESIAN_POINT('Ctrl Pts',(-1.05221457990015,1.,3.80095039790678));
#49676=CARTESIAN_POINT('Ctrl Pts',(-1.04810913267641,1.,3.79459440308793));
#49677=CARTESIAN_POINT('Ctrl Pts',(-1.04404924374426,1.,3.78821910787195));
#49678=CARTESIAN_POINT('Ctrl Pts',(-1.04003862055804,1.,3.78183535008192));
#49679=CARTESIAN_POINT('Ctrl Pts',(-1.03608074678013,1.,3.77545283140445));
#49680=CARTESIAN_POINT('Ctrl Pts',(-1.0321778660492,1.,3.76907609832522));
#49681=CARTESIAN_POINT('Ctrl Pts',(-1.02833014458181,1.,3.76270122291232));
#49682=CARTESIAN_POINT('Ctrl Pts',(-1.0245342944466,1.,3.75631037456194));
#49683=CARTESIAN_POINT('Ctrl Pts',(-1.02078510487428,1.,3.74987777155834));
#49684=CARTESIAN_POINT('Ctrl Pts',(-1.01707794311079,1.,3.74337942504959));
#49685=CARTESIAN_POINT('Ctrl Pts',(-1.01341114319903,1.,3.73680245055734));
#49686=CARTESIAN_POINT('Ctrl Pts',(-1.00978798539496,1.,3.73015276704426));
#49687=CARTESIAN_POINT('Ctrl Pts',(-1.0062200073571,1.,3.72346803750595));
#49688=CARTESIAN_POINT('Ctrl Pts',(-1.00272423396822,1.,3.71680667125118));
#49689=CARTESIAN_POINT('Ctrl Pts',(-0.999317260756531,1.,3.71022439713938));
#49690=CARTESIAN_POINT('Ctrl Pts',(-0.996009819772518,1.,3.70375282282138));
#49691=CARTESIAN_POINT('Ctrl Pts',(-0.99280221833201,1.,3.69738123415662));
#49692=CARTESIAN_POINT('Ctrl Pts',(-0.989676715398558,1.,3.69102682138846));
#49693=CARTESIAN_POINT('Ctrl Pts',(-0.986602639863838,1.,3.68455317926068));
#49694=CARTESIAN_POINT('Ctrl Pts',(-0.983550791470419,1.,3.67782408841715));
#49695=CARTESIAN_POINT('Ctrl Pts',(-0.980505922458267,1.,3.67074983340361));
#49696=CARTESIAN_POINT('Ctrl Pts',(-0.977478312751618,1.,3.66333049637475));
#49697=CARTESIAN_POINT('Ctrl Pts',(-0.974519971354848,1.,3.65571576735126));
#49698=CARTESIAN_POINT('Ctrl Pts',(-0.971722122061341,1.,3.64819756447455));
#49699=CARTESIAN_POINT('Ctrl Pts',(-0.969195124675866,1.,3.64113946505766));
#49700=CARTESIAN_POINT('Ctrl Pts',(-0.967052554541386,1.,3.63492122081143));
#49701=CARTESIAN_POINT('Ctrl Pts',(-0.965395153165293,1.,3.62988252139846));
#49702=CARTESIAN_POINT('Ctrl Pts',(-0.964373850166457,1.,3.62652618145335));
#49703=CARTESIAN_POINT('Ctrl Pts',(-0.963957782642843,1.,3.62489305727662));
#49704=CARTESIAN_POINT('Ctrl Pts',(-0.963861297423241,1.,3.62424461507588));
#49705=CARTESIAN_POINT('Ctrl Pts',(-0.963880158555582,1.,3.6240482887845));
#49706=CARTESIAN_POINT('Ctrl Pts',(-0.963899035117249,1.,3.62400312501245));
#49707=CARTESIAN_POINT('',(-1.22531898815164,0.,4.01728681790024));
#49708=CARTESIAN_POINT('Ctrl Pts',(-1.35022972712301,-1.,3.49848248301936));
#49709=CARTESIAN_POINT('Ctrl Pts',(-1.35022972712301,1.,3.49848248301936));
#49710=CARTESIAN_POINT('Ctrl Pts',(-1.35026426118402,-1.,3.4984026005375));
#49711=CARTESIAN_POINT('Ctrl Pts',(-1.35026426118402,1.,3.4984026005375));
#49712=CARTESIAN_POINT('Ctrl Pts',(-1.35037650303019,-1.,3.49840357193736));
#49713=CARTESIAN_POINT('Ctrl Pts',(-1.35037650303019,1.,3.49840357193736));
#49714=CARTESIAN_POINT('Ctrl Pts',(-1.35067437417483,-1.,3.49888720257132));
#49715=CARTESIAN_POINT('Ctrl Pts',(-1.35067437417483,1.,3.49888720257132));
#49716=CARTESIAN_POINT('Ctrl Pts',(-1.3513307633124,-1.,3.5004970706414));
#49717=CARTESIAN_POINT('Ctrl Pts',(-1.3513307633124,1.,3.5004970706414));
#49718=CARTESIAN_POINT('Ctrl Pts',(-1.35257032843486,-1.,3.50408168106261));
#49719=CARTESIAN_POINT('Ctrl Pts',(-1.35257032843486,1.,3.50408168106261));
#49720=CARTESIAN_POINT('Ctrl Pts',(-1.35419113575956,-1.,3.50913227059999));
#49721=CARTESIAN_POINT('Ctrl Pts',(-1.35419113575956,1.,3.50913227059999));
#49722=CARTESIAN_POINT('Ctrl Pts',(-1.35611275237152,-1.,3.51542230699556));
#49723=CARTESIAN_POINT('Ctrl Pts',(-1.35611275237152,1.,3.51542230699556));
#49724=CARTESIAN_POINT('Ctrl Pts',(-1.35821701528836,-1.,3.52261776116748));
#49725=CARTESIAN_POINT('Ctrl Pts',(-1.35821701528836,1.,3.52261776116748));
#49726=CARTESIAN_POINT('Ctrl Pts',(-1.36037259643734,-1.,3.530344649616));
#49727=CARTESIAN_POINT('Ctrl Pts',(-1.36037259643734,1.,3.530344649616));
#49728=CARTESIAN_POINT('Ctrl Pts',(-1.36245507339307,-1.,3.53824396424961));
#49729=CARTESIAN_POINT('Ctrl Pts',(-1.36245507339307,1.,3.53824396424961));
#49730=CARTESIAN_POINT('Ctrl Pts',(-1.36436666257598,-1.,3.54602591832973));
#49731=CARTESIAN_POINT('Ctrl Pts',(-1.36436666257598,1.,3.54602591832973));
#49732=CARTESIAN_POINT('Ctrl Pts',(-1.3660614545677,-1.,3.55353883995949));
#49733=CARTESIAN_POINT('Ctrl Pts',(-1.3660614545677,1.,3.55353883995949));
#49734=CARTESIAN_POINT('Ctrl Pts',(-1.36754771771233,-1.,3.56077662028649));
#49735=CARTESIAN_POINT('Ctrl Pts',(-1.36754771771233,1.,3.56077662028649));
#49736=CARTESIAN_POINT('Ctrl Pts',(-1.36886584973389,-1.,3.5678208030466));
#49737=CARTESIAN_POINT('Ctrl Pts',(-1.36886584973389,1.,3.5678208030466));
#49738=CARTESIAN_POINT('Ctrl Pts',(-1.37007229485659,-1.,3.57479875549486));
#49739=CARTESIAN_POINT('Ctrl Pts',(-1.37007229485659,1.,3.57479875549486));
#49740=CARTESIAN_POINT('Ctrl Pts',(-1.37122241663062,-1.,3.58183885982715));
#49741=CARTESIAN_POINT('Ctrl Pts',(-1.37122241663062,1.,3.58183885982715));
#49742=CARTESIAN_POINT('Ctrl Pts',(-1.37235053660976,-1.,3.58901853846365));
#49743=CARTESIAN_POINT('Ctrl Pts',(-1.37235053660976,1.,3.58901853846365));
#49744=CARTESIAN_POINT('Ctrl Pts',(-1.37346320103157,-1.,3.59634627869048));
#49745=CARTESIAN_POINT('Ctrl Pts',(-1.37346320103157,1.,3.59634627869048));
#49746=CARTESIAN_POINT('Ctrl Pts',(-1.37455051379623,-1.,3.60379020123988));
#49747=CARTESIAN_POINT('Ctrl Pts',(-1.37455051379623,1.,3.60379020123988));
#49748=CARTESIAN_POINT('Ctrl Pts',(-1.37559314436634,-1.,3.61129546591064));
#49749=CARTESIAN_POINT('Ctrl Pts',(-1.37559314436634,1.,3.61129546591064));
#49750=CARTESIAN_POINT('Ctrl Pts',(-1.37657053403107,-1.,3.6188048116042));
#49751=CARTESIAN_POINT('Ctrl Pts',(-1.37657053403107,1.,3.6188048116042));
#49752=CARTESIAN_POINT('Ctrl Pts',(-1.37746987919881,-1.,3.62628098665145));
#49753=CARTESIAN_POINT('Ctrl Pts',(-1.37746987919881,1.,3.62628098665145));
#49754=CARTESIAN_POINT('Ctrl Pts',(-1.37829035457339,-1.,3.63371727442486));
#49755=CARTESIAN_POINT('Ctrl Pts',(-1.37829035457339,1.,3.63371727442486));
#49756=CARTESIAN_POINT('Ctrl Pts',(-1.37903818567359,-1.,3.64112507791141));
#49757=CARTESIAN_POINT('Ctrl Pts',(-1.37903818567359,1.,3.64112507791141));
#49758=CARTESIAN_POINT('Ctrl Pts',(-1.37972372481603,-1.,3.64852652756456));
#49759=CARTESIAN_POINT('Ctrl Pts',(-1.37972372481603,1.,3.64852652756456));
#49760=CARTESIAN_POINT('Ctrl Pts',(-1.38035791051213,-1.,3.6559455440439));
#49761=CARTESIAN_POINT('Ctrl Pts',(-1.38035791051213,1.,3.6559455440439));
#49762=CARTESIAN_POINT('Ctrl Pts',(-1.38094856333552,-1.,3.66339848520857));
#49763=CARTESIAN_POINT('Ctrl Pts',(-1.38094856333552,1.,3.66339848520857));
#49764=CARTESIAN_POINT('Ctrl Pts',(-1.38149812653868,-1.,3.67088843112262));
#49765=CARTESIAN_POINT('Ctrl Pts',(-1.38149812653868,1.,3.67088843112262));
#49766=CARTESIAN_POINT('Ctrl Pts',(-1.3820057429062,-1.,3.67841038482414));
#49767=CARTESIAN_POINT('Ctrl Pts',(-1.3820057429062,1.,3.67841038482414));
#49768=CARTESIAN_POINT('Ctrl Pts',(-1.38246852827182,-1.,3.68595444983837));
#49769=CARTESIAN_POINT('Ctrl Pts',(-1.38246852827182,1.,3.68595444983837));
#49770=CARTESIAN_POINT('Ctrl Pts',(-1.38288311171651,-1.,3.69350967899526));
#49771=CARTESIAN_POINT('Ctrl Pts',(-1.38288311171651,1.,3.69350967899526));
#49772=CARTESIAN_POINT('Ctrl Pts',(-1.38324717612865,-1.,3.701067921679));
#49773=CARTESIAN_POINT('Ctrl Pts',(-1.38324717612865,1.,3.701067921679));
#49774=CARTESIAN_POINT('Ctrl Pts',(-1.38356065402124,-1.,3.70862680753347));
#49775=CARTESIAN_POINT('Ctrl Pts',(-1.38356065402124,1.,3.70862680753347));
#49776=CARTESIAN_POINT('Ctrl Pts',(-1.38382489984586,-1.,3.7161876605181));
#49777=CARTESIAN_POINT('Ctrl Pts',(-1.38382489984586,1.,3.7161876605181));
#49778=CARTESIAN_POINT('Ctrl Pts',(-1.3840421342895,-1.,3.72375409358803));
#49779=CARTESIAN_POINT('Ctrl Pts',(-1.3840421342895,1.,3.72375409358803));
#49780=CARTESIAN_POINT('Ctrl Pts',(-1.38421479111531,-1.,3.73133035859282));
#49781=CARTESIAN_POINT('Ctrl Pts',(-1.38421479111531,1.,3.73133035859282));
#49782=CARTESIAN_POINT('Ctrl Pts',(-1.38434489156458,-1.,3.73891976418104));
#49783=CARTESIAN_POINT('Ctrl Pts',(-1.38434489156458,1.,3.73891976418104));
#49784=CARTESIAN_POINT('Ctrl Pts',(-1.38443344984394,-1.,3.74652317167876));
#49785=CARTESIAN_POINT('Ctrl Pts',(-1.38443344984394,1.,3.74652317167876));
#49786=CARTESIAN_POINT('Ctrl Pts',(-1.38448077997163,-1.,3.7541397631875));
#49787=CARTESIAN_POINT('Ctrl Pts',(-1.38448077997163,1.,3.7541397631875));
#49788=CARTESIAN_POINT('Ctrl Pts',(-1.3844867525335,-1.,3.76176768271367));
#49789=CARTESIAN_POINT('Ctrl Pts',(-1.3844867525335,1.,3.76176768271367));
#49790=CARTESIAN_POINT('Ctrl Pts',(-1.38445107339518,-1.,3.76940473185779));
#49791=CARTESIAN_POINT('Ctrl Pts',(-1.38445107339518,1.,3.76940473185779));
#49792=CARTESIAN_POINT('Ctrl Pts',(-1.38437354551428,-1.,3.77704902230418));
#49793=CARTESIAN_POINT('Ctrl Pts',(-1.38437354551428,1.,3.77704902230418));
#49794=CARTESIAN_POINT('Ctrl Pts',(-1.38425435883756,-1.,3.78469969805082));
#49795=CARTESIAN_POINT('Ctrl Pts',(-1.38425435883756,1.,3.78469969805082));
#49796=CARTESIAN_POINT('Ctrl Pts',(-1.38409399694566,-1.,3.79235669640841));
#49797=CARTESIAN_POINT('Ctrl Pts',(-1.38409399694566,1.,3.79235669640841));
#49798=CARTESIAN_POINT('Ctrl Pts',(-1.38389311766682,-1.,3.80002044322111));
#49799=CARTESIAN_POINT('Ctrl Pts',(-1.38389311766682,1.,3.80002044322111));
#49800=CARTESIAN_POINT('Ctrl Pts',(-1.3836524404622,-1.,3.80769156398411));
#49801=CARTESIAN_POINT('Ctrl Pts',(-1.3836524404622,1.,3.80769156398411));
#49802=CARTESIAN_POINT('Ctrl Pts',(-1.38337263902782,-1.,3.81537060817811));
#49803=CARTESIAN_POINT('Ctrl Pts',(-1.38337263902782,1.,3.81537060817811));
#49804=CARTESIAN_POINT('Ctrl Pts',(-1.38305421262763,-1.,3.82305771743829));
#49805=CARTESIAN_POINT('Ctrl Pts',(-1.38305421262763,1.,3.82305771743829));
#49806=CARTESIAN_POINT('Ctrl Pts',(-1.38269750245138,-1.,3.8307526698229));
#49807=CARTESIAN_POINT('Ctrl Pts',(-1.38269750245138,1.,3.8307526698229));
#49808=CARTESIAN_POINT('Ctrl Pts',(-1.38230274828822,-1.,3.83845502790746));
#49809=CARTESIAN_POINT('Ctrl Pts',(-1.38230274828822,1.,3.83845502790746));
#49810=CARTESIAN_POINT('Ctrl Pts',(-1.38187013346109,-1.,3.84616425605764));
#49811=CARTESIAN_POINT('Ctrl Pts',(-1.38187013346109,1.,3.84616425605764));
#49812=CARTESIAN_POINT('Ctrl Pts',(-1.38139983115049,-1.,3.85387983979481));
#49813=CARTESIAN_POINT('Ctrl Pts',(-1.38139983115049,1.,3.85387983979481));
#49814=CARTESIAN_POINT('Ctrl Pts',(-1.38089205992989,-1.,3.86160143043959));
#49815=CARTESIAN_POINT('Ctrl Pts',(-1.38089205992989,1.,3.86160143043959));
#49816=CARTESIAN_POINT('Ctrl Pts',(-1.38034709213014,-1.,3.86932885813068));
#49817=CARTESIAN_POINT('Ctrl Pts',(-1.38034709213014,1.,3.86932885813068));
#49818=CARTESIAN_POINT('Ctrl Pts',(-1.37976523097073,-1.,3.87706205830532));
#49819=CARTESIAN_POINT('Ctrl Pts',(-1.37976523097073,1.,3.87706205830532));
#49820=CARTESIAN_POINT('Ctrl Pts',(-1.37914679719383,-1.,3.88480102249277));
#49821=CARTESIAN_POINT('Ctrl Pts',(-1.37914679719383,1.,3.88480102249277));
#49822=CARTESIAN_POINT('Ctrl Pts',(-1.3784921128802,-1.,3.89254574338496));
#49823=CARTESIAN_POINT('Ctrl Pts',(-1.3784921128802,1.,3.89254574338496));
#49824=CARTESIAN_POINT('Ctrl Pts',(-1.37780148512792,-1.,3.90029615196727));
#49825=CARTESIAN_POINT('Ctrl Pts',(-1.37780148512792,1.,3.90029615196727));
#49826=CARTESIAN_POINT('Ctrl Pts',(-1.3770751963402,-1.,3.90805209523486));
#49827=CARTESIAN_POINT('Ctrl Pts',(-1.3770751963402,1.,3.90805209523486));
#49828=CARTESIAN_POINT('Ctrl Pts',(-1.37631350505797,-1.,3.91581337462644));
#49829=CARTESIAN_POINT('Ctrl Pts',(-1.37631350505797,1.,3.91581337462644));
#49830=CARTESIAN_POINT('Ctrl Pts',(-1.37551664448242,-1.,3.92357976987672));
#49831=CARTESIAN_POINT('Ctrl Pts',(-1.37551664448242,1.,3.92357976987672));
#49832=CARTESIAN_POINT('Ctrl Pts',(-1.37468482215751,-1.,3.93135106761844));
#49833=CARTESIAN_POINT('Ctrl Pts',(-1.37468482215751,1.,3.93135106761844));
#49834=CARTESIAN_POINT('Ctrl Pts',(-1.37381821967165,-1.,3.93912709040818));
#49835=CARTESIAN_POINT('Ctrl Pts',(-1.37381821967165,1.,3.93912709040818));
#49836=CARTESIAN_POINT('Ctrl Pts',(-1.37291699202807,-1.,3.94690771785133));
#49837=CARTESIAN_POINT('Ctrl Pts',(-1.37291699202807,1.,3.94690771785133));
#49838=CARTESIAN_POINT('Ctrl Pts',(-1.37198126432386,-1.,3.95469287280914));
#49839=CARTESIAN_POINT('Ctrl Pts',(-1.37198126432386,1.,3.95469287280914));
#49840=CARTESIAN_POINT('Ctrl Pts',(-1.3712051561502,-1.,3.96092458506535));
#49841=CARTESIAN_POINT('Ctrl Pts',(-1.3712051561502,1.,3.96092458506535));
#49842=CARTESIAN_POINT('Ctrl Pts',(-1.37060761745635,-1.,3.96560037974645));
#49843=CARTESIAN_POINT('Ctrl Pts',(-1.37060761745635,1.,3.96560037974645));
#49844=CARTESIAN_POINT('Ctrl Pts',(-1.37020239094614,-1.,3.9687184694131));
#49845=CARTESIAN_POINT('Ctrl Pts',(-1.37020239094614,1.,3.9687184694131));
#49846=CARTESIAN_POINT('Ctrl Pts',(-1.36999806084572,-1.,3.97027773754922));
#49847=CARTESIAN_POINT('Ctrl Pts',(-1.36999806084572,1.,3.97027773754922));
#49848=CARTESIAN_POINT('',(-1.35032489087101,1.,3.4984457533445));
#49849=CARTESIAN_POINT('Ctrl Pts',(-1.35032489087101,-1.,3.4984457533445));
#49850=CARTESIAN_POINT('Ctrl Pts',(-1.35032489087101,-0.666666666666667,
3.4984457533445));
#49851=CARTESIAN_POINT('Ctrl Pts',(-1.35032489087101,-0.333333333333333,
3.4984457533445));
#49852=CARTESIAN_POINT('Ctrl Pts',(-1.35032489087101,0.333333333333333,
3.4984457533445));
#49853=CARTESIAN_POINT('Ctrl Pts',(-1.35032489087101,0.666666666666667,
3.4984457533445));
#49854=CARTESIAN_POINT('Ctrl Pts',(-1.35032489087101,1.,3.4984457533445));
#49855=CARTESIAN_POINT('',(-1.36999806084572,1.,3.97027773754922));
#49856=CARTESIAN_POINT('',(-1.36999806084572,0.,3.97027773754922));
#49857=CARTESIAN_POINT('Ctrl Pts',(-1.35032489087101,1.,3.4984457533445));
#49858=CARTESIAN_POINT('Ctrl Pts',(-1.35036670892966,1.,3.49847119623846));
#49859=CARTESIAN_POINT('Ctrl Pts',(-1.35049736560527,1.,3.49861894124827));
#49860=CARTESIAN_POINT('Ctrl Pts',(-1.35080045218587,1.,3.49920025459723));
#49861=CARTESIAN_POINT('Ctrl Pts',(-1.35142377279517,1.,3.5007660381649));
#49862=CARTESIAN_POINT('Ctrl Pts',(-1.35257032843486,1.,3.50408168106261));
#49863=CARTESIAN_POINT('Ctrl Pts',(-1.35419113575956,1.,3.50913227059999));
#49864=CARTESIAN_POINT('Ctrl Pts',(-1.35611275237152,1.,3.51542230699556));
#49865=CARTESIAN_POINT('Ctrl Pts',(-1.35821701528836,1.,3.52261776116748));
#49866=CARTESIAN_POINT('Ctrl Pts',(-1.36037259643734,1.,3.530344649616));
#49867=CARTESIAN_POINT('Ctrl Pts',(-1.36245507339307,1.,3.53824396424961));
#49868=CARTESIAN_POINT('Ctrl Pts',(-1.36436666257598,1.,3.54602591832973));
#49869=CARTESIAN_POINT('Ctrl Pts',(-1.3660614545677,1.,3.55353883995949));
#49870=CARTESIAN_POINT('Ctrl Pts',(-1.36754771771233,1.,3.56077662028649));
#49871=CARTESIAN_POINT('Ctrl Pts',(-1.36886584973389,1.,3.5678208030466));
#49872=CARTESIAN_POINT('Ctrl Pts',(-1.37007229485659,1.,3.57479875549486));
#49873=CARTESIAN_POINT('Ctrl Pts',(-1.37122241663062,1.,3.58183885982715));
#49874=CARTESIAN_POINT('Ctrl Pts',(-1.37235053660976,1.,3.58901853846365));
#49875=CARTESIAN_POINT('Ctrl Pts',(-1.37346320103157,1.,3.59634627869048));
#49876=CARTESIAN_POINT('Ctrl Pts',(-1.37455051379623,1.,3.60379020123988));
#49877=CARTESIAN_POINT('Ctrl Pts',(-1.37559314436634,1.,3.61129546591064));
#49878=CARTESIAN_POINT('Ctrl Pts',(-1.37657053403107,1.,3.6188048116042));
#49879=CARTESIAN_POINT('Ctrl Pts',(-1.37746987919881,1.,3.62628098665145));
#49880=CARTESIAN_POINT('Ctrl Pts',(-1.37829035457339,1.,3.63371727442486));
#49881=CARTESIAN_POINT('Ctrl Pts',(-1.37903818567359,1.,3.64112507791141));
#49882=CARTESIAN_POINT('Ctrl Pts',(-1.37972372481603,1.,3.64852652756456));
#49883=CARTESIAN_POINT('Ctrl Pts',(-1.38035791051213,1.,3.6559455440439));
#49884=CARTESIAN_POINT('Ctrl Pts',(-1.38094856333552,1.,3.66339848520857));
#49885=CARTESIAN_POINT('Ctrl Pts',(-1.38149812653868,1.,3.67088843112262));
#49886=CARTESIAN_POINT('Ctrl Pts',(-1.3820057429062,1.,3.67841038482414));
#49887=CARTESIAN_POINT('Ctrl Pts',(-1.38246852827182,1.,3.68595444983837));
#49888=CARTESIAN_POINT('Ctrl Pts',(-1.38288311171651,1.,3.69350967899526));
#49889=CARTESIAN_POINT('Ctrl Pts',(-1.38324717612865,1.,3.701067921679));
#49890=CARTESIAN_POINT('Ctrl Pts',(-1.38356065402124,1.,3.70862680753347));
#49891=CARTESIAN_POINT('Ctrl Pts',(-1.38382489984586,1.,3.7161876605181));
#49892=CARTESIAN_POINT('Ctrl Pts',(-1.3840421342895,1.,3.72375409358803));
#49893=CARTESIAN_POINT('Ctrl Pts',(-1.38421479111531,1.,3.73133035859282));
#49894=CARTESIAN_POINT('Ctrl Pts',(-1.38434489156458,1.,3.73891976418104));
#49895=CARTESIAN_POINT('Ctrl Pts',(-1.38443344984394,1.,3.74652317167876));
#49896=CARTESIAN_POINT('Ctrl Pts',(-1.38448077997163,1.,3.7541397631875));
#49897=CARTESIAN_POINT('Ctrl Pts',(-1.3844867525335,1.,3.76176768271367));
#49898=CARTESIAN_POINT('Ctrl Pts',(-1.38445107339518,1.,3.76940473185779));
#49899=CARTESIAN_POINT('Ctrl Pts',(-1.38437354551428,1.,3.77704902230418));
#49900=CARTESIAN_POINT('Ctrl Pts',(-1.38425435883756,1.,3.78469969805082));
#49901=CARTESIAN_POINT('Ctrl Pts',(-1.38409399694566,1.,3.79235669640841));
#49902=CARTESIAN_POINT('Ctrl Pts',(-1.38389311766682,1.,3.80002044322111));
#49903=CARTESIAN_POINT('Ctrl Pts',(-1.3836524404622,1.,3.80769156398411));
#49904=CARTESIAN_POINT('Ctrl Pts',(-1.38337263902782,1.,3.81537060817811));
#49905=CARTESIAN_POINT('Ctrl Pts',(-1.38305421262763,1.,3.82305771743829));
#49906=CARTESIAN_POINT('Ctrl Pts',(-1.38269750245138,1.,3.8307526698229));
#49907=CARTESIAN_POINT('Ctrl Pts',(-1.38230274828822,1.,3.83845502790746));
#49908=CARTESIAN_POINT('Ctrl Pts',(-1.38187013346109,1.,3.84616425605764));
#49909=CARTESIAN_POINT('Ctrl Pts',(-1.38139983115049,1.,3.85387983979481));
#49910=CARTESIAN_POINT('Ctrl Pts',(-1.38089205992989,1.,3.86160143043959));
#49911=CARTESIAN_POINT('Ctrl Pts',(-1.38034709213014,1.,3.86932885813068));
#49912=CARTESIAN_POINT('Ctrl Pts',(-1.37976523097073,1.,3.87706205830532));
#49913=CARTESIAN_POINT('Ctrl Pts',(-1.37914679719383,1.,3.88480102249277));
#49914=CARTESIAN_POINT('Ctrl Pts',(-1.3784921128802,1.,3.89254574338496));
#49915=CARTESIAN_POINT('Ctrl Pts',(-1.37780148512792,1.,3.90029615196727));
#49916=CARTESIAN_POINT('Ctrl Pts',(-1.3770751963402,1.,3.90805209523486));
#49917=CARTESIAN_POINT('Ctrl Pts',(-1.37631350505797,1.,3.91581337462644));
#49918=CARTESIAN_POINT('Ctrl Pts',(-1.37551664448242,1.,3.92357976987672));
#49919=CARTESIAN_POINT('Ctrl Pts',(-1.37468482215751,1.,3.93135106761844));
#49920=CARTESIAN_POINT('Ctrl Pts',(-1.37381821967165,1.,3.93912709040818));
#49921=CARTESIAN_POINT('Ctrl Pts',(-1.37291699202807,1.,3.94690771785133));
#49922=CARTESIAN_POINT('Ctrl Pts',(-1.37198126432386,1.,3.95469287280914));
#49923=CARTESIAN_POINT('Ctrl Pts',(-1.3712051561502,1.,3.96092458506535));
#49924=CARTESIAN_POINT('Ctrl Pts',(-1.37060761745635,1.,3.96560037974645));
#49925=CARTESIAN_POINT('Ctrl Pts',(-1.37020239094614,1.,3.9687184694131));
#49926=CARTESIAN_POINT('Ctrl Pts',(-1.36999806084572,1.,3.97027773754922));
#49927=CARTESIAN_POINT('Origin',(-1.36999806084572,0.,3.97027773754922));
#49928=CARTESIAN_POINT('',(-1.22531898815164,1.,4.01728681790024));
#49929=CARTESIAN_POINT('Origin',(0.,0.,0.));
#49930=CARTESIAN_POINT('',(-1.51895082866166,1.,3.42859860294378));
#49931=CARTESIAN_POINT('Origin',(0.,1.,0.));
#49932=CARTESIAN_POINT('Ctrl Pts',(-1.51895082866166,1.,3.42859860294378));
#49933=CARTESIAN_POINT('Ctrl Pts',(-1.51895082866166,0.666666666666667,
3.42859860294378));
#49934=CARTESIAN_POINT('Ctrl Pts',(-1.51895082866166,0.333333333333333,
3.42859860294378));
#49935=CARTESIAN_POINT('Ctrl Pts',(-1.51895082866166,-0.333333333333333,
3.42859860294378));
#49936=CARTESIAN_POINT('Ctrl Pts',(-1.51895082866166,-0.666666666666667,
3.42859860294378));
#49937=CARTESIAN_POINT('Ctrl Pts',(-1.51895082866166,-1.,3.42859860294378));
#49938=CARTESIAN_POINT('Ctrl Pts',(-1.83867539237861,-1.,3.77614523045147));
#49939=CARTESIAN_POINT('Ctrl Pts',(-1.83867539237861,1.,3.77614523045147));
#49940=CARTESIAN_POINT('Ctrl Pts',(-1.83742834010821,-1.,3.77518714458232));
#49941=CARTESIAN_POINT('Ctrl Pts',(-1.83742834010821,1.,3.77518714458232));
#49942=CARTESIAN_POINT('Ctrl Pts',(-1.83493697935064,-1.,3.77326886065484));
#49943=CARTESIAN_POINT('Ctrl Pts',(-1.83493697935064,1.,3.77326886065484));
#49944=CARTESIAN_POINT('Ctrl Pts',(-1.83120816956515,-1.,3.77038509819777));
#49945=CARTESIAN_POINT('Ctrl Pts',(-1.83120816956515,1.,3.77038509819777));
#49946=CARTESIAN_POINT('Ctrl Pts',(-1.82625289221933,-1.,3.76652740355856));
#49947=CARTESIAN_POINT('Ctrl Pts',(-1.82625289221933,1.,3.76652740355856));
#49948=CARTESIAN_POINT('Ctrl Pts',(-1.82008629694924,-1.,3.76168412709652));
#49949=CARTESIAN_POINT('Ctrl Pts',(-1.82008629694924,1.,3.76168412709652));
#49950=CARTESIAN_POINT('Ctrl Pts',(-1.81394729834032,-1.,3.75681965683995));
#49951=CARTESIAN_POINT('Ctrl Pts',(-1.81394729834032,1.,3.75681965683995));
#49952=CARTESIAN_POINT('Ctrl Pts',(-1.80783603939662,-1.,3.75193395888069));
#49953=CARTESIAN_POINT('Ctrl Pts',(-1.80783603939662,1.,3.75193395888069));
#49954=CARTESIAN_POINT('Ctrl Pts',(-1.80175271485519,-1.,3.74702700874954));
#49955=CARTESIAN_POINT('Ctrl Pts',(-1.80175271485519,1.,3.74702700874954));
#49956=CARTESIAN_POINT('Ctrl Pts',(-1.79569757859041,-1.,3.74209880351667));
#49957=CARTESIAN_POINT('Ctrl Pts',(-1.79569757859041,1.,3.74209880351667));
#49958=CARTESIAN_POINT('Ctrl Pts',(-1.78967092823139,-1.,3.73714934729962));
#49959=CARTESIAN_POINT('Ctrl Pts',(-1.78967092823139,1.,3.73714934729962));
#49960=CARTESIAN_POINT('Ctrl Pts',(-1.78367308442682,-1.,3.73217863095022));
#49961=CARTESIAN_POINT('Ctrl Pts',(-1.78367308442682,1.,3.73217863095022));
#49962=CARTESIAN_POINT('Ctrl Pts',(-1.77770437039606,-1.,3.72718661205504));
#49963=CARTESIAN_POINT('Ctrl Pts',(-1.77770437039606,1.,3.72718661205504));
#49964=CARTESIAN_POINT('Ctrl Pts',(-1.77176509401846,-1.,3.72217319911429));
#49965=CARTESIAN_POINT('Ctrl Pts',(-1.77176509401846,1.,3.72217319911429));
#49966=CARTESIAN_POINT('Ctrl Pts',(-1.76585552124549,-1.,3.71713822377675));
#49967=CARTESIAN_POINT('Ctrl Pts',(-1.76585552124549,1.,3.71713822377675));
#49968=CARTESIAN_POINT('Ctrl Pts',(-1.75997588499021,-1.,3.71208146346454));
#49969=CARTESIAN_POINT('Ctrl Pts',(-1.75997588499021,1.,3.71208146346454));
#49970=CARTESIAN_POINT('Ctrl Pts',(-1.75412641804148,-1.,3.70700269736876));
#49971=CARTESIAN_POINT('Ctrl Pts',(-1.75412641804148,1.,3.70700269736876));
#49972=CARTESIAN_POINT('Ctrl Pts',(-1.74830738046092,-1.,3.70190175673422));
#49973=CARTESIAN_POINT('Ctrl Pts',(-1.74830738046092,1.,3.70190175673422));
#49974=CARTESIAN_POINT('Ctrl Pts',(-1.74251908492589,-1.,3.6967785691046));
#49975=CARTESIAN_POINT('Ctrl Pts',(-1.74251908492589,1.,3.6967785691046));
#49976=CARTESIAN_POINT('Ctrl Pts',(-1.73676193254493,-1.,3.69163322647906));
#49977=CARTESIAN_POINT('Ctrl Pts',(-1.73676193254493,1.,3.69163322647906));
#49978=CARTESIAN_POINT('Ctrl Pts',(-1.73103640956647,-1.,3.68646597019188));
#49979=CARTESIAN_POINT('Ctrl Pts',(-1.73103640956647,1.,3.68646597019188));
#49980=CARTESIAN_POINT('Ctrl Pts',(-1.72534302437003,-1.,3.68127704936472));
#49981=CARTESIAN_POINT('Ctrl Pts',(-1.72534302437003,1.,3.68127704936472));
#49982=CARTESIAN_POINT('Ctrl Pts',(-1.71968225581787,-1.,3.67606660374665));
#49983=CARTESIAN_POINT('Ctrl Pts',(-1.71968225581787,1.,3.67606660374665));
#49984=CARTESIAN_POINT('Ctrl Pts',(-1.71405450210392,-1.,3.67083454901629));
#49985=CARTESIAN_POINT('Ctrl Pts',(-1.71405450210392,1.,3.67083454901629));
#49986=CARTESIAN_POINT('Ctrl Pts',(-1.70846001610983,-1.,3.6655804319893));
#49987=CARTESIAN_POINT('Ctrl Pts',(-1.70846001610983,1.,3.6655804319893));
#49988=CARTESIAN_POINT('Ctrl Pts',(-1.70289888566904,-1.,3.6603033877491));
#49989=CARTESIAN_POINT('Ctrl Pts',(-1.70289888566904,1.,3.6603033877491));
#49990=CARTESIAN_POINT('Ctrl Pts',(-1.69737117722559,-1.,3.65500246526798));
#49991=CARTESIAN_POINT('Ctrl Pts',(-1.69737117722559,1.,3.65500246526798));
#49992=CARTESIAN_POINT('Ctrl Pts',(-1.691877054817,-1.,3.64967689827393));
#49993=CARTESIAN_POINT('Ctrl Pts',(-1.691877054817,1.,3.64967689827393));
#49994=CARTESIAN_POINT('Ctrl Pts',(-1.68641690471455,-1.,3.64432638915199));
#49995=CARTESIAN_POINT('Ctrl Pts',(-1.68641690471455,1.,3.64432638915199));
#49996=CARTESIAN_POINT('Ctrl Pts',(-1.68099146651577,-1.,3.63895140887443));
#49997=CARTESIAN_POINT('Ctrl Pts',(-1.68099146651577,1.,3.63895140887443));
#49998=CARTESIAN_POINT('Ctrl Pts',(-1.67560193613145,-1.,3.63355343201211));
#49999=CARTESIAN_POINT('Ctrl Pts',(-1.67560193613145,1.,3.63355343201211));
#50000=CARTESIAN_POINT('Ctrl Pts',(-1.67024966008037,-1.,3.62813422105257));
#50001=CARTESIAN_POINT('Ctrl Pts',(-1.67024966008037,1.,3.62813422105257));
#50002=CARTESIAN_POINT('Ctrl Pts',(-1.66493585923853,-1.,3.62269517989104));
#50003=CARTESIAN_POINT('Ctrl Pts',(-1.66493585923853,1.,3.62269517989104));
#50004=CARTESIAN_POINT('Ctrl Pts',(-1.65966133399186,-1.,3.61723666482457));
#50005=CARTESIAN_POINT('Ctrl Pts',(-1.65966133399186,1.,3.61723666482457));
#50006=CARTESIAN_POINT('Ctrl Pts',(-1.65442619244327,-1.,3.61175734965129));
#50007=CARTESIAN_POINT('Ctrl Pts',(-1.65442619244327,1.,3.61175734965129));
#50008=CARTESIAN_POINT('Ctrl Pts',(-1.64922952425833,-1.,3.60625346556992));
#50009=CARTESIAN_POINT('Ctrl Pts',(-1.64922952425833,1.,3.60625346556992));
#50010=CARTESIAN_POINT('Ctrl Pts',(-1.6440700438558,-1.,3.6007202851384));
#50011=CARTESIAN_POINT('Ctrl Pts',(-1.6440700438558,1.,3.6007202851384));
#50012=CARTESIAN_POINT('Ctrl Pts',(-1.63894676675349,-1.,3.59515368334887));
#50013=CARTESIAN_POINT('Ctrl Pts',(-1.63894676675349,1.,3.59515368334887));
#50014=CARTESIAN_POINT('Ctrl Pts',(-1.63385971451259,-1.,3.58955176627876));
#50015=CARTESIAN_POINT('Ctrl Pts',(-1.63385971451259,1.,3.58955176627876));
#50016=CARTESIAN_POINT('Ctrl Pts',(-1.62881051550748,-1.,3.5839162577435));
#50017=CARTESIAN_POINT('Ctrl Pts',(-1.62881051550748,1.,3.5839162577435));
#50018=CARTESIAN_POINT('Ctrl Pts',(-1.62380329464851,-1.,3.57825455954405));
#50019=CARTESIAN_POINT('Ctrl Pts',(-1.62380329464851,1.,3.57825455954405));
#50020=CARTESIAN_POINT('Ctrl Pts',(-1.61884340915412,-1.,3.57257679609826));
#50021=CARTESIAN_POINT('Ctrl Pts',(-1.61884340915412,1.,3.57257679609826));
#50022=CARTESIAN_POINT('Ctrl Pts',(-1.61393581747522,-1.,3.56689200468404));
#50023=CARTESIAN_POINT('Ctrl Pts',(-1.61393581747522,1.,3.56689200468404));
#50024=CARTESIAN_POINT('Ctrl Pts',(-1.60908344685459,-1.,3.56120432482986));
#50025=CARTESIAN_POINT('Ctrl Pts',(-1.60908344685459,1.,3.56120432482986));
#50026=CARTESIAN_POINT('Ctrl Pts',(-1.60428584699848,-1.,3.55550985096117));
#50027=CARTESIAN_POINT('Ctrl Pts',(-1.60428584699848,1.,3.55550985096117));
#50028=CARTESIAN_POINT('Ctrl Pts',(-1.59953698113444,-1.,3.54979148634426));
#50029=CARTESIAN_POINT('Ctrl Pts',(-1.59953698113444,1.,3.54979148634426));
#50030=CARTESIAN_POINT('Ctrl Pts',(-1.5948276694975,-1.,3.544024581823));
#50031=CARTESIAN_POINT('Ctrl Pts',(-1.5948276694975,1.,3.544024581823));
#50032=CARTESIAN_POINT('Ctrl Pts',(-1.59014958368725,-1.,3.53818616861045));
#50033=CARTESIAN_POINT('Ctrl Pts',(-1.59014958368725,1.,3.53818616861045));
#50034=CARTESIAN_POINT('Ctrl Pts',(-1.58549906268083,-1.,3.53226378147068));
#50035=CARTESIAN_POINT('Ctrl Pts',(-1.58549906268083,1.,3.53226378147068));
#50036=CARTESIAN_POINT('Ctrl Pts',(-1.58088027227856,-1.,3.52626275334899));
#50037=CARTESIAN_POINT('Ctrl Pts',(-1.58088027227856,1.,3.52626275334899));
#50038=CARTESIAN_POINT('Ctrl Pts',(-1.5763104998818,-1.,3.52021847865961));
#50039=CARTESIAN_POINT('Ctrl Pts',(-1.5763104998818,1.,3.52021847865961));
#50040=CARTESIAN_POINT('Ctrl Pts',(-1.57181569799774,-1.,3.51418598431733));
#50041=CARTESIAN_POINT('Ctrl Pts',(-1.57181569799774,1.,3.51418598431733));
#50042=CARTESIAN_POINT('Ctrl Pts',(-1.56742097575041,-1.,3.50821771695427));
#50043=CARTESIAN_POINT('Ctrl Pts',(-1.56742097575041,1.,3.50821771695427));
#50044=CARTESIAN_POINT('Ctrl Pts',(-1.56314187758689,-1.,3.50234321621607));
#50045=CARTESIAN_POINT('Ctrl Pts',(-1.56314187758689,1.,3.50234321621607));
#50046=CARTESIAN_POINT('Ctrl Pts',(-1.55897703097859,-1.,3.49655185179623));
#50047=CARTESIAN_POINT('Ctrl Pts',(-1.55897703097859,1.,3.49655185179623));
#50048=CARTESIAN_POINT('Ctrl Pts',(-1.5548959590107,-1.,3.49076460877317));
#50049=CARTESIAN_POINT('Ctrl Pts',(-1.5548959590107,1.,3.49076460877317));
#50050=CARTESIAN_POINT('Ctrl Pts',(-1.55084702970382,-1.,3.48485155928414));
#50051=CARTESIAN_POINT('Ctrl Pts',(-1.55084702970382,1.,3.48485155928414));
#50052=CARTESIAN_POINT('Ctrl Pts',(-1.54678009290207,-1.,3.47868272898599));
#50053=CARTESIAN_POINT('Ctrl Pts',(-1.54678009290207,1.,3.47868272898599));
#50054=CARTESIAN_POINT('Ctrl Pts',(-1.54266605398152,-1.,3.47217189224576));
#50055=CARTESIAN_POINT('Ctrl Pts',(-1.54266605398152,1.,3.47217189224576));
#50056=CARTESIAN_POINT('Ctrl Pts',(-1.53851507915533,-1.,3.46531752207222));
#50057=CARTESIAN_POINT('Ctrl Pts',(-1.53851507915533,1.,3.46531752207222));
#50058=CARTESIAN_POINT('Ctrl Pts',(-1.53440195378902,-1.,3.45825932955273));
#50059=CARTESIAN_POINT('Ctrl Pts',(-1.53440195378902,1.,3.45825932955273));
#50060=CARTESIAN_POINT('Ctrl Pts',(-1.530462444618,-1.,3.45127136828667));
#50061=CARTESIAN_POINT('Ctrl Pts',(-1.530462444618,1.,3.45127136828667));
#50062=CARTESIAN_POINT('Ctrl Pts',(-1.52686242875717,-1.,3.44469547527));
#50063=CARTESIAN_POINT('Ctrl Pts',(-1.52686242875717,1.,3.44469547527));
#50064=CARTESIAN_POINT('Ctrl Pts',(-1.52377348950429,-1.,3.43888895974182));
#50065=CARTESIAN_POINT('Ctrl Pts',(-1.52377348950429,1.,3.43888895974182));
#50066=CARTESIAN_POINT('Ctrl Pts',(-1.52134826724227,-1.,3.43417156977749));
#50067=CARTESIAN_POINT('Ctrl Pts',(-1.52134826724227,1.,3.43417156977749));
#50068=CARTESIAN_POINT('Ctrl Pts',(-1.51969006980792,-1.,3.43076036253384));
#50069=CARTESIAN_POINT('Ctrl Pts',(-1.51969006980792,1.,3.43076036253384));
#50070=CARTESIAN_POINT('Ctrl Pts',(-1.51901585838879,-1.,3.42915787669388));
#50071=CARTESIAN_POINT('Ctrl Pts',(-1.51901585838879,1.,3.42915787669388));
#50072=CARTESIAN_POINT('Ctrl Pts',(-1.51888450659497,-1.,3.42860527148835));
#50073=CARTESIAN_POINT('Ctrl Pts',(-1.51888450659497,1.,3.42860527148835));
#50074=CARTESIAN_POINT('Ctrl Pts',(-1.51896318668306,-1.,3.42852521763648));
#50075=CARTESIAN_POINT('Ctrl Pts',(-1.51896318668306,1.,3.42852521763648));
#50076=CARTESIAN_POINT('Ctrl Pts',(-1.519044091397,-1.,3.42855728381368));
#50077=CARTESIAN_POINT('Ctrl Pts',(-1.519044091397,1.,3.42855728381368));
#50078=CARTESIAN_POINT('',(-1.83867539237861,1.,3.77614523045147));
#50079=CARTESIAN_POINT('Ctrl Pts',(-1.83867539237861,1.,3.77614523045147));
#50080=CARTESIAN_POINT('Ctrl Pts',(-1.83742834010821,1.,3.77518714458232));
#50081=CARTESIAN_POINT('Ctrl Pts',(-1.83493697935064,1.,3.77326886065484));
#50082=CARTESIAN_POINT('Ctrl Pts',(-1.83120816956515,1.,3.77038509819777));
#50083=CARTESIAN_POINT('Ctrl Pts',(-1.82625289221933,1.,3.76652740355856));
#50084=CARTESIAN_POINT('Ctrl Pts',(-1.82008629694924,1.,3.76168412709652));
#50085=CARTESIAN_POINT('Ctrl Pts',(-1.81394729834032,1.,3.75681965683995));
#50086=CARTESIAN_POINT('Ctrl Pts',(-1.80783603939662,1.,3.75193395888069));
#50087=CARTESIAN_POINT('Ctrl Pts',(-1.80175271485519,1.,3.74702700874954));
#50088=CARTESIAN_POINT('Ctrl Pts',(-1.79569757859041,1.,3.74209880351667));
#50089=CARTESIAN_POINT('Ctrl Pts',(-1.78967092823139,1.,3.73714934729962));
#50090=CARTESIAN_POINT('Ctrl Pts',(-1.78367308442682,1.,3.73217863095022));
#50091=CARTESIAN_POINT('Ctrl Pts',(-1.77770437039606,1.,3.72718661205504));
#50092=CARTESIAN_POINT('Ctrl Pts',(-1.77176509401846,1.,3.72217319911429));
#50093=CARTESIAN_POINT('Ctrl Pts',(-1.76585552124549,1.,3.71713822377675));
#50094=CARTESIAN_POINT('Ctrl Pts',(-1.75997588499021,1.,3.71208146346454));
#50095=CARTESIAN_POINT('Ctrl Pts',(-1.75412641804148,1.,3.70700269736876));
#50096=CARTESIAN_POINT('Ctrl Pts',(-1.74830738046092,1.,3.70190175673422));
#50097=CARTESIAN_POINT('Ctrl Pts',(-1.74251908492589,1.,3.6967785691046));
#50098=CARTESIAN_POINT('Ctrl Pts',(-1.73676193254493,1.,3.69163322647906));
#50099=CARTESIAN_POINT('Ctrl Pts',(-1.73103640956647,1.,3.68646597019188));
#50100=CARTESIAN_POINT('Ctrl Pts',(-1.72534302437003,1.,3.68127704936472));
#50101=CARTESIAN_POINT('Ctrl Pts',(-1.71968225581787,1.,3.67606660374665));
#50102=CARTESIAN_POINT('Ctrl Pts',(-1.71405450210392,1.,3.67083454901629));
#50103=CARTESIAN_POINT('Ctrl Pts',(-1.70846001610983,1.,3.6655804319893));
#50104=CARTESIAN_POINT('Ctrl Pts',(-1.70289888566904,1.,3.6603033877491));
#50105=CARTESIAN_POINT('Ctrl Pts',(-1.69737117722559,1.,3.65500246526798));
#50106=CARTESIAN_POINT('Ctrl Pts',(-1.691877054817,1.,3.64967689827393));
#50107=CARTESIAN_POINT('Ctrl Pts',(-1.68641690471455,1.,3.64432638915199));
#50108=CARTESIAN_POINT('Ctrl Pts',(-1.68099146651577,1.,3.63895140887443));
#50109=CARTESIAN_POINT('Ctrl Pts',(-1.67560193613145,1.,3.63355343201211));
#50110=CARTESIAN_POINT('Ctrl Pts',(-1.67024966008037,1.,3.62813422105257));
#50111=CARTESIAN_POINT('Ctrl Pts',(-1.66493585923853,1.,3.62269517989104));
#50112=CARTESIAN_POINT('Ctrl Pts',(-1.65966133399186,1.,3.61723666482457));
#50113=CARTESIAN_POINT('Ctrl Pts',(-1.65442619244327,1.,3.61175734965129));
#50114=CARTESIAN_POINT('Ctrl Pts',(-1.64922952425833,1.,3.60625346556992));
#50115=CARTESIAN_POINT('Ctrl Pts',(-1.6440700438558,1.,3.6007202851384));
#50116=CARTESIAN_POINT('Ctrl Pts',(-1.63894676675349,1.,3.59515368334887));
#50117=CARTESIAN_POINT('Ctrl Pts',(-1.63385971451259,1.,3.58955176627876));
#50118=CARTESIAN_POINT('Ctrl Pts',(-1.62881051550748,1.,3.5839162577435));
#50119=CARTESIAN_POINT('Ctrl Pts',(-1.62380329464851,1.,3.57825455954405));
#50120=CARTESIAN_POINT('Ctrl Pts',(-1.61884340915412,1.,3.57257679609826));
#50121=CARTESIAN_POINT('Ctrl Pts',(-1.61393581747522,1.,3.56689200468404));
#50122=CARTESIAN_POINT('Ctrl Pts',(-1.60908344685459,1.,3.56120432482986));
#50123=CARTESIAN_POINT('Ctrl Pts',(-1.60428584699848,1.,3.55550985096117));
#50124=CARTESIAN_POINT('Ctrl Pts',(-1.59953698113444,1.,3.54979148634426));
#50125=CARTESIAN_POINT('Ctrl Pts',(-1.5948276694975,1.,3.544024581823));
#50126=CARTESIAN_POINT('Ctrl Pts',(-1.59014958368725,1.,3.53818616861045));
#50127=CARTESIAN_POINT('Ctrl Pts',(-1.58549906268083,1.,3.53226378147068));
#50128=CARTESIAN_POINT('Ctrl Pts',(-1.58088027227856,1.,3.52626275334899));
#50129=CARTESIAN_POINT('Ctrl Pts',(-1.5763104998818,1.,3.52021847865961));
#50130=CARTESIAN_POINT('Ctrl Pts',(-1.57181569799774,1.,3.51418598431733));
#50131=CARTESIAN_POINT('Ctrl Pts',(-1.56742097575041,1.,3.50821771695427));
#50132=CARTESIAN_POINT('Ctrl Pts',(-1.56314187758689,1.,3.50234321621607));
#50133=CARTESIAN_POINT('Ctrl Pts',(-1.55897703097859,1.,3.49655185179623));
#50134=CARTESIAN_POINT('Ctrl Pts',(-1.5548959590107,1.,3.49076460877317));
#50135=CARTESIAN_POINT('Ctrl Pts',(-1.55084702970382,1.,3.48485155928414));
#50136=CARTESIAN_POINT('Ctrl Pts',(-1.54678009290207,1.,3.47868272898599));
#50137=CARTESIAN_POINT('Ctrl Pts',(-1.54266605398152,1.,3.47217189224576));
#50138=CARTESIAN_POINT('Ctrl Pts',(-1.53851507915533,1.,3.46531752207222));
#50139=CARTESIAN_POINT('Ctrl Pts',(-1.53440195378902,1.,3.45825932955273));
#50140=CARTESIAN_POINT('Ctrl Pts',(-1.530462444618,1.,3.45127136828667));
#50141=CARTESIAN_POINT('Ctrl Pts',(-1.52686242875717,1.,3.44469547527));
#50142=CARTESIAN_POINT('Ctrl Pts',(-1.52377348950429,1.,3.43888895974182));
#50143=CARTESIAN_POINT('Ctrl Pts',(-1.52134826724227,1.,3.43417156977749));
#50144=CARTESIAN_POINT('Ctrl Pts',(-1.5198144909343,1.,3.4310163189349));
#50145=CARTESIAN_POINT('Ctrl Pts',(-1.51914806898539,1.,3.42946838852728));
#50146=CARTESIAN_POINT('Ctrl Pts',(-1.51895133295017,1.,3.42884302333978));
#50147=CARTESIAN_POINT('Ctrl Pts',(-1.51893924967231,1.,3.42864616361967));
#50148=CARTESIAN_POINT('Ctrl Pts',(-1.51895082866166,1.,3.42859860294378));
#50149=CARTESIAN_POINT('',(-1.83867539237861,0.,3.77614523045147));
#50150=CARTESIAN_POINT('Ctrl Pts',(-1.88088939428811,-1.,3.24418789321065));
#50151=CARTESIAN_POINT('Ctrl Pts',(-1.88088939428811,1.,3.24418789321065));
#50152=CARTESIAN_POINT('Ctrl Pts',(-1.8809110068042,-1.,3.24410359189733));
#50153=CARTESIAN_POINT('Ctrl Pts',(-1.8809110068042,1.,3.24410359189733));
#50154=CARTESIAN_POINT('Ctrl Pts',(-1.8810220187274,-1.,3.24408699284449));
#50155=CARTESIAN_POINT('Ctrl Pts',(-1.8810220187274,1.,3.24408699284449));
#50156=CARTESIAN_POINT('Ctrl Pts',(-1.88139187908347,-1.,3.24451807186964));
#50157=CARTESIAN_POINT('Ctrl Pts',(-1.88139187908347,1.,3.24451807186964));
#50158=CARTESIAN_POINT('Ctrl Pts',(-1.88229202583187,-1.,3.24600543790876));
#50159=CARTESIAN_POINT('Ctrl Pts',(-1.88229202583187,1.,3.24600543790876));
#50160=CARTESIAN_POINT('Ctrl Pts',(-1.88407708646435,-1.,3.24935200512055));
#50161=CARTESIAN_POINT('Ctrl Pts',(-1.88407708646435,1.,3.24935200512055));
#50162=CARTESIAN_POINT('Ctrl Pts',(-1.88646802523372,-1.,3.25408686339298));
#50163=CARTESIAN_POINT('Ctrl Pts',(-1.88646802523372,1.,3.25408686339298));
#50164=CARTESIAN_POINT('Ctrl Pts',(-1.88934996203508,-1.,3.2599988519361));
#50165=CARTESIAN_POINT('Ctrl Pts',(-1.88934996203508,1.,3.2599988519361));
#50166=CARTESIAN_POINT('Ctrl Pts',(-1.89255393500769,-1.,3.2667765388833));
#50167=CARTESIAN_POINT('Ctrl Pts',(-1.89255393500769,1.,3.2667765388833));
#50168=CARTESIAN_POINT('Ctrl Pts',(-1.89589172903662,-1.,3.27407108932908));
#50169=CARTESIAN_POINT('Ctrl Pts',(-1.89589172903662,1.,3.27407108932908));
#50170=CARTESIAN_POINT('Ctrl Pts',(-1.89918429230425,-1.,3.28154737912287));
#50171=CARTESIAN_POINT('Ctrl Pts',(-1.89918429230425,1.,3.28154737912287));
#50172=CARTESIAN_POINT('Ctrl Pts',(-1.9022897124757,-1.,3.28893448600364));
#50173=CARTESIAN_POINT('Ctrl Pts',(-1.9022897124757,1.,3.28893448600364));
#50174=CARTESIAN_POINT('Ctrl Pts',(-1.9051389186417,-1.,3.29608978722258));
#50175=CARTESIAN_POINT('Ctrl Pts',(-1.9051389186417,1.,3.29608978722258));
#50176=CARTESIAN_POINT('Ctrl Pts',(-1.90773912171424,-1.,3.30300595568341));
#50177=CARTESIAN_POINT('Ctrl Pts',(-1.90773912171424,1.,3.30300595568341));
#50178=CARTESIAN_POINT('Ctrl Pts',(-1.91014297830502,-1.,3.30975721158694));
#50179=CARTESIAN_POINT('Ctrl Pts',(-1.91014297830502,1.,3.30975721158694));
#50180=CARTESIAN_POINT('Ctrl Pts',(-1.91242616234459,-1.,3.31646052426395));
#50181=CARTESIAN_POINT('Ctrl Pts',(-1.91242616234459,1.,3.31646052426395));
#50182=CARTESIAN_POINT('Ctrl Pts',(-1.91466343916612,-1.,3.32323403454507));
#50183=CARTESIAN_POINT('Ctrl Pts',(-1.91466343916612,1.,3.32323403454507));
#50184=CARTESIAN_POINT('Ctrl Pts',(-1.91690081930297,-1.,3.33014884257812));
#50185=CARTESIAN_POINT('Ctrl Pts',(-1.91690081930297,1.,3.33014884257812));
#50186=CARTESIAN_POINT('Ctrl Pts',(-1.91914609610173,-1.,3.33721230709948));
#50187=CARTESIAN_POINT('Ctrl Pts',(-1.91914609610173,1.,3.33721230709948));
#50188=CARTESIAN_POINT('Ctrl Pts',(-1.92138450828378,-1.,3.34439448941915));
#50189=CARTESIAN_POINT('Ctrl Pts',(-1.92138450828378,1.,3.34439448941915));
#50190=CARTESIAN_POINT('Ctrl Pts',(-1.92358838440518,-1.,3.35164424847206));
#50191=CARTESIAN_POINT('Ctrl Pts',(-1.92358838440518,1.,3.35164424847206));
#50192=CARTESIAN_POINT('Ctrl Pts',(-1.92572846125763,-1.,3.35890824422976));
#50193=CARTESIAN_POINT('Ctrl Pts',(-1.92572846125763,1.,3.35890824422976));
#50194=CARTESIAN_POINT('Ctrl Pts',(-1.92778626543803,-1.,3.36615168657597));
#50195=CARTESIAN_POINT('Ctrl Pts',(-1.92778626543803,1.,3.36615168657597));
#50196=CARTESIAN_POINT('Ctrl Pts',(-1.92975993109897,-1.,3.37336807068078));
#50197=CARTESIAN_POINT('Ctrl Pts',(-1.92975993109897,1.,3.37336807068078));
#50198=CARTESIAN_POINT('Ctrl Pts',(-1.93165739093292,-1.,3.38056768525577));
#50199=CARTESIAN_POINT('Ctrl Pts',(-1.93165739093292,1.,3.38056768525577));
#50200=CARTESIAN_POINT('Ctrl Pts',(-1.93349233176794,-1.,3.38777076883267));
#50201=CARTESIAN_POINT('Ctrl Pts',(-1.93349233176794,1.,3.38777076883267));
#50202=CARTESIAN_POINT('Ctrl Pts',(-1.93527929945982,-1.,3.39499923640789));
#50203=CARTESIAN_POINT('Ctrl Pts',(-1.93527929945982,1.,3.39499923640789));
#50204=CARTESIAN_POINT('Ctrl Pts',(-1.93702857723089,-1.,3.40226802104093));
#50205=CARTESIAN_POINT('Ctrl Pts',(-1.93702857723089,1.,3.40226802104093));
#50206=CARTESIAN_POINT('Ctrl Pts',(-1.93874306008132,-1.,3.40957978266622));
#50207=CARTESIAN_POINT('Ctrl Pts',(-1.93874306008132,1.,3.40957978266622));
#50208=CARTESIAN_POINT('Ctrl Pts',(-1.94042111965237,-1.,3.41692971994082));
#50209=CARTESIAN_POINT('Ctrl Pts',(-1.94042111965237,1.,3.41692971994082));
#50210=CARTESIAN_POINT('Ctrl Pts',(-1.94205835913692,-1.,3.42430850941497));
#50211=CARTESIAN_POINT('Ctrl Pts',(-1.94205835913692,1.,3.42430850941497));
#50212=CARTESIAN_POINT('Ctrl Pts',(-1.94364973660285,-1.,3.43170586602436));
#50213=CARTESIAN_POINT('Ctrl Pts',(-1.94364973660285,1.,3.43170586602436));
#50214=CARTESIAN_POINT('Ctrl Pts',(-1.94519168842883,-1.,3.43911410197693));
#50215=CARTESIAN_POINT('Ctrl Pts',(-1.94519168842883,1.,3.43911410197693));
#50216=CARTESIAN_POINT('Ctrl Pts',(-1.94668377715332,-1.,3.44653088665685));
#50217=CARTESIAN_POINT('Ctrl Pts',(-1.94668377715332,1.,3.44653088665685));
#50218=CARTESIAN_POINT('Ctrl Pts',(-1.94812754766524,-1.,3.45395731584051));
#50219=CARTESIAN_POINT('Ctrl Pts',(-1.94812754766524,1.,3.45395731584051));
#50220=CARTESIAN_POINT('Ctrl Pts',(-1.94952575850196,-1.,3.46139661060959));
#50221=CARTESIAN_POINT('Ctrl Pts',(-1.94952575850196,1.,3.46139661060959));
#50222=CARTESIAN_POINT('Ctrl Pts',(-1.95088147859876,-1.,3.4688525897419));
#50223=CARTESIAN_POINT('Ctrl Pts',(-1.95088147859876,1.,3.4688525897419));
#50224=CARTESIAN_POINT('Ctrl Pts',(-1.95219722189878,-1.,3.47632820495926));
#50225=CARTESIAN_POINT('Ctrl Pts',(-1.95219722189878,1.,3.47632820495926));
#50226=CARTESIAN_POINT('Ctrl Pts',(-1.95347412486316,-1.,3.48382414832648));
#50227=CARTESIAN_POINT('Ctrl Pts',(-1.95347412486316,1.,3.48382414832648));
#50228=CARTESIAN_POINT('Ctrl Pts',(-1.95471236969653,-1.,3.49133956289154));
#50229=CARTESIAN_POINT('Ctrl Pts',(-1.95471236969653,1.,3.49133956289154));
#50230=CARTESIAN_POINT('Ctrl Pts',(-1.9559115382367,-1.,3.49887263575602));
#50231=CARTESIAN_POINT('Ctrl Pts',(-1.9559115382367,1.,3.49887263575602));
#50232=CARTESIAN_POINT('Ctrl Pts',(-1.95707099606514,-1.,3.50642124159913));
#50233=CARTESIAN_POINT('Ctrl Pts',(-1.95707099606514,1.,3.50642124159913));
#50234=CARTESIAN_POINT('Ctrl Pts',(-1.95819025316768,-1.,3.51398354617772));
#50235=CARTESIAN_POINT('Ctrl Pts',(-1.95819025316768,1.,3.51398354617772));
#50236=CARTESIAN_POINT('Ctrl Pts',(-1.95926936324436,-1.,3.52155867431438));
#50237=CARTESIAN_POINT('Ctrl Pts',(-1.95926936324436,1.,3.52155867431438));
#50238=CARTESIAN_POINT('Ctrl Pts',(-1.96030879411534,-1.,3.52914648844289));
#50239=CARTESIAN_POINT('Ctrl Pts',(-1.96030879411534,1.,3.52914648844289));
#50240=CARTESIAN_POINT('Ctrl Pts',(-1.96130926212661,-1.,3.53674730625759));
#50241=CARTESIAN_POINT('Ctrl Pts',(-1.96130926212661,1.,3.53674730625759));
#50242=CARTESIAN_POINT('Ctrl Pts',(-1.96227157573058,-1.,3.54436163300425));
#50243=CARTESIAN_POINT('Ctrl Pts',(-1.96227157573058,1.,3.54436163300425));
#50244=CARTESIAN_POINT('Ctrl Pts',(-1.96319648628667,-1.,3.55198990600929));
#50245=CARTESIAN_POINT('Ctrl Pts',(-1.96319648628667,1.,3.55198990600929));
#50246=CARTESIAN_POINT('Ctrl Pts',(-1.96408450906868,-1.,3.55963218706201));
#50247=CARTESIAN_POINT('Ctrl Pts',(-1.96408450906868,1.,3.55963218706201));
#50248=CARTESIAN_POINT('Ctrl Pts',(-1.96493594634643,-1.,3.56728820357933));
#50249=CARTESIAN_POINT('Ctrl Pts',(-1.96493594634643,1.,3.56728820357933));
#50250=CARTESIAN_POINT('Ctrl Pts',(-1.96575096652857,-1.,3.57495748601088));
#50251=CARTESIAN_POINT('Ctrl Pts',(-1.96575096652857,1.,3.57495748601088));
#50252=CARTESIAN_POINT('Ctrl Pts',(-1.9665296668894,-1.,3.58263947663884));
#50253=CARTESIAN_POINT('Ctrl Pts',(-1.9665296668894,1.,3.58263947663884));
#50254=CARTESIAN_POINT('Ctrl Pts',(-1.96727213799507,-1.,3.5903336402273));
#50255=CARTESIAN_POINT('Ctrl Pts',(-1.96727213799507,1.,3.5903336402273));
#50256=CARTESIAN_POINT('Ctrl Pts',(-1.96797854118257,-1.,3.59803959819725));
#50257=CARTESIAN_POINT('Ctrl Pts',(-1.96797854118257,1.,3.59803959819725));
#50258=CARTESIAN_POINT('Ctrl Pts',(-1.96864911885775,-1.,3.60575714017676));
#50259=CARTESIAN_POINT('Ctrl Pts',(-1.96864911885775,1.,3.60575714017676));
#50260=CARTESIAN_POINT('Ctrl Pts',(-1.96928416040712,-1.,3.61348615496393));
#50261=CARTESIAN_POINT('Ctrl Pts',(-1.96928416040712,1.,3.61348615496393));
#50262=CARTESIAN_POINT('Ctrl Pts',(-1.96988398129888,-1.,3.62122658401722));
#50263=CARTESIAN_POINT('Ctrl Pts',(-1.96988398129888,1.,3.62122658401722));
#50264=CARTESIAN_POINT('Ctrl Pts',(-1.97044889850518,-1.,3.62897836973397));
#50265=CARTESIAN_POINT('Ctrl Pts',(-1.97044889850518,1.,3.62897836973397));
#50266=CARTESIAN_POINT('Ctrl Pts',(-1.97097920454698,-1.,3.63674139590853));
#50267=CARTESIAN_POINT('Ctrl Pts',(-1.97097920454698,1.,3.63674139590853));
#50268=CARTESIAN_POINT('Ctrl Pts',(-1.97147515441539,-1.,3.64451546724221));
#50269=CARTESIAN_POINT('Ctrl Pts',(-1.97147515441539,1.,3.64451546724221));
#50270=CARTESIAN_POINT('Ctrl Pts',(-1.97193697240645,-1.,3.65230034717364));
#50271=CARTESIAN_POINT('Ctrl Pts',(-1.97193697240645,1.,3.65230034717364));
#50272=CARTESIAN_POINT('Ctrl Pts',(-1.97236485439317,-1.,3.66009578166865));
#50273=CARTESIAN_POINT('Ctrl Pts',(-1.97236485439317,1.,3.66009578166865));
#50274=CARTESIAN_POINT('Ctrl Pts',(-1.9727589719863,-1.,3.66790152751984));
#50275=CARTESIAN_POINT('Ctrl Pts',(-1.9727589719863,1.,3.66790152751984));
#50276=CARTESIAN_POINT('Ctrl Pts',(-1.97311947678035,-1.,3.67571738106175));
#50277=CARTESIAN_POINT('Ctrl Pts',(-1.97311947678035,1.,3.67571738106175));
#50278=CARTESIAN_POINT('Ctrl Pts',(-1.97344650303631,-1.,3.68354319913416));
#50279=CARTESIAN_POINT('Ctrl Pts',(-1.97344650303631,1.,3.68354319913416));
#50280=CARTESIAN_POINT('Ctrl Pts',(-1.97374016224397,-1.,3.69137888597855));
#50281=CARTESIAN_POINT('Ctrl Pts',(-1.97374016224397,1.,3.69137888597855));
#50282=CARTESIAN_POINT('Ctrl Pts',(-1.97394846382289,-1.,3.69765528558292));
#50283=CARTESIAN_POINT('Ctrl Pts',(-1.97394846382289,1.,3.69765528558292));
#50284=CARTESIAN_POINT('Ctrl Pts',(-1.97408973726149,-1.,3.70236698911837));
#50285=CARTESIAN_POINT('Ctrl Pts',(-1.97408973726149,1.,3.70236698911837));
#50286=CARTESIAN_POINT('Ctrl Pts',(-1.974177276451,-1.,3.7055100813194));
#50287=CARTESIAN_POINT('Ctrl Pts',(-1.974177276451,1.,3.7055100813194));
#50288=CARTESIAN_POINT('Ctrl Pts',(-1.97421938526992,-1.,3.70708211654725));
#50289=CARTESIAN_POINT('Ctrl Pts',(-1.97421938526992,1.,3.70708211654725));
#50290=CARTESIAN_POINT('',(-1.88097764062542,1.,3.24413672884902));
#50291=CARTESIAN_POINT('Ctrl Pts',(-1.88097764062542,-1.,3.24413672884902));
#50292=CARTESIAN_POINT('Ctrl Pts',(-1.88097764062542,-0.666666666666667,
3.24413672884902));
#50293=CARTESIAN_POINT('Ctrl Pts',(-1.88097764062542,-0.333333333333333,
3.24413672884902));
#50294=CARTESIAN_POINT('Ctrl Pts',(-1.88097764062542,0.333333333333333,
3.24413672884902));
#50295=CARTESIAN_POINT('Ctrl Pts',(-1.88097764062542,0.666666666666667,
3.24413672884902));
#50296=CARTESIAN_POINT('Ctrl Pts',(-1.88097764062542,1.,3.24413672884902));
#50297=CARTESIAN_POINT('',(-1.97421938526992,1.,3.70708211654725));
#50298=CARTESIAN_POINT('',(-1.97421938526992,0.,3.70708211654725));
#50299=CARTESIAN_POINT('Ctrl Pts',(-1.88097764062542,1.,3.24413672884902));
#50300=CARTESIAN_POINT('Ctrl Pts',(-1.88102292397987,1.,3.24415531671311));
#50301=CARTESIAN_POINT('Ctrl Pts',(-1.88117508446657,1.,3.24428080352952));
#50302=CARTESIAN_POINT('Ctrl Pts',(-1.88156537699118,1.,3.24480754675942));
#50303=CARTESIAN_POINT('Ctrl Pts',(-1.88242596600422,1.,3.24625654410705));
#50304=CARTESIAN_POINT('Ctrl Pts',(-1.88407708646435,1.,3.24935200512055));
#50305=CARTESIAN_POINT('Ctrl Pts',(-1.88646802523372,1.,3.25408686339298));
#50306=CARTESIAN_POINT('Ctrl Pts',(-1.88934996203508,1.,3.2599988519361));
#50307=CARTESIAN_POINT('Ctrl Pts',(-1.89255393500769,1.,3.2667765388833));
#50308=CARTESIAN_POINT('Ctrl Pts',(-1.89589172903662,1.,3.27407108932908));
#50309=CARTESIAN_POINT('Ctrl Pts',(-1.89918429230425,1.,3.28154737912287));
#50310=CARTESIAN_POINT('Ctrl Pts',(-1.9022897124757,1.,3.28893448600364));
#50311=CARTESIAN_POINT('Ctrl Pts',(-1.9051389186417,1.,3.29608978722258));
#50312=CARTESIAN_POINT('Ctrl Pts',(-1.90773912171424,1.,3.30300595568341));
#50313=CARTESIAN_POINT('Ctrl Pts',(-1.91014297830502,1.,3.30975721158694));
#50314=CARTESIAN_POINT('Ctrl Pts',(-1.91242616234459,1.,3.31646052426395));
#50315=CARTESIAN_POINT('Ctrl Pts',(-1.91466343916612,1.,3.32323403454507));
#50316=CARTESIAN_POINT('Ctrl Pts',(-1.91690081930297,1.,3.33014884257812));
#50317=CARTESIAN_POINT('Ctrl Pts',(-1.91914609610173,1.,3.33721230709948));
#50318=CARTESIAN_POINT('Ctrl Pts',(-1.92138450828378,1.,3.34439448941915));
#50319=CARTESIAN_POINT('Ctrl Pts',(-1.92358838440518,1.,3.35164424847206));
#50320=CARTESIAN_POINT('Ctrl Pts',(-1.92572846125763,1.,3.35890824422976));
#50321=CARTESIAN_POINT('Ctrl Pts',(-1.92778626543803,1.,3.36615168657597));
#50322=CARTESIAN_POINT('Ctrl Pts',(-1.92975993109897,1.,3.37336807068078));
#50323=CARTESIAN_POINT('Ctrl Pts',(-1.93165739093292,1.,3.38056768525577));
#50324=CARTESIAN_POINT('Ctrl Pts',(-1.93349233176794,1.,3.38777076883267));
#50325=CARTESIAN_POINT('Ctrl Pts',(-1.93527929945982,1.,3.39499923640789));
#50326=CARTESIAN_POINT('Ctrl Pts',(-1.93702857723089,1.,3.40226802104093));
#50327=CARTESIAN_POINT('Ctrl Pts',(-1.93874306008132,1.,3.40957978266622));
#50328=CARTESIAN_POINT('Ctrl Pts',(-1.94042111965237,1.,3.41692971994082));
#50329=CARTESIAN_POINT('Ctrl Pts',(-1.94205835913692,1.,3.42430850941497));
#50330=CARTESIAN_POINT('Ctrl Pts',(-1.94364973660285,1.,3.43170586602436));
#50331=CARTESIAN_POINT('Ctrl Pts',(-1.94519168842883,1.,3.43911410197693));
#50332=CARTESIAN_POINT('Ctrl Pts',(-1.94668377715332,1.,3.44653088665685));
#50333=CARTESIAN_POINT('Ctrl Pts',(-1.94812754766524,1.,3.45395731584051));
#50334=CARTESIAN_POINT('Ctrl Pts',(-1.94952575850196,1.,3.46139661060959));
#50335=CARTESIAN_POINT('Ctrl Pts',(-1.95088147859876,1.,3.4688525897419));
#50336=CARTESIAN_POINT('Ctrl Pts',(-1.95219722189878,1.,3.47632820495926));
#50337=CARTESIAN_POINT('Ctrl Pts',(-1.95347412486316,1.,3.48382414832648));
#50338=CARTESIAN_POINT('Ctrl Pts',(-1.95471236969653,1.,3.49133956289154));
#50339=CARTESIAN_POINT('Ctrl Pts',(-1.9559115382367,1.,3.49887263575602));
#50340=CARTESIAN_POINT('Ctrl Pts',(-1.95707099606514,1.,3.50642124159913));
#50341=CARTESIAN_POINT('Ctrl Pts',(-1.95819025316768,1.,3.51398354617772));
#50342=CARTESIAN_POINT('Ctrl Pts',(-1.95926936324436,1.,3.52155867431438));
#50343=CARTESIAN_POINT('Ctrl Pts',(-1.96030879411534,1.,3.52914648844289));
#50344=CARTESIAN_POINT('Ctrl Pts',(-1.96130926212661,1.,3.53674730625759));
#50345=CARTESIAN_POINT('Ctrl Pts',(-1.96227157573058,1.,3.54436163300425));
#50346=CARTESIAN_POINT('Ctrl Pts',(-1.96319648628667,1.,3.55198990600929));
#50347=CARTESIAN_POINT('Ctrl Pts',(-1.96408450906868,1.,3.55963218706201));
#50348=CARTESIAN_POINT('Ctrl Pts',(-1.96493594634643,1.,3.56728820357933));
#50349=CARTESIAN_POINT('Ctrl Pts',(-1.96575096652857,1.,3.57495748601088));
#50350=CARTESIAN_POINT('Ctrl Pts',(-1.9665296668894,1.,3.58263947663884));
#50351=CARTESIAN_POINT('Ctrl Pts',(-1.96727213799507,1.,3.5903336402273));
#50352=CARTESIAN_POINT('Ctrl Pts',(-1.96797854118257,1.,3.59803959819725));
#50353=CARTESIAN_POINT('Ctrl Pts',(-1.96864911885775,1.,3.60575714017676));
#50354=CARTESIAN_POINT('Ctrl Pts',(-1.96928416040712,1.,3.61348615496393));
#50355=CARTESIAN_POINT('Ctrl Pts',(-1.96988398129888,1.,3.62122658401722));
#50356=CARTESIAN_POINT('Ctrl Pts',(-1.97044889850518,1.,3.62897836973397));
#50357=CARTESIAN_POINT('Ctrl Pts',(-1.97097920454698,1.,3.63674139590853));
#50358=CARTESIAN_POINT('Ctrl Pts',(-1.97147515441539,1.,3.64451546724221));
#50359=CARTESIAN_POINT('Ctrl Pts',(-1.97193697240645,1.,3.65230034717364));
#50360=CARTESIAN_POINT('Ctrl Pts',(-1.97236485439317,1.,3.66009578166865));
#50361=CARTESIAN_POINT('Ctrl Pts',(-1.9727589719863,1.,3.66790152751984));
#50362=CARTESIAN_POINT('Ctrl Pts',(-1.97311947678035,1.,3.67571738106175));
#50363=CARTESIAN_POINT('Ctrl Pts',(-1.97344650303631,1.,3.68354319913416));
#50364=CARTESIAN_POINT('Ctrl Pts',(-1.97374016224397,1.,3.69137888597855));
#50365=CARTESIAN_POINT('Ctrl Pts',(-1.97394846382289,1.,3.69765528558292));
#50366=CARTESIAN_POINT('Ctrl Pts',(-1.97408973726149,1.,3.70236698911837));
#50367=CARTESIAN_POINT('Ctrl Pts',(-1.974177276451,1.,3.7055100813194));
#50368=CARTESIAN_POINT('Ctrl Pts',(-1.97421938526992,1.,3.70708211654725));
#50369=CARTESIAN_POINT('Origin',(-1.97421938526992,0.,3.70708211654725));
#50370=CARTESIAN_POINT('',(-1.83867539237861,1.,3.77614523045147));
#50371=CARTESIAN_POINT('Origin',(0.,0.,0.));
#50372=CARTESIAN_POINT('',(-2.03660101169564,1.,3.14877060440425));
#50373=CARTESIAN_POINT('Origin',(0.,1.,0.));
#50374=CARTESIAN_POINT('Ctrl Pts',(-2.03660101169564,1.,3.14877060440425));
#50375=CARTESIAN_POINT('Ctrl Pts',(-2.03660101169564,0.666666666666667,
3.14877060440425));
#50376=CARTESIAN_POINT('Ctrl Pts',(-2.03660101169564,0.333333333333333,
3.14877060440425));
#50377=CARTESIAN_POINT('Ctrl Pts',(-2.03660101169564,-0.333333333333333,
3.14877060440425));
#50378=CARTESIAN_POINT('Ctrl Pts',(-2.03660101169564,-0.666666666666667,
3.14877060440425));
#50379=CARTESIAN_POINT('Ctrl Pts',(-2.03660101169564,-1.,3.14877060440425));
#50380=CARTESIAN_POINT('Ctrl Pts',(-2.40675750623143,-1.,3.44202241512147));
#50381=CARTESIAN_POINT('Ctrl Pts',(-2.40675750623143,1.,3.44202241512147));
#50382=CARTESIAN_POINT('Ctrl Pts',(-2.40537592959345,-1.,3.44127120683402));
#50383=CARTESIAN_POINT('Ctrl Pts',(-2.40537592959345,1.,3.44127120683402));
#50384=CARTESIAN_POINT('Ctrl Pts',(-2.40261515590099,-1.,3.43976627485223));
#50385=CARTESIAN_POINT('Ctrl Pts',(-2.40261515590099,1.,3.43976627485223));
#50386=CARTESIAN_POINT('Ctrl Pts',(-2.39848113411429,-1.,3.43750133066036));
#50387=CARTESIAN_POINT('Ctrl Pts',(-2.39848113411429,1.,3.43750133066036));
#50388=CARTESIAN_POINT('Ctrl Pts',(-2.39298338805823,-1.,3.43446630680436));
#50389=CARTESIAN_POINT('Ctrl Pts',(-2.39298338805823,1.,3.43446630680436));
#50390=CARTESIAN_POINT('Ctrl Pts',(-2.38613505844641,-1.,3.43064732714472));
#50391=CARTESIAN_POINT('Ctrl Pts',(-2.38613505844641,1.,3.43064732714472));
#50392=CARTESIAN_POINT('Ctrl Pts',(-2.37931067029517,-1.,3.42680309755241));
#50393=CARTESIAN_POINT('Ctrl Pts',(-2.37931067029517,1.,3.42680309755241));
#50394=CARTESIAN_POINT('Ctrl Pts',(-2.37251035954351,-1.,3.42293356216595));
#50395=CARTESIAN_POINT('Ctrl Pts',(-2.37251035954351,1.,3.42293356216595));
#50396=CARTESIAN_POINT('Ctrl Pts',(-2.36573431470314,-1.,3.41903866635384));
#50397=CARTESIAN_POINT('Ctrl Pts',(-2.36573431470314,1.,3.41903866635384));
#50398=CARTESIAN_POINT('Ctrl Pts',(-2.35898278606449,-1.,3.4151183675076));
#50399=CARTESIAN_POINT('Ctrl Pts',(-2.35898278606449,1.,3.4151183675076));
#50400=CARTESIAN_POINT('Ctrl Pts',(-2.35225606823649,-1.,3.41117262313464));
#50401=CARTESIAN_POINT('Ctrl Pts',(-2.35225606823649,1.,3.41117262313464));
#50402=CARTESIAN_POINT('Ctrl Pts',(-2.34555447648901,-1.,3.40720137403888));
#50403=CARTESIAN_POINT('Ctrl Pts',(-2.34555447648901,1.,3.40720137403888));
#50404=CARTESIAN_POINT('Ctrl Pts',(-2.33887832342715,-1.,3.40320452776646));
#50405=CARTESIAN_POINT('Ctrl Pts',(-2.33887832342715,1.,3.40320452776646));
#50406=CARTESIAN_POINT('Ctrl Pts',(-2.33222789882601,-1.,3.39918194578115));
#50407=CARTESIAN_POINT('Ctrl Pts',(-2.33222789882601,1.,3.39918194578115));
#50408=CARTESIAN_POINT('Ctrl Pts',(-2.32560343902683,-1.,3.39513342020045));
#50409=CARTESIAN_POINT('Ctrl Pts',(-2.32560343902683,1.,3.39513342020045));
#50410=CARTESIAN_POINT('Ctrl Pts',(-2.31900513925627,-1.,3.39105869475112));
#50411=CARTESIAN_POINT('Ctrl Pts',(-2.31900513925627,1.,3.39105869475112));
#50412=CARTESIAN_POINT('Ctrl Pts',(-2.31243319489505,-1.,3.38695751492659));
#50413=CARTESIAN_POINT('Ctrl Pts',(-2.31243319489505,1.,3.38695751492659));
#50414=CARTESIAN_POINT('Ctrl Pts',(-2.30588783640389,-1.,3.38282967336676));
#50415=CARTESIAN_POINT('Ctrl Pts',(-2.30588783640389,1.,3.38282967336676));
#50416=CARTESIAN_POINT('Ctrl Pts',(-2.29936936127588,-1.,3.37867504959382));
#50417=CARTESIAN_POINT('Ctrl Pts',(-2.29936936127588,1.,3.37867504959382));
#50418=CARTESIAN_POINT('Ctrl Pts',(-2.2928781800731,-1.,3.37449367172707));
#50419=CARTESIAN_POINT('Ctrl Pts',(-2.2928781800731,1.,3.37449367172707));
#50420=CARTESIAN_POINT('Ctrl Pts',(-2.28641481081045,-1.,3.37028570206357));
#50421=CARTESIAN_POINT('Ctrl Pts',(-2.28641481081045,1.,3.37028570206357));
#50422=CARTESIAN_POINT('Ctrl Pts',(-2.27997979457968,-1.,3.36605130712978));
#50423=CARTESIAN_POINT('Ctrl Pts',(-2.27997979457968,1.,3.36605130712978));
#50424=CARTESIAN_POINT('Ctrl Pts',(-2.27357362620902,-1.,3.36179055004369));
#50425=CARTESIAN_POINT('Ctrl Pts',(-2.27357362620902,1.,3.36179055004369));
#50426=CARTESIAN_POINT('Ctrl Pts',(-2.26719668579921,-1.,3.35750328523077));
#50427=CARTESIAN_POINT('Ctrl Pts',(-2.26719668579921,1.,3.35750328523077));
#50428=CARTESIAN_POINT('Ctrl Pts',(-2.26084915222484,-1.,3.35318902552676));
#50429=CARTESIAN_POINT('Ctrl Pts',(-2.26084915222484,1.,3.35318902552676));
#50430=CARTESIAN_POINT('Ctrl Pts',(-2.25453097693524,-1.,3.34884690292342));
#50431=CARTESIAN_POINT('Ctrl Pts',(-2.25453097693524,1.,3.34884690292342));
#50432=CARTESIAN_POINT('Ctrl Pts',(-2.24824207678288,-1.,3.34447596770768));
#50433=CARTESIAN_POINT('Ctrl Pts',(-2.24824207678288,1.,3.34447596770768));
#50434=CARTESIAN_POINT('Ctrl Pts',(-2.24198249391437,-1.,3.34007543738044));
#50435=CARTESIAN_POINT('Ctrl Pts',(-2.24198249391437,1.,3.34007543738044));
#50436=CARTESIAN_POINT('Ctrl Pts',(-2.2357525632881,-1.,3.33564495756478));
#50437=CARTESIAN_POINT('Ctrl Pts',(-2.2357525632881,1.,3.33564495756478));
#50438=CARTESIAN_POINT('Ctrl Pts',(-2.22955308907221,-1.,3.33118487773593));
#50439=CARTESIAN_POINT('Ctrl Pts',(-2.22955308907221,1.,3.33118487773593));
#50440=CARTESIAN_POINT('Ctrl Pts',(-2.22338548312758,-1.,3.32669646722871));
#50441=CARTESIAN_POINT('Ctrl Pts',(-2.22338548312758,1.,3.32669646722871));
#50442=CARTESIAN_POINT('Ctrl Pts',(-2.21725135110889,-1.,3.32218125618955));
#50443=CARTESIAN_POINT('Ctrl Pts',(-2.21725135110889,1.,3.32218125618955));
#50444=CARTESIAN_POINT('Ctrl Pts',(-2.21115211847872,-1.,3.31764044024231));
#50445=CARTESIAN_POINT('Ctrl Pts',(-2.21115211847872,1.,3.31764044024231));
#50446=CARTESIAN_POINT('Ctrl Pts',(-2.20508863150608,-1.,3.3130742460895));
#50447=CARTESIAN_POINT('Ctrl Pts',(-2.20508863150608,1.,3.3130742460895));
#50448=CARTESIAN_POINT('Ctrl Pts',(-2.19906078949924,-1.,3.30848134694596));
#50449=CARTESIAN_POINT('Ctrl Pts',(-2.19906078949924,1.,3.30848134694596));
#50450=CARTESIAN_POINT('Ctrl Pts',(-2.19306710376112,-1.,3.30385816281831));
#50451=CARTESIAN_POINT('Ctrl Pts',(-2.19306710376112,1.,3.30385816281831));
#50452=CARTESIAN_POINT('Ctrl Pts',(-2.18710556500325,-1.,3.29920022557635));
#50453=CARTESIAN_POINT('Ctrl Pts',(-2.18710556500325,1.,3.29920022557635));
#50454=CARTESIAN_POINT('Ctrl Pts',(-2.18117455557062,-1.,3.29450361500484));
#50455=CARTESIAN_POINT('Ctrl Pts',(-2.18117455557062,1.,3.29450361500484));
#50456=CARTESIAN_POINT('Ctrl Pts',(-2.17527380048422,-1.,3.28976645712566));
#50457=CARTESIAN_POINT('Ctrl Pts',(-2.17527380048422,1.,3.28976645712566));
#50458=CARTESIAN_POINT('Ctrl Pts',(-2.16940517773459,-1.,3.2849901997973));
#50459=CARTESIAN_POINT('Ctrl Pts',(-2.16940517773459,1.,3.2849901997973));
#50460=CARTESIAN_POINT('Ctrl Pts',(-2.16357391934434,-1.,3.28018150841414));
#50461=CARTESIAN_POINT('Ctrl Pts',(-2.16357391934434,1.,3.28018150841414));
#50462=CARTESIAN_POINT('Ctrl Pts',(-2.15778690038359,-1.,3.27534954469206));
#50463=CARTESIAN_POINT('Ctrl Pts',(-2.15778690038359,1.,3.27534954469206));
#50464=CARTESIAN_POINT('Ctrl Pts',(-2.15205043199818,-1.,3.27050245897244));
#50465=CARTESIAN_POINT('Ctrl Pts',(-2.15205043199818,1.,3.27050245897244));
#50466=CARTESIAN_POINT('Ctrl Pts',(-2.14636805295663,-1.,3.26564388189764));
#50467=CARTESIAN_POINT('Ctrl Pts',(-2.14636805295663,1.,3.26564388189764));
#50468=CARTESIAN_POINT('Ctrl Pts',(-2.14073870754257,-1.,3.26077002641868));
#50469=CARTESIAN_POINT('Ctrl Pts',(-2.14073870754257,1.,3.26077002641868));
#50470=CARTESIAN_POINT('Ctrl Pts',(-2.13515375878786,-1.,3.25586495065027));
#50471=CARTESIAN_POINT('Ctrl Pts',(-2.13515375878786,1.,3.25586495065027));
#50472=CARTESIAN_POINT('Ctrl Pts',(-2.1296002839681,-1.,3.25090574493994));
#50473=CARTESIAN_POINT('Ctrl Pts',(-2.1296002839681,1.,3.25090574493994));
#50474=CARTESIAN_POINT('Ctrl Pts',(-2.12406646410943,-1.,3.24587102613347));
#50475=CARTESIAN_POINT('Ctrl Pts',(-2.12406646410943,1.,3.24587102613347));
#50476=CARTESIAN_POINT('Ctrl Pts',(-2.11854673326972,-1.,3.24074905517282));
#50477=CARTESIAN_POINT('Ctrl Pts',(-2.11854673326972,1.,3.24074905517282));
#50478=CARTESIAN_POINT('Ctrl Pts',(-2.11304604021784,-1.,3.23554444767115));
#50479=CARTESIAN_POINT('Ctrl Pts',(-2.11304604021784,1.,3.23554444767115));
#50480=CARTESIAN_POINT('Ctrl Pts',(-2.1075869964248,-1.,3.23028945793334));
#50481=CARTESIAN_POINT('Ctrl Pts',(-2.1075869964248,1.,3.23028945793334));
#50482=CARTESIAN_POINT('Ctrl Pts',(-2.10220384298533,-1.,3.22503437553496));
#50483=CARTESIAN_POINT('Ctrl Pts',(-2.10220384298533,1.,3.22503437553496));
#50484=CARTESIAN_POINT('Ctrl Pts',(-2.09692958434933,-1.,3.21982707347067));
#50485=CARTESIAN_POINT('Ctrl Pts',(-2.09692958434933,1.,3.21982707347067));
#50486=CARTESIAN_POINT('Ctrl Pts',(-2.0917841946046,-1.,3.2146942960168));
#50487=CARTESIAN_POINT('Ctrl Pts',(-2.0917841946046,1.,3.2146942960168));
#50488=CARTESIAN_POINT('Ctrl Pts',(-2.08676465517435,-1.,3.20962575845433));
#50489=CARTESIAN_POINT('Ctrl Pts',(-2.08676465517435,1.,3.20962575845433));
#50490=CARTESIAN_POINT('Ctrl Pts',(-2.08182850370816,-1.,3.20454818630635));
#50491=CARTESIAN_POINT('Ctrl Pts',(-2.08182850370816,1.,3.20454818630635));
#50492=CARTESIAN_POINT('Ctrl Pts',(-2.0769044187063,-1.,3.19934132835879));
#50493=CARTESIAN_POINT('Ctrl Pts',(-2.0769044187063,1.,3.19934132835879));
#50494=CARTESIAN_POINT('Ctrl Pts',(-2.07192253497765,-1.,3.19388465568113));
#50495=CARTESIAN_POINT('Ctrl Pts',(-2.07192253497765,1.,3.19388465568113));
#50496=CARTESIAN_POINT('Ctrl Pts',(-2.06684062744065,-1.,3.18809755562297));
#50497=CARTESIAN_POINT('Ctrl Pts',(-2.06684062744065,1.,3.18809755562297));
#50498=CARTESIAN_POINT('Ctrl Pts',(-2.06166849827143,-1.,3.18197692964677));
#50499=CARTESIAN_POINT('Ctrl Pts',(-2.06166849827143,1.,3.18197692964677));
#50500=CARTESIAN_POINT('Ctrl Pts',(-2.05650186773279,-1.,3.17564906975592));
#50501=CARTESIAN_POINT('Ctrl Pts',(-2.05650186773279,1.,3.17564906975592));
#50502=CARTESIAN_POINT('Ctrl Pts',(-2.05151770247452,-1.,3.16936341689859));
#50503=CARTESIAN_POINT('Ctrl Pts',(-2.05151770247452,1.,3.16936341689859));
#50504=CARTESIAN_POINT('Ctrl Pts',(-2.0469333124766,-1.,3.16343165059235));
#50505=CARTESIAN_POINT('Ctrl Pts',(-2.0469333124766,1.,3.16343165059235));
#50506=CARTESIAN_POINT('Ctrl Pts',(-2.04297406404132,-1.,3.15817983946525));
#50507=CARTESIAN_POINT('Ctrl Pts',(-2.04297406404132,1.,3.15817983946525));
#50508=CARTESIAN_POINT('Ctrl Pts',(-2.03984073791432,-1.,3.1538999167466));
#50509=CARTESIAN_POINT('Ctrl Pts',(-2.03984073791432,1.,3.1538999167466));
#50510=CARTESIAN_POINT('Ctrl Pts',(-2.03766932526171,-1.,3.15079010635326));
#50511=CARTESIAN_POINT('Ctrl Pts',(-2.03766932526171,1.,3.15079010635326));
#50512=CARTESIAN_POINT('Ctrl Pts',(-2.03675273048882,-1.,3.14931281967585));
#50513=CARTESIAN_POINT('Ctrl Pts',(-2.03675273048882,1.,3.14931281967585));
#50514=CARTESIAN_POINT('Ctrl Pts',(-2.03653654935384,-1.,3.14878756590499));
#50515=CARTESIAN_POINT('Ctrl Pts',(-2.03653654935384,1.,3.14878756590499));
#50516=CARTESIAN_POINT('Ctrl Pts',(-2.036601737578,-1.,3.14869618937138));
#50517=CARTESIAN_POINT('Ctrl Pts',(-2.036601737578,1.,3.14869618937138));
#50518=CARTESIAN_POINT('Ctrl Pts',(-2.03668666247593,-1.,3.1487152044751));
#50519=CARTESIAN_POINT('Ctrl Pts',(-2.03668666247593,1.,3.1487152044751));
#50520=CARTESIAN_POINT('',(-2.40675750623143,1.,3.44202241512147));
#50521=CARTESIAN_POINT('Ctrl Pts',(-2.40675750623143,1.,3.44202241512147));
#50522=CARTESIAN_POINT('Ctrl Pts',(-2.40537592959345,1.,3.44127120683402));
#50523=CARTESIAN_POINT('Ctrl Pts',(-2.40261515590099,1.,3.43976627485223));
#50524=CARTESIAN_POINT('Ctrl Pts',(-2.39848113411429,1.,3.43750133066036));
#50525=CARTESIAN_POINT('Ctrl Pts',(-2.39298338805823,1.,3.43446630680436));
#50526=CARTESIAN_POINT('Ctrl Pts',(-2.38613505844641,1.,3.43064732714472));
#50527=CARTESIAN_POINT('Ctrl Pts',(-2.37931067029517,1.,3.42680309755241));
#50528=CARTESIAN_POINT('Ctrl Pts',(-2.37251035954351,1.,3.42293356216595));
#50529=CARTESIAN_POINT('Ctrl Pts',(-2.36573431470314,1.,3.41903866635384));
#50530=CARTESIAN_POINT('Ctrl Pts',(-2.35898278606449,1.,3.4151183675076));
#50531=CARTESIAN_POINT('Ctrl Pts',(-2.35225606823649,1.,3.41117262313464));
#50532=CARTESIAN_POINT('Ctrl Pts',(-2.34555447648901,1.,3.40720137403888));
#50533=CARTESIAN_POINT('Ctrl Pts',(-2.33887832342715,1.,3.40320452776646));
#50534=CARTESIAN_POINT('Ctrl Pts',(-2.33222789882601,1.,3.39918194578115));
#50535=CARTESIAN_POINT('Ctrl Pts',(-2.32560343902683,1.,3.39513342020045));
#50536=CARTESIAN_POINT('Ctrl Pts',(-2.31900513925627,1.,3.39105869475112));
#50537=CARTESIAN_POINT('Ctrl Pts',(-2.31243319489505,1.,3.38695751492659));
#50538=CARTESIAN_POINT('Ctrl Pts',(-2.30588783640389,1.,3.38282967336676));
#50539=CARTESIAN_POINT('Ctrl Pts',(-2.29936936127588,1.,3.37867504959382));
#50540=CARTESIAN_POINT('Ctrl Pts',(-2.2928781800731,1.,3.37449367172707));
#50541=CARTESIAN_POINT('Ctrl Pts',(-2.28641481081045,1.,3.37028570206357));
#50542=CARTESIAN_POINT('Ctrl Pts',(-2.27997979457968,1.,3.36605130712978));
#50543=CARTESIAN_POINT('Ctrl Pts',(-2.27357362620902,1.,3.36179055004369));
#50544=CARTESIAN_POINT('Ctrl Pts',(-2.26719668579921,1.,3.35750328523077));
#50545=CARTESIAN_POINT('Ctrl Pts',(-2.26084915222484,1.,3.35318902552676));
#50546=CARTESIAN_POINT('Ctrl Pts',(-2.25453097693524,1.,3.34884690292342));
#50547=CARTESIAN_POINT('Ctrl Pts',(-2.24824207678288,1.,3.34447596770768));
#50548=CARTESIAN_POINT('Ctrl Pts',(-2.24198249391437,1.,3.34007543738044));
#50549=CARTESIAN_POINT('Ctrl Pts',(-2.2357525632881,1.,3.33564495756478));
#50550=CARTESIAN_POINT('Ctrl Pts',(-2.22955308907221,1.,3.33118487773593));
#50551=CARTESIAN_POINT('Ctrl Pts',(-2.22338548312758,1.,3.32669646722871));
#50552=CARTESIAN_POINT('Ctrl Pts',(-2.21725135110889,1.,3.32218125618955));
#50553=CARTESIAN_POINT('Ctrl Pts',(-2.21115211847872,1.,3.31764044024231));
#50554=CARTESIAN_POINT('Ctrl Pts',(-2.20508863150608,1.,3.3130742460895));
#50555=CARTESIAN_POINT('Ctrl Pts',(-2.19906078949924,1.,3.30848134694596));
#50556=CARTESIAN_POINT('Ctrl Pts',(-2.19306710376112,1.,3.30385816281831));
#50557=CARTESIAN_POINT('Ctrl Pts',(-2.18710556500325,1.,3.29920022557635));
#50558=CARTESIAN_POINT('Ctrl Pts',(-2.18117455557062,1.,3.29450361500484));
#50559=CARTESIAN_POINT('Ctrl Pts',(-2.17527380048422,1.,3.28976645712566));
#50560=CARTESIAN_POINT('Ctrl Pts',(-2.16940517773459,1.,3.2849901997973));
#50561=CARTESIAN_POINT('Ctrl Pts',(-2.16357391934434,1.,3.28018150841414));
#50562=CARTESIAN_POINT('Ctrl Pts',(-2.15778690038359,1.,3.27534954469206));
#50563=CARTESIAN_POINT('Ctrl Pts',(-2.15205043199818,1.,3.27050245897244));
#50564=CARTESIAN_POINT('Ctrl Pts',(-2.14636805295663,1.,3.26564388189764));
#50565=CARTESIAN_POINT('Ctrl Pts',(-2.14073870754257,1.,3.26077002641868));
#50566=CARTESIAN_POINT('Ctrl Pts',(-2.13515375878786,1.,3.25586495065027));
#50567=CARTESIAN_POINT('Ctrl Pts',(-2.1296002839681,1.,3.25090574493994));
#50568=CARTESIAN_POINT('Ctrl Pts',(-2.12406646410943,1.,3.24587102613347));
#50569=CARTESIAN_POINT('Ctrl Pts',(-2.11854673326972,1.,3.24074905517282));
#50570=CARTESIAN_POINT('Ctrl Pts',(-2.11304604021784,1.,3.23554444767115));
#50571=CARTESIAN_POINT('Ctrl Pts',(-2.1075869964248,1.,3.23028945793334));
#50572=CARTESIAN_POINT('Ctrl Pts',(-2.10220384298533,1.,3.22503437553496));
#50573=CARTESIAN_POINT('Ctrl Pts',(-2.09692958434933,1.,3.21982707347067));
#50574=CARTESIAN_POINT('Ctrl Pts',(-2.0917841946046,1.,3.2146942960168));
#50575=CARTESIAN_POINT('Ctrl Pts',(-2.08676465517435,1.,3.20962575845433));
#50576=CARTESIAN_POINT('Ctrl Pts',(-2.08182850370816,1.,3.20454818630635));
#50577=CARTESIAN_POINT('Ctrl Pts',(-2.0769044187063,1.,3.19934132835879));
#50578=CARTESIAN_POINT('Ctrl Pts',(-2.07192253497765,1.,3.19388465568113));
#50579=CARTESIAN_POINT('Ctrl Pts',(-2.06684062744065,1.,3.18809755562297));
#50580=CARTESIAN_POINT('Ctrl Pts',(-2.06166849827143,1.,3.18197692964677));
#50581=CARTESIAN_POINT('Ctrl Pts',(-2.05650186773279,1.,3.17564906975592));
#50582=CARTESIAN_POINT('Ctrl Pts',(-2.05151770247452,1.,3.16936341689859));
#50583=CARTESIAN_POINT('Ctrl Pts',(-2.0469333124766,1.,3.16343165059235));
#50584=CARTESIAN_POINT('Ctrl Pts',(-2.04297406404132,1.,3.15817983946525));
#50585=CARTESIAN_POINT('Ctrl Pts',(-2.03984073791432,1.,3.1538999167466));
#50586=CARTESIAN_POINT('Ctrl Pts',(-2.03783225496023,1.,3.15102344775396));
#50587=CARTESIAN_POINT('Ctrl Pts',(-2.03693188810614,1.,3.14959882629936));
#50588=CARTESIAN_POINT('Ctrl Pts',(-2.03663974554941,1.,3.14901193669147));
#50589=CARTESIAN_POINT('Ctrl Pts',(-2.03659701539175,1.,3.1488193908823));
#50590=CARTESIAN_POINT('Ctrl Pts',(-2.03660101169564,1.,3.14877060440425));
#50591=CARTESIAN_POINT('',(-2.40675750623143,0.,3.44202241512147));
#50592=CARTESIAN_POINT('Ctrl Pts',(-2.36523532225181,-1.,2.91001063062876));
#50593=CARTESIAN_POINT('Ctrl Pts',(-2.36523532225181,1.,2.91001063062876));
#50594=CARTESIAN_POINT('Ctrl Pts',(-2.36524348105112,-1.,2.90992398626211));
#50595=CARTESIAN_POINT('Ctrl Pts',(-2.36524348105112,1.,2.90992398626211));
#50596=CARTESIAN_POINT('Ctrl Pts',(-2.36535052956938,-1.,2.90989022548032));
#50597=CARTESIAN_POINT('Ctrl Pts',(-2.36535052956938,1.,2.90989022548032));
#50598=CARTESIAN_POINT('Ctrl Pts',(-2.36578327194741,-1.,2.91025813830041));
#50599=CARTESIAN_POINT('Ctrl Pts',(-2.36578327194741,1.,2.91025813830041));
#50600=CARTESIAN_POINT('Ctrl Pts',(-2.36690501170627,-1.,2.9115863784204));
#50601=CARTESIAN_POINT('Ctrl Pts',(-2.36690501170627,1.,2.9115863784204));
#50602=CARTESIAN_POINT('Ctrl Pts',(-2.36919161373173,-1.,2.9146124988314));
#50603=CARTESIAN_POINT('Ctrl Pts',(-2.36919161373173,1.,2.9146124988314));
#50604=CARTESIAN_POINT('Ctrl Pts',(-2.37229381109821,-1.,2.91891503791411));
#50605=CARTESIAN_POINT('Ctrl Pts',(-2.37229381109821,1.,2.91891503791411));
#50606=CARTESIAN_POINT('Ctrl Pts',(-2.3760651052403,-1.,2.92430340582608));
#50607=CARTESIAN_POINT('Ctrl Pts',(-2.3760651052403,1.,2.92430340582608));
#50608=CARTESIAN_POINT('Ctrl Pts',(-2.38028989582073,-1.,2.93049643640206));
#50609=CARTESIAN_POINT('Ctrl Pts',(-2.38028989582073,1.,2.93049643640206));
#50610=CARTESIAN_POINT('Ctrl Pts',(-2.38472771516311,-1.,2.93717903280391));
#50611=CARTESIAN_POINT('Ctrl Pts',(-2.38472771516311,1.,2.93717903280391));
#50612=CARTESIAN_POINT('Ctrl Pts',(-2.38914929090759,-1.,2.94404820669076));
#50613=CARTESIAN_POINT('Ctrl Pts',(-2.38914929090759,1.,2.94404820669076));
#50614=CARTESIAN_POINT('Ctrl Pts',(-2.39337207631667,-1.,2.95085857128439));
#50615=CARTESIAN_POINT('Ctrl Pts',(-2.39337207631667,1.,2.95085857128439));
#50616=CARTESIAN_POINT('Ctrl Pts',(-2.39730553974517,-1.,2.95748006482942));
#50617=CARTESIAN_POINT('Ctrl Pts',(-2.39730553974517,1.,2.95748006482942));
#50618=CARTESIAN_POINT('Ctrl Pts',(-2.4009556571164,-1.,2.96390432240312));
#50619=CARTESIAN_POINT('Ctrl Pts',(-2.4009556571164,1.,2.96390432240312));
#50620=CARTESIAN_POINT('Ctrl Pts',(-2.40438604734919,-1.,2.9701964131236));
#50621=CARTESIAN_POINT('Ctrl Pts',(-2.40438604734919,1.,2.9701964131236));
#50622=CARTESIAN_POINT('Ctrl Pts',(-2.40768975073713,-1.,2.97646002822422));
#50623=CARTESIAN_POINT('Ctrl Pts',(-2.40768975073713,1.,2.97646002822422));
#50624=CARTESIAN_POINT('Ctrl Pts',(-2.41095909342571,-1.,2.98280015815107));
#50625=CARTESIAN_POINT('Ctrl Pts',(-2.41095909342571,1.,2.98280015815107));
#50626=CARTESIAN_POINT('Ctrl Pts',(-2.41425064199586,-1.,2.98927983005796));
#50627=CARTESIAN_POINT('Ctrl Pts',(-2.41425064199586,1.,2.98927983005796));
#50628=CARTESIAN_POINT('Ctrl Pts',(-2.41757324500514,-1.,2.99590509293503));
#50629=CARTESIAN_POINT('Ctrl Pts',(-2.41757324500514,1.,2.99590509293503));
#50630=CARTESIAN_POINT('Ctrl Pts',(-2.42090763946779,-1.,3.00264868585996));
#50631=CARTESIAN_POINT('Ctrl Pts',(-2.42090763946779,1.,3.00264868585996));
#50632=CARTESIAN_POINT('Ctrl Pts',(-2.42421849439613,-1.,3.00946442616658));
#50633=CARTESIAN_POINT('Ctrl Pts',(-2.42421849439613,1.,3.00946442616658));
#50634=CARTESIAN_POINT('Ctrl Pts',(-2.42746856264168,-1.,3.01630420830504));
#50635=CARTESIAN_POINT('Ctrl Pts',(-2.42746856264168,1.,3.01630420830504));
#50636=CARTESIAN_POINT('Ctrl Pts',(-2.43063415586637,-1.,3.02313656036004));
#50637=CARTESIAN_POINT('Ctrl Pts',(-2.43063415586637,1.,3.02313656036004));
#50638=CARTESIAN_POINT('Ctrl Pts',(-2.43371241361488,-1.,3.02995534946978));
#50639=CARTESIAN_POINT('Ctrl Pts',(-2.43371241361488,1.,3.02995534946978));
#50640=CARTESIAN_POINT('Ctrl Pts',(-2.43671278042414,-1.,3.03676949672821));
#50641=CARTESIAN_POINT('Ctrl Pts',(-2.43671278042414,1.,3.03676949672821));
#50642=CARTESIAN_POINT('Ctrl Pts',(-2.43965194061857,-1.,3.04359685040555));
#50643=CARTESIAN_POINT('Ctrl Pts',(-2.43965194061857,1.,3.04359685040555));
#50644=CARTESIAN_POINT('Ctrl Pts',(-2.44254768923105,-1.,3.05045678021504));
#50645=CARTESIAN_POINT('Ctrl Pts',(-2.44254768923105,1.,3.05045678021504));
#50646=CARTESIAN_POINT('Ctrl Pts',(-2.44541251892556,-1.,3.05736242671506));
#50647=CARTESIAN_POINT('Ctrl Pts',(-2.44541251892556,1.,3.05736242671506));
#50648=CARTESIAN_POINT('Ctrl Pts',(-2.44824970516544,-1.,3.06431596421405));
#50649=CARTESIAN_POINT('Ctrl Pts',(-2.44824970516544,1.,3.06431596421405));
#50650=CARTESIAN_POINT('Ctrl Pts',(-2.45105688854422,-1.,3.07131290521297));
#50651=CARTESIAN_POINT('Ctrl Pts',(-2.45105688854422,1.,3.07131290521297));
#50652=CARTESIAN_POINT('Ctrl Pts',(-2.4538282678779,-1.,3.07834472886139));
#50653=CARTESIAN_POINT('Ctrl Pts',(-2.4538282678779,1.,3.07834472886139));
#50654=CARTESIAN_POINT('Ctrl Pts',(-2.45655725437039,-1.,3.08540206545315));
#50655=CARTESIAN_POINT('Ctrl Pts',(-2.45655725437039,1.,3.08540206545315));
#50656=CARTESIAN_POINT('Ctrl Pts',(-2.4592391256388,-1.,3.09247787931887));
#50657=CARTESIAN_POINT('Ctrl Pts',(-2.4592391256388,1.,3.09247787931887));
#50658=CARTESIAN_POINT('Ctrl Pts',(-2.46187308501884,-1.,3.09956993697052));
#50659=CARTESIAN_POINT('Ctrl Pts',(-2.46187308501884,1.,3.09956993697052));
#50660=CARTESIAN_POINT('Ctrl Pts',(-2.46446082979646,-1.,3.1066790790198));
#50661=CARTESIAN_POINT('Ctrl Pts',(-2.46446082979646,1.,3.1066790790198));
#50662=CARTESIAN_POINT('Ctrl Pts',(-2.46700558843506,-1.,3.11380805536122));
#50663=CARTESIAN_POINT('Ctrl Pts',(-2.46700558843506,1.,3.11380805536122));
#50664=CARTESIAN_POINT('Ctrl Pts',(-2.46951098947469,-1.,3.12096015766983));
#50665=CARTESIAN_POINT('Ctrl Pts',(-2.46951098947469,1.,3.12096015766983));
#50666=CARTESIAN_POINT('Ctrl Pts',(-2.47197997765871,-1.,3.12813790805952));
#50667=CARTESIAN_POINT('Ctrl Pts',(-2.47197997765871,1.,3.12813790805952));
#50668=CARTESIAN_POINT('Ctrl Pts',(-2.47441378371932,-1.,3.13534181229295));
#50669=CARTESIAN_POINT('Ctrl Pts',(-2.47441378371932,1.,3.13534181229295));
#50670=CARTESIAN_POINT('Ctrl Pts',(-2.47681245356109,-1.,3.1425709954655));
#50671=CARTESIAN_POINT('Ctrl Pts',(-2.47681245356109,1.,3.1425709954655));
#50672=CARTESIAN_POINT('Ctrl Pts',(-2.47917529057029,-1.,3.14982373241352));
#50673=CARTESIAN_POINT('Ctrl Pts',(-2.47917529057029,1.,3.14982373241352));
#50674=CARTESIAN_POINT('Ctrl Pts',(-2.48150133566571,-1.,3.15709802322739));
#50675=CARTESIAN_POINT('Ctrl Pts',(-2.48150133566571,1.,3.15709802322739));
#50676=CARTESIAN_POINT('Ctrl Pts',(-2.48378981792725,-1.,3.16439213290161));
#50677=CARTESIAN_POINT('Ctrl Pts',(-2.48378981792725,1.,3.16439213290161));
#50678=CARTESIAN_POINT('Ctrl Pts',(-2.48604065348587,-1.,3.17170518863313));
#50679=CARTESIAN_POINT('Ctrl Pts',(-2.48604065348587,1.,3.17170518863313));
#50680=CARTESIAN_POINT('Ctrl Pts',(-2.48825428288201,-1.,3.17903698136622));
#50681=CARTESIAN_POINT('Ctrl Pts',(-2.48825428288201,1.,3.17903698136622));
#50682=CARTESIAN_POINT('Ctrl Pts',(-2.49043146334059,-1.,3.18638771282266));
#50683=CARTESIAN_POINT('Ctrl Pts',(-2.49043146334059,1.,3.18638771282266));
#50684=CARTESIAN_POINT('Ctrl Pts',(-2.49257307239848,-1.,3.19375775555798));
#50685=CARTESIAN_POINT('Ctrl Pts',(-2.49257307239848,1.,3.19375775555798));
#50686=CARTESIAN_POINT('Ctrl Pts',(-2.49467992057755,-1.,3.20114742397588));
#50687=CARTESIAN_POINT('Ctrl Pts',(-2.49467992057755,1.,3.20114742397588));
#50688=CARTESIAN_POINT('Ctrl Pts',(-2.4967525264737,-1.,3.20855669849836));
#50689=CARTESIAN_POINT('Ctrl Pts',(-2.4967525264737,1.,3.20855669849836));
#50690=CARTESIAN_POINT('Ctrl Pts',(-2.4987911459939,-1.,3.21598526261286));
#50691=CARTESIAN_POINT('Ctrl Pts',(-2.4987911459939,1.,3.21598526261286));
#50692=CARTESIAN_POINT('Ctrl Pts',(-2.50079587201957,-1.,3.22343262620503));
#50693=CARTESIAN_POINT('Ctrl Pts',(-2.50079587201957,1.,3.22343262620503));
#50694=CARTESIAN_POINT('Ctrl Pts',(-2.50276671338111,-1.,3.23089822320646));
#50695=CARTESIAN_POINT('Ctrl Pts',(-2.50276671338111,1.,3.23089822320646));
#50696=CARTESIAN_POINT('Ctrl Pts',(-2.5047036758003,-1.,3.23838151080319));
#50697=CARTESIAN_POINT('Ctrl Pts',(-2.5047036758003,1.,3.23838151080319));
#50698=CARTESIAN_POINT('Ctrl Pts',(-2.506606859405,-1.,3.24588208983849));
#50699=CARTESIAN_POINT('Ctrl Pts',(-2.506606859405,1.,3.24588208983849));
#50700=CARTESIAN_POINT('Ctrl Pts',(-2.50847647070723,-1.,3.25339971460982));
#50701=CARTESIAN_POINT('Ctrl Pts',(-2.50847647070723,1.,3.25339971460982));
#50702=CARTESIAN_POINT('Ctrl Pts',(-2.51031277813486,-1.,3.26093423001434));
#50703=CARTESIAN_POINT('Ctrl Pts',(-2.51031277813486,1.,3.26093423001434));
#50704=CARTESIAN_POINT('Ctrl Pts',(-2.51211608411423,-1.,3.26848552888115));
#50705=CARTESIAN_POINT('Ctrl Pts',(-2.51211608411423,1.,3.26848552888115));
#50706=CARTESIAN_POINT('Ctrl Pts',(-2.513886692704,-1.,3.27605350473142));
#50707=CARTESIAN_POINT('Ctrl Pts',(-2.513886692704,1.,3.27605350473142));
#50708=CARTESIAN_POINT('Ctrl Pts',(-2.51562487464514,-1.,3.28363799702982));
#50709=CARTESIAN_POINT('Ctrl Pts',(-2.51562487464514,1.,3.28363799702982));
#50710=CARTESIAN_POINT('Ctrl Pts',(-2.51733085123797,-1.,3.2912387729927));
#50711=CARTESIAN_POINT('Ctrl Pts',(-2.51733085123797,1.,3.2912387729927));
#50712=CARTESIAN_POINT('Ctrl Pts',(-2.51900480701069,-1.,3.29885556388352));
#50713=CARTESIAN_POINT('Ctrl Pts',(-2.51900480701069,1.,3.29885556388352));
#50714=CARTESIAN_POINT('Ctrl Pts',(-2.52064689568511,-1.,3.30648808815442));
#50715=CARTESIAN_POINT('Ctrl Pts',(-2.52064689568511,1.,3.30648808815442));
#50716=CARTESIAN_POINT('Ctrl Pts',(-2.52225724871313,-1.,3.31413607874645));
#50717=CARTESIAN_POINT('Ctrl Pts',(-2.52225724871313,1.,3.31413607874645));
#50718=CARTESIAN_POINT('Ctrl Pts',(-2.5238359839626,-1.,3.32179931078699));
#50719=CARTESIAN_POINT('Ctrl Pts',(-2.5238359839626,1.,3.32179931078699));
#50720=CARTESIAN_POINT('Ctrl Pts',(-2.52538321164634,-1.,3.32947762187533));
#50721=CARTESIAN_POINT('Ctrl Pts',(-2.52538321164634,1.,3.32947762187533));
#50722=CARTESIAN_POINT('Ctrl Pts',(-2.52689902690158,-1.,3.33717089999103));
#50723=CARTESIAN_POINT('Ctrl Pts',(-2.52689902690158,1.,3.33717089999103));
#50724=CARTESIAN_POINT('Ctrl Pts',(-2.52808660915689,-1.,3.34333744115511));
#50725=CARTESIAN_POINT('Ctrl Pts',(-2.52808660915689,1.,3.34333744115511));
#50726=CARTESIAN_POINT('Ctrl Pts',(-2.52896321610703,-1.,3.34796903576663));
#50727=CARTESIAN_POINT('Ctrl Pts',(-2.52896321610703,1.,3.34796903576663));
#50728=CARTESIAN_POINT('Ctrl Pts',(-2.5295413654909,-1.,3.35105973714071));
#50729=CARTESIAN_POINT('Ctrl Pts',(-2.5295413654909,1.,3.35105973714071));
#50730=CARTESIAN_POINT('Ctrl Pts',(-2.52982887637028,-1.,3.35260583073571));
#50731=CARTESIAN_POINT('Ctrl Pts',(-2.52982887637028,1.,3.35260583073571));
#50732=CARTESIAN_POINT('',(-2.36531447826073,1.,2.90994629141676));
#50733=CARTESIAN_POINT('Ctrl Pts',(-2.36531447826073,-1.,2.90994629141676));
#50734=CARTESIAN_POINT('Ctrl Pts',(-2.36531447826073,-0.666666666666667,
2.90994629141676));
#50735=CARTESIAN_POINT('Ctrl Pts',(-2.36531447826073,-0.333333333333333,
2.90994629141676));
#50736=CARTESIAN_POINT('Ctrl Pts',(-2.36531447826073,0.333333333333333,
2.90994629141676));
#50737=CARTESIAN_POINT('Ctrl Pts',(-2.36531447826073,0.666666666666667,
2.90994629141676));
#50738=CARTESIAN_POINT('Ctrl Pts',(-2.36531447826073,1.,2.90994629141676));
#50739=CARTESIAN_POINT('',(-2.52982887637028,1.,3.35260583073571));
#50740=CARTESIAN_POINT('',(-2.52982887637028,0.,3.35260583073571));
#50741=CARTESIAN_POINT('Ctrl Pts',(-2.36531447826073,1.,2.90994629141676));
#50742=CARTESIAN_POINT('Ctrl Pts',(-2.36536211188453,1.,2.90995756655606));
#50743=CARTESIAN_POINT('Ctrl Pts',(-2.36553202948613,1.,2.91005770527719));
#50744=CARTESIAN_POINT('Ctrl Pts',(-2.36599991765749,1.,2.91051690822156));
#50745=CARTESIAN_POINT('Ctrl Pts',(-2.36707658451664,1.,2.91181344022549));
#50746=CARTESIAN_POINT('Ctrl Pts',(-2.36919161373173,1.,2.9146124988314));
#50747=CARTESIAN_POINT('Ctrl Pts',(-2.37229381109821,1.,2.91891503791411));
#50748=CARTESIAN_POINT('Ctrl Pts',(-2.3760651052403,1.,2.92430340582608));
#50749=CARTESIAN_POINT('Ctrl Pts',(-2.38028989582073,1.,2.93049643640206));
#50750=CARTESIAN_POINT('Ctrl Pts',(-2.38472771516311,1.,2.93717903280391));
#50751=CARTESIAN_POINT('Ctrl Pts',(-2.38914929090759,1.,2.94404820669076));
#50752=CARTESIAN_POINT('Ctrl Pts',(-2.39337207631667,1.,2.95085857128439));
#50753=CARTESIAN_POINT('Ctrl Pts',(-2.39730553974517,1.,2.95748006482942));
#50754=CARTESIAN_POINT('Ctrl Pts',(-2.4009556571164,1.,2.96390432240312));
#50755=CARTESIAN_POINT('Ctrl Pts',(-2.40438604734919,1.,2.9701964131236));
#50756=CARTESIAN_POINT('Ctrl Pts',(-2.40768975073713,1.,2.97646002822422));
#50757=CARTESIAN_POINT('Ctrl Pts',(-2.41095909342571,1.,2.98280015815107));
#50758=CARTESIAN_POINT('Ctrl Pts',(-2.41425064199586,1.,2.98927983005796));
#50759=CARTESIAN_POINT('Ctrl Pts',(-2.41757324500514,1.,2.99590509293503));
#50760=CARTESIAN_POINT('Ctrl Pts',(-2.42090763946779,1.,3.00264868585996));
#50761=CARTESIAN_POINT('Ctrl Pts',(-2.42421849439613,1.,3.00946442616658));
#50762=CARTESIAN_POINT('Ctrl Pts',(-2.42746856264168,1.,3.01630420830504));
#50763=CARTESIAN_POINT('Ctrl Pts',(-2.43063415586637,1.,3.02313656036004));
#50764=CARTESIAN_POINT('Ctrl Pts',(-2.43371241361488,1.,3.02995534946978));
#50765=CARTESIAN_POINT('Ctrl Pts',(-2.43671278042414,1.,3.03676949672821));
#50766=CARTESIAN_POINT('Ctrl Pts',(-2.43965194061857,1.,3.04359685040555));
#50767=CARTESIAN_POINT('Ctrl Pts',(-2.44254768923105,1.,3.05045678021504));
#50768=CARTESIAN_POINT('Ctrl Pts',(-2.44541251892556,1.,3.05736242671506));
#50769=CARTESIAN_POINT('Ctrl Pts',(-2.44824970516544,1.,3.06431596421405));
#50770=CARTESIAN_POINT('Ctrl Pts',(-2.45105688854422,1.,3.07131290521297));
#50771=CARTESIAN_POINT('Ctrl Pts',(-2.4538282678779,1.,3.07834472886139));
#50772=CARTESIAN_POINT('Ctrl Pts',(-2.45655725437039,1.,3.08540206545315));
#50773=CARTESIAN_POINT('Ctrl Pts',(-2.4592391256388,1.,3.09247787931887));
#50774=CARTESIAN_POINT('Ctrl Pts',(-2.46187308501884,1.,3.09956993697052));
#50775=CARTESIAN_POINT('Ctrl Pts',(-2.46446082979646,1.,3.1066790790198));
#50776=CARTESIAN_POINT('Ctrl Pts',(-2.46700558843506,1.,3.11380805536122));
#50777=CARTESIAN_POINT('Ctrl Pts',(-2.46951098947469,1.,3.12096015766983));
#50778=CARTESIAN_POINT('Ctrl Pts',(-2.47197997765871,1.,3.12813790805952));
#50779=CARTESIAN_POINT('Ctrl Pts',(-2.47441378371932,1.,3.13534181229295));
#50780=CARTESIAN_POINT('Ctrl Pts',(-2.47681245356109,1.,3.1425709954655));
#50781=CARTESIAN_POINT('Ctrl Pts',(-2.47917529057029,1.,3.14982373241352));
#50782=CARTESIAN_POINT('Ctrl Pts',(-2.48150133566571,1.,3.15709802322739));
#50783=CARTESIAN_POINT('Ctrl Pts',(-2.48378981792725,1.,3.16439213290161));
#50784=CARTESIAN_POINT('Ctrl Pts',(-2.48604065348587,1.,3.17170518863313));
#50785=CARTESIAN_POINT('Ctrl Pts',(-2.48825428288201,1.,3.17903698136622));
#50786=CARTESIAN_POINT('Ctrl Pts',(-2.49043146334059,1.,3.18638771282266));
#50787=CARTESIAN_POINT('Ctrl Pts',(-2.49257307239848,1.,3.19375775555798));
#50788=CARTESIAN_POINT('Ctrl Pts',(-2.49467992057755,1.,3.20114742397588));
#50789=CARTESIAN_POINT('Ctrl Pts',(-2.4967525264737,1.,3.20855669849836));
#50790=CARTESIAN_POINT('Ctrl Pts',(-2.4987911459939,1.,3.21598526261286));
#50791=CARTESIAN_POINT('Ctrl Pts',(-2.50079587201957,1.,3.22343262620503));
#50792=CARTESIAN_POINT('Ctrl Pts',(-2.50276671338111,1.,3.23089822320646));
#50793=CARTESIAN_POINT('Ctrl Pts',(-2.5047036758003,1.,3.23838151080319));
#50794=CARTESIAN_POINT('Ctrl Pts',(-2.506606859405,1.,3.24588208983849));
#50795=CARTESIAN_POINT('Ctrl Pts',(-2.50847647070723,1.,3.25339971460982));
#50796=CARTESIAN_POINT('Ctrl Pts',(-2.51031277813486,1.,3.26093423001434));
#50797=CARTESIAN_POINT('Ctrl Pts',(-2.51211608411423,1.,3.26848552888115));
#50798=CARTESIAN_POINT('Ctrl Pts',(-2.513886692704,1.,3.27605350473142));
#50799=CARTESIAN_POINT('Ctrl Pts',(-2.51562487464514,1.,3.28363799702982));
#50800=CARTESIAN_POINT('Ctrl Pts',(-2.51733085123797,1.,3.2912387729927));
#50801=CARTESIAN_POINT('Ctrl Pts',(-2.51900480701069,1.,3.29885556388352));
#50802=CARTESIAN_POINT('Ctrl Pts',(-2.52064689568511,1.,3.30648808815442));
#50803=CARTESIAN_POINT('Ctrl Pts',(-2.52225724871313,1.,3.31413607874645));
#50804=CARTESIAN_POINT('Ctrl Pts',(-2.5238359839626,1.,3.32179931078699));
#50805=CARTESIAN_POINT('Ctrl Pts',(-2.52538321164634,1.,3.32947762187533));
#50806=CARTESIAN_POINT('Ctrl Pts',(-2.52689902690158,1.,3.33717089999103));
#50807=CARTESIAN_POINT('Ctrl Pts',(-2.52808660915689,1.,3.34333744115511));
#50808=CARTESIAN_POINT('Ctrl Pts',(-2.52896321610703,1.,3.34796903576663));
#50809=CARTESIAN_POINT('Ctrl Pts',(-2.5295413654909,1.,3.35105973714071));
#50810=CARTESIAN_POINT('Ctrl Pts',(-2.52982887637028,1.,3.35260583073571));
#50811=CARTESIAN_POINT('Origin',(-2.52982887637028,0.,3.35260583073571));
#50812=CARTESIAN_POINT('',(-2.40675750623143,1.,3.44202241512147));
#50813=CARTESIAN_POINT('Origin',(0.,0.,0.));
#50814=CARTESIAN_POINT('',(-2.50410331873042,1.,2.79140942341378));
#50815=CARTESIAN_POINT('Origin',(0.,1.,0.));
#50816=CARTESIAN_POINT('Ctrl Pts',(-2.50410331873042,1.,2.79140942341378));
#50817=CARTESIAN_POINT('Ctrl Pts',(-2.50410331873042,0.666666666666667,
2.79140942341378));
#50818=CARTESIAN_POINT('Ctrl Pts',(-2.50410331873043,0.333333333333333,
2.79140942341378));
#50819=CARTESIAN_POINT('Ctrl Pts',(-2.50410331873043,-0.333333333333333,
2.79140942341378));
#50820=CARTESIAN_POINT('Ctrl Pts',(-2.50410331873043,-0.666666666666667,
2.79140942341378));
#50821=CARTESIAN_POINT('Ctrl Pts',(-2.50410331873043,-1.,2.79140942341378));
#50822=CARTESIAN_POINT('Ctrl Pts',(-2.91557726271063,-1.,3.02314558451372));
#50823=CARTESIAN_POINT('Ctrl Pts',(-2.91557726271063,1.,3.02314558451372));
#50824=CARTESIAN_POINT('Ctrl Pts',(-2.91409518070707,-1.,3.02261975104912));
#50825=CARTESIAN_POINT('Ctrl Pts',(-2.91409518070707,1.,3.02261975104912));
#50826=CARTESIAN_POINT('Ctrl Pts',(-2.91113297349052,-1.,3.02156522743299));
#50827=CARTESIAN_POINT('Ctrl Pts',(-2.91113297349052,1.,3.02156522743299));
#50828=CARTESIAN_POINT('Ctrl Pts',(-2.90669553303902,-1.,3.01997487194926));
#50829=CARTESIAN_POINT('Ctrl Pts',(-2.90669553303902,1.,3.01997487194926));
#50830=CARTESIAN_POINT('Ctrl Pts',(-2.90079069102661,-1.,3.01783725123646));
#50831=CARTESIAN_POINT('Ctrl Pts',(-2.90079069102661,1.,3.01783725123646));
#50832=CARTESIAN_POINT('Ctrl Pts',(-2.8934292556764,-1.,3.01513660433291));
#50833=CARTESIAN_POINT('Ctrl Pts',(-2.8934292556764,1.,3.01513660433291));
#50834=CARTESIAN_POINT('Ctrl Pts',(-2.88608751706796,-1.,3.01240727309568));
#50835=CARTESIAN_POINT('Ctrl Pts',(-2.88608751706796,1.,3.01240727309568));
#50836=CARTESIAN_POINT('Ctrl Pts',(-2.87876560072799,-1.,3.0096491810855));
#50837=CARTESIAN_POINT('Ctrl Pts',(-2.87876560072799,1.,3.0096491810855));
#50838=CARTESIAN_POINT('Ctrl Pts',(-2.87146368430104,-1.,3.00686224485374));
#50839=CARTESIAN_POINT('Ctrl Pts',(-2.87146368430104,1.,3.00686224485374));
#50840=CARTESIAN_POINT('Ctrl Pts',(-2.86418200833065,-1.,3.00404638316245));
#50841=CARTESIAN_POINT('Ctrl Pts',(-2.86418200833065,1.,3.00404638316245));
#50842=CARTESIAN_POINT('Ctrl Pts',(-2.85692085715129,-1.,3.0012015079552));
#50843=CARTESIAN_POINT('Ctrl Pts',(-2.85692085715129,1.,3.0012015079552));
#50844=CARTESIAN_POINT('Ctrl Pts',(-2.84968053289104,-1.,2.99832751144566));
#50845=CARTESIAN_POINT('Ctrl Pts',(-2.84968053289104,1.,2.99832751144566));
#50846=CARTESIAN_POINT('Ctrl Pts',(-2.84246132984334,-1.,2.995424253416));
#50847=CARTESIAN_POINT('Ctrl Pts',(-2.84246132984334,1.,2.995424253416));
#50848=CARTESIAN_POINT('Ctrl Pts',(-2.83526351254383,-1.,2.99249155170479));
#50849=CARTESIAN_POINT('Ctrl Pts',(-2.83526351254383,1.,2.99249155170479));
#50850=CARTESIAN_POINT('Ctrl Pts',(-2.82808728190402,-1.,2.98952916401699));
#50851=CARTESIAN_POINT('Ctrl Pts',(-2.82808728190402,1.,2.98952916401699));
#50852=CARTESIAN_POINT('Ctrl Pts',(-2.82093279065704,-1.,2.98653680669434));
#50853=CARTESIAN_POINT('Ctrl Pts',(-2.82093279065704,1.,2.98653680669434));
#50854=CARTESIAN_POINT('Ctrl Pts',(-2.81380019196454,-1.,2.9835141977994));
#50855=CARTESIAN_POINT('Ctrl Pts',(-2.81380019196454,1.,2.9835141977994));
#50856=CARTESIAN_POINT('Ctrl Pts',(-2.80668968101162,-1.,2.98046109647299));
#50857=CARTESIAN_POINT('Ctrl Pts',(-2.80668968101162,1.,2.98046109647299));
#50858=CARTESIAN_POINT('Ctrl Pts',(-2.79960153278186,-1.,2.97737733718242));
#50859=CARTESIAN_POINT('Ctrl Pts',(-2.79960153278186,1.,2.97737733718242));
#50860=CARTESIAN_POINT('Ctrl Pts',(-2.79253615718147,-1.,2.97426288347475));
#50861=CARTESIAN_POINT('Ctrl Pts',(-2.79253615718147,1.,2.97426288347475));
#50862=CARTESIAN_POINT('Ctrl Pts',(-2.78549409123657,-1.,2.97111781461349));
#50863=CARTESIAN_POINT('Ctrl Pts',(-2.78549409123657,1.,2.97111781461349));
#50864=CARTESIAN_POINT('Ctrl Pts',(-2.77847589542767,-1.,2.9679422104295));
#50865=CARTESIAN_POINT('Ctrl Pts',(-2.77847589542767,1.,2.9679422104295));
#50866=CARTESIAN_POINT('Ctrl Pts',(-2.77148206836464,-1.,2.96473605585548));
#50867=CARTESIAN_POINT('Ctrl Pts',(-2.77148206836464,1.,2.96473605585548));
#50868=CARTESIAN_POINT('Ctrl Pts',(-2.76451296269571,-1.,2.96149914764832));
#50869=CARTESIAN_POINT('Ctrl Pts',(-2.76451296269571,1.,2.96149914764832));
#50870=CARTESIAN_POINT('Ctrl Pts',(-2.75756867888393,-1.,2.9582309766594));
#50871=CARTESIAN_POINT('Ctrl Pts',(-2.75756867888393,1.,2.9582309766594));
#50872=CARTESIAN_POINT('Ctrl Pts',(-2.75064903318996,-1.,2.95493069316211));
#50873=CARTESIAN_POINT('Ctrl Pts',(-2.75064903318996,1.,2.95493069316211));
#50874=CARTESIAN_POINT('Ctrl Pts',(-2.7437537949221,-1.,2.95159737214305));
#50875=CARTESIAN_POINT('Ctrl Pts',(-2.7437537949221,1.,2.95159737214305));
#50876=CARTESIAN_POINT('Ctrl Pts',(-2.73688288329825,-1.,2.94823023414381));
#50877=CARTESIAN_POINT('Ctrl Pts',(-2.73688288329825,1.,2.94823023414381));
#50878=CARTESIAN_POINT('Ctrl Pts',(-2.73003657371613,-1.,2.94482887675139));
#50879=CARTESIAN_POINT('Ctrl Pts',(-2.73003657371613,1.,2.94482887675139));
#50880=CARTESIAN_POINT('Ctrl Pts',(-2.72321571511322,-1.,2.94139351933882));
#50881=CARTESIAN_POINT('Ctrl Pts',(-2.72321571511322,1.,2.94139351933882));
#50882=CARTESIAN_POINT('Ctrl Pts',(-2.71642190053575,-1.,2.93792519474955));
#50883=CARTESIAN_POINT('Ctrl Pts',(-2.71642190053575,1.,2.93792519474955));
#50884=CARTESIAN_POINT('Ctrl Pts',(-2.70965695523776,-1.,2.93442516311168));
#50885=CARTESIAN_POINT('Ctrl Pts',(-2.70965695523776,1.,2.93442516311168));
#50886=CARTESIAN_POINT('Ctrl Pts',(-2.70292247416881,-1.,2.93089438233746));
#50887=CARTESIAN_POINT('Ctrl Pts',(-2.70292247416881,1.,2.93089438233746));
#50888=CARTESIAN_POINT('Ctrl Pts',(-2.69621932864302,-1.,2.92733294395268));
#50889=CARTESIAN_POINT('Ctrl Pts',(-2.69621932864302,1.,2.92733294395268));
#50890=CARTESIAN_POINT('Ctrl Pts',(-2.68954721165342,-1.,2.92373955325876));
#50891=CARTESIAN_POINT('Ctrl Pts',(-2.68954721165342,1.,2.92373955325876));
#50892=CARTESIAN_POINT('Ctrl Pts',(-2.68290409279689,-1.,2.92011090722152));
#50893=CARTESIAN_POINT('Ctrl Pts',(-2.68290409279689,1.,2.92011090722152));
#50894=CARTESIAN_POINT('Ctrl Pts',(-2.67628728855309,-1.,2.91644290704281));
#50895=CARTESIAN_POINT('Ctrl Pts',(-2.67628728855309,1.,2.91644290704281));
#50896=CARTESIAN_POINT('Ctrl Pts',(-2.66969458792627,-1.,2.91273193382876));
#50897=CARTESIAN_POINT('Ctrl Pts',(-2.66969458792627,1.,2.91273193382876));
#50898=CARTESIAN_POINT('Ctrl Pts',(-2.66312542616809,-1.,2.90897617968921));
#50899=CARTESIAN_POINT('Ctrl Pts',(-2.66312542616809,1.,2.90897617968921));
#50900=CARTESIAN_POINT('Ctrl Pts',(-2.65658188464287,-1.,2.90517678087467));
#50901=CARTESIAN_POINT('Ctrl Pts',(-2.65658188464287,1.,2.90517678087467));
#50902=CARTESIAN_POINT('Ctrl Pts',(-2.65007017365576,-1.,2.90133950224879));
#50903=CARTESIAN_POINT('Ctrl Pts',(-2.65007017365576,1.,2.90133950224879));
#50904=CARTESIAN_POINT('Ctrl Pts',(-2.64359851684146,-1.,2.89747231723361));
#50905=CARTESIAN_POINT('Ctrl Pts',(-2.64359851684146,1.,2.89747231723361));
#50906=CARTESIAN_POINT('Ctrl Pts',(-2.63717442263944,-1.,2.89358228854557));
#50907=CARTESIAN_POINT('Ctrl Pts',(-2.63717442263944,1.,2.89358228854557));
#50908=CARTESIAN_POINT('Ctrl Pts',(-2.63080195420771,-1.,2.88967244854243));
#50909=CARTESIAN_POINT('Ctrl Pts',(-2.63080195420771,1.,2.88967244854243));
#50910=CARTESIAN_POINT('Ctrl Pts',(-2.62447947640253,-1.,2.88573922195049));
#50911=CARTESIAN_POINT('Ctrl Pts',(-2.62447947640253,1.,2.88573922195049));
#50912=CARTESIAN_POINT('Ctrl Pts',(-2.61819596473087,-1.,2.88176821427502));
#50913=CARTESIAN_POINT('Ctrl Pts',(-2.61819596473087,1.,2.88176821427502));
#50914=CARTESIAN_POINT('Ctrl Pts',(-2.61193507170928,-1.,2.87773881947885));
#50915=CARTESIAN_POINT('Ctrl Pts',(-2.61193507170928,1.,2.87773881947885));
#50916=CARTESIAN_POINT('Ctrl Pts',(-2.6056817788128,-1.,2.87363176656475));
#50917=CARTESIAN_POINT('Ctrl Pts',(-2.6056817788128,1.,2.87363176656475));
#50918=CARTESIAN_POINT('Ctrl Pts',(-2.59942875223202,-1.,2.86943633170712));
#50919=CARTESIAN_POINT('Ctrl Pts',(-2.59942875223202,1.,2.86943633170712));
#50920=CARTESIAN_POINT('Ctrl Pts',(-2.59318160184921,-1.,2.86515629953528));
#50921=CARTESIAN_POINT('Ctrl Pts',(-2.59318160184921,1.,2.86515629953528));
#50922=CARTESIAN_POINT('Ctrl Pts',(-2.5869677064356,-1.,2.86081999003668));
#50923=CARTESIAN_POINT('Ctrl Pts',(-2.5869677064356,1.,2.86081999003668));
#50924=CARTESIAN_POINT('Ctrl Pts',(-2.58082875254407,-1.,2.85647171715147));
#50925=CARTESIAN_POINT('Ctrl Pts',(-2.58082875254407,1.,2.85647171715147));
#50926=CARTESIAN_POINT('Ctrl Pts',(-2.57480482727128,-1.,2.85215360144483));
#50927=CARTESIAN_POINT('Ctrl Pts',(-2.57480482727128,1.,2.85215360144483));
#50928=CARTESIAN_POINT('Ctrl Pts',(-2.56891984251743,-1.,2.84788893329091));
#50929=CARTESIAN_POINT('Ctrl Pts',(-2.56891984251743,1.,2.84788893329091));
#50930=CARTESIAN_POINT('Ctrl Pts',(-2.56316920798489,-1.,2.84366802680211));
#50931=CARTESIAN_POINT('Ctrl Pts',(-2.56316920798489,1.,2.84366802680211));
#50932=CARTESIAN_POINT('Ctrl Pts',(-2.55749952145165,-1.,2.83942515220699));
#50933=CARTESIAN_POINT('Ctrl Pts',(-2.55749952145165,1.,2.83942515220699));
#50934=CARTESIAN_POINT('Ctrl Pts',(-2.55182152806964,-1.,2.83505269592412));
#50935=CARTESIAN_POINT('Ctrl Pts',(-2.55182152806964,1.,2.83505269592412));
#50936=CARTESIAN_POINT('Ctrl Pts',(-2.54604736792542,-1.,2.83044254225794));
#50937=CARTESIAN_POINT('Ctrl Pts',(-2.54604736792542,1.,2.83044254225794));
#50938=CARTESIAN_POINT('Ctrl Pts',(-2.54012272520141,-1.,2.82552167649157));
#50939=CARTESIAN_POINT('Ctrl Pts',(-2.54012272520141,1.,2.82552167649157));
#50940=CARTESIAN_POINT('Ctrl Pts',(-2.53405679667463,-1.,2.82028550483744));
#50941=CARTESIAN_POINT('Ctrl Pts',(-2.53405679667463,1.,2.82028550483744));
#50942=CARTESIAN_POINT('Ctrl Pts',(-2.52796388055457,-1.,2.8148437904867));
#50943=CARTESIAN_POINT('Ctrl Pts',(-2.52796388055457,1.,2.8148437904867));
#50944=CARTESIAN_POINT('Ctrl Pts',(-2.52205778589922,-1.,2.80941521967234));
#50945=CARTESIAN_POINT('Ctrl Pts',(-2.52205778589922,1.,2.80941521967234));
#50946=CARTESIAN_POINT('Ctrl Pts',(-2.51660190466067,-1.,2.80427363984939));
#50947=CARTESIAN_POINT('Ctrl Pts',(-2.51660190466067,1.,2.80427363984939));
#50948=CARTESIAN_POINT('Ctrl Pts',(-2.51186983687947,-1.,2.79970585014308));
#50949=CARTESIAN_POINT('Ctrl Pts',(-2.51186983687947,1.,2.79970585014308));
#50950=CARTESIAN_POINT('Ctrl Pts',(-2.50810555977564,-1.,2.7959687805717));
#50951=CARTESIAN_POINT('Ctrl Pts',(-2.50810555977564,1.,2.7959687805717));
#50952=CARTESIAN_POINT('Ctrl Pts',(-2.50547439929077,-1.,2.79323694088143));
#50953=CARTESIAN_POINT('Ctrl Pts',(-2.50547439929077,1.,2.79323694088143));
#50954=CARTESIAN_POINT('Ctrl Pts',(-2.50433799076945,-1.,2.79192122906739));
#50955=CARTESIAN_POINT('Ctrl Pts',(-2.50433799076945,1.,2.79192122906739));
#50956=CARTESIAN_POINT('Ctrl Pts',(-2.50404230339032,-1.,2.79143626022225));
#50957=CARTESIAN_POINT('Ctrl Pts',(-2.50404230339032,1.,2.79143626022225));
#50958=CARTESIAN_POINT('Ctrl Pts',(-2.50409239460011,-1.,2.79133581100044));
#50959=CARTESIAN_POINT('Ctrl Pts',(-2.50409239460011,1.,2.79133581100044));
#50960=CARTESIAN_POINT('Ctrl Pts',(-2.50417924854921,-1.,2.79134130681569));
#50961=CARTESIAN_POINT('Ctrl Pts',(-2.50417924854921,1.,2.79134130681569));
#50962=CARTESIAN_POINT('',(-2.91557726271063,1.,3.02314558451372));
#50963=CARTESIAN_POINT('Ctrl Pts',(-2.91557726271063,1.,3.02314558451372));
#50964=CARTESIAN_POINT('Ctrl Pts',(-2.91409518070707,1.,3.02261975104912));
#50965=CARTESIAN_POINT('Ctrl Pts',(-2.91113297349052,1.,3.02156522743299));
#50966=CARTESIAN_POINT('Ctrl Pts',(-2.90669553303902,1.,3.01997487194926));
#50967=CARTESIAN_POINT('Ctrl Pts',(-2.90079069102661,1.,3.01783725123646));
#50968=CARTESIAN_POINT('Ctrl Pts',(-2.8934292556764,1.,3.01513660433291));
#50969=CARTESIAN_POINT('Ctrl Pts',(-2.88608751706796,1.,3.01240727309568));
#50970=CARTESIAN_POINT('Ctrl Pts',(-2.87876560072799,1.,3.0096491810855));
#50971=CARTESIAN_POINT('Ctrl Pts',(-2.87146368430104,1.,3.00686224485374));
#50972=CARTESIAN_POINT('Ctrl Pts',(-2.86418200833065,1.,3.00404638316245));
#50973=CARTESIAN_POINT('Ctrl Pts',(-2.85692085715129,1.,3.0012015079552));
#50974=CARTESIAN_POINT('Ctrl Pts',(-2.84968053289104,1.,2.99832751144566));
#50975=CARTESIAN_POINT('Ctrl Pts',(-2.84246132984334,1.,2.995424253416));
#50976=CARTESIAN_POINT('Ctrl Pts',(-2.83526351254383,1.,2.99249155170479));
#50977=CARTESIAN_POINT('Ctrl Pts',(-2.82808728190402,1.,2.98952916401699));
#50978=CARTESIAN_POINT('Ctrl Pts',(-2.82093279065704,1.,2.98653680669434));
#50979=CARTESIAN_POINT('Ctrl Pts',(-2.81380019196454,1.,2.9835141977994));
#50980=CARTESIAN_POINT('Ctrl Pts',(-2.80668968101162,1.,2.98046109647299));
#50981=CARTESIAN_POINT('Ctrl Pts',(-2.79960153278186,1.,2.97737733718242));
#50982=CARTESIAN_POINT('Ctrl Pts',(-2.79253615718147,1.,2.97426288347475));
#50983=CARTESIAN_POINT('Ctrl Pts',(-2.78549409123657,1.,2.97111781461349));
#50984=CARTESIAN_POINT('Ctrl Pts',(-2.77847589542767,1.,2.9679422104295));
#50985=CARTESIAN_POINT('Ctrl Pts',(-2.77148206836464,1.,2.96473605585548));
#50986=CARTESIAN_POINT('Ctrl Pts',(-2.76451296269571,1.,2.96149914764832));
#50987=CARTESIAN_POINT('Ctrl Pts',(-2.75756867888393,1.,2.9582309766594));
#50988=CARTESIAN_POINT('Ctrl Pts',(-2.75064903318996,1.,2.95493069316211));
#50989=CARTESIAN_POINT('Ctrl Pts',(-2.7437537949221,1.,2.95159737214305));
#50990=CARTESIAN_POINT('Ctrl Pts',(-2.73688288329825,1.,2.94823023414381));
#50991=CARTESIAN_POINT('Ctrl Pts',(-2.73003657371613,1.,2.94482887675139));
#50992=CARTESIAN_POINT('Ctrl Pts',(-2.72321571511322,1.,2.94139351933882));
#50993=CARTESIAN_POINT('Ctrl Pts',(-2.71642190053575,1.,2.93792519474955));
#50994=CARTESIAN_POINT('Ctrl Pts',(-2.70965695523776,1.,2.93442516311168));
#50995=CARTESIAN_POINT('Ctrl Pts',(-2.70292247416881,1.,2.93089438233746));
#50996=CARTESIAN_POINT('Ctrl Pts',(-2.69621932864302,1.,2.92733294395268));
#50997=CARTESIAN_POINT('Ctrl Pts',(-2.68954721165342,1.,2.92373955325876));
#50998=CARTESIAN_POINT('Ctrl Pts',(-2.68290409279689,1.,2.92011090722152));
#50999=CARTESIAN_POINT('Ctrl Pts',(-2.67628728855309,1.,2.91644290704281));
#51000=CARTESIAN_POINT('Ctrl Pts',(-2.66969458792627,1.,2.91273193382876));
#51001=CARTESIAN_POINT('Ctrl Pts',(-2.66312542616809,1.,2.90897617968921));
#51002=CARTESIAN_POINT('Ctrl Pts',(-2.65658188464287,1.,2.90517678087467));
#51003=CARTESIAN_POINT('Ctrl Pts',(-2.65007017365576,1.,2.90133950224879));
#51004=CARTESIAN_POINT('Ctrl Pts',(-2.64359851684146,1.,2.89747231723361));
#51005=CARTESIAN_POINT('Ctrl Pts',(-2.63717442263944,1.,2.89358228854557));
#51006=CARTESIAN_POINT('Ctrl Pts',(-2.63080195420771,1.,2.88967244854243));
#51007=CARTESIAN_POINT('Ctrl Pts',(-2.62447947640253,1.,2.88573922195049));
#51008=CARTESIAN_POINT('Ctrl Pts',(-2.61819596473087,1.,2.88176821427502));
#51009=CARTESIAN_POINT('Ctrl Pts',(-2.61193507170928,1.,2.87773881947885));
#51010=CARTESIAN_POINT('Ctrl Pts',(-2.6056817788128,1.,2.87363176656475));
#51011=CARTESIAN_POINT('Ctrl Pts',(-2.59942875223202,1.,2.86943633170712));
#51012=CARTESIAN_POINT('Ctrl Pts',(-2.59318160184921,1.,2.86515629953528));
#51013=CARTESIAN_POINT('Ctrl Pts',(-2.5869677064356,1.,2.86081999003668));
#51014=CARTESIAN_POINT('Ctrl Pts',(-2.58082875254407,1.,2.85647171715147));
#51015=CARTESIAN_POINT('Ctrl Pts',(-2.57480482727128,1.,2.85215360144483));
#51016=CARTESIAN_POINT('Ctrl Pts',(-2.56891984251743,1.,2.84788893329091));
#51017=CARTESIAN_POINT('Ctrl Pts',(-2.56316920798489,1.,2.84366802680211));
#51018=CARTESIAN_POINT('Ctrl Pts',(-2.55749952145165,1.,2.83942515220699));
#51019=CARTESIAN_POINT('Ctrl Pts',(-2.55182152806964,1.,2.83505269592412));
#51020=CARTESIAN_POINT('Ctrl Pts',(-2.54604736792542,1.,2.83044254225794));
#51021=CARTESIAN_POINT('Ctrl Pts',(-2.54012272520141,1.,2.82552167649157));
#51022=CARTESIAN_POINT('Ctrl Pts',(-2.53405679667463,1.,2.82028550483744));
#51023=CARTESIAN_POINT('Ctrl Pts',(-2.52796388055457,1.,2.8148437904867));
#51024=CARTESIAN_POINT('Ctrl Pts',(-2.52205778589922,1.,2.80941521967234));
#51025=CARTESIAN_POINT('Ctrl Pts',(-2.51660190466067,1.,2.80427363984939));
#51026=CARTESIAN_POINT('Ctrl Pts',(-2.51186983687947,1.,2.79970585014308));
#51027=CARTESIAN_POINT('Ctrl Pts',(-2.50810555977564,1.,2.7959687805717));
#51028=CARTESIAN_POINT('Ctrl Pts',(-2.50567182569153,1.,2.79344192164204));
#51029=CARTESIAN_POINT('Ctrl Pts',(-2.50455968395235,1.,2.79217568804874));
#51030=CARTESIAN_POINT('Ctrl Pts',(-2.50417932839343,1.,2.79164172519039));
#51031=CARTESIAN_POINT('Ctrl Pts',(-2.50410700351427,1.,2.79145823440899));
#51032=CARTESIAN_POINT('Ctrl Pts',(-2.50410331873043,1.,2.79140942341378));
#51033=CARTESIAN_POINT('',(-2.91557726271063,0.,3.02314558451372));
#51034=CARTESIAN_POINT('Ctrl Pts',(-2.79134130681569,-1.,2.50417924854921));
#51035=CARTESIAN_POINT('Ctrl Pts',(-2.79134130681569,1.,2.50417924854921));
#51036=CARTESIAN_POINT('Ctrl Pts',(-2.7913358110015,-1.,2.50409239460108));
#51037=CARTESIAN_POINT('Ctrl Pts',(-2.7913358110015,1.,2.50409239460108));
#51038=CARTESIAN_POINT('Ctrl Pts',(-2.79143626022503,-1.,2.50404230339286));
#51039=CARTESIAN_POINT('Ctrl Pts',(-2.79143626022503,1.,2.50404230339286));
#51040=CARTESIAN_POINT('Ctrl Pts',(-2.79192122907148,-1.,2.5043379907732));
#51041=CARTESIAN_POINT('Ctrl Pts',(-2.79192122907148,1.,2.5043379907732));
#51042=CARTESIAN_POINT('Ctrl Pts',(-2.7932369408851,-1.,2.50547439929414));
#51043=CARTESIAN_POINT('Ctrl Pts',(-2.7932369408851,1.,2.50547439929414));
#51044=CARTESIAN_POINT('Ctrl Pts',(-2.79596878057287,-1.,2.50810555977671));
#51045=CARTESIAN_POINT('Ctrl Pts',(-2.79596878057287,1.,2.50810555977671));
#51046=CARTESIAN_POINT('Ctrl Pts',(-2.79970585014168,-1.,2.51186983687818));
#51047=CARTESIAN_POINT('Ctrl Pts',(-2.79970585014168,1.,2.51186983687818));
#51048=CARTESIAN_POINT('Ctrl Pts',(-2.80427363984653,-1.,2.51660190465805));
#51049=CARTESIAN_POINT('Ctrl Pts',(-2.80427363984653,1.,2.51660190465805));
#51050=CARTESIAN_POINT('Ctrl Pts',(-2.80941521966941,-1.,2.52205778589653));
#51051=CARTESIAN_POINT('Ctrl Pts',(-2.80941521966941,1.,2.52205778589653));
#51052=CARTESIAN_POINT('Ctrl Pts',(-2.81484379048475,-1.,2.52796388055278));
#51053=CARTESIAN_POINT('Ctrl Pts',(-2.81484379048475,1.,2.52796388055278));
#51054=CARTESIAN_POINT('Ctrl Pts',(-2.82028550483689,-1.,2.53405679667412));
#51055=CARTESIAN_POINT('Ctrl Pts',(-2.82028550483689,1.,2.53405679667412));
#51056=CARTESIAN_POINT('Ctrl Pts',(-2.8255216764922,-1.,2.54012272520199));
#51057=CARTESIAN_POINT('Ctrl Pts',(-2.8255216764922,1.,2.54012272520199));
#51058=CARTESIAN_POINT('Ctrl Pts',(-2.83044254225917,-1.,2.54604736792655));
#51059=CARTESIAN_POINT('Ctrl Pts',(-2.83044254225917,1.,2.54604736792655));
#51060=CARTESIAN_POINT('Ctrl Pts',(-2.83505269592536,-1.,2.55182152807077));
#51061=CARTESIAN_POINT('Ctrl Pts',(-2.83505269592536,1.,2.55182152807077));
#51062=CARTESIAN_POINT('Ctrl Pts',(-2.83942515220782,-1.,2.55749952145241));
#51063=CARTESIAN_POINT('Ctrl Pts',(-2.83942515220782,1.,2.55749952145241));
#51064=CARTESIAN_POINT('Ctrl Pts',(-2.84366802680237,-1.,2.56316920798513));
#51065=CARTESIAN_POINT('Ctrl Pts',(-2.84366802680237,1.,2.56316920798513));
#51066=CARTESIAN_POINT('Ctrl Pts',(-2.84788893329067,-1.,2.56891984251721));
#51067=CARTESIAN_POINT('Ctrl Pts',(-2.84788893329067,1.,2.56891984251721));
#51068=CARTESIAN_POINT('Ctrl Pts',(-2.85215360144431,-1.,2.57480482727081));
#51069=CARTESIAN_POINT('Ctrl Pts',(-2.85215360144431,1.,2.57480482727081));
#51070=CARTESIAN_POINT('Ctrl Pts',(-2.85647171715092,-1.,2.58082875254357));
#51071=CARTESIAN_POINT('Ctrl Pts',(-2.85647171715092,1.,2.58082875254357));
#51072=CARTESIAN_POINT('Ctrl Pts',(-2.86081999003629,-1.,2.58696770643524));
#51073=CARTESIAN_POINT('Ctrl Pts',(-2.86081999003629,1.,2.58696770643524));
#51074=CARTESIAN_POINT('Ctrl Pts',(-2.86515629953513,-1.,2.59318160184908));
#51075=CARTESIAN_POINT('Ctrl Pts',(-2.86515629953513,1.,2.59318160184908));
#51076=CARTESIAN_POINT('Ctrl Pts',(-2.86943633170722,-1.,2.5994287522321));
#51077=CARTESIAN_POINT('Ctrl Pts',(-2.86943633170722,1.,2.5994287522321));
#51078=CARTESIAN_POINT('Ctrl Pts',(-2.87363176656501,-1.,2.60568177881303));
#51079=CARTESIAN_POINT('Ctrl Pts',(-2.87363176656501,1.,2.60568177881303));
#51080=CARTESIAN_POINT('Ctrl Pts',(-2.87773881947916,-1.,2.61193507170955));
#51081=CARTESIAN_POINT('Ctrl Pts',(-2.87773881947916,1.,2.61193507170955));
#51082=CARTESIAN_POINT('Ctrl Pts',(-2.88176821427525,-1.,2.61819596473108));
#51083=CARTESIAN_POINT('Ctrl Pts',(-2.88176821427525,1.,2.61819596473108));
#51084=CARTESIAN_POINT('Ctrl Pts',(-2.88573922195059,-1.,2.62447947640262));
#51085=CARTESIAN_POINT('Ctrl Pts',(-2.88573922195059,1.,2.62447947640262));
#51086=CARTESIAN_POINT('Ctrl Pts',(-2.88967244854239,-1.,2.63080195420767));
#51087=CARTESIAN_POINT('Ctrl Pts',(-2.88967244854239,1.,2.63080195420767));
#51088=CARTESIAN_POINT('Ctrl Pts',(-2.89358228854544,-1.,2.63717442263932));
#51089=CARTESIAN_POINT('Ctrl Pts',(-2.89358228854544,1.,2.63717442263932));
#51090=CARTESIAN_POINT('Ctrl Pts',(-2.89747231723345,-1.,2.64359851684131));
#51091=CARTESIAN_POINT('Ctrl Pts',(-2.89747231723345,1.,2.64359851684131));
#51092=CARTESIAN_POINT('Ctrl Pts',(-2.90133950224867,-1.,2.65007017365564));
#51093=CARTESIAN_POINT('Ctrl Pts',(-2.90133950224867,1.,2.65007017365564));
#51094=CARTESIAN_POINT('Ctrl Pts',(-2.90517678087461,-1.,2.65658188464282));
#51095=CARTESIAN_POINT('Ctrl Pts',(-2.90517678087461,1.,2.65658188464282));
#51096=CARTESIAN_POINT('Ctrl Pts',(-2.90897617968923,-1.,2.6631254261681));
#51097=CARTESIAN_POINT('Ctrl Pts',(-2.90897617968923,1.,2.6631254261681));
#51098=CARTESIAN_POINT('Ctrl Pts',(-2.91273193382882,-1.,2.66969458792631));
#51099=CARTESIAN_POINT('Ctrl Pts',(-2.91273193382882,1.,2.66969458792631));
#51100=CARTESIAN_POINT('Ctrl Pts',(-2.91644290704285,-1.,2.67628728855312));
#51101=CARTESIAN_POINT('Ctrl Pts',(-2.91644290704285,1.,2.67628728855312));
#51102=CARTESIAN_POINT('Ctrl Pts',(-2.92011090722152,-1.,2.68290409279688));
#51103=CARTESIAN_POINT('Ctrl Pts',(-2.92011090722152,1.,2.68290409279688));
#51104=CARTESIAN_POINT('Ctrl Pts',(-2.92373955325875,-1.,2.68954721165339));
#51105=CARTESIAN_POINT('Ctrl Pts',(-2.92373955325875,1.,2.68954721165339));
#51106=CARTESIAN_POINT('Ctrl Pts',(-2.92733294395267,-1.,2.69621932864301));
#51107=CARTESIAN_POINT('Ctrl Pts',(-2.92733294395267,1.,2.69621932864301));
#51108=CARTESIAN_POINT('Ctrl Pts',(-2.9308943823375,-1.,2.70292247416885));
#51109=CARTESIAN_POINT('Ctrl Pts',(-2.9308943823375,1.,2.70292247416885));
#51110=CARTESIAN_POINT('Ctrl Pts',(-2.93442516311179,-1.,2.70965695523787));
#51111=CARTESIAN_POINT('Ctrl Pts',(-2.93442516311179,1.,2.70965695523787));
#51112=CARTESIAN_POINT('Ctrl Pts',(-2.93792519474972,-1.,2.71642190053592));
#51113=CARTESIAN_POINT('Ctrl Pts',(-2.93792519474972,1.,2.71642190053592));
#51114=CARTESIAN_POINT('Ctrl Pts',(-2.94139351933897,-1.,2.72321571511337));
#51115=CARTESIAN_POINT('Ctrl Pts',(-2.94139351933897,1.,2.72321571511337));
#51116=CARTESIAN_POINT('Ctrl Pts',(-2.94482887675143,-1.,2.73003657371617));
#51117=CARTESIAN_POINT('Ctrl Pts',(-2.94482887675143,1.,2.73003657371617));
#51118=CARTESIAN_POINT('Ctrl Pts',(-2.94823023414364,-1.,2.73688288329808));
#51119=CARTESIAN_POINT('Ctrl Pts',(-2.94823023414364,1.,2.73688288329808));
#51120=CARTESIAN_POINT('Ctrl Pts',(-2.95159737214266,-1.,2.74375379492172));
#51121=CARTESIAN_POINT('Ctrl Pts',(-2.95159737214266,1.,2.74375379492172));
#51122=CARTESIAN_POINT('Ctrl Pts',(-2.95493069316161,-1.,2.75064903318947));
#51123=CARTESIAN_POINT('Ctrl Pts',(-2.95493069316161,1.,2.75064903318947));
#51124=CARTESIAN_POINT('Ctrl Pts',(-2.95823097665896,-1.,2.7575686788835));
#51125=CARTESIAN_POINT('Ctrl Pts',(-2.95823097665896,1.,2.7575686788835));
#51126=CARTESIAN_POINT('Ctrl Pts',(-2.96149914764818,-1.,2.76451296269557));
#51127=CARTESIAN_POINT('Ctrl Pts',(-2.96149914764818,1.,2.76451296269557));
#51128=CARTESIAN_POINT('Ctrl Pts',(-2.96473605585583,-1.,2.77148206836498));
#51129=CARTESIAN_POINT('Ctrl Pts',(-2.96473605585583,1.,2.77148206836498));
#51130=CARTESIAN_POINT('Ctrl Pts',(-2.96794221043036,-1.,2.7784758954285));
#51131=CARTESIAN_POINT('Ctrl Pts',(-2.96794221043036,1.,2.7784758954285));
#51132=CARTESIAN_POINT('Ctrl Pts',(-2.97111781461465,-1.,2.78549409123769));
#51133=CARTESIAN_POINT('Ctrl Pts',(-2.97111781461465,1.,2.78549409123769));
#51134=CARTESIAN_POINT('Ctrl Pts',(-2.9742628834758,-1.,2.79253615718248));
#51135=CARTESIAN_POINT('Ctrl Pts',(-2.9742628834758,1.,2.79253615718248));
#51136=CARTESIAN_POINT('Ctrl Pts',(-2.97737733718287,-1.,2.7996015327823));
#51137=CARTESIAN_POINT('Ctrl Pts',(-2.97737733718287,1.,2.7996015327823));
#51138=CARTESIAN_POINT('Ctrl Pts',(-2.98046109647241,-1.,2.80668968101106));
#51139=CARTESIAN_POINT('Ctrl Pts',(-2.98046109647241,1.,2.80668968101106));
#51140=CARTESIAN_POINT('Ctrl Pts',(-2.98351419779767,-1.,2.81380019196286));
#51141=CARTESIAN_POINT('Ctrl Pts',(-2.98351419779767,1.,2.81380019196286));
#51142=CARTESIAN_POINT('Ctrl Pts',(-2.9865368066918,-1.,2.82093279065457));
#51143=CARTESIAN_POINT('Ctrl Pts',(-2.9865368066918,1.,2.82093279065457));
#51144=CARTESIAN_POINT('Ctrl Pts',(-2.98952916401446,-1.,2.82808728190157));
#51145=CARTESIAN_POINT('Ctrl Pts',(-2.98952916401446,1.,2.82808728190157));
#51146=CARTESIAN_POINT('Ctrl Pts',(-2.9924915517034,-1.,2.83526351254248));
#51147=CARTESIAN_POINT('Ctrl Pts',(-2.9924915517034,1.,2.83526351254248));
#51148=CARTESIAN_POINT('Ctrl Pts',(-2.99542425341685,-1.,2.84246132984415));
#51149=CARTESIAN_POINT('Ctrl Pts',(-2.99542425341685,1.,2.84246132984415));
#51150=CARTESIAN_POINT('Ctrl Pts',(-2.99832751144925,-1.,2.84968053289451));
#51151=CARTESIAN_POINT('Ctrl Pts',(-2.99832751144925,1.,2.84968053289451));
#51152=CARTESIAN_POINT('Ctrl Pts',(-3.00120150796095,-1.,2.85692085715686));
#51153=CARTESIAN_POINT('Ctrl Pts',(-3.00120150796095,1.,2.85692085715686));
#51154=CARTESIAN_POINT('Ctrl Pts',(-3.00404638316867,-1.,2.86418200833667));
#51155=CARTESIAN_POINT('Ctrl Pts',(-3.00404638316867,1.,2.86418200833667));
#51156=CARTESIAN_POINT('Ctrl Pts',(-3.00686224485784,-1.,2.87146368430502));
#51157=CARTESIAN_POINT('Ctrl Pts',(-3.00686224485784,1.,2.87146368430502));
#51158=CARTESIAN_POINT('Ctrl Pts',(-3.00964918108476,-1.,2.87876560072727));
#51159=CARTESIAN_POINT('Ctrl Pts',(-3.00964918108476,1.,2.87876560072727));
#51160=CARTESIAN_POINT('Ctrl Pts',(-3.01240727308829,-1.,2.8860875170608));
#51161=CARTESIAN_POINT('Ctrl Pts',(-3.01240727308829,1.,2.8860875170608));
#51162=CARTESIAN_POINT('Ctrl Pts',(-3.01513660431928,-1.,2.89342925566321));
#51163=CARTESIAN_POINT('Ctrl Pts',(-3.01513660431928,1.,2.89342925566321));
#51164=CARTESIAN_POINT('Ctrl Pts',(-3.01783725121981,-1.,2.9007906910105));
#51165=CARTESIAN_POINT('Ctrl Pts',(-3.01783725121981,1.,2.9007906910105));
#51166=CARTESIAN_POINT('Ctrl Pts',(-3.01997487193503,-1.,2.90669553302526));
#51167=CARTESIAN_POINT('Ctrl Pts',(-3.01997487193503,1.,2.90669553302526));
#51168=CARTESIAN_POINT('Ctrl Pts',(-3.02156522742431,-1.,2.91113297348212));
#51169=CARTESIAN_POINT('Ctrl Pts',(-3.02156522742431,1.,2.91113297348212));
#51170=CARTESIAN_POINT('Ctrl Pts',(-3.02261975104593,-1.,2.91409518070399));
#51171=CARTESIAN_POINT('Ctrl Pts',(-3.02261975104593,1.,2.91409518070399));
#51172=CARTESIAN_POINT('Ctrl Pts',(-3.02314558451372,-1.,2.91557726271063));
#51173=CARTESIAN_POINT('Ctrl Pts',(-3.02314558451372,1.,2.91557726271063));
#51174=CARTESIAN_POINT('',(-2.79140942341258,1.,2.50410331873176));
#51175=CARTESIAN_POINT('Ctrl Pts',(-2.79140942341258,-1.,2.50410331873176));
#51176=CARTESIAN_POINT('Ctrl Pts',(-2.79140942341258,-0.666666666666667,
2.50410331873176));
#51177=CARTESIAN_POINT('Ctrl Pts',(-2.79140942341258,-0.333333333333333,
2.50410331873176));
#51178=CARTESIAN_POINT('Ctrl Pts',(-2.79140942341258,0.333333333333333,
2.50410331873176));
#51179=CARTESIAN_POINT('Ctrl Pts',(-2.79140942341258,0.666666666666667,
2.50410331873176));
#51180=CARTESIAN_POINT('Ctrl Pts',(-2.79140942341258,1.,2.50410331873176));
#51181=CARTESIAN_POINT('',(-3.02314558451372,1.,2.91557726271063));
#51182=CARTESIAN_POINT('',(-3.02314558451372,0.,2.91557726271063));
#51183=CARTESIAN_POINT('Ctrl Pts',(-2.79140942341258,1.,2.50410331873176));
#51184=CARTESIAN_POINT('Ctrl Pts',(-2.79145823440781,1.,2.50410700351493));
#51185=CARTESIAN_POINT('Ctrl Pts',(-2.79164172518905,1.,2.50417932839313));
#51186=CARTESIAN_POINT('Ctrl Pts',(-2.79217568804755,1.,2.50455968395146));
#51187=CARTESIAN_POINT('Ctrl Pts',(-2.79344192164147,1.,2.50567182569081));
#51188=CARTESIAN_POINT('Ctrl Pts',(-2.79596878057287,1.,2.50810555977671));
#51189=CARTESIAN_POINT('Ctrl Pts',(-2.79970585014168,1.,2.51186983687818));
#51190=CARTESIAN_POINT('Ctrl Pts',(-2.80427363984653,1.,2.51660190465805));
#51191=CARTESIAN_POINT('Ctrl Pts',(-2.80941521966941,1.,2.52205778589653));
#51192=CARTESIAN_POINT('Ctrl Pts',(-2.81484379048475,1.,2.52796388055278));
#51193=CARTESIAN_POINT('Ctrl Pts',(-2.82028550483689,1.,2.53405679667412));
#51194=CARTESIAN_POINT('Ctrl Pts',(-2.8255216764922,1.,2.54012272520199));
#51195=CARTESIAN_POINT('Ctrl Pts',(-2.83044254225917,1.,2.54604736792655));
#51196=CARTESIAN_POINT('Ctrl Pts',(-2.83505269592536,1.,2.55182152807077));
#51197=CARTESIAN_POINT('Ctrl Pts',(-2.83942515220782,1.,2.55749952145241));
#51198=CARTESIAN_POINT('Ctrl Pts',(-2.84366802680237,1.,2.56316920798513));
#51199=CARTESIAN_POINT('Ctrl Pts',(-2.84788893329067,1.,2.56891984251721));
#51200=CARTESIAN_POINT('Ctrl Pts',(-2.85215360144431,1.,2.57480482727081));
#51201=CARTESIAN_POINT('Ctrl Pts',(-2.85647171715092,1.,2.58082875254357));
#51202=CARTESIAN_POINT('Ctrl Pts',(-2.86081999003629,1.,2.58696770643524));
#51203=CARTESIAN_POINT('Ctrl Pts',(-2.86515629953513,1.,2.59318160184908));
#51204=CARTESIAN_POINT('Ctrl Pts',(-2.86943633170722,1.,2.5994287522321));
#51205=CARTESIAN_POINT('Ctrl Pts',(-2.87363176656501,1.,2.60568177881303));
#51206=CARTESIAN_POINT('Ctrl Pts',(-2.87773881947916,1.,2.61193507170955));
#51207=CARTESIAN_POINT('Ctrl Pts',(-2.88176821427525,1.,2.61819596473108));
#51208=CARTESIAN_POINT('Ctrl Pts',(-2.88573922195059,1.,2.62447947640262));
#51209=CARTESIAN_POINT('Ctrl Pts',(-2.88967244854239,1.,2.63080195420767));
#51210=CARTESIAN_POINT('Ctrl Pts',(-2.89358228854544,1.,2.63717442263932));
#51211=CARTESIAN_POINT('Ctrl Pts',(-2.89747231723345,1.,2.64359851684131));
#51212=CARTESIAN_POINT('Ctrl Pts',(-2.90133950224867,1.,2.65007017365564));
#51213=CARTESIAN_POINT('Ctrl Pts',(-2.90517678087461,1.,2.65658188464282));
#51214=CARTESIAN_POINT('Ctrl Pts',(-2.90897617968923,1.,2.6631254261681));
#51215=CARTESIAN_POINT('Ctrl Pts',(-2.91273193382882,1.,2.66969458792631));
#51216=CARTESIAN_POINT('Ctrl Pts',(-2.91644290704285,1.,2.67628728855312));
#51217=CARTESIAN_POINT('Ctrl Pts',(-2.92011090722152,1.,2.68290409279688));
#51218=CARTESIAN_POINT('Ctrl Pts',(-2.92373955325875,1.,2.68954721165339));
#51219=CARTESIAN_POINT('Ctrl Pts',(-2.92733294395267,1.,2.69621932864301));
#51220=CARTESIAN_POINT('Ctrl Pts',(-2.9308943823375,1.,2.70292247416885));
#51221=CARTESIAN_POINT('Ctrl Pts',(-2.93442516311179,1.,2.70965695523787));
#51222=CARTESIAN_POINT('Ctrl Pts',(-2.93792519474972,1.,2.71642190053592));
#51223=CARTESIAN_POINT('Ctrl Pts',(-2.94139351933897,1.,2.72321571511337));
#51224=CARTESIAN_POINT('Ctrl Pts',(-2.94482887675143,1.,2.73003657371617));
#51225=CARTESIAN_POINT('Ctrl Pts',(-2.94823023414364,1.,2.73688288329808));
#51226=CARTESIAN_POINT('Ctrl Pts',(-2.95159737214266,1.,2.74375379492172));
#51227=CARTESIAN_POINT('Ctrl Pts',(-2.95493069316161,1.,2.75064903318947));
#51228=CARTESIAN_POINT('Ctrl Pts',(-2.95823097665896,1.,2.7575686788835));
#51229=CARTESIAN_POINT('Ctrl Pts',(-2.96149914764818,1.,2.76451296269557));
#51230=CARTESIAN_POINT('Ctrl Pts',(-2.96473605585583,1.,2.77148206836498));
#51231=CARTESIAN_POINT('Ctrl Pts',(-2.96794221043036,1.,2.7784758954285));
#51232=CARTESIAN_POINT('Ctrl Pts',(-2.97111781461465,1.,2.78549409123769));
#51233=CARTESIAN_POINT('Ctrl Pts',(-2.9742628834758,1.,2.79253615718248));
#51234=CARTESIAN_POINT('Ctrl Pts',(-2.97737733718287,1.,2.7996015327823));
#51235=CARTESIAN_POINT('Ctrl Pts',(-2.98046109647241,1.,2.80668968101106));
#51236=CARTESIAN_POINT('Ctrl Pts',(-2.98351419779767,1.,2.81380019196286));
#51237=CARTESIAN_POINT('Ctrl Pts',(-2.9865368066918,1.,2.82093279065457));
#51238=CARTESIAN_POINT('Ctrl Pts',(-2.98952916401446,1.,2.82808728190157));
#51239=CARTESIAN_POINT('Ctrl Pts',(-2.9924915517034,1.,2.83526351254248));
#51240=CARTESIAN_POINT('Ctrl Pts',(-2.99542425341685,1.,2.84246132984415));
#51241=CARTESIAN_POINT('Ctrl Pts',(-2.99832751144925,1.,2.84968053289451));
#51242=CARTESIAN_POINT('Ctrl Pts',(-3.00120150796095,1.,2.85692085715686));
#51243=CARTESIAN_POINT('Ctrl Pts',(-3.00404638316867,1.,2.86418200833667));
#51244=CARTESIAN_POINT('Ctrl Pts',(-3.00686224485784,1.,2.87146368430502));
#51245=CARTESIAN_POINT('Ctrl Pts',(-3.00964918108476,1.,2.87876560072727));
#51246=CARTESIAN_POINT('Ctrl Pts',(-3.01240727308829,1.,2.8860875170608));
#51247=CARTESIAN_POINT('Ctrl Pts',(-3.01513660431928,1.,2.89342925566321));
#51248=CARTESIAN_POINT('Ctrl Pts',(-3.01783725121981,1.,2.9007906910105));
#51249=CARTESIAN_POINT('Ctrl Pts',(-3.01997487193503,1.,2.90669553302526));
#51250=CARTESIAN_POINT('Ctrl Pts',(-3.02156522742431,1.,2.91113297348212));
#51251=CARTESIAN_POINT('Ctrl Pts',(-3.02261975104593,1.,2.91409518070399));
#51252=CARTESIAN_POINT('Ctrl Pts',(-3.02314558451372,1.,2.91557726271063));
#51253=CARTESIAN_POINT('Origin',(-3.02314558451372,0.,2.91557726271063));
#51254=CARTESIAN_POINT('',(-2.91557726271063,1.,3.02314558451372));
#51255=CARTESIAN_POINT('Origin',(0.,0.,0.));
#51256=CARTESIAN_POINT('',(-2.90994629141562,1.,2.36531447826213));
#51257=CARTESIAN_POINT('Origin',(0.,1.,0.));
#51258=CARTESIAN_POINT('Ctrl Pts',(-2.90994629141562,1.,2.36531447826213));
#51259=CARTESIAN_POINT('Ctrl Pts',(-2.90994629141562,0.666666666666667,
2.36531447826213));
#51260=CARTESIAN_POINT('Ctrl Pts',(-2.90994629141562,0.333333333333333,
2.36531447826213));
#51261=CARTESIAN_POINT('Ctrl Pts',(-2.90994629141562,-0.333333333333333,
2.36531447826213));
#51262=CARTESIAN_POINT('Ctrl Pts',(-2.90994629141562,-0.666666666666667,
2.36531447826213));
#51263=CARTESIAN_POINT('Ctrl Pts',(-2.90994629141562,-1.,2.36531447826213));
#51264=CARTESIAN_POINT('Ctrl Pts',(-3.35260583073571,-1.,2.52982887637028));
#51265=CARTESIAN_POINT('Ctrl Pts',(-3.35260583073571,1.,2.52982887637028));
#51266=CARTESIAN_POINT('Ctrl Pts',(-3.35105973714426,-1.,2.52954136549357));
#51267=CARTESIAN_POINT('Ctrl Pts',(-3.35105973714426,1.,2.52954136549357));
#51268=CARTESIAN_POINT('Ctrl Pts',(-3.34796903577628,-1.,2.5289632161143));
#51269=CARTESIAN_POINT('Ctrl Pts',(-3.34796903577628,1.,2.5289632161143));
#51270=CARTESIAN_POINT('Ctrl Pts',(-3.34333744117093,-1.,2.52808660916879));
#51271=CARTESIAN_POINT('Ctrl Pts',(-3.34333744117093,1.,2.52808660916879));
#51272=CARTESIAN_POINT('Ctrl Pts',(-3.33717090000955,-1.,2.52689902691551));
#51273=CARTESIAN_POINT('Ctrl Pts',(-3.33717090000955,1.,2.52689902691551));
#51274=CARTESIAN_POINT('Ctrl Pts',(-3.32947762189049,-1.,2.52538321165774));
#51275=CARTESIAN_POINT('Ctrl Pts',(-3.32947762189049,1.,2.52538321165774));
#51276=CARTESIAN_POINT('Ctrl Pts',(-3.32179931079521,-1.,2.52383598396878));
#51277=CARTESIAN_POINT('Ctrl Pts',(-3.32179931079521,1.,2.52383598396878));
#51278=CARTESIAN_POINT('Ctrl Pts',(-3.31413607874727,-1.,2.52225724871375));
#51279=CARTESIAN_POINT('Ctrl Pts',(-3.31413607874727,1.,2.52225724871375));
#51280=CARTESIAN_POINT('Ctrl Pts',(-3.30648808814986,-1.,2.52064689568167));
#51281=CARTESIAN_POINT('Ctrl Pts',(-3.30648808814986,1.,2.52064689568167));
#51282=CARTESIAN_POINT('Ctrl Pts',(-3.29885556387661,-1.,2.51900480700548));
#51283=CARTESIAN_POINT('Ctrl Pts',(-3.29885556387661,1.,2.51900480700548));
#51284=CARTESIAN_POINT('Ctrl Pts',(-3.2912387729863,-1.,2.51733085123316));
#51285=CARTESIAN_POINT('Ctrl Pts',(-3.2912387729863,1.,2.51733085123316));
#51286=CARTESIAN_POINT('Ctrl Pts',(-3.28363799702583,-1.,2.51562487464215));
#51287=CARTESIAN_POINT('Ctrl Pts',(-3.28363799702583,1.,2.51562487464215));
#51288=CARTESIAN_POINT('Ctrl Pts',(-3.27605350473048,-1.,2.51388669270329));
#51289=CARTESIAN_POINT('Ctrl Pts',(-3.27605350473048,1.,2.51388669270329));
#51290=CARTESIAN_POINT('Ctrl Pts',(-3.26848552888271,-1.,2.51211608411539));
#51291=CARTESIAN_POINT('Ctrl Pts',(-3.26848552888271,1.,2.51211608411539));
#51292=CARTESIAN_POINT('Ctrl Pts',(-3.26093423001716,-1.,2.51031277813697));
#51293=CARTESIAN_POINT('Ctrl Pts',(-3.26093423001716,1.,2.51031277813697));
#51294=CARTESIAN_POINT('Ctrl Pts',(-3.25339971461265,-1.,2.50847647070936));
#51295=CARTESIAN_POINT('Ctrl Pts',(-3.25339971461265,1.,2.50847647070936));
#51296=CARTESIAN_POINT('Ctrl Pts',(-3.24588208984042,-1.,2.50660685940645));
#51297=CARTESIAN_POINT('Ctrl Pts',(-3.24588208984042,1.,2.50660685940645));
#51298=CARTESIAN_POINT('Ctrl Pts',(-3.23838151080383,-1.,2.50470367580078));
#51299=CARTESIAN_POINT('Ctrl Pts',(-3.23838151080383,1.,2.50470367580078));
#51300=CARTESIAN_POINT('Ctrl Pts',(-3.23089822320596,-1.,2.50276671338074));
#51301=CARTESIAN_POINT('Ctrl Pts',(-3.23089822320596,1.,2.50276671338074));
#51302=CARTESIAN_POINT('Ctrl Pts',(-3.22343262620387,-1.,2.5007958720187));
#51303=CARTESIAN_POINT('Ctrl Pts',(-3.22343262620387,1.,2.5007958720187));
#51304=CARTESIAN_POINT('Ctrl Pts',(-3.21598526261157,-1.,2.49879114599293));
#51305=CARTESIAN_POINT('Ctrl Pts',(-3.21598526261157,1.,2.49879114599293));
#51306=CARTESIAN_POINT('Ctrl Pts',(-3.2085566984974,-1.,2.49675252647298));
#51307=CARTESIAN_POINT('Ctrl Pts',(-3.2085566984974,1.,2.49675252647298));
#51308=CARTESIAN_POINT('Ctrl Pts',(-3.20114742397549,-1.,2.49467992057726));
#51309=CARTESIAN_POINT('Ctrl Pts',(-3.20114742397549,1.,2.49467992057726));
#51310=CARTESIAN_POINT('Ctrl Pts',(-3.19375775555814,-1.,2.4925730723986));
#51311=CARTESIAN_POINT('Ctrl Pts',(-3.19375775555814,1.,2.4925730723986));
#51312=CARTESIAN_POINT('Ctrl Pts',(-3.18638771282315,-1.,2.49043146334095));
#51313=CARTESIAN_POINT('Ctrl Pts',(-3.18638771282315,1.,2.49043146334095));
#51314=CARTESIAN_POINT('Ctrl Pts',(-3.17903698136679,-1.,2.48825428288243));
#51315=CARTESIAN_POINT('Ctrl Pts',(-3.17903698136679,1.,2.48825428288243));
#51316=CARTESIAN_POINT('Ctrl Pts',(-3.17170518863357,-1.,2.48604065348619));
#51317=CARTESIAN_POINT('Ctrl Pts',(-3.17170518863357,1.,2.48604065348619));
#51318=CARTESIAN_POINT('Ctrl Pts',(-3.16439213290181,-1.,2.48378981792739));
#51319=CARTESIAN_POINT('Ctrl Pts',(-3.16439213290181,1.,2.48378981792739));
#51320=CARTESIAN_POINT('Ctrl Pts',(-3.15709802322735,-1.,2.48150133566568));
#51321=CARTESIAN_POINT('Ctrl Pts',(-3.15709802322735,1.,2.48150133566568));
#51322=CARTESIAN_POINT('Ctrl Pts',(-3.14982373241335,-1.,2.47917529057016));
#51323=CARTESIAN_POINT('Ctrl Pts',(-3.14982373241335,1.,2.47917529057016));
#51324=CARTESIAN_POINT('Ctrl Pts',(-3.14257099546531,-1.,2.47681245356095));
#51325=CARTESIAN_POINT('Ctrl Pts',(-3.14257099546531,1.,2.47681245356095));
#51326=CARTESIAN_POINT('Ctrl Pts',(-3.13534181229282,-1.,2.47441378371923));
#51327=CARTESIAN_POINT('Ctrl Pts',(-3.13534181229282,1.,2.47441378371923));
#51328=CARTESIAN_POINT('Ctrl Pts',(-3.12813790805948,-1.,2.47197997765868));
#51329=CARTESIAN_POINT('Ctrl Pts',(-3.12813790805948,1.,2.47197997765868));
#51330=CARTESIAN_POINT('Ctrl Pts',(-3.12096015766984,-1.,2.4695109894747));
#51331=CARTESIAN_POINT('Ctrl Pts',(-3.12096015766984,1.,2.4695109894747));
#51332=CARTESIAN_POINT('Ctrl Pts',(-3.11380805536124,-1.,2.46700558843507));
#51333=CARTESIAN_POINT('Ctrl Pts',(-3.11380805536124,1.,2.46700558843507));
#51334=CARTESIAN_POINT('Ctrl Pts',(-3.10667907901981,-1.,2.46446082979645));
#51335=CARTESIAN_POINT('Ctrl Pts',(-3.10667907901981,1.,2.46446082979645));
#51336=CARTESIAN_POINT('Ctrl Pts',(-3.09956993697048,-1.,2.4618730850188));
#51337=CARTESIAN_POINT('Ctrl Pts',(-3.09956993697048,1.,2.4618730850188));
#51338=CARTESIAN_POINT('Ctrl Pts',(-3.09247787931881,-1.,2.45923912563875));
#51339=CARTESIAN_POINT('Ctrl Pts',(-3.09247787931881,1.,2.45923912563875));
#51340=CARTESIAN_POINT('Ctrl Pts',(-3.08540206545313,-1.,2.45655725437037));
#51341=CARTESIAN_POINT('Ctrl Pts',(-3.08540206545313,1.,2.45655725437037));
#51342=CARTESIAN_POINT('Ctrl Pts',(-3.07834472886145,-1.,2.45382826787795));
#51343=CARTESIAN_POINT('Ctrl Pts',(-3.07834472886145,1.,2.45382826787795));
#51344=CARTESIAN_POINT('Ctrl Pts',(-3.0713129052131,-1.,2.45105688854432));
#51345=CARTESIAN_POINT('Ctrl Pts',(-3.0713129052131,1.,2.45105688854432));
#51346=CARTESIAN_POINT('Ctrl Pts',(-3.06431596421422,-1.,2.44824970516558));
#51347=CARTESIAN_POINT('Ctrl Pts',(-3.06431596421422,1.,2.44824970516558));
#51348=CARTESIAN_POINT('Ctrl Pts',(-3.05736242671521,-1.,2.44541251892568));
#51349=CARTESIAN_POINT('Ctrl Pts',(-3.05736242671521,1.,2.44541251892568));
#51350=CARTESIAN_POINT('Ctrl Pts',(-3.05045678021509,-1.,2.44254768923109));
#51351=CARTESIAN_POINT('Ctrl Pts',(-3.05045678021509,1.,2.44254768923109));
#51352=CARTESIAN_POINT('Ctrl Pts',(-3.04359685040545,-1.,2.43965194061849));
#51353=CARTESIAN_POINT('Ctrl Pts',(-3.04359685040545,1.,2.43965194061849));
#51354=CARTESIAN_POINT('Ctrl Pts',(-3.03676949672797,-1.,2.43671278042394));
#51355=CARTESIAN_POINT('Ctrl Pts',(-3.03676949672797,1.,2.43671278042394));
#51356=CARTESIAN_POINT('Ctrl Pts',(-3.02995534946946,-1.,2.43371241361462));
#51357=CARTESIAN_POINT('Ctrl Pts',(-3.02995534946946,1.,2.43371241361462));
#51358=CARTESIAN_POINT('Ctrl Pts',(-3.02313656035977,-1.,2.43063415586615));
#51359=CARTESIAN_POINT('Ctrl Pts',(-3.02313656035977,1.,2.43063415586615));
#51360=CARTESIAN_POINT('Ctrl Pts',(-3.01630420830494,-1.,2.4274685626416));
#51361=CARTESIAN_POINT('Ctrl Pts',(-3.01630420830494,1.,2.4274685626416));
#51362=CARTESIAN_POINT('Ctrl Pts',(-3.00946442616674,-1.,2.42421849439625));
#51363=CARTESIAN_POINT('Ctrl Pts',(-3.00946442616674,1.,2.42421849439625));
#51364=CARTESIAN_POINT('Ctrl Pts',(-3.00264868586038,-1.,2.42090763946812));
#51365=CARTESIAN_POINT('Ctrl Pts',(-3.00264868586038,1.,2.42090763946812));
#51366=CARTESIAN_POINT('Ctrl Pts',(-2.99590509293561,-1.,2.4175732450056));
#51367=CARTESIAN_POINT('Ctrl Pts',(-2.99590509293561,1.,2.4175732450056));
#51368=CARTESIAN_POINT('Ctrl Pts',(-2.98927983005851,-1.,2.4142506419963));
#51369=CARTESIAN_POINT('Ctrl Pts',(-2.98927983005851,1.,2.4142506419963));
#51370=CARTESIAN_POINT('Ctrl Pts',(-2.98280015815132,-1.,2.41095909342591));
#51371=CARTESIAN_POINT('Ctrl Pts',(-2.98280015815132,1.,2.41095909342591));
#51372=CARTESIAN_POINT('Ctrl Pts',(-2.97646002822395,-1.,2.40768975073691));
#51373=CARTESIAN_POINT('Ctrl Pts',(-2.97646002822395,1.,2.40768975073691));
#51374=CARTESIAN_POINT('Ctrl Pts',(-2.97019641312272,-1.,2.40438604734848));
#51375=CARTESIAN_POINT('Ctrl Pts',(-2.97019641312272,1.,2.40438604734848));
#51376=CARTESIAN_POINT('Ctrl Pts',(-2.96390432240181,-1.,2.40095565711535));
#51377=CARTESIAN_POINT('Ctrl Pts',(-2.96390432240181,1.,2.40095565711535));
#51378=CARTESIAN_POINT('Ctrl Pts',(-2.95748006482811,-1.,2.39730553974412));
#51379=CARTESIAN_POINT('Ctrl Pts',(-2.95748006482811,1.,2.39730553974412));
#51380=CARTESIAN_POINT('Ctrl Pts',(-2.95085857128372,-1.,2.39337207631613));
#51381=CARTESIAN_POINT('Ctrl Pts',(-2.95085857128372,1.,2.39337207631613));
#51382=CARTESIAN_POINT('Ctrl Pts',(-2.94404820669135,-1.,2.38914929090806));
#51383=CARTESIAN_POINT('Ctrl Pts',(-2.94404820669135,1.,2.38914929090806));
#51384=CARTESIAN_POINT('Ctrl Pts',(-2.93717903280599,-1.,2.38472771516476));
#51385=CARTESIAN_POINT('Ctrl Pts',(-2.93717903280599,1.,2.38472771516476));
#51386=CARTESIAN_POINT('Ctrl Pts',(-2.93049643640517,-1.,2.3802898958232));
#51387=CARTESIAN_POINT('Ctrl Pts',(-2.93049643640517,1.,2.3802898958232));
#51388=CARTESIAN_POINT('Ctrl Pts',(-2.92430340582912,-1.,2.37606510524271));
#51389=CARTESIAN_POINT('Ctrl Pts',(-2.92430340582912,1.,2.37606510524271));
#51390=CARTESIAN_POINT('Ctrl Pts',(-2.9189150379156,-1.,2.37229381109939));
#51391=CARTESIAN_POINT('Ctrl Pts',(-2.9189150379156,1.,2.37229381109939));
#51392=CARTESIAN_POINT('Ctrl Pts',(-2.91461249883016,-1.,2.36919161373074));
#51393=CARTESIAN_POINT('Ctrl Pts',(-2.91461249883016,1.,2.36919161373074));
#51394=CARTESIAN_POINT('Ctrl Pts',(-2.9115863784165,-1.,2.36690501170317));
#51395=CARTESIAN_POINT('Ctrl Pts',(-2.9115863784165,1.,2.36690501170317));
#51396=CARTESIAN_POINT('Ctrl Pts',(-2.91025813829606,-1.,2.36578327194396));
#51397=CARTESIAN_POINT('Ctrl Pts',(-2.91025813829606,1.,2.36578327194396));
#51398=CARTESIAN_POINT('Ctrl Pts',(-2.90989022547738,-1.,2.36535052956704));
#51399=CARTESIAN_POINT('Ctrl Pts',(-2.90989022547738,1.,2.36535052956704));
#51400=CARTESIAN_POINT('Ctrl Pts',(-2.90992398626098,-1.,2.36524348105023));
#51401=CARTESIAN_POINT('Ctrl Pts',(-2.90992398626098,1.,2.36524348105023));
#51402=CARTESIAN_POINT('Ctrl Pts',(-2.91001063062876,-1.,2.36523532225181));
#51403=CARTESIAN_POINT('Ctrl Pts',(-2.91001063062876,1.,2.36523532225181));
#51404=CARTESIAN_POINT('',(-3.35260583073571,1.,2.52982887637028));
#51405=CARTESIAN_POINT('Ctrl Pts',(-3.35260583073571,1.,2.52982887637028));
#51406=CARTESIAN_POINT('Ctrl Pts',(-3.35105973714426,1.,2.52954136549357));
#51407=CARTESIAN_POINT('Ctrl Pts',(-3.34796903577628,1.,2.5289632161143));
#51408=CARTESIAN_POINT('Ctrl Pts',(-3.34333744117093,1.,2.52808660916879));
#51409=CARTESIAN_POINT('Ctrl Pts',(-3.33717090000955,1.,2.52689902691551));
#51410=CARTESIAN_POINT('Ctrl Pts',(-3.32947762189049,1.,2.52538321165774));
#51411=CARTESIAN_POINT('Ctrl Pts',(-3.32179931079521,1.,2.52383598396878));
#51412=CARTESIAN_POINT('Ctrl Pts',(-3.31413607874727,1.,2.52225724871375));
#51413=CARTESIAN_POINT('Ctrl Pts',(-3.30648808814986,1.,2.52064689568167));
#51414=CARTESIAN_POINT('Ctrl Pts',(-3.29885556387661,1.,2.51900480700548));
#51415=CARTESIAN_POINT('Ctrl Pts',(-3.2912387729863,1.,2.51733085123316));
#51416=CARTESIAN_POINT('Ctrl Pts',(-3.28363799702583,1.,2.51562487464215));
#51417=CARTESIAN_POINT('Ctrl Pts',(-3.27605350473048,1.,2.51388669270329));
#51418=CARTESIAN_POINT('Ctrl Pts',(-3.26848552888271,1.,2.51211608411539));
#51419=CARTESIAN_POINT('Ctrl Pts',(-3.26093423001716,1.,2.51031277813697));
#51420=CARTESIAN_POINT('Ctrl Pts',(-3.25339971461265,1.,2.50847647070936));
#51421=CARTESIAN_POINT('Ctrl Pts',(-3.24588208984042,1.,2.50660685940645));
#51422=CARTESIAN_POINT('Ctrl Pts',(-3.23838151080383,1.,2.50470367580078));
#51423=CARTESIAN_POINT('Ctrl Pts',(-3.23089822320596,1.,2.50276671338074));
#51424=CARTESIAN_POINT('Ctrl Pts',(-3.22343262620387,1.,2.5007958720187));
#51425=CARTESIAN_POINT('Ctrl Pts',(-3.21598526261157,1.,2.49879114599293));
#51426=CARTESIAN_POINT('Ctrl Pts',(-3.2085566984974,1.,2.49675252647298));
#51427=CARTESIAN_POINT('Ctrl Pts',(-3.20114742397549,1.,2.49467992057726));
#51428=CARTESIAN_POINT('Ctrl Pts',(-3.19375775555814,1.,2.4925730723986));
#51429=CARTESIAN_POINT('Ctrl Pts',(-3.18638771282315,1.,2.49043146334095));
#51430=CARTESIAN_POINT('Ctrl Pts',(-3.17903698136679,1.,2.48825428288243));
#51431=CARTESIAN_POINT('Ctrl Pts',(-3.17170518863357,1.,2.48604065348619));
#51432=CARTESIAN_POINT('Ctrl Pts',(-3.16439213290181,1.,2.48378981792739));
#51433=CARTESIAN_POINT('Ctrl Pts',(-3.15709802322735,1.,2.48150133566568));
#51434=CARTESIAN_POINT('Ctrl Pts',(-3.14982373241335,1.,2.47917529057016));
#51435=CARTESIAN_POINT('Ctrl Pts',(-3.14257099546531,1.,2.47681245356095));
#51436=CARTESIAN_POINT('Ctrl Pts',(-3.13534181229282,1.,2.47441378371923));
#51437=CARTESIAN_POINT('Ctrl Pts',(-3.12813790805948,1.,2.47197997765868));
#51438=CARTESIAN_POINT('Ctrl Pts',(-3.12096015766984,1.,2.4695109894747));
#51439=CARTESIAN_POINT('Ctrl Pts',(-3.11380805536124,1.,2.46700558843507));
#51440=CARTESIAN_POINT('Ctrl Pts',(-3.10667907901981,1.,2.46446082979645));
#51441=CARTESIAN_POINT('Ctrl Pts',(-3.09956993697048,1.,2.4618730850188));
#51442=CARTESIAN_POINT('Ctrl Pts',(-3.09247787931881,1.,2.45923912563875));
#51443=CARTESIAN_POINT('Ctrl Pts',(-3.08540206545313,1.,2.45655725437037));
#51444=CARTESIAN_POINT('Ctrl Pts',(-3.07834472886145,1.,2.45382826787795));
#51445=CARTESIAN_POINT('Ctrl Pts',(-3.0713129052131,1.,2.45105688854432));
#51446=CARTESIAN_POINT('Ctrl Pts',(-3.06431596421422,1.,2.44824970516558));
#51447=CARTESIAN_POINT('Ctrl Pts',(-3.05736242671521,1.,2.44541251892568));
#51448=CARTESIAN_POINT('Ctrl Pts',(-3.05045678021509,1.,2.44254768923109));
#51449=CARTESIAN_POINT('Ctrl Pts',(-3.04359685040545,1.,2.43965194061849));
#51450=CARTESIAN_POINT('Ctrl Pts',(-3.03676949672797,1.,2.43671278042394));
#51451=CARTESIAN_POINT('Ctrl Pts',(-3.02995534946946,1.,2.43371241361462));
#51452=CARTESIAN_POINT('Ctrl Pts',(-3.02313656035977,1.,2.43063415586615));
#51453=CARTESIAN_POINT('Ctrl Pts',(-3.01630420830494,1.,2.4274685626416));
#51454=CARTESIAN_POINT('Ctrl Pts',(-3.00946442616674,1.,2.42421849439625));
#51455=CARTESIAN_POINT('Ctrl Pts',(-3.00264868586038,1.,2.42090763946812));
#51456=CARTESIAN_POINT('Ctrl Pts',(-2.99590509293561,1.,2.4175732450056));
#51457=CARTESIAN_POINT('Ctrl Pts',(-2.98927983005851,1.,2.4142506419963));
#51458=CARTESIAN_POINT('Ctrl Pts',(-2.98280015815132,1.,2.41095909342591));
#51459=CARTESIAN_POINT('Ctrl Pts',(-2.97646002822395,1.,2.40768975073691));
#51460=CARTESIAN_POINT('Ctrl Pts',(-2.97019641312272,1.,2.40438604734848));
#51461=CARTESIAN_POINT('Ctrl Pts',(-2.96390432240181,1.,2.40095565711535));
#51462=CARTESIAN_POINT('Ctrl Pts',(-2.95748006482811,1.,2.39730553974412));
#51463=CARTESIAN_POINT('Ctrl Pts',(-2.95085857128372,1.,2.39337207631613));
#51464=CARTESIAN_POINT('Ctrl Pts',(-2.94404820669135,1.,2.38914929090806));
#51465=CARTESIAN_POINT('Ctrl Pts',(-2.93717903280599,1.,2.38472771516476));
#51466=CARTESIAN_POINT('Ctrl Pts',(-2.93049643640517,1.,2.3802898958232));
#51467=CARTESIAN_POINT('Ctrl Pts',(-2.92430340582912,1.,2.37606510524271));
#51468=CARTESIAN_POINT('Ctrl Pts',(-2.9189150379156,1.,2.37229381109939));
#51469=CARTESIAN_POINT('Ctrl Pts',(-2.91461249883016,1.,2.36919161373074));
#51470=CARTESIAN_POINT('Ctrl Pts',(-2.91181344022628,1.,2.36707658451709));
#51471=CARTESIAN_POINT('Ctrl Pts',(-2.91051690822262,1.,2.36599991765853));
#51472=CARTESIAN_POINT('Ctrl Pts',(-2.9100577052777,1.,2.36553202948741));
#51473=CARTESIAN_POINT('Ctrl Pts',(-2.90995756655559,1.,2.3653621118858));
#51474=CARTESIAN_POINT('Ctrl Pts',(-2.90994629141563,1.,2.36531447826213));
#51475=CARTESIAN_POINT('',(-3.35260583073571,0.,2.52982887637028));
#51476=CARTESIAN_POINT('Ctrl Pts',(-3.1487152044751,-1.,2.03668666247593));
#51477=CARTESIAN_POINT('Ctrl Pts',(-3.1487152044751,1.,2.03668666247593));
#51478=CARTESIAN_POINT('Ctrl Pts',(-3.14869618937258,-1.,2.03660173757879));
#51479=CARTESIAN_POINT('Ctrl Pts',(-3.14869618937258,1.,2.03660173757879));
#51480=CARTESIAN_POINT('Ctrl Pts',(-3.14878756590812,-1.,2.03653654935592));
#51481=CARTESIAN_POINT('Ctrl Pts',(-3.14878756590812,1.,2.03653654935592));
#51482=CARTESIAN_POINT('Ctrl Pts',(-3.14931281968048,-1.,2.03675273049189));
#51483=CARTESIAN_POINT('Ctrl Pts',(-3.14931281968048,1.,2.03675273049189));
#51484=CARTESIAN_POINT('Ctrl Pts',(-3.15079010635742,-1.,2.03766932526445));
#51485=CARTESIAN_POINT('Ctrl Pts',(-3.15079010635742,1.,2.03766932526445));
#51486=CARTESIAN_POINT('Ctrl Pts',(-3.15389991674792,-1.,2.03984073791519));
#51487=CARTESIAN_POINT('Ctrl Pts',(-3.15389991674792,1.,2.03984073791519));
#51488=CARTESIAN_POINT('Ctrl Pts',(-3.15817983946367,-1.,2.04297406404027));
#51489=CARTESIAN_POINT('Ctrl Pts',(-3.15817983946367,1.,2.04297406404027));
#51490=CARTESIAN_POINT('Ctrl Pts',(-3.16343165058912,-1.,2.04693331247446));
#51491=CARTESIAN_POINT('Ctrl Pts',(-3.16343165058912,1.,2.04693331247446));
#51492=CARTESIAN_POINT('Ctrl Pts',(-3.16936341689527,-1.,2.05151770247233));
#51493=CARTESIAN_POINT('Ctrl Pts',(-3.16936341689527,1.,2.05151770247233));
#51494=CARTESIAN_POINT('Ctrl Pts',(-3.17564906975371,-1.,2.05650186773132));
#51495=CARTESIAN_POINT('Ctrl Pts',(-3.17564906975371,1.,2.05650186773132));
#51496=CARTESIAN_POINT('Ctrl Pts',(-3.18197692964614,-1.,2.06166849827101));
#51497=CARTESIAN_POINT('Ctrl Pts',(-3.18197692964614,1.,2.06166849827101));
#51498=CARTESIAN_POINT('Ctrl Pts',(-3.18809755562368,-1.,2.06684062744112));
#51499=CARTESIAN_POINT('Ctrl Pts',(-3.18809755562368,1.,2.06684062744112));
#51500=CARTESIAN_POINT('Ctrl Pts',(-3.19388465568252,-1.,2.07192253497857));
#51501=CARTESIAN_POINT('Ctrl Pts',(-3.19388465568252,1.,2.07192253497857));
#51502=CARTESIAN_POINT('Ctrl Pts',(-3.19934132836019,-1.,2.07690441870722));
#51503=CARTESIAN_POINT('Ctrl Pts',(-3.19934132836019,1.,2.07690441870722));
#51504=CARTESIAN_POINT('Ctrl Pts',(-3.2045481863073,-1.,2.08182850370878));
#51505=CARTESIAN_POINT('Ctrl Pts',(-3.2045481863073,1.,2.08182850370878));
#51506=CARTESIAN_POINT('Ctrl Pts',(-3.20962575845463,-1.,2.08676465517455));
#51507=CARTESIAN_POINT('Ctrl Pts',(-3.20962575845463,1.,2.08676465517455));
#51508=CARTESIAN_POINT('Ctrl Pts',(-3.21469429601654,-1.,2.09178419460443));
#51509=CARTESIAN_POINT('Ctrl Pts',(-3.21469429601654,1.,2.09178419460443));
#51510=CARTESIAN_POINT('Ctrl Pts',(-3.21982707347009,-1.,2.09692958434895));
#51511=CARTESIAN_POINT('Ctrl Pts',(-3.21982707347009,1.,2.09692958434895));
#51512=CARTESIAN_POINT('Ctrl Pts',(-3.22503437553434,-1.,2.10220384298492));
#51513=CARTESIAN_POINT('Ctrl Pts',(-3.22503437553434,1.,2.10220384298492));
#51514=CARTESIAN_POINT('Ctrl Pts',(-3.23028945793289,-1.,2.10758699642451));
#51515=CARTESIAN_POINT('Ctrl Pts',(-3.23028945793289,1.,2.10758699642451));
#51516=CARTESIAN_POINT('Ctrl Pts',(-3.23554444767099,-1.,2.11304604021773));
#51517=CARTESIAN_POINT('Ctrl Pts',(-3.23554444767099,1.,2.11304604021773));
#51518=CARTESIAN_POINT('Ctrl Pts',(-3.24074905517293,-1.,2.11854673326979));
#51519=CARTESIAN_POINT('Ctrl Pts',(-3.24074905517293,1.,2.11854673326979));
#51520=CARTESIAN_POINT('Ctrl Pts',(-3.24587102613376,-1.,2.12406646410962));
#51521=CARTESIAN_POINT('Ctrl Pts',(-3.24587102613376,1.,2.12406646410962));
#51522=CARTESIAN_POINT('Ctrl Pts',(-3.25090574494028,-1.,2.12960028396832));
#51523=CARTESIAN_POINT('Ctrl Pts',(-3.25090574494028,1.,2.12960028396832));
#51524=CARTESIAN_POINT('Ctrl Pts',(-3.25586495065054,-1.,2.13515375878803));
#51525=CARTESIAN_POINT('Ctrl Pts',(-3.25586495065054,1.,2.13515375878803));
#51526=CARTESIAN_POINT('Ctrl Pts',(-3.26077002641879,-1.,2.14073870754264));
#51527=CARTESIAN_POINT('Ctrl Pts',(-3.26077002641879,1.,2.14073870754264));
#51528=CARTESIAN_POINT('Ctrl Pts',(-3.26564388189759,-1.,2.1463680529566));
#51529=CARTESIAN_POINT('Ctrl Pts',(-3.26564388189759,1.,2.1463680529566));
#51530=CARTESIAN_POINT('Ctrl Pts',(-3.27050245897228,-1.,2.15205043199808));
#51531=CARTESIAN_POINT('Ctrl Pts',(-3.27050245897228,1.,2.15205043199808));
#51532=CARTESIAN_POINT('Ctrl Pts',(-3.27534954469187,-1.,2.15778690038347));
#51533=CARTESIAN_POINT('Ctrl Pts',(-3.27534954469187,1.,2.15778690038347));
#51534=CARTESIAN_POINT('Ctrl Pts',(-3.280181508414,-1.,2.16357391934425));
#51535=CARTESIAN_POINT('Ctrl Pts',(-3.280181508414,1.,2.16357391934425));
#51536=CARTESIAN_POINT('Ctrl Pts',(-3.28499019979724,-1.,2.16940517773455));
#51537=CARTESIAN_POINT('Ctrl Pts',(-3.28499019979724,1.,2.16940517773455));
#51538=CARTESIAN_POINT('Ctrl Pts',(-3.28976645712568,-1.,2.17527380048423));
#51539=CARTESIAN_POINT('Ctrl Pts',(-3.28976645712568,1.,2.17527380048423));
#51540=CARTESIAN_POINT('Ctrl Pts',(-3.2945036150049,-1.,2.18117455557065));
#51541=CARTESIAN_POINT('Ctrl Pts',(-3.2945036150049,1.,2.18117455557065));
#51542=CARTESIAN_POINT('Ctrl Pts',(-3.29920022557639,-1.,2.18710556500327));
#51543=CARTESIAN_POINT('Ctrl Pts',(-3.29920022557639,1.,2.18710556500327));
#51544=CARTESIAN_POINT('Ctrl Pts',(-3.30385816281831,-1.,2.19306710376111));
#51545=CARTESIAN_POINT('Ctrl Pts',(-3.30385816281831,1.,2.19306710376111));
#51546=CARTESIAN_POINT('Ctrl Pts',(-3.30848134694595,-1.,2.19906078949923));
#51547=CARTESIAN_POINT('Ctrl Pts',(-3.30848134694595,1.,2.19906078949923));
#51548=CARTESIAN_POINT('Ctrl Pts',(-3.31307424608949,-1.,2.20508863150607));
#51549=CARTESIAN_POINT('Ctrl Pts',(-3.31307424608949,1.,2.20508863150607));
#51550=CARTESIAN_POINT('Ctrl Pts',(-3.31764044024235,-1.,2.21115211847875));
#51551=CARTESIAN_POINT('Ctrl Pts',(-3.31764044024235,1.,2.21115211847875));
#51552=CARTESIAN_POINT('Ctrl Pts',(-3.32218125618968,-1.,2.21725135110898));
#51553=CARTESIAN_POINT('Ctrl Pts',(-3.32218125618968,1.,2.21725135110898));
#51554=CARTESIAN_POINT('Ctrl Pts',(-3.3266964672289,-1.,2.22338548312772));
#51555=CARTESIAN_POINT('Ctrl Pts',(-3.3266964672289,1.,2.22338548312772));
#51556=CARTESIAN_POINT('Ctrl Pts',(-3.33118487773611,-1.,2.22955308907233));
#51557=CARTESIAN_POINT('Ctrl Pts',(-3.33118487773611,1.,2.22955308907233));
#51558=CARTESIAN_POINT('Ctrl Pts',(-3.33564495756482,-1.,2.23575256328812));
#51559=CARTESIAN_POINT('Ctrl Pts',(-3.33564495756482,1.,2.23575256328812));
#51560=CARTESIAN_POINT('Ctrl Pts',(-3.34007543738025,-1.,2.24198249391422));
#51561=CARTESIAN_POINT('Ctrl Pts',(-3.34007543738025,1.,2.24198249391422));
#51562=CARTESIAN_POINT('Ctrl Pts',(-3.34447596770723,-1.,2.24824207678256));
#51563=CARTESIAN_POINT('Ctrl Pts',(-3.34447596770723,1.,2.24824207678256));
#51564=CARTESIAN_POINT('Ctrl Pts',(-3.34884690292285,-1.,2.25453097693483));
#51565=CARTESIAN_POINT('Ctrl Pts',(-3.34884690292285,1.,2.25453097693483));
#51566=CARTESIAN_POINT('Ctrl Pts',(-3.35318902552626,-1.,2.26084915222449));
#51567=CARTESIAN_POINT('Ctrl Pts',(-3.35318902552626,1.,2.26084915222449));
#51568=CARTESIAN_POINT('Ctrl Pts',(-3.35750328523061,-1.,2.2671966857991));
#51569=CARTESIAN_POINT('Ctrl Pts',(-3.35750328523061,1.,2.2671966857991));
#51570=CARTESIAN_POINT('Ctrl Pts',(-3.36179055004409,-1.,2.2735736262093));
#51571=CARTESIAN_POINT('Ctrl Pts',(-3.36179055004409,1.,2.2735736262093));
#51572=CARTESIAN_POINT('Ctrl Pts',(-3.36605130713076,-1.,2.27997979458037));
#51573=CARTESIAN_POINT('Ctrl Pts',(-3.36605130713076,1.,2.27997979458037));
#51574=CARTESIAN_POINT('Ctrl Pts',(-3.37028570206488,-1.,2.28641481081137));
#51575=CARTESIAN_POINT('Ctrl Pts',(-3.37028570206488,1.,2.28641481081137));
#51576=CARTESIAN_POINT('Ctrl Pts',(-3.37449367172826,-1.,2.29287818007393));
#51577=CARTESIAN_POINT('Ctrl Pts',(-3.37449367172826,1.,2.29287818007393));
#51578=CARTESIAN_POINT('Ctrl Pts',(-3.37867504959433,-1.,2.29936936127624));
#51579=CARTESIAN_POINT('Ctrl Pts',(-3.37867504959433,1.,2.29936936127624));
#51580=CARTESIAN_POINT('Ctrl Pts',(-3.3828296733661,-1.,2.30588783640343));
#51581=CARTESIAN_POINT('Ctrl Pts',(-3.3828296733661,1.,2.30588783640343));
#51582=CARTESIAN_POINT('Ctrl Pts',(-3.38695751492462,-1.,2.31243319489367));
#51583=CARTESIAN_POINT('Ctrl Pts',(-3.38695751492462,1.,2.31243319489367));
#51584=CARTESIAN_POINT('Ctrl Pts',(-3.39105869474822,-1.,2.31900513925424));
#51585=CARTESIAN_POINT('Ctrl Pts',(-3.39105869474822,1.,2.31900513925424));
#51586=CARTESIAN_POINT('Ctrl Pts',(-3.39513342019756,-1.,2.3256034390248));
#51587=CARTESIAN_POINT('Ctrl Pts',(-3.39513342019756,1.,2.3256034390248));
#51588=CARTESIAN_POINT('Ctrl Pts',(-3.39918194577956,-1.,2.33222789882489));
#51589=CARTESIAN_POINT('Ctrl Pts',(-3.39918194577956,1.,2.33222789882489));
#51590=CARTESIAN_POINT('Ctrl Pts',(-3.40320452776743,-1.,2.33887832342782));
#51591=CARTESIAN_POINT('Ctrl Pts',(-3.40320452776743,1.,2.33887832342782));
#51592=CARTESIAN_POINT('Ctrl Pts',(-3.40720137404297,-1.,2.34555447649188));
#51593=CARTESIAN_POINT('Ctrl Pts',(-3.40720137404297,1.,2.34555447649188));
#51594=CARTESIAN_POINT('Ctrl Pts',(-3.41117262314119,-1.,2.35225606824109));
#51595=CARTESIAN_POINT('Ctrl Pts',(-3.41117262314119,1.,2.35225606824109));
#51596=CARTESIAN_POINT('Ctrl Pts',(-3.41511836751469,-1.,2.35898278606946));
#51597=CARTESIAN_POINT('Ctrl Pts',(-3.41511836751469,1.,2.35898278606946));
#51598=CARTESIAN_POINT('Ctrl Pts',(-3.41903866635852,-1.,2.36573431470642));
#51599=CARTESIAN_POINT('Ctrl Pts',(-3.41903866635852,1.,2.36573431470642));
#51600=CARTESIAN_POINT('Ctrl Pts',(-3.42293356216511,-1.,2.37251035954292));
#51601=CARTESIAN_POINT('Ctrl Pts',(-3.42293356216511,1.,2.37251035954292));
#51602=CARTESIAN_POINT('Ctrl Pts',(-3.42680309754399,-1.,2.37931067028926));
#51603=CARTESIAN_POINT('Ctrl Pts',(-3.42680309754399,1.,2.37931067028926));
#51604=CARTESIAN_POINT('Ctrl Pts',(-3.4306473271292,-1.,2.38613505843552));
#51605=CARTESIAN_POINT('Ctrl Pts',(-3.4306473271292,1.,2.38613505843552));
#51606=CARTESIAN_POINT('Ctrl Pts',(-3.4344663067854,-1.,2.39298338804493));
#51607=CARTESIAN_POINT('Ctrl Pts',(-3.4344663067854,1.,2.39298338804493));
#51608=CARTESIAN_POINT('Ctrl Pts',(-3.43750133064416,-1.,2.39848113410292));
#51609=CARTESIAN_POINT('Ctrl Pts',(-3.43750133064416,1.,2.39848113410292));
#51610=CARTESIAN_POINT('Ctrl Pts',(-3.43976627484234,-1.,2.40261515589405));
#51611=CARTESIAN_POINT('Ctrl Pts',(-3.43976627484234,1.,2.40261515589405));
#51612=CARTESIAN_POINT('Ctrl Pts',(-3.44127120683039,-1.,2.4053759295909));
#51613=CARTESIAN_POINT('Ctrl Pts',(-3.44127120683039,1.,2.4053759295909));
#51614=CARTESIAN_POINT('Ctrl Pts',(-3.44202241512147,-1.,2.40675750623143));
#51615=CARTESIAN_POINT('Ctrl Pts',(-3.44202241512147,1.,2.40675750623143));
#51616=CARTESIAN_POINT('',(-3.14877060440327,1.,2.03660101169715));
#51617=CARTESIAN_POINT('Ctrl Pts',(-3.14877060440327,-1.,2.03660101169715));
#51618=CARTESIAN_POINT('Ctrl Pts',(-3.14877060440327,-0.666666666666667,
2.03660101169715));
#51619=CARTESIAN_POINT('Ctrl Pts',(-3.14877060440327,-0.333333333333333,
2.03660101169715));
#51620=CARTESIAN_POINT('Ctrl Pts',(-3.14877060440327,0.333333333333333,
2.03660101169715));
#51621=CARTESIAN_POINT('Ctrl Pts',(-3.14877060440327,0.666666666666667,
2.03660101169715));
#51622=CARTESIAN_POINT('Ctrl Pts',(-3.14877060440327,1.,2.03660101169715));
#51623=CARTESIAN_POINT('',(-3.44202241512147,1.,2.40675750623143));
#51624=CARTESIAN_POINT('',(-3.44202241512147,0.,2.40675750623143));
#51625=CARTESIAN_POINT('Ctrl Pts',(-3.14877060440327,1.,2.03660101169715));
#51626=CARTESIAN_POINT('Ctrl Pts',(-3.14881939088124,1.,2.03659701539259));
#51627=CARTESIAN_POINT('Ctrl Pts',(-3.1490119366901,1.,2.03663974554932));
#51628=CARTESIAN_POINT('Ctrl Pts',(-3.14959882629805,1.,2.03693188810544));
#51629=CARTESIAN_POINT('Ctrl Pts',(-3.15102344775328,1.,2.03783225495961));
#51630=CARTESIAN_POINT('Ctrl Pts',(-3.15389991674792,1.,2.03984073791519));
#51631=CARTESIAN_POINT('Ctrl Pts',(-3.15817983946367,1.,2.04297406404027));
#51632=CARTESIAN_POINT('Ctrl Pts',(-3.16343165058912,1.,2.04693331247446));
#51633=CARTESIAN_POINT('Ctrl Pts',(-3.16936341689527,1.,2.05151770247233));
#51634=CARTESIAN_POINT('Ctrl Pts',(-3.17564906975371,1.,2.05650186773132));
#51635=CARTESIAN_POINT('Ctrl Pts',(-3.18197692964614,1.,2.06166849827101));
#51636=CARTESIAN_POINT('Ctrl Pts',(-3.18809755562368,1.,2.06684062744112));
#51637=CARTESIAN_POINT('Ctrl Pts',(-3.19388465568252,1.,2.07192253497857));
#51638=CARTESIAN_POINT('Ctrl Pts',(-3.19934132836019,1.,2.07690441870722));
#51639=CARTESIAN_POINT('Ctrl Pts',(-3.2045481863073,1.,2.08182850370878));
#51640=CARTESIAN_POINT('Ctrl Pts',(-3.20962575845463,1.,2.08676465517455));
#51641=CARTESIAN_POINT('Ctrl Pts',(-3.21469429601654,1.,2.09178419460443));
#51642=CARTESIAN_POINT('Ctrl Pts',(-3.21982707347009,1.,2.09692958434895));
#51643=CARTESIAN_POINT('Ctrl Pts',(-3.22503437553434,1.,2.10220384298492));
#51644=CARTESIAN_POINT('Ctrl Pts',(-3.23028945793289,1.,2.10758699642451));
#51645=CARTESIAN_POINT('Ctrl Pts',(-3.23554444767099,1.,2.11304604021773));
#51646=CARTESIAN_POINT('Ctrl Pts',(-3.24074905517293,1.,2.11854673326979));
#51647=CARTESIAN_POINT('Ctrl Pts',(-3.24587102613376,1.,2.12406646410962));
#51648=CARTESIAN_POINT('Ctrl Pts',(-3.25090574494028,1.,2.12960028396832));
#51649=CARTESIAN_POINT('Ctrl Pts',(-3.25586495065054,1.,2.13515375878803));
#51650=CARTESIAN_POINT('Ctrl Pts',(-3.26077002641879,1.,2.14073870754264));
#51651=CARTESIAN_POINT('Ctrl Pts',(-3.26564388189759,1.,2.1463680529566));
#51652=CARTESIAN_POINT('Ctrl Pts',(-3.27050245897228,1.,2.15205043199808));
#51653=CARTESIAN_POINT('Ctrl Pts',(-3.27534954469187,1.,2.15778690038347));
#51654=CARTESIAN_POINT('Ctrl Pts',(-3.280181508414,1.,2.16357391934425));
#51655=CARTESIAN_POINT('Ctrl Pts',(-3.28499019979724,1.,2.16940517773455));
#51656=CARTESIAN_POINT('Ctrl Pts',(-3.28976645712568,1.,2.17527380048423));
#51657=CARTESIAN_POINT('Ctrl Pts',(-3.2945036150049,1.,2.18117455557065));
#51658=CARTESIAN_POINT('Ctrl Pts',(-3.29920022557639,1.,2.18710556500327));
#51659=CARTESIAN_POINT('Ctrl Pts',(-3.30385816281831,1.,2.19306710376111));
#51660=CARTESIAN_POINT('Ctrl Pts',(-3.30848134694595,1.,2.19906078949923));
#51661=CARTESIAN_POINT('Ctrl Pts',(-3.31307424608949,1.,2.20508863150607));
#51662=CARTESIAN_POINT('Ctrl Pts',(-3.31764044024235,1.,2.21115211847875));
#51663=CARTESIAN_POINT('Ctrl Pts',(-3.32218125618968,1.,2.21725135110898));
#51664=CARTESIAN_POINT('Ctrl Pts',(-3.3266964672289,1.,2.22338548312772));
#51665=CARTESIAN_POINT('Ctrl Pts',(-3.33118487773611,1.,2.22955308907233));
#51666=CARTESIAN_POINT('Ctrl Pts',(-3.33564495756482,1.,2.23575256328812));
#51667=CARTESIAN_POINT('Ctrl Pts',(-3.34007543738025,1.,2.24198249391422));
#51668=CARTESIAN_POINT('Ctrl Pts',(-3.34447596770723,1.,2.24824207678256));
#51669=CARTESIAN_POINT('Ctrl Pts',(-3.34884690292285,1.,2.25453097693483));
#51670=CARTESIAN_POINT('Ctrl Pts',(-3.35318902552626,1.,2.26084915222449));
#51671=CARTESIAN_POINT('Ctrl Pts',(-3.35750328523061,1.,2.2671966857991));
#51672=CARTESIAN_POINT('Ctrl Pts',(-3.36179055004409,1.,2.2735736262093));
#51673=CARTESIAN_POINT('Ctrl Pts',(-3.36605130713076,1.,2.27997979458037));
#51674=CARTESIAN_POINT('Ctrl Pts',(-3.37028570206488,1.,2.28641481081137));
#51675=CARTESIAN_POINT('Ctrl Pts',(-3.37449367172826,1.,2.29287818007393));
#51676=CARTESIAN_POINT('Ctrl Pts',(-3.37867504959433,1.,2.29936936127624));
#51677=CARTESIAN_POINT('Ctrl Pts',(-3.3828296733661,1.,2.30588783640343));
#51678=CARTESIAN_POINT('Ctrl Pts',(-3.38695751492462,1.,2.31243319489367));
#51679=CARTESIAN_POINT('Ctrl Pts',(-3.39105869474822,1.,2.31900513925424));
#51680=CARTESIAN_POINT('Ctrl Pts',(-3.39513342019756,1.,2.3256034390248));
#51681=CARTESIAN_POINT('Ctrl Pts',(-3.39918194577956,1.,2.33222789882489));
#51682=CARTESIAN_POINT('Ctrl Pts',(-3.40320452776743,1.,2.33887832342782));
#51683=CARTESIAN_POINT('Ctrl Pts',(-3.40720137404297,1.,2.34555447649188));
#51684=CARTESIAN_POINT('Ctrl Pts',(-3.41117262314119,1.,2.35225606824109));
#51685=CARTESIAN_POINT('Ctrl Pts',(-3.41511836751469,1.,2.35898278606946));
#51686=CARTESIAN_POINT('Ctrl Pts',(-3.41903866635852,1.,2.36573431470642));
#51687=CARTESIAN_POINT('Ctrl Pts',(-3.42293356216511,1.,2.37251035954292));
#51688=CARTESIAN_POINT('Ctrl Pts',(-3.42680309754399,1.,2.37931067028926));
#51689=CARTESIAN_POINT('Ctrl Pts',(-3.4306473271292,1.,2.38613505843552));
#51690=CARTESIAN_POINT('Ctrl Pts',(-3.4344663067854,1.,2.39298338804493));
#51691=CARTESIAN_POINT('Ctrl Pts',(-3.43750133064416,1.,2.39848113410292));
#51692=CARTESIAN_POINT('Ctrl Pts',(-3.43976627484234,1.,2.40261515589405));
#51693=CARTESIAN_POINT('Ctrl Pts',(-3.44127120683039,1.,2.4053759295909));
#51694=CARTESIAN_POINT('Ctrl Pts',(-3.44202241512147,1.,2.40675750623143));
#51695=CARTESIAN_POINT('Origin',(-3.44202241512147,0.,2.40675750623143));
#51696=CARTESIAN_POINT('',(-3.35260583073571,1.,2.52982887637028));
#51697=CARTESIAN_POINT('Origin',(0.,0.,0.));
#51698=CARTESIAN_POINT('',(-3.24413672884812,1.,1.88097764062697));
#51699=CARTESIAN_POINT('Origin',(0.,1.,0.));
#51700=CARTESIAN_POINT('Ctrl Pts',(-3.24413672884812,1.,1.88097764062697));
#51701=CARTESIAN_POINT('Ctrl Pts',(-3.24413672884812,0.666666666666667,
1.88097764062697));
#51702=CARTESIAN_POINT('Ctrl Pts',(-3.24413672884812,0.333333333333333,
1.88097764062697));
#51703=CARTESIAN_POINT('Ctrl Pts',(-3.24413672884812,-0.333333333333333,
1.88097764062697));
#51704=CARTESIAN_POINT('Ctrl Pts',(-3.24413672884812,-0.666666666666667,
1.88097764062697));
#51705=CARTESIAN_POINT('Ctrl Pts',(-3.24413672884812,-1.,1.88097764062697));
#51706=CARTESIAN_POINT('Ctrl Pts',(-3.70708211654725,-1.,1.97421938526992));
#51707=CARTESIAN_POINT('Ctrl Pts',(-3.70708211654725,1.,1.97421938526992));
#51708=CARTESIAN_POINT('Ctrl Pts',(-3.70551008132332,-1.,1.97417727645308));
#51709=CARTESIAN_POINT('Ctrl Pts',(-3.70551008132332,1.,1.97417727645308));
#51710=CARTESIAN_POINT('Ctrl Pts',(-3.70236698912904,-1.,1.97408973726715));
#51711=CARTESIAN_POINT('Ctrl Pts',(-3.70236698912904,1.,1.97408973726715));
#51712=CARTESIAN_POINT('Ctrl Pts',(-3.6976552856004,-1.,1.97394846383216));
#51713=CARTESIAN_POINT('Ctrl Pts',(-3.6976552856004,1.,1.97394846383216));
#51714=CARTESIAN_POINT('Ctrl Pts',(-3.69137888599902,-1.,1.97374016225483));
#51715=CARTESIAN_POINT('Ctrl Pts',(-3.69137888599902,1.,1.97374016225483));
#51716=CARTESIAN_POINT('Ctrl Pts',(-3.68354319915092,-1.,1.97344650304519));
#51717=CARTESIAN_POINT('Ctrl Pts',(-3.68354319915092,1.,1.97344650304519));
#51718=CARTESIAN_POINT('Ctrl Pts',(-3.67571738107084,-1.,1.97311947678516));
#51719=CARTESIAN_POINT('Ctrl Pts',(-3.67571738107084,1.,1.97311947678516));
#51720=CARTESIAN_POINT('Ctrl Pts',(-3.66790152752075,-1.,1.97275897198678));
#51721=CARTESIAN_POINT('Ctrl Pts',(-3.66790152752075,1.,1.97275897198678));
#51722=CARTESIAN_POINT('Ctrl Pts',(-3.6600957816636,-1.,1.9723648543905));
#51723=CARTESIAN_POINT('Ctrl Pts',(-3.6600957816636,1.,1.9723648543905));
#51724=CARTESIAN_POINT('Ctrl Pts',(-3.652300347166,-1.,1.9719369724024));
#51725=CARTESIAN_POINT('Ctrl Pts',(-3.652300347166,1.,1.9719369724024));
#51726=CARTESIAN_POINT('Ctrl Pts',(-3.64451546723514,-1.,1.97147515441164));
#51727=CARTESIAN_POINT('Ctrl Pts',(-3.64451546723514,1.,1.97147515441164));
#51728=CARTESIAN_POINT('Ctrl Pts',(-3.63674139590412,-1.,1.97097920454464));
#51729=CARTESIAN_POINT('Ctrl Pts',(-3.63674139590412,1.,1.97097920454464));
#51730=CARTESIAN_POINT('Ctrl Pts',(-3.62897836973293,-1.,1.97044889850463));
#51731=CARTESIAN_POINT('Ctrl Pts',(-3.62897836973293,1.,1.97044889850463));
#51732=CARTESIAN_POINT('Ctrl Pts',(-3.62122658401893,-1.,1.96988398129978));
#51733=CARTESIAN_POINT('Ctrl Pts',(-3.62122658401893,1.,1.96988398129978));
#51734=CARTESIAN_POINT('Ctrl Pts',(-3.61348615496704,-1.,1.96928416040877));
#51735=CARTESIAN_POINT('Ctrl Pts',(-3.61348615496704,1.,1.96928416040877));
#51736=CARTESIAN_POINT('Ctrl Pts',(-3.60575714017989,-1.,1.9686491188594));
#51737=CARTESIAN_POINT('Ctrl Pts',(-3.60575714017989,1.,1.9686491188594));
#51738=CARTESIAN_POINT('Ctrl Pts',(-3.59803959819938,-1.,1.96797854118369));
#51739=CARTESIAN_POINT('Ctrl Pts',(-3.59803959819938,1.,1.96797854118369));
#51740=CARTESIAN_POINT('Ctrl Pts',(-3.59033364022801,-1.,1.96727213799544));
#51741=CARTESIAN_POINT('Ctrl Pts',(-3.59033364022801,1.,1.96727213799544));
#51742=CARTESIAN_POINT('Ctrl Pts',(-3.58263947663829,-1.,1.96652966688911));
#51743=CARTESIAN_POINT('Ctrl Pts',(-3.58263947663829,1.,1.96652966688911));
#51744=CARTESIAN_POINT('Ctrl Pts',(-3.57495748600959,-1.,1.96575096652789));
#51745=CARTESIAN_POINT('Ctrl Pts',(-3.57495748600959,1.,1.96575096652789));
#51746=CARTESIAN_POINT('Ctrl Pts',(-3.56728820357791,-1.,1.96493594634567));
#51747=CARTESIAN_POINT('Ctrl Pts',(-3.56728820357791,1.,1.96493594634567));
#51748=CARTESIAN_POINT('Ctrl Pts',(-3.55963218706096,-1.,1.96408450906812));
#51749=CARTESIAN_POINT('Ctrl Pts',(-3.55963218706096,1.,1.96408450906812));
#51750=CARTESIAN_POINT('Ctrl Pts',(-3.55198990600886,-1.,1.96319648628644));
#51751=CARTESIAN_POINT('Ctrl Pts',(-3.55198990600886,1.,1.96319648628644));
#51752=CARTESIAN_POINT('Ctrl Pts',(-3.54436163300443,-1.,1.96227157573067));
#51753=CARTESIAN_POINT('Ctrl Pts',(-3.54436163300443,1.,1.96227157573067));
#51754=CARTESIAN_POINT('Ctrl Pts',(-3.53674730625813,-1.,1.96130926212689));
#51755=CARTESIAN_POINT('Ctrl Pts',(-3.53674730625813,1.,1.96130926212689));
#51756=CARTESIAN_POINT('Ctrl Pts',(-3.52914648844351,-1.,1.96030879411566));
#51757=CARTESIAN_POINT('Ctrl Pts',(-3.52914648844351,1.,1.96030879411566));
#51758=CARTESIAN_POINT('Ctrl Pts',(-3.52155867431486,-1.,1.95926936324461));
#51759=CARTESIAN_POINT('Ctrl Pts',(-3.52155867431486,1.,1.95926936324461));
#51760=CARTESIAN_POINT('Ctrl Pts',(-3.51398354617794,-1.,1.95819025316779));
#51761=CARTESIAN_POINT('Ctrl Pts',(-3.51398354617794,1.,1.95819025316779));
#51762=CARTESIAN_POINT('Ctrl Pts',(-3.50642124159909,-1.,1.95707099606511));
#51763=CARTESIAN_POINT('Ctrl Pts',(-3.50642124159909,1.,1.95707099606511));
#51764=CARTESIAN_POINT('Ctrl Pts',(-3.49887263575583,-1.,1.95591153823661));
#51765=CARTESIAN_POINT('Ctrl Pts',(-3.49887263575583,1.,1.95591153823661));
#51766=CARTESIAN_POINT('Ctrl Pts',(-3.49133956289133,-1.,1.95471236969643));
#51767=CARTESIAN_POINT('Ctrl Pts',(-3.49133956289133,1.,1.95471236969643));
#51768=CARTESIAN_POINT('Ctrl Pts',(-3.48382414832634,-1.,1.95347412486308));
#51769=CARTESIAN_POINT('Ctrl Pts',(-3.48382414832634,1.,1.95347412486308));
#51770=CARTESIAN_POINT('Ctrl Pts',(-3.47632820495921,-1.,1.95219722189876));
#51771=CARTESIAN_POINT('Ctrl Pts',(-3.47632820495921,1.,1.95219722189876));
#51772=CARTESIAN_POINT('Ctrl Pts',(-3.46885258974191,-1.,1.95088147859876));
#51773=CARTESIAN_POINT('Ctrl Pts',(-3.46885258974191,1.,1.95088147859876));
#51774=CARTESIAN_POINT('Ctrl Pts',(-3.46139661060962,-1.,1.94952575850197));
#51775=CARTESIAN_POINT('Ctrl Pts',(-3.46139661060962,1.,1.94952575850197));
#51776=CARTESIAN_POINT('Ctrl Pts',(-3.45395731584051,-1.,1.94812754766524));
#51777=CARTESIAN_POINT('Ctrl Pts',(-3.45395731584051,1.,1.94812754766524));
#51778=CARTESIAN_POINT('Ctrl Pts',(-3.44653088665681,-1.,1.94668377715329));
#51779=CARTESIAN_POINT('Ctrl Pts',(-3.44653088665681,1.,1.94668377715329));
#51780=CARTESIAN_POINT('Ctrl Pts',(-3.43911410197687,-1.,1.94519168842879));
#51781=CARTESIAN_POINT('Ctrl Pts',(-3.43911410197687,1.,1.94519168842879));
#51782=CARTESIAN_POINT('Ctrl Pts',(-3.43170586602434,-1.,1.94364973660284));
#51783=CARTESIAN_POINT('Ctrl Pts',(-3.43170586602434,1.,1.94364973660284));
#51784=CARTESIAN_POINT('Ctrl Pts',(-3.42430850941503,-1.,1.94205835913696));
#51785=CARTESIAN_POINT('Ctrl Pts',(-3.42430850941503,1.,1.94205835913696));
#51786=CARTESIAN_POINT('Ctrl Pts',(-3.41692971994096,-1.,1.94042111965246));
#51787=CARTESIAN_POINT('Ctrl Pts',(-3.41692971994096,1.,1.94042111965246));
#51788=CARTESIAN_POINT('Ctrl Pts',(-3.40957978266642,-1.,1.93874306008143));
#51789=CARTESIAN_POINT('Ctrl Pts',(-3.40957978266642,1.,1.93874306008143));
#51790=CARTESIAN_POINT('Ctrl Pts',(-3.40226802104109,-1.,1.93702857723098));
#51791=CARTESIAN_POINT('Ctrl Pts',(-3.40226802104109,1.,1.93702857723098));
#51792=CARTESIAN_POINT('Ctrl Pts',(-3.39499923640795,-1.,1.93527929945985));
#51793=CARTESIAN_POINT('Ctrl Pts',(-3.39499923640795,1.,1.93527929945985));
#51794=CARTESIAN_POINT('Ctrl Pts',(-3.38777076883256,-1.,1.93349233176788));
#51795=CARTESIAN_POINT('Ctrl Pts',(-3.38777076883256,1.,1.93349233176788));
#51796=CARTESIAN_POINT('Ctrl Pts',(-3.3805676852555,-1.,1.93165739093276));
#51797=CARTESIAN_POINT('Ctrl Pts',(-3.3805676852555,1.,1.93165739093276));
#51798=CARTESIAN_POINT('Ctrl Pts',(-3.37336807068043,-1.,1.92975993109877));
#51799=CARTESIAN_POINT('Ctrl Pts',(-3.37336807068043,1.,1.92975993109877));
#51800=CARTESIAN_POINT('Ctrl Pts',(-3.36615168657567,-1.,1.92778626543786));
#51801=CARTESIAN_POINT('Ctrl Pts',(-3.36615168657567,1.,1.92778626543786));
#51802=CARTESIAN_POINT('Ctrl Pts',(-3.35890824422965,-1.,1.92572846125756));
#51803=CARTESIAN_POINT('Ctrl Pts',(-3.35890824422965,1.,1.92572846125756));
#51804=CARTESIAN_POINT('Ctrl Pts',(-3.35164424847223,-1.,1.92358838440528));
#51805=CARTESIAN_POINT('Ctrl Pts',(-3.35164424847223,1.,1.92358838440528));
#51806=CARTESIAN_POINT('Ctrl Pts',(-3.34439448941961,-1.,1.92138450828404));
#51807=CARTESIAN_POINT('Ctrl Pts',(-3.34439448941961,1.,1.92138450828404));
#51808=CARTESIAN_POINT('Ctrl Pts',(-3.33721230710012,-1.,1.9191460961021));
#51809=CARTESIAN_POINT('Ctrl Pts',(-3.33721230710012,1.,1.9191460961021));
#51810=CARTESIAN_POINT('Ctrl Pts',(-3.33014884257873,-1.,1.91690081930331));
#51811=CARTESIAN_POINT('Ctrl Pts',(-3.33014884257873,1.,1.91690081930331));
#51812=CARTESIAN_POINT('Ctrl Pts',(-3.32323403454535,-1.,1.91466343916628));
#51813=CARTESIAN_POINT('Ctrl Pts',(-3.32323403454535,1.,1.91466343916628));
#51814=CARTESIAN_POINT('Ctrl Pts',(-3.31646052426364,-1.,1.91242616234442));
#51815=CARTESIAN_POINT('Ctrl Pts',(-3.31646052426364,1.,1.91242616234442));
#51816=CARTESIAN_POINT('Ctrl Pts',(-3.30975721158596,-1.,1.91014297830446));
#51817=CARTESIAN_POINT('Ctrl Pts',(-3.30975721158596,1.,1.91014297830446));
#51818=CARTESIAN_POINT('Ctrl Pts',(-3.30300595568195,-1.,1.90773912171341));
#51819=CARTESIAN_POINT('Ctrl Pts',(-3.30300595568195,1.,1.90773912171341));
#51820=CARTESIAN_POINT('Ctrl Pts',(-3.29608978722113,-1.,1.90513891864087));
#51821=CARTESIAN_POINT('Ctrl Pts',(-3.29608978722113,1.,1.90513891864087));
#51822=CARTESIAN_POINT('Ctrl Pts',(-3.2889344860029,-1.,1.90228971247527));
#51823=CARTESIAN_POINT('Ctrl Pts',(-3.2889344860029,1.,1.90228971247527));
#51824=CARTESIAN_POINT('Ctrl Pts',(-3.28154737912352,-1.,1.89918429230462));
#51825=CARTESIAN_POINT('Ctrl Pts',(-3.28154737912352,1.,1.89918429230462));
#51826=CARTESIAN_POINT('Ctrl Pts',(-3.27407108933139,-1.,1.89589172903793));
#51827=CARTESIAN_POINT('Ctrl Pts',(-3.27407108933139,1.,1.89589172903793));
#51828=CARTESIAN_POINT('Ctrl Pts',(-3.26677653888676,-1.,1.89255393500965));
#51829=CARTESIAN_POINT('Ctrl Pts',(-3.26677653888676,1.,1.89255393500965));
#51830=CARTESIAN_POINT('Ctrl Pts',(-3.25999885193947,-1.,1.88934996203698));
#51831=CARTESIAN_POINT('Ctrl Pts',(-3.25999885193947,1.,1.88934996203698));
#51832=CARTESIAN_POINT('Ctrl Pts',(-3.25408686339463,-1.,1.88646802523466));
#51833=CARTESIAN_POINT('Ctrl Pts',(-3.25408686339463,1.,1.88646802523466));
#51834=CARTESIAN_POINT('Ctrl Pts',(-3.24935200511918,-1.,1.88407708646357));
#51835=CARTESIAN_POINT('Ctrl Pts',(-3.24935200511918,1.,1.88407708646357));
#51836=CARTESIAN_POINT('Ctrl Pts',(-3.24600543790443,-1.,1.88229202582941));
#51837=CARTESIAN_POINT('Ctrl Pts',(-3.24600543790443,1.,1.88229202582941));
#51838=CARTESIAN_POINT('Ctrl Pts',(-3.24451807186481,-1.,1.88139187908074));
#51839=CARTESIAN_POINT('Ctrl Pts',(-3.24451807186481,1.,1.88139187908074));
#51840=CARTESIAN_POINT('Ctrl Pts',(-3.24408699284121,-1.,1.88102201872555));
#51841=CARTESIAN_POINT('Ctrl Pts',(-3.24408699284121,1.,1.88102201872555));
#51842=CARTESIAN_POINT('Ctrl Pts',(-3.24410359189609,-1.,1.88091100680349));
#51843=CARTESIAN_POINT('Ctrl Pts',(-3.24410359189609,1.,1.88091100680349));
#51844=CARTESIAN_POINT('Ctrl Pts',(-3.24418789321065,-1.,1.8808893942881));
#51845=CARTESIAN_POINT('Ctrl Pts',(-3.24418789321065,1.,1.8808893942881));
#51846=CARTESIAN_POINT('',(-3.70708211654725,1.,1.97421938526992));
#51847=CARTESIAN_POINT('Ctrl Pts',(-3.70708211654725,1.,1.97421938526992));
#51848=CARTESIAN_POINT('Ctrl Pts',(-3.70551008132332,1.,1.97417727645308));
#51849=CARTESIAN_POINT('Ctrl Pts',(-3.70236698912904,1.,1.97408973726715));
#51850=CARTESIAN_POINT('Ctrl Pts',(-3.6976552856004,1.,1.97394846383216));
#51851=CARTESIAN_POINT('Ctrl Pts',(-3.69137888599902,1.,1.97374016225483));
#51852=CARTESIAN_POINT('Ctrl Pts',(-3.68354319915092,1.,1.97344650304519));
#51853=CARTESIAN_POINT('Ctrl Pts',(-3.67571738107084,1.,1.97311947678516));
#51854=CARTESIAN_POINT('Ctrl Pts',(-3.66790152752075,1.,1.97275897198678));
#51855=CARTESIAN_POINT('Ctrl Pts',(-3.6600957816636,1.,1.9723648543905));
#51856=CARTESIAN_POINT('Ctrl Pts',(-3.652300347166,1.,1.9719369724024));
#51857=CARTESIAN_POINT('Ctrl Pts',(-3.64451546723514,1.,1.97147515441164));
#51858=CARTESIAN_POINT('Ctrl Pts',(-3.63674139590412,1.,1.97097920454464));
#51859=CARTESIAN_POINT('Ctrl Pts',(-3.62897836973293,1.,1.97044889850463));
#51860=CARTESIAN_POINT('Ctrl Pts',(-3.62122658401893,1.,1.96988398129978));
#51861=CARTESIAN_POINT('Ctrl Pts',(-3.61348615496704,1.,1.96928416040877));
#51862=CARTESIAN_POINT('Ctrl Pts',(-3.60575714017989,1.,1.9686491188594));
#51863=CARTESIAN_POINT('Ctrl Pts',(-3.59803959819938,1.,1.96797854118369));
#51864=CARTESIAN_POINT('Ctrl Pts',(-3.59033364022801,1.,1.96727213799544));
#51865=CARTESIAN_POINT('Ctrl Pts',(-3.58263947663829,1.,1.96652966688911));
#51866=CARTESIAN_POINT('Ctrl Pts',(-3.57495748600959,1.,1.96575096652789));
#51867=CARTESIAN_POINT('Ctrl Pts',(-3.56728820357791,1.,1.96493594634567));
#51868=CARTESIAN_POINT('Ctrl Pts',(-3.55963218706096,1.,1.96408450906812));
#51869=CARTESIAN_POINT('Ctrl Pts',(-3.55198990600886,1.,1.96319648628644));
#51870=CARTESIAN_POINT('Ctrl Pts',(-3.54436163300443,1.,1.96227157573067));
#51871=CARTESIAN_POINT('Ctrl Pts',(-3.53674730625813,1.,1.96130926212689));
#51872=CARTESIAN_POINT('Ctrl Pts',(-3.52914648844351,1.,1.96030879411566));
#51873=CARTESIAN_POINT('Ctrl Pts',(-3.52155867431486,1.,1.95926936324461));
#51874=CARTESIAN_POINT('Ctrl Pts',(-3.51398354617794,1.,1.95819025316779));
#51875=CARTESIAN_POINT('Ctrl Pts',(-3.50642124159909,1.,1.95707099606511));
#51876=CARTESIAN_POINT('Ctrl Pts',(-3.49887263575583,1.,1.95591153823661));
#51877=CARTESIAN_POINT('Ctrl Pts',(-3.49133956289133,1.,1.95471236969643));
#51878=CARTESIAN_POINT('Ctrl Pts',(-3.48382414832634,1.,1.95347412486308));
#51879=CARTESIAN_POINT('Ctrl Pts',(-3.47632820495921,1.,1.95219722189876));
#51880=CARTESIAN_POINT('Ctrl Pts',(-3.46885258974191,1.,1.95088147859876));
#51881=CARTESIAN_POINT('Ctrl Pts',(-3.46139661060962,1.,1.94952575850197));
#51882=CARTESIAN_POINT('Ctrl Pts',(-3.45395731584051,1.,1.94812754766524));
#51883=CARTESIAN_POINT('Ctrl Pts',(-3.44653088665681,1.,1.94668377715329));
#51884=CARTESIAN_POINT('Ctrl Pts',(-3.43911410197687,1.,1.94519168842879));
#51885=CARTESIAN_POINT('Ctrl Pts',(-3.43170586602434,1.,1.94364973660284));
#51886=CARTESIAN_POINT('Ctrl Pts',(-3.42430850941503,1.,1.94205835913696));
#51887=CARTESIAN_POINT('Ctrl Pts',(-3.41692971994096,1.,1.94042111965246));
#51888=CARTESIAN_POINT('Ctrl Pts',(-3.40957978266642,1.,1.93874306008143));
#51889=CARTESIAN_POINT('Ctrl Pts',(-3.40226802104109,1.,1.93702857723098));
#51890=CARTESIAN_POINT('Ctrl Pts',(-3.39499923640795,1.,1.93527929945985));
#51891=CARTESIAN_POINT('Ctrl Pts',(-3.38777076883256,1.,1.93349233176788));
#51892=CARTESIAN_POINT('Ctrl Pts',(-3.3805676852555,1.,1.93165739093276));
#51893=CARTESIAN_POINT('Ctrl Pts',(-3.37336807068043,1.,1.92975993109877));
#51894=CARTESIAN_POINT('Ctrl Pts',(-3.36615168657567,1.,1.92778626543786));
#51895=CARTESIAN_POINT('Ctrl Pts',(-3.35890824422965,1.,1.92572846125756));
#51896=CARTESIAN_POINT('Ctrl Pts',(-3.35164424847223,1.,1.92358838440528));
#51897=CARTESIAN_POINT('Ctrl Pts',(-3.34439448941961,1.,1.92138450828404));
#51898=CARTESIAN_POINT('Ctrl Pts',(-3.33721230710012,1.,1.9191460961021));
#51899=CARTESIAN_POINT('Ctrl Pts',(-3.33014884257873,1.,1.91690081930331));
#51900=CARTESIAN_POINT('Ctrl Pts',(-3.32323403454535,1.,1.91466343916628));
#51901=CARTESIAN_POINT('Ctrl Pts',(-3.31646052426364,1.,1.91242616234442));
#51902=CARTESIAN_POINT('Ctrl Pts',(-3.30975721158596,1.,1.91014297830446));
#51903=CARTESIAN_POINT('Ctrl Pts',(-3.30300595568195,1.,1.90773912171341));
#51904=CARTESIAN_POINT('Ctrl Pts',(-3.29608978722113,1.,1.90513891864087));
#51905=CARTESIAN_POINT('Ctrl Pts',(-3.2889344860029,1.,1.90228971247527));
#51906=CARTESIAN_POINT('Ctrl Pts',(-3.28154737912352,1.,1.89918429230462));
#51907=CARTESIAN_POINT('Ctrl Pts',(-3.27407108933139,1.,1.89589172903793));
#51908=CARTESIAN_POINT('Ctrl Pts',(-3.26677653888676,1.,1.89255393500965));
#51909=CARTESIAN_POINT('Ctrl Pts',(-3.25999885193947,1.,1.88934996203698));
#51910=CARTESIAN_POINT('Ctrl Pts',(-3.25408686339463,1.,1.88646802523466));
#51911=CARTESIAN_POINT('Ctrl Pts',(-3.24935200511918,1.,1.88407708646357));
#51912=CARTESIAN_POINT('Ctrl Pts',(-3.2462565441079,1.,1.88242596600454));
#51913=CARTESIAN_POINT('Ctrl Pts',(-3.24480754676064,1.,1.88156537699203));
#51914=CARTESIAN_POINT('Ctrl Pts',(-3.24428080353022,1.,1.88117508446775));
#51915=CARTESIAN_POINT('Ctrl Pts',(-3.24415531671284,1.,1.8810229239812));
#51916=CARTESIAN_POINT('Ctrl Pts',(-3.24413672884812,1.,1.88097764062697));
#51917=CARTESIAN_POINT('',(-3.70708211654725,0.,1.97421938526992));
#51918=CARTESIAN_POINT('Ctrl Pts',(-3.42855728381368,-1.,1.519044091397));
#51919=CARTESIAN_POINT('Ctrl Pts',(-3.42855728381368,1.,1.519044091397));
#51920=CARTESIAN_POINT('Ctrl Pts',(-3.42852521763778,-1.,1.51896318668366));
#51921=CARTESIAN_POINT('Ctrl Pts',(-3.42852521763778,1.,1.51896318668366));
#51922=CARTESIAN_POINT('Ctrl Pts',(-3.42860527149177,-1.,1.51888450659652));
#51923=CARTESIAN_POINT('Ctrl Pts',(-3.42860527149177,1.,1.51888450659652));
#51924=CARTESIAN_POINT('Ctrl Pts',(-3.42915787669893,-1.,1.51901585839109));
#51925=CARTESIAN_POINT('Ctrl Pts',(-3.42915787669893,1.,1.51901585839109));
#51926=CARTESIAN_POINT('Ctrl Pts',(-3.43076036253837,-1.,1.51969006980999));
#51927=CARTESIAN_POINT('Ctrl Pts',(-3.43076036253837,1.,1.51969006980999));
#51928=CARTESIAN_POINT('Ctrl Pts',(-3.43417156977893,-1.,1.52134826724292));
#51929=CARTESIAN_POINT('Ctrl Pts',(-3.43417156977893,1.,1.52134826724292));
#51930=CARTESIAN_POINT('Ctrl Pts',(-3.4388889597401,-1.,1.5237734895035));
#51931=CARTESIAN_POINT('Ctrl Pts',(-3.4388889597401,1.,1.5237734895035));
#51932=CARTESIAN_POINT('Ctrl Pts',(-3.44469547526647,-1.,1.52686242875556));
#51933=CARTESIAN_POINT('Ctrl Pts',(-3.44469547526647,1.,1.52686242875556));
#51934=CARTESIAN_POINT('Ctrl Pts',(-3.45127136828305,-1.,1.53046244461635));
#51935=CARTESIAN_POINT('Ctrl Pts',(-3.45127136828305,1.,1.53046244461635));
#51936=CARTESIAN_POINT('Ctrl Pts',(-3.45825932955032,-1.,1.53440195378792));
#51937=CARTESIAN_POINT('Ctrl Pts',(-3.45825932955032,1.,1.53440195378792));
#51938=CARTESIAN_POINT('Ctrl Pts',(-3.46531752207153,-1.,1.53851507915502));
#51939=CARTESIAN_POINT('Ctrl Pts',(-3.46531752207153,1.,1.53851507915502));
#51940=CARTESIAN_POINT('Ctrl Pts',(-3.47217189224653,-1.,1.54266605398187));
#51941=CARTESIAN_POINT('Ctrl Pts',(-3.47217189224653,1.,1.54266605398187));
#51942=CARTESIAN_POINT('Ctrl Pts',(-3.47868272898751,-1.,1.54678009290276));
#51943=CARTESIAN_POINT('Ctrl Pts',(-3.47868272898751,1.,1.54678009290276));
#51944=CARTESIAN_POINT('Ctrl Pts',(-3.48485155928567,-1.,1.55084702970452));
#51945=CARTESIAN_POINT('Ctrl Pts',(-3.48485155928567,1.,1.55084702970452));
#51946=CARTESIAN_POINT('Ctrl Pts',(-3.4907646087742,-1.,1.55489595901116));
#51947=CARTESIAN_POINT('Ctrl Pts',(-3.4907646087742,1.,1.55489595901116));
#51948=CARTESIAN_POINT('Ctrl Pts',(-3.49655185179655,-1.,1.55897703097874));
#51949=CARTESIAN_POINT('Ctrl Pts',(-3.49655185179655,1.,1.55897703097874));
#51950=CARTESIAN_POINT('Ctrl Pts',(-3.50234321621578,-1.,1.56314187758675));
#51951=CARTESIAN_POINT('Ctrl Pts',(-3.50234321621578,1.,1.56314187758675));
#51952=CARTESIAN_POINT('Ctrl Pts',(-3.50821771695363,-1.,1.56742097575012));
#51953=CARTESIAN_POINT('Ctrl Pts',(-3.50821771695363,1.,1.56742097575012));
#51954=CARTESIAN_POINT('Ctrl Pts',(-3.51418598431665,-1.,1.57181569799743));
#51955=CARTESIAN_POINT('Ctrl Pts',(-3.51418598431665,1.,1.57181569799743));
#51956=CARTESIAN_POINT('Ctrl Pts',(-3.52021847865912,-1.,1.57631049988158));
#51957=CARTESIAN_POINT('Ctrl Pts',(-3.52021847865912,1.,1.57631049988158));
#51958=CARTESIAN_POINT('Ctrl Pts',(-3.52626275334881,-1.,1.58088027227848));
#51959=CARTESIAN_POINT('Ctrl Pts',(-3.52626275334881,1.,1.58088027227848));
#51960=CARTESIAN_POINT('Ctrl Pts',(-3.5322637814708,-1.,1.58549906268088));
#51961=CARTESIAN_POINT('Ctrl Pts',(-3.5322637814708,1.,1.58549906268088));
#51962=CARTESIAN_POINT('Ctrl Pts',(-3.53818616861077,-1.,1.59014958368739));
#51963=CARTESIAN_POINT('Ctrl Pts',(-3.53818616861077,1.,1.59014958368739));
#51964=CARTESIAN_POINT('Ctrl Pts',(-3.54402458182337,-1.,1.59482766949766));
#51965=CARTESIAN_POINT('Ctrl Pts',(-3.54402458182337,1.,1.59482766949766));
#51966=CARTESIAN_POINT('Ctrl Pts',(-3.54979148634454,-1.,1.59953698113457));
#51967=CARTESIAN_POINT('Ctrl Pts',(-3.54979148634454,1.,1.59953698113457));
#51968=CARTESIAN_POINT('Ctrl Pts',(-3.55550985096129,-1.,1.60428584699853));
#51969=CARTESIAN_POINT('Ctrl Pts',(-3.55550985096129,1.,1.60428584699853));
#51970=CARTESIAN_POINT('Ctrl Pts',(-3.5612043248298,-1.,1.60908344685457));
#51971=CARTESIAN_POINT('Ctrl Pts',(-3.5612043248298,1.,1.60908344685457));
#51972=CARTESIAN_POINT('Ctrl Pts',(-3.56689200468387,-1.,1.61393581747514));
#51973=CARTESIAN_POINT('Ctrl Pts',(-3.56689200468387,1.,1.61393581747514));
#51974=CARTESIAN_POINT('Ctrl Pts',(-3.57257679609806,-1.,1.61884340915404));
#51975=CARTESIAN_POINT('Ctrl Pts',(-3.57257679609806,1.,1.61884340915404));
#51976=CARTESIAN_POINT('Ctrl Pts',(-3.5782545595439,-1.,1.62380329464844));
#51977=CARTESIAN_POINT('Ctrl Pts',(-3.5782545595439,1.,1.62380329464844));
#51978=CARTESIAN_POINT('Ctrl Pts',(-3.58391625774343,-1.,1.62881051550745));
#51979=CARTESIAN_POINT('Ctrl Pts',(-3.58391625774343,1.,1.62881051550745));
#51980=CARTESIAN_POINT('Ctrl Pts',(-3.58955176627879,-1.,1.6338597145126));
#51981=CARTESIAN_POINT('Ctrl Pts',(-3.58955176627879,1.,1.6338597145126));
#51982=CARTESIAN_POINT('Ctrl Pts',(-3.59515368334893,-1.,1.63894676675352));
#51983=CARTESIAN_POINT('Ctrl Pts',(-3.59515368334893,1.,1.63894676675352));
#51984=CARTESIAN_POINT('Ctrl Pts',(-3.60072028513845,-1.,1.64407004385582));
#51985=CARTESIAN_POINT('Ctrl Pts',(-3.60072028513845,1.,1.64407004385582));
#51986=CARTESIAN_POINT('Ctrl Pts',(-3.60625346556992,-1.,1.64922952425832));
#51987=CARTESIAN_POINT('Ctrl Pts',(-3.60625346556992,1.,1.64922952425832));
#51988=CARTESIAN_POINT('Ctrl Pts',(-3.61175734965127,-1.,1.65442619244325));
#51989=CARTESIAN_POINT('Ctrl Pts',(-3.61175734965127,1.,1.65442619244325));
#51990=CARTESIAN_POINT('Ctrl Pts',(-3.61723666482456,-1.,1.65966133399186));
#51991=CARTESIAN_POINT('Ctrl Pts',(-3.61723666482456,1.,1.65966133399186));
#51992=CARTESIAN_POINT('Ctrl Pts',(-3.62269517989109,-1.,1.66493585923855));
#51993=CARTESIAN_POINT('Ctrl Pts',(-3.62269517989109,1.,1.66493585923855));
#51994=CARTESIAN_POINT('Ctrl Pts',(-3.62813422105271,-1.,1.67024966008045));
#51995=CARTESIAN_POINT('Ctrl Pts',(-3.62813422105271,1.,1.67024966008045));
#51996=CARTESIAN_POINT('Ctrl Pts',(-3.63355343201232,-1.,1.67560193613156));
#51997=CARTESIAN_POINT('Ctrl Pts',(-3.63355343201232,1.,1.67560193613156));
#51998=CARTESIAN_POINT('Ctrl Pts',(-3.63895140887462,-1.,1.68099146651586));
#51999=CARTESIAN_POINT('Ctrl Pts',(-3.63895140887462,1.,1.68099146651586));
#52000=CARTESIAN_POINT('Ctrl Pts',(-3.64432638915203,-1.,1.68641690471457));
#52001=CARTESIAN_POINT('Ctrl Pts',(-3.64432638915203,1.,1.68641690471457));
#52002=CARTESIAN_POINT('Ctrl Pts',(-3.64967689827371,-1.,1.69187705481689));
#52003=CARTESIAN_POINT('Ctrl Pts',(-3.64967689827371,1.,1.69187705481689));
#52004=CARTESIAN_POINT('Ctrl Pts',(-3.65500246526749,-1.,1.69737117722534));
#52005=CARTESIAN_POINT('Ctrl Pts',(-3.65500246526749,1.,1.69737117722534));
#52006=CARTESIAN_POINT('Ctrl Pts',(-3.66030338774847,-1.,1.70289888566873));
#52007=CARTESIAN_POINT('Ctrl Pts',(-3.66030338774847,1.,1.70289888566873));
#52008=CARTESIAN_POINT('Ctrl Pts',(-3.66558043198876,-1.,1.70846001610956));
#52009=CARTESIAN_POINT('Ctrl Pts',(-3.66558043198876,1.,1.70846001610956));
#52010=CARTESIAN_POINT('Ctrl Pts',(-3.67083454901611,-1.,1.71405450210383));
#52011=CARTESIAN_POINT('Ctrl Pts',(-3.67083454901611,1.,1.71405450210383));
#52012=CARTESIAN_POINT('Ctrl Pts',(-3.67606660374709,-1.,1.71968225581808));
#52013=CARTESIAN_POINT('Ctrl Pts',(-3.67606660374709,1.,1.71968225581808));
#52014=CARTESIAN_POINT('Ctrl Pts',(-3.68127704936579,-1.,1.72534302437056));
#52015=CARTESIAN_POINT('Ctrl Pts',(-3.68127704936579,1.,1.72534302437056));
#52016=CARTESIAN_POINT('Ctrl Pts',(-3.68646597019332,-1.,1.73103640956717));
#52017=CARTESIAN_POINT('Ctrl Pts',(-3.68646597019332,1.,1.73103640956717));
#52018=CARTESIAN_POINT('Ctrl Pts',(-3.69163322648036,-1.,1.73676193254557));
#52019=CARTESIAN_POINT('Ctrl Pts',(-3.69163322648036,1.,1.73676193254557));
#52020=CARTESIAN_POINT('Ctrl Pts',(-3.69677856910517,-1.,1.74251908492617));
#52021=CARTESIAN_POINT('Ctrl Pts',(-3.69677856910517,1.,1.74251908492617));
#52022=CARTESIAN_POINT('Ctrl Pts',(-3.7019017567335,-1.,1.74830738046057));
#52023=CARTESIAN_POINT('Ctrl Pts',(-3.7019017567335,1.,1.74830738046057));
#52024=CARTESIAN_POINT('Ctrl Pts',(-3.70700269736659,-1.,1.75412641804042));
#52025=CARTESIAN_POINT('Ctrl Pts',(-3.70700269736659,1.,1.75412641804042));
#52026=CARTESIAN_POINT('Ctrl Pts',(-3.71208146346136,-1.,1.75997588498865));
#52027=CARTESIAN_POINT('Ctrl Pts',(-3.71208146346136,1.,1.75997588498865));
#52028=CARTESIAN_POINT('Ctrl Pts',(-3.71713822377359,-1.,1.76585552124394));
#52029=CARTESIAN_POINT('Ctrl Pts',(-3.71713822377359,1.,1.76585552124394));
#52030=CARTESIAN_POINT('Ctrl Pts',(-3.72217319911254,-1.,1.77176509401761));
#52031=CARTESIAN_POINT('Ctrl Pts',(-3.72217319911254,1.,1.77176509401761));
#52032=CARTESIAN_POINT('Ctrl Pts',(-3.72718661205609,-1.,1.77770437039658));
#52033=CARTESIAN_POINT('Ctrl Pts',(-3.72718661205609,1.,1.77770437039658));
#52034=CARTESIAN_POINT('Ctrl Pts',(-3.7321786309547,-1.,1.78367308442901));
#52035=CARTESIAN_POINT('Ctrl Pts',(-3.7321786309547,1.,1.78367308442901));
#52036=CARTESIAN_POINT('Ctrl Pts',(-3.73714934730681,-1.,1.78967092823491));
#52037=CARTESIAN_POINT('Ctrl Pts',(-3.73714934730681,1.,1.78967092823491));
#52038=CARTESIAN_POINT('Ctrl Pts',(-3.74209880352445,-1.,1.79569757859422));
#52039=CARTESIAN_POINT('Ctrl Pts',(-3.74209880352445,1.,1.79569757859422));
#52040=CARTESIAN_POINT('Ctrl Pts',(-3.74702700875467,-1.,1.8017527148577));
#52041=CARTESIAN_POINT('Ctrl Pts',(-3.74702700875467,1.,1.8017527148577));
#52042=CARTESIAN_POINT('Ctrl Pts',(-3.75193395887977,-1.,1.80783603939617));
#52043=CARTESIAN_POINT('Ctrl Pts',(-3.75193395887977,1.,1.80783603939617));
#52044=CARTESIAN_POINT('Ctrl Pts',(-3.75681965683071,-1.,1.8139472983358));
#52045=CARTESIAN_POINT('Ctrl Pts',(-3.75681965683071,1.,1.8139472983358));
#52046=CARTESIAN_POINT('Ctrl Pts',(-3.76168412707948,-1.,1.82008629694091));
#52047=CARTESIAN_POINT('Ctrl Pts',(-3.76168412707948,1.,1.82008629694091));
#52048=CARTESIAN_POINT('Ctrl Pts',(-3.76652740353775,-1.,1.82625289220915));
#52049=CARTESIAN_POINT('Ctrl Pts',(-3.76652740353775,1.,1.82625289220915));
#52050=CARTESIAN_POINT('Ctrl Pts',(-3.77038509817999,-1.,1.83120816955645));
#52051=CARTESIAN_POINT('Ctrl Pts',(-3.77038509817999,1.,1.83120816955645));
#52052=CARTESIAN_POINT('Ctrl Pts',(-3.77326886064398,-1.,1.83493697934534));
#52053=CARTESIAN_POINT('Ctrl Pts',(-3.77326886064398,1.,1.83493697934534));
#52054=CARTESIAN_POINT('Ctrl Pts',(-3.77518714457833,-1.,1.83742834010626));
#52055=CARTESIAN_POINT('Ctrl Pts',(-3.77518714457833,1.,1.83742834010626));
#52056=CARTESIAN_POINT('Ctrl Pts',(-3.77614523045147,-1.,1.8386753923786));
#52057=CARTESIAN_POINT('Ctrl Pts',(-3.77614523045147,1.,1.8386753923786));
#52058=CARTESIAN_POINT('',(-3.42859860294306,1.,1.5189508286633));
#52059=CARTESIAN_POINT('Ctrl Pts',(-3.42859860294306,-1.,1.5189508286633));
#52060=CARTESIAN_POINT('Ctrl Pts',(-3.42859860294306,-0.666666666666667,
1.5189508286633));
#52061=CARTESIAN_POINT('Ctrl Pts',(-3.42859860294306,-0.333333333333333,
1.5189508286633));
#52062=CARTESIAN_POINT('Ctrl Pts',(-3.42859860294306,0.333333333333333,
1.5189508286633));
#52063=CARTESIAN_POINT('Ctrl Pts',(-3.42859860294306,0.666666666666667,
1.5189508286633));
#52064=CARTESIAN_POINT('Ctrl Pts',(-3.42859860294306,1.,1.5189508286633));
#52065=CARTESIAN_POINT('',(-3.77614523045147,1.,1.8386753923786));
#52066=CARTESIAN_POINT('',(-3.77614523045147,0.,1.8386753923786));
#52067=CARTESIAN_POINT('Ctrl Pts',(-3.42859860294306,1.,1.5189508286633));
#52068=CARTESIAN_POINT('Ctrl Pts',(-3.42864616361875,1.,1.51893924967331));
#52069=CARTESIAN_POINT('Ctrl Pts',(-3.42884302333841,1.,1.5189513329503));
#52070=CARTESIAN_POINT('Ctrl Pts',(-3.42946838852587,1.,1.51914806898491));
#52071=CARTESIAN_POINT('Ctrl Pts',(-3.43101631893414,1.,1.5198144909338));
#52072=CARTESIAN_POINT('Ctrl Pts',(-3.43417156977893,1.,1.52134826724292));
#52073=CARTESIAN_POINT('Ctrl Pts',(-3.4388889597401,1.,1.5237734895035));
#52074=CARTESIAN_POINT('Ctrl Pts',(-3.44469547526647,1.,1.52686242875556));
#52075=CARTESIAN_POINT('Ctrl Pts',(-3.45127136828305,1.,1.53046244461635));
#52076=CARTESIAN_POINT('Ctrl Pts',(-3.45825932955032,1.,1.53440195378792));
#52077=CARTESIAN_POINT('Ctrl Pts',(-3.46531752207153,1.,1.53851507915502));
#52078=CARTESIAN_POINT('Ctrl Pts',(-3.47217189224653,1.,1.54266605398187));
#52079=CARTESIAN_POINT('Ctrl Pts',(-3.47868272898751,1.,1.54678009290276));
#52080=CARTESIAN_POINT('Ctrl Pts',(-3.48485155928567,1.,1.55084702970452));
#52081=CARTESIAN_POINT('Ctrl Pts',(-3.4907646087742,1.,1.55489595901116));
#52082=CARTESIAN_POINT('Ctrl Pts',(-3.49655185179655,1.,1.55897703097874));
#52083=CARTESIAN_POINT('Ctrl Pts',(-3.50234321621578,1.,1.56314187758675));
#52084=CARTESIAN_POINT('Ctrl Pts',(-3.50821771695363,1.,1.56742097575012));
#52085=CARTESIAN_POINT('Ctrl Pts',(-3.51418598431665,1.,1.57181569799743));
#52086=CARTESIAN_POINT('Ctrl Pts',(-3.52021847865912,1.,1.57631049988158));
#52087=CARTESIAN_POINT('Ctrl Pts',(-3.52626275334881,1.,1.58088027227848));
#52088=CARTESIAN_POINT('Ctrl Pts',(-3.5322637814708,1.,1.58549906268088));
#52089=CARTESIAN_POINT('Ctrl Pts',(-3.53818616861077,1.,1.59014958368739));
#52090=CARTESIAN_POINT('Ctrl Pts',(-3.54402458182337,1.,1.59482766949766));
#52091=CARTESIAN_POINT('Ctrl Pts',(-3.54979148634454,1.,1.59953698113457));
#52092=CARTESIAN_POINT('Ctrl Pts',(-3.55550985096129,1.,1.60428584699853));
#52093=CARTESIAN_POINT('Ctrl Pts',(-3.5612043248298,1.,1.60908344685457));
#52094=CARTESIAN_POINT('Ctrl Pts',(-3.56689200468387,1.,1.61393581747514));
#52095=CARTESIAN_POINT('Ctrl Pts',(-3.57257679609806,1.,1.61884340915404));
#52096=CARTESIAN_POINT('Ctrl Pts',(-3.5782545595439,1.,1.62380329464844));
#52097=CARTESIAN_POINT('Ctrl Pts',(-3.58391625774343,1.,1.62881051550745));
#52098=CARTESIAN_POINT('Ctrl Pts',(-3.58955176627879,1.,1.6338597145126));
#52099=CARTESIAN_POINT('Ctrl Pts',(-3.59515368334893,1.,1.63894676675352));
#52100=CARTESIAN_POINT('Ctrl Pts',(-3.60072028513845,1.,1.64407004385582));
#52101=CARTESIAN_POINT('Ctrl Pts',(-3.60625346556992,1.,1.64922952425832));
#52102=CARTESIAN_POINT('Ctrl Pts',(-3.61175734965127,1.,1.65442619244325));
#52103=CARTESIAN_POINT('Ctrl Pts',(-3.61723666482456,1.,1.65966133399186));
#52104=CARTESIAN_POINT('Ctrl Pts',(-3.62269517989109,1.,1.66493585923855));
#52105=CARTESIAN_POINT('Ctrl Pts',(-3.62813422105271,1.,1.67024966008045));
#52106=CARTESIAN_POINT('Ctrl Pts',(-3.63355343201232,1.,1.67560193613156));
#52107=CARTESIAN_POINT('Ctrl Pts',(-3.63895140887462,1.,1.68099146651586));
#52108=CARTESIAN_POINT('Ctrl Pts',(-3.64432638915203,1.,1.68641690471457));
#52109=CARTESIAN_POINT('Ctrl Pts',(-3.64967689827371,1.,1.69187705481689));
#52110=CARTESIAN_POINT('Ctrl Pts',(-3.65500246526749,1.,1.69737117722534));
#52111=CARTESIAN_POINT('Ctrl Pts',(-3.66030338774847,1.,1.70289888566873));
#52112=CARTESIAN_POINT('Ctrl Pts',(-3.66558043198876,1.,1.70846001610956));
#52113=CARTESIAN_POINT('Ctrl Pts',(-3.67083454901611,1.,1.71405450210383));
#52114=CARTESIAN_POINT('Ctrl Pts',(-3.67606660374709,1.,1.71968225581808));
#52115=CARTESIAN_POINT('Ctrl Pts',(-3.68127704936579,1.,1.72534302437056));
#52116=CARTESIAN_POINT('Ctrl Pts',(-3.68646597019332,1.,1.73103640956717));
#52117=CARTESIAN_POINT('Ctrl Pts',(-3.69163322648036,1.,1.73676193254557));
#52118=CARTESIAN_POINT('Ctrl Pts',(-3.69677856910517,1.,1.74251908492617));
#52119=CARTESIAN_POINT('Ctrl Pts',(-3.7019017567335,1.,1.74830738046057));
#52120=CARTESIAN_POINT('Ctrl Pts',(-3.70700269736659,1.,1.75412641804042));
#52121=CARTESIAN_POINT('Ctrl Pts',(-3.71208146346136,1.,1.75997588498865));
#52122=CARTESIAN_POINT('Ctrl Pts',(-3.71713822377359,1.,1.76585552124394));
#52123=CARTESIAN_POINT('Ctrl Pts',(-3.72217319911254,1.,1.77176509401761));
#52124=CARTESIAN_POINT('Ctrl Pts',(-3.72718661205609,1.,1.77770437039658));
#52125=CARTESIAN_POINT('Ctrl Pts',(-3.7321786309547,1.,1.78367308442901));
#52126=CARTESIAN_POINT('Ctrl Pts',(-3.73714934730681,1.,1.78967092823491));
#52127=CARTESIAN_POINT('Ctrl Pts',(-3.74209880352445,1.,1.79569757859422));
#52128=CARTESIAN_POINT('Ctrl Pts',(-3.74702700875467,1.,1.8017527148577));
#52129=CARTESIAN_POINT('Ctrl Pts',(-3.75193395887977,1.,1.80783603939617));
#52130=CARTESIAN_POINT('Ctrl Pts',(-3.75681965683071,1.,1.8139472983358));
#52131=CARTESIAN_POINT('Ctrl Pts',(-3.76168412707948,1.,1.82008629694091));
#52132=CARTESIAN_POINT('Ctrl Pts',(-3.76652740353775,1.,1.82625289220915));
#52133=CARTESIAN_POINT('Ctrl Pts',(-3.77038509817999,1.,1.83120816955645));
#52134=CARTESIAN_POINT('Ctrl Pts',(-3.77326886064398,1.,1.83493697934534));
#52135=CARTESIAN_POINT('Ctrl Pts',(-3.77518714457833,1.,1.83742834010626));
#52136=CARTESIAN_POINT('Ctrl Pts',(-3.77614523045147,1.,1.8386753923786));
#52137=CARTESIAN_POINT('Origin',(-3.77614523045147,0.,1.8386753923786));
#52138=CARTESIAN_POINT('',(-3.70708211654725,1.,1.97421938526992));
#52139=CARTESIAN_POINT('Origin',(0.,0.,0.));
#52140=CARTESIAN_POINT('',(-3.49844575334386,1.,1.35032489087269));
#52141=CARTESIAN_POINT('Origin',(0.,1.,0.));
#52142=CARTESIAN_POINT('Ctrl Pts',(-3.49844575334386,1.,1.35032489087269));
#52143=CARTESIAN_POINT('Ctrl Pts',(-3.49844575334386,0.666666666666667,
1.35032489087269));
#52144=CARTESIAN_POINT('Ctrl Pts',(-3.49844575334386,0.333333333333333,
1.35032489087269));
#52145=CARTESIAN_POINT('Ctrl Pts',(-3.49844575334386,-0.333333333333333,
1.35032489087269));
#52146=CARTESIAN_POINT('Ctrl Pts',(-3.49844575334386,-0.666666666666667,
1.35032489087269));
#52147=CARTESIAN_POINT('Ctrl Pts',(-3.49844575334386,-1.,1.35032489087269));
#52148=CARTESIAN_POINT('Ctrl Pts',(-3.97027773754922,-1.,1.36999806084572));
#52149=CARTESIAN_POINT('Ctrl Pts',(-3.97027773754922,1.,1.36999806084572));
#52150=CARTESIAN_POINT('Ctrl Pts',(-3.9687184694173,-1.,1.37020239094758));
#52151=CARTESIAN_POINT('Ctrl Pts',(-3.9687184694173,1.,1.37020239094758));
#52152=CARTESIAN_POINT('Ctrl Pts',(-3.96560037975788,-1.,1.37060761746027));
#52153=CARTESIAN_POINT('Ctrl Pts',(-3.96560037975788,1.,1.37060761746027));
#52154=CARTESIAN_POINT('Ctrl Pts',(-3.96092458508407,-1.,1.37120515615663));
#52155=CARTESIAN_POINT('Ctrl Pts',(-3.96092458508407,1.,1.37120515615663));
#52156=CARTESIAN_POINT('Ctrl Pts',(-3.95469287283105,-1.,1.37198126433139));
#52157=CARTESIAN_POINT('Ctrl Pts',(-3.95469287283105,1.,1.37198126433139));
#52158=CARTESIAN_POINT('Ctrl Pts',(-3.94690771786926,-1.,1.37291699203423));
#52159=CARTESIAN_POINT('Ctrl Pts',(-3.94690771786926,1.,1.37291699203423));
#52160=CARTESIAN_POINT('Ctrl Pts',(-3.93912709041791,-1.,1.37381821967499));
#52161=CARTESIAN_POINT('Ctrl Pts',(-3.93912709041791,1.,1.37381821967499));
#52162=CARTESIAN_POINT('Ctrl Pts',(-3.93135106761941,-1.,1.37468482215784));
#52163=CARTESIAN_POINT('Ctrl Pts',(-3.93135106761941,1.,1.37468482215784));
#52164=CARTESIAN_POINT('Ctrl Pts',(-3.92357976987132,-1.,1.37551664448057));
#52165=CARTESIAN_POINT('Ctrl Pts',(-3.92357976987132,1.,1.37551664448057));
#52166=CARTESIAN_POINT('Ctrl Pts',(-3.91581337461825,-1.,1.37631350505516));
#52167=CARTESIAN_POINT('Ctrl Pts',(-3.91581337461825,1.,1.37631350505516));
#52168=CARTESIAN_POINT('Ctrl Pts',(-3.90805209522729,-1.,1.3770751963376));
#52169=CARTESIAN_POINT('Ctrl Pts',(-3.90805209522729,1.,1.3770751963376));
#52170=CARTESIAN_POINT('Ctrl Pts',(-3.90029615196255,-1.,1.3778014851263));
#52171=CARTESIAN_POINT('Ctrl Pts',(-3.90029615196255,1.,1.3778014851263));
#52172=CARTESIAN_POINT('Ctrl Pts',(-3.89254574338385,-1.,1.37849211287981));
#52173=CARTESIAN_POINT('Ctrl Pts',(-3.89254574338385,1.,1.37849211287981));
#52174=CARTESIAN_POINT('Ctrl Pts',(-3.88480102249461,-1.,1.37914679719446));
#52175=CARTESIAN_POINT('Ctrl Pts',(-3.88480102249461,1.,1.37914679719446));
#52176=CARTESIAN_POINT('Ctrl Pts',(-3.87706205830865,-1.,1.37976523097187));
#52177=CARTESIAN_POINT('Ctrl Pts',(-3.87706205830865,1.,1.37976523097187));
#52178=CARTESIAN_POINT('Ctrl Pts',(-3.86932885813403,-1.,1.38034709213129));
#52179=CARTESIAN_POINT('Ctrl Pts',(-3.86932885813403,1.,1.38034709213129));
#52180=CARTESIAN_POINT('Ctrl Pts',(-3.86160143044187,-1.,1.38089205993067));
#52181=CARTESIAN_POINT('Ctrl Pts',(-3.86160143044187,1.,1.38089205993067));
#52182=CARTESIAN_POINT('Ctrl Pts',(-3.85387983979557,-1.,1.38139983115075));
#52183=CARTESIAN_POINT('Ctrl Pts',(-3.85387983979557,1.,1.38139983115075));
#52184=CARTESIAN_POINT('Ctrl Pts',(-3.84616425605705,-1.,1.38187013346089));
#52185=CARTESIAN_POINT('Ctrl Pts',(-3.84616425605705,1.,1.38187013346089));
#52186=CARTESIAN_POINT('Ctrl Pts',(-3.83845502790609,-1.,1.38230274828774));
#52187=CARTESIAN_POINT('Ctrl Pts',(-3.83845502790609,1.,1.38230274828774));
#52188=CARTESIAN_POINT('Ctrl Pts',(-3.83075266982138,-1.,1.38269750245086));
#52189=CARTESIAN_POINT('Ctrl Pts',(-3.83075266982138,1.,1.38269750245086));
#52190=CARTESIAN_POINT('Ctrl Pts',(-3.82305771743715,-1.,1.38305421262724));
#52191=CARTESIAN_POINT('Ctrl Pts',(-3.82305771743715,1.,1.38305421262724));
#52192=CARTESIAN_POINT('Ctrl Pts',(-3.81537060817765,-1.,1.38337263902766));
#52193=CARTESIAN_POINT('Ctrl Pts',(-3.81537060817765,1.,1.38337263902766));
#52194=CARTESIAN_POINT('Ctrl Pts',(-3.80769156398429,-1.,1.38365244046226));
#52195=CARTESIAN_POINT('Ctrl Pts',(-3.80769156398429,1.,1.38365244046226));
#52196=CARTESIAN_POINT('Ctrl Pts',(-3.80002044322169,-1.,1.38389311766701));
#52197=CARTESIAN_POINT('Ctrl Pts',(-3.80002044322169,1.,1.38389311766701));
#52198=CARTESIAN_POINT('Ctrl Pts',(-3.79235669640907,-1.,1.38409399694588));
#52199=CARTESIAN_POINT('Ctrl Pts',(-3.79235669640907,1.,1.38409399694588));
#52200=CARTESIAN_POINT('Ctrl Pts',(-3.78469969805134,-1.,1.38425435883773));
#52201=CARTESIAN_POINT('Ctrl Pts',(-3.78469969805134,1.,1.38425435883773));
#52202=CARTESIAN_POINT('Ctrl Pts',(-3.77704902230441,-1.,1.38437354551435));
#52203=CARTESIAN_POINT('Ctrl Pts',(-3.77704902230441,1.,1.38437354551435));
#52204=CARTESIAN_POINT('Ctrl Pts',(-3.76940473185775,-1.,1.38445107339517));
#52205=CARTESIAN_POINT('Ctrl Pts',(-3.76940473185775,1.,1.38445107339517));
#52206=CARTESIAN_POINT('Ctrl Pts',(-3.76176768271347,-1.,1.38448675253343));
#52207=CARTESIAN_POINT('Ctrl Pts',(-3.76176768271347,1.,1.38448675253343));
#52208=CARTESIAN_POINT('Ctrl Pts',(-3.75413976318727,-1.,1.38448077997155));
#52209=CARTESIAN_POINT('Ctrl Pts',(-3.75413976318727,1.,1.38448077997155));
#52210=CARTESIAN_POINT('Ctrl Pts',(-3.7465231716786,-1.,1.38443344984389));
#52211=CARTESIAN_POINT('Ctrl Pts',(-3.7465231716786,1.,1.38443344984389));
#52212=CARTESIAN_POINT('Ctrl Pts',(-3.73891976418099,-1.,1.38434489156456));
#52213=CARTESIAN_POINT('Ctrl Pts',(-3.73891976418099,1.,1.38434489156456));
#52214=CARTESIAN_POINT('Ctrl Pts',(-3.73133035859283,-1.,1.38421479111531));
#52215=CARTESIAN_POINT('Ctrl Pts',(-3.73133035859283,1.,1.38421479111531));
#52216=CARTESIAN_POINT('Ctrl Pts',(-3.72375409358805,-1.,1.3840421342895));
#52217=CARTESIAN_POINT('Ctrl Pts',(-3.72375409358805,1.,1.3840421342895));
#52218=CARTESIAN_POINT('Ctrl Pts',(-3.7161876605181,-1.,1.38382489984585));
#52219=CARTESIAN_POINT('Ctrl Pts',(-3.7161876605181,1.,1.38382489984585));
#52220=CARTESIAN_POINT('Ctrl Pts',(-3.70862680753343,-1.,1.38356065402122));
#52221=CARTESIAN_POINT('Ctrl Pts',(-3.70862680753343,1.,1.38356065402122));
#52222=CARTESIAN_POINT('Ctrl Pts',(-3.70106792167894,-1.,1.38324717612862));
#52223=CARTESIAN_POINT('Ctrl Pts',(-3.70106792167894,1.,1.38324717612862));
#52224=CARTESIAN_POINT('Ctrl Pts',(-3.69350967899523,-1.,1.38288311171649));
#52225=CARTESIAN_POINT('Ctrl Pts',(-3.69350967899523,1.,1.38288311171649));
#52226=CARTESIAN_POINT('Ctrl Pts',(-3.68595444983844,-1.,1.38246852827185));
#52227=CARTESIAN_POINT('Ctrl Pts',(-3.68595444983844,1.,1.38246852827185));
#52228=CARTESIAN_POINT('Ctrl Pts',(-3.6784103848243,-1.,1.38200574290626));
#52229=CARTESIAN_POINT('Ctrl Pts',(-3.6784103848243,1.,1.38200574290626));
#52230=CARTESIAN_POINT('Ctrl Pts',(-3.67088843112282,-1.,1.38149812653876));
#52231=CARTESIAN_POINT('Ctrl Pts',(-3.67088843112282,1.,1.38149812653876));
#52232=CARTESIAN_POINT('Ctrl Pts',(-3.66339848520874,-1.,1.38094856333558));
#52233=CARTESIAN_POINT('Ctrl Pts',(-3.66339848520874,1.,1.38094856333558));
#52234=CARTESIAN_POINT('Ctrl Pts',(-3.65594554404396,-1.,1.38035791051215));
#52235=CARTESIAN_POINT('Ctrl Pts',(-3.65594554404396,1.,1.38035791051215));
#52236=CARTESIAN_POINT('Ctrl Pts',(-3.64852652756444,-1.,1.37972372481598));
#52237=CARTESIAN_POINT('Ctrl Pts',(-3.64852652756444,1.,1.37972372481598));
#52238=CARTESIAN_POINT('Ctrl Pts',(-3.64112507791112,-1.,1.37903818567347));
#52239=CARTESIAN_POINT('Ctrl Pts',(-3.64112507791112,1.,1.37903818567347));
#52240=CARTESIAN_POINT('Ctrl Pts',(-3.63371727442448,-1.,1.37829035457324));
#52241=CARTESIAN_POINT('Ctrl Pts',(-3.63371727442448,1.,1.37829035457324));
#52242=CARTESIAN_POINT('Ctrl Pts',(-3.62628098665112,-1.,1.37746987919868));
#52243=CARTESIAN_POINT('Ctrl Pts',(-3.62628098665112,1.,1.37746987919868));
#52244=CARTESIAN_POINT('Ctrl Pts',(-3.61880481160408,-1.,1.37657053403102));
#52245=CARTESIAN_POINT('Ctrl Pts',(-3.61880481160408,1.,1.37657053403102));
#52246=CARTESIAN_POINT('Ctrl Pts',(-3.61129546591082,-1.,1.37559314436641));
#52247=CARTESIAN_POINT('Ctrl Pts',(-3.61129546591082,1.,1.37559314436641));
#52248=CARTESIAN_POINT('Ctrl Pts',(-3.60379020124038,-1.,1.37455051379642));
#52249=CARTESIAN_POINT('Ctrl Pts',(-3.60379020124038,1.,1.37455051379642));
#52250=CARTESIAN_POINT('Ctrl Pts',(-3.59634627869117,-1.,1.37346320103184));
#52251=CARTESIAN_POINT('Ctrl Pts',(-3.59634627869117,1.,1.37346320103184));
#52252=CARTESIAN_POINT('Ctrl Pts',(-3.5890185384643,-1.,1.37235053661));
#52253=CARTESIAN_POINT('Ctrl Pts',(-3.5890185384643,1.,1.37235053661));
#52254=CARTESIAN_POINT('Ctrl Pts',(-3.58183885982745,-1.,1.37122241663073));
#52255=CARTESIAN_POINT('Ctrl Pts',(-3.58183885982745,1.,1.37122241663073));
#52256=CARTESIAN_POINT('Ctrl Pts',(-3.57479875549453,-1.,1.37007229485646));
#52257=CARTESIAN_POINT('Ctrl Pts',(-3.57479875549453,1.,1.37007229485646));
#52258=CARTESIAN_POINT('Ctrl Pts',(-3.56782080304554,-1.,1.36886584973349));
#52259=CARTESIAN_POINT('Ctrl Pts',(-3.56782080304554,1.,1.36886584973349));
#52260=CARTESIAN_POINT('Ctrl Pts',(-3.56077662028492,-1.,1.36754771771174));
#52261=CARTESIAN_POINT('Ctrl Pts',(-3.56077662028492,1.,1.36754771771174));
#52262=CARTESIAN_POINT('Ctrl Pts',(-3.55353883995793,-1.,1.36606145456711));
#52263=CARTESIAN_POINT('Ctrl Pts',(-3.55353883995793,1.,1.36606145456711));
#52264=CARTESIAN_POINT('Ctrl Pts',(-3.54602591832893,-1.,1.36436666257567));
#52265=CARTESIAN_POINT('Ctrl Pts',(-3.54602591832893,1.,1.36436666257567));
#52266=CARTESIAN_POINT('Ctrl Pts',(-3.53824396425032,-1.,1.36245507339334));
#52267=CARTESIAN_POINT('Ctrl Pts',(-3.53824396425032,1.,1.36245507339334));
#52268=CARTESIAN_POINT('Ctrl Pts',(-3.53034464961849,-1.,1.36037259643827));
#52269=CARTESIAN_POINT('Ctrl Pts',(-3.53034464961849,1.,1.36037259643827));
#52270=CARTESIAN_POINT('Ctrl Pts',(-3.52261776117121,-1.,1.35821701528975));
#52271=CARTESIAN_POINT('Ctrl Pts',(-3.52261776117121,1.,1.35821701528975));
#52272=CARTESIAN_POINT('Ctrl Pts',(-3.51542230699919,-1.,1.35611275237288));
#52273=CARTESIAN_POINT('Ctrl Pts',(-3.51542230699919,1.,1.35611275237288));
#52274=CARTESIAN_POINT('Ctrl Pts',(-3.50913227060177,-1.,1.35419113576022));
#52275=CARTESIAN_POINT('Ctrl Pts',(-3.50913227060177,1.,1.35419113576022));
#52276=CARTESIAN_POINT('Ctrl Pts',(-3.50408168106113,-1.,1.3525703284343));
#52277=CARTESIAN_POINT('Ctrl Pts',(-3.50408168106113,1.,1.3525703284343));
#52278=CARTESIAN_POINT('Ctrl Pts',(-3.50049707063673,-1.,1.35133076331065));
#52279=CARTESIAN_POINT('Ctrl Pts',(-3.50049707063673,1.,1.35133076331065));
#52280=CARTESIAN_POINT('Ctrl Pts',(-3.49888720256612,-1.,1.35067437417289));
#52281=CARTESIAN_POINT('Ctrl Pts',(-3.49888720256612,1.,1.35067437417289));
#52282=CARTESIAN_POINT('Ctrl Pts',(-3.49840357193384,-1.,1.35037650302887));
#52283=CARTESIAN_POINT('Ctrl Pts',(-3.49840357193384,1.,1.35037650302887));
#52284=CARTESIAN_POINT('Ctrl Pts',(-3.49840260053616,-1.,1.35026426118351));
#52285=CARTESIAN_POINT('Ctrl Pts',(-3.49840260053616,1.,1.35026426118351));
#52286=CARTESIAN_POINT('Ctrl Pts',(-3.49848248301936,-1.,1.35022972712301));
#52287=CARTESIAN_POINT('Ctrl Pts',(-3.49848248301936,1.,1.35022972712301));
#52288=CARTESIAN_POINT('',(-3.97027773754922,1.,1.36999806084572));
#52289=CARTESIAN_POINT('Ctrl Pts',(-3.97027773754922,1.,1.36999806084572));
#52290=CARTESIAN_POINT('Ctrl Pts',(-3.9687184694173,1.,1.37020239094758));
#52291=CARTESIAN_POINT('Ctrl Pts',(-3.96560037975788,1.,1.37060761746027));
#52292=CARTESIAN_POINT('Ctrl Pts',(-3.96092458508407,1.,1.37120515615663));
#52293=CARTESIAN_POINT('Ctrl Pts',(-3.95469287283105,1.,1.37198126433139));
#52294=CARTESIAN_POINT('Ctrl Pts',(-3.94690771786926,1.,1.37291699203423));
#52295=CARTESIAN_POINT('Ctrl Pts',(-3.93912709041791,1.,1.37381821967499));
#52296=CARTESIAN_POINT('Ctrl Pts',(-3.93135106761941,1.,1.37468482215784));
#52297=CARTESIAN_POINT('Ctrl Pts',(-3.92357976987132,1.,1.37551664448057));
#52298=CARTESIAN_POINT('Ctrl Pts',(-3.91581337461825,1.,1.37631350505516));
#52299=CARTESIAN_POINT('Ctrl Pts',(-3.90805209522729,1.,1.3770751963376));
#52300=CARTESIAN_POINT('Ctrl Pts',(-3.90029615196255,1.,1.3778014851263));
#52301=CARTESIAN_POINT('Ctrl Pts',(-3.89254574338385,1.,1.37849211287981));
#52302=CARTESIAN_POINT('Ctrl Pts',(-3.88480102249461,1.,1.37914679719446));
#52303=CARTESIAN_POINT('Ctrl Pts',(-3.87706205830865,1.,1.37976523097187));
#52304=CARTESIAN_POINT('Ctrl Pts',(-3.86932885813403,1.,1.38034709213129));
#52305=CARTESIAN_POINT('Ctrl Pts',(-3.86160143044187,1.,1.38089205993067));
#52306=CARTESIAN_POINT('Ctrl Pts',(-3.85387983979557,1.,1.38139983115075));
#52307=CARTESIAN_POINT('Ctrl Pts',(-3.84616425605705,1.,1.38187013346089));
#52308=CARTESIAN_POINT('Ctrl Pts',(-3.83845502790609,1.,1.38230274828774));
#52309=CARTESIAN_POINT('Ctrl Pts',(-3.83075266982138,1.,1.38269750245086));
#52310=CARTESIAN_POINT('Ctrl Pts',(-3.82305771743715,1.,1.38305421262724));
#52311=CARTESIAN_POINT('Ctrl Pts',(-3.81537060817765,1.,1.38337263902766));
#52312=CARTESIAN_POINT('Ctrl Pts',(-3.80769156398429,1.,1.38365244046226));
#52313=CARTESIAN_POINT('Ctrl Pts',(-3.80002044322169,1.,1.38389311766701));
#52314=CARTESIAN_POINT('Ctrl Pts',(-3.79235669640907,1.,1.38409399694588));
#52315=CARTESIAN_POINT('Ctrl Pts',(-3.78469969805134,1.,1.38425435883773));
#52316=CARTESIAN_POINT('Ctrl Pts',(-3.77704902230441,1.,1.38437354551435));
#52317=CARTESIAN_POINT('Ctrl Pts',(-3.76940473185775,1.,1.38445107339517));
#52318=CARTESIAN_POINT('Ctrl Pts',(-3.76176768271347,1.,1.38448675253343));
#52319=CARTESIAN_POINT('Ctrl Pts',(-3.75413976318727,1.,1.38448077997155));
#52320=CARTESIAN_POINT('Ctrl Pts',(-3.7465231716786,1.,1.38443344984389));
#52321=CARTESIAN_POINT('Ctrl Pts',(-3.73891976418099,1.,1.38434489156456));
#52322=CARTESIAN_POINT('Ctrl Pts',(-3.73133035859283,1.,1.38421479111531));
#52323=CARTESIAN_POINT('Ctrl Pts',(-3.72375409358805,1.,1.3840421342895));
#52324=CARTESIAN_POINT('Ctrl Pts',(-3.7161876605181,1.,1.38382489984585));
#52325=CARTESIAN_POINT('Ctrl Pts',(-3.70862680753343,1.,1.38356065402122));
#52326=CARTESIAN_POINT('Ctrl Pts',(-3.70106792167894,1.,1.38324717612862));
#52327=CARTESIAN_POINT('Ctrl Pts',(-3.69350967899523,1.,1.38288311171649));
#52328=CARTESIAN_POINT('Ctrl Pts',(-3.68595444983844,1.,1.38246852827185));
#52329=CARTESIAN_POINT('Ctrl Pts',(-3.6784103848243,1.,1.38200574290626));
#52330=CARTESIAN_POINT('Ctrl Pts',(-3.67088843112282,1.,1.38149812653876));
#52331=CARTESIAN_POINT('Ctrl Pts',(-3.66339848520874,1.,1.38094856333558));
#52332=CARTESIAN_POINT('Ctrl Pts',(-3.65594554404396,1.,1.38035791051215));
#52333=CARTESIAN_POINT('Ctrl Pts',(-3.64852652756444,1.,1.37972372481598));
#52334=CARTESIAN_POINT('Ctrl Pts',(-3.64112507791112,1.,1.37903818567347));
#52335=CARTESIAN_POINT('Ctrl Pts',(-3.63371727442448,1.,1.37829035457324));
#52336=CARTESIAN_POINT('Ctrl Pts',(-3.62628098665112,1.,1.37746987919868));
#52337=CARTESIAN_POINT('Ctrl Pts',(-3.61880481160408,1.,1.37657053403102));
#52338=CARTESIAN_POINT('Ctrl Pts',(-3.61129546591082,1.,1.37559314436641));
#52339=CARTESIAN_POINT('Ctrl Pts',(-3.60379020124038,1.,1.37455051379642));
#52340=CARTESIAN_POINT('Ctrl Pts',(-3.59634627869117,1.,1.37346320103184));
#52341=CARTESIAN_POINT('Ctrl Pts',(-3.5890185384643,1.,1.37235053661));
#52342=CARTESIAN_POINT('Ctrl Pts',(-3.58183885982745,1.,1.37122241663073));
#52343=CARTESIAN_POINT('Ctrl Pts',(-3.57479875549453,1.,1.37007229485646));
#52344=CARTESIAN_POINT('Ctrl Pts',(-3.56782080304554,1.,1.36886584973349));
#52345=CARTESIAN_POINT('Ctrl Pts',(-3.56077662028492,1.,1.36754771771174));
#52346=CARTESIAN_POINT('Ctrl Pts',(-3.55353883995793,1.,1.36606145456711));
#52347=CARTESIAN_POINT('Ctrl Pts',(-3.54602591832893,1.,1.36436666257567));
#52348=CARTESIAN_POINT('Ctrl Pts',(-3.53824396425032,1.,1.36245507339334));
#52349=CARTESIAN_POINT('Ctrl Pts',(-3.53034464961849,1.,1.36037259643827));
#52350=CARTESIAN_POINT('Ctrl Pts',(-3.52261776117121,1.,1.35821701528975));
#52351=CARTESIAN_POINT('Ctrl Pts',(-3.51542230699919,1.,1.35611275237288));
#52352=CARTESIAN_POINT('Ctrl Pts',(-3.50913227060177,1.,1.35419113576022));
#52353=CARTESIAN_POINT('Ctrl Pts',(-3.50408168106113,1.,1.3525703284343));
#52354=CARTESIAN_POINT('Ctrl Pts',(-3.5007660381658,1.,1.35142377279535));
#52355=CARTESIAN_POINT('Ctrl Pts',(-3.49920025459856,1.,1.35080045218652));
#52356=CARTESIAN_POINT('Ctrl Pts',(-3.49861894124915,1.,1.35049736560633));
#52357=CARTESIAN_POINT('Ctrl Pts',(-3.49847119623841,1.,1.35036670893102));
#52358=CARTESIAN_POINT('Ctrl Pts',(-3.49844575334386,1.,1.35032489087269));
#52359=CARTESIAN_POINT('',(-3.97027773754922,0.,1.36999806084572));
#52360=CARTESIAN_POINT('Ctrl Pts',(-3.62397690409552,-1.,0.96399761336957));
#52361=CARTESIAN_POINT('Ctrl Pts',(-3.62397690409552,1.,0.96399761336957));
#52362=CARTESIAN_POINT('Ctrl Pts',(-3.62393257642191,-1.,0.963922720982576));
#52363=CARTESIAN_POINT('Ctrl Pts',(-3.62393257642191,1.,0.963922720982576));
#52364=CARTESIAN_POINT('Ctrl Pts',(-3.62399933640277,-1.,0.963832486396055));
#52365=CARTESIAN_POINT('Ctrl Pts',(-3.62399933640277,1.,0.963832486396055));
#52366=CARTESIAN_POINT('Ctrl Pts',(-3.62456568607055,-1.,0.963875774532102));
#52367=CARTESIAN_POINT('Ctrl Pts',(-3.62456568607055,1.,0.963875774532102));
#52368=CARTESIAN_POINT('Ctrl Pts',(-3.62625391255277,-1.,0.964291001274618));
#52369=CARTESIAN_POINT('Ctrl Pts',(-3.62625391255277,1.,0.964291001274618));
#52370=CARTESIAN_POINT('Ctrl Pts',(-3.62988252139998,-1.,0.965395153165716));
#52371=CARTESIAN_POINT('Ctrl Pts',(-3.62988252139998,1.,0.965395153165716));
#52372=CARTESIAN_POINT('Ctrl Pts',(-3.6349212208096,-1.,0.967052554540877));
#52373=CARTESIAN_POINT('Ctrl Pts',(-3.6349212208096,1.,0.967052554540877));
#52374=CARTESIAN_POINT('Ctrl Pts',(-3.64113946505393,-1.,0.969195124674829));
#52375=CARTESIAN_POINT('Ctrl Pts',(-3.64113946505393,1.,0.969195124674829));
#52376=CARTESIAN_POINT('Ctrl Pts',(-3.64819756447072,-1.,0.971722122060277));
#52377=CARTESIAN_POINT('Ctrl Pts',(-3.64819756447072,1.,0.971722122060277));
#52378=CARTESIAN_POINT('Ctrl Pts',(-3.6557157673487,-1.,0.974519971354138));
#52379=CARTESIAN_POINT('Ctrl Pts',(-3.6557157673487,1.,0.974519971354138));
#52380=CARTESIAN_POINT('Ctrl Pts',(-3.66333049637403,-1.,0.977478312751416));
#52381=CARTESIAN_POINT('Ctrl Pts',(-3.66333049637403,1.,0.977478312751416));
#52382=CARTESIAN_POINT('Ctrl Pts',(-3.67074983340444,-1.,0.980505922458494));
#52383=CARTESIAN_POINT('Ctrl Pts',(-3.67074983340444,1.,0.980505922458494));
#52384=CARTESIAN_POINT('Ctrl Pts',(-3.67782408841876,-1.,0.983550791470864));
#52385=CARTESIAN_POINT('Ctrl Pts',(-3.67782408841876,1.,0.983550791470864));
#52386=CARTESIAN_POINT('Ctrl Pts',(-3.6845531792623,-1.,0.986602639864285));
#52387=CARTESIAN_POINT('Ctrl Pts',(-3.6845531792623,1.,0.986602639864285));
#52388=CARTESIAN_POINT('Ctrl Pts',(-3.69102682138955,-1.,0.989676715398858));
#52389=CARTESIAN_POINT('Ctrl Pts',(-3.69102682138955,1.,0.989676715398858));
#52390=CARTESIAN_POINT('Ctrl Pts',(-3.69738123415696,-1.,0.992802218332103));
#52391=CARTESIAN_POINT('Ctrl Pts',(-3.69738123415696,1.,0.992802218332103));
#52392=CARTESIAN_POINT('Ctrl Pts',(-3.70375282282107,-1.,0.996009819772431));
#52393=CARTESIAN_POINT('Ctrl Pts',(-3.70375282282107,1.,0.996009819772431));
#52394=CARTESIAN_POINT('Ctrl Pts',(-3.7102243971387,-1.,0.999317260756344));
#52395=CARTESIAN_POINT('Ctrl Pts',(-3.7102243971387,1.,0.999317260756344));
#52396=CARTESIAN_POINT('Ctrl Pts',(-3.71680667125047,-1.,1.00272423396802));
#52397=CARTESIAN_POINT('Ctrl Pts',(-3.71680667125047,1.,1.00272423396802));
#52398=CARTESIAN_POINT('Ctrl Pts',(-3.72346803750544,-1.,1.00622000735696));
#52399=CARTESIAN_POINT('Ctrl Pts',(-3.72346803750544,1.,1.00622000735696));
#52400=CARTESIAN_POINT('Ctrl Pts',(-3.73015276704407,-1.,1.00978798539491));
#52401=CARTESIAN_POINT('Ctrl Pts',(-3.73015276704407,1.,1.00978798539491));
#52402=CARTESIAN_POINT('Ctrl Pts',(-3.73680245055747,-1.,1.01341114319906));
#52403=CARTESIAN_POINT('Ctrl Pts',(-3.73680245055747,1.,1.01341114319906));
#52404=CARTESIAN_POINT('Ctrl Pts',(-3.74337942504993,-1.,1.01707794311088));
#52405=CARTESIAN_POINT('Ctrl Pts',(-3.74337942504993,1.,1.01707794311088));
#52406=CARTESIAN_POINT('Ctrl Pts',(-3.74987777155873,-1.,1.02078510487439));
#52407=CARTESIAN_POINT('Ctrl Pts',(-3.74987777155873,1.,1.02078510487439));
#52408=CARTESIAN_POINT('Ctrl Pts',(-3.75631037456224,-1.,1.02453429444668));
#52409=CARTESIAN_POINT('Ctrl Pts',(-3.75631037456224,1.,1.02453429444668));
#52410=CARTESIAN_POINT('Ctrl Pts',(-3.76270122291245,-1.,1.02833014458184));
#52411=CARTESIAN_POINT('Ctrl Pts',(-3.76270122291245,1.,1.02833014458184));
#52412=CARTESIAN_POINT('Ctrl Pts',(-3.76907609832516,-1.,1.03217786604919));
#52413=CARTESIAN_POINT('Ctrl Pts',(-3.76907609832516,1.,1.03217786604919));
#52414=CARTESIAN_POINT('Ctrl Pts',(-3.77545283140427,-1.,1.03608074678008));
#52415=CARTESIAN_POINT('Ctrl Pts',(-3.77545283140427,1.,1.03608074678008));
#52416=CARTESIAN_POINT('Ctrl Pts',(-3.7818353500817,-1.,1.04003862055798));
#52417=CARTESIAN_POINT('Ctrl Pts',(-3.7818353500817,1.,1.04003862055798));
#52418=CARTESIAN_POINT('Ctrl Pts',(-3.78821910787179,-1.,1.04404924374422));
#52419=CARTESIAN_POINT('Ctrl Pts',(-3.78821910787179,1.,1.04404924374422));
#52420=CARTESIAN_POINT('Ctrl Pts',(-3.79459440308786,-1.,1.04810913267639));
#52421=CARTESIAN_POINT('Ctrl Pts',(-3.79459440308786,1.,1.04810913267639));
#52422=CARTESIAN_POINT('Ctrl Pts',(-3.80095039790681,-1.,1.05221457990016));
#52423=CARTESIAN_POINT('Ctrl Pts',(-3.80095039790681,1.,1.05221457990016));
#52424=CARTESIAN_POINT('Ctrl Pts',(-3.80727913637791,-1.,1.05636266918644));
#52425=CARTESIAN_POINT('Ctrl Pts',(-3.80727913637791,1.,1.05636266918644));
#52426=CARTESIAN_POINT('Ctrl Pts',(-3.8135786611749,-1.,1.06055206187299));
#52427=CARTESIAN_POINT('Ctrl Pts',(-3.8135786611749,1.,1.06055206187299));
#52428=CARTESIAN_POINT('Ctrl Pts',(-3.81985083953012,-1.,1.0647824403893));
#52429=CARTESIAN_POINT('Ctrl Pts',(-3.81985083953012,1.,1.0647824403893));
#52430=CARTESIAN_POINT('Ctrl Pts',(-3.82609989967276,-1.,1.06905413180359));
#52431=CARTESIAN_POINT('Ctrl Pts',(-3.82609989967276,1.,1.06905413180359));
#52432=CARTESIAN_POINT('Ctrl Pts',(-3.83233071195144,-1.,1.07336766633459));
#52433=CARTESIAN_POINT('Ctrl Pts',(-3.83233071195144,1.,1.07336766633459));
#52434=CARTESIAN_POINT('Ctrl Pts',(-3.83854714117491,-1.,1.07772335353858));
#52435=CARTESIAN_POINT('Ctrl Pts',(-3.83854714117491,1.,1.07772335353858));
#52436=CARTESIAN_POINT('Ctrl Pts',(-3.8447504803063,-1.,1.08212087917991));
#52437=CARTESIAN_POINT('Ctrl Pts',(-3.8447504803063,1.,1.08212087917991));
#52438=CARTESIAN_POINT('Ctrl Pts',(-3.85094025222713,-1.,1.08655950846384));
#52439=CARTESIAN_POINT('Ctrl Pts',(-3.85094025222713,1.,1.08655950846384));
#52440=CARTESIAN_POINT('Ctrl Pts',(-3.85711487933931,-1.,1.09103825516294));
#52441=CARTESIAN_POINT('Ctrl Pts',(-3.85711487933931,1.,1.09103825516294));
#52442=CARTESIAN_POINT('Ctrl Pts',(-3.86327241021247,-1.,1.09555606505013));
#52443=CARTESIAN_POINT('Ctrl Pts',(-3.86327241021247,1.,1.09555606505013));
#52444=CARTESIAN_POINT('Ctrl Pts',(-3.86941120134849,-1.,1.10011198761195));
#52445=CARTESIAN_POINT('Ctrl Pts',(-3.86941120134849,1.,1.10011198761195));
#52446=CARTESIAN_POINT('Ctrl Pts',(-3.87553067187514,-1.,1.10470536603287));
#52447=CARTESIAN_POINT('Ctrl Pts',(-3.87553067187514,1.,1.10470536603287));
#52448=CARTESIAN_POINT('Ctrl Pts',(-3.88163105531724,-1.,1.10933577224008));
#52449=CARTESIAN_POINT('Ctrl Pts',(-3.88163105531724,1.,1.10933577224008));
#52450=CARTESIAN_POINT('Ctrl Pts',(-3.88771308285171,-1.,1.11400292434429));
#52451=CARTESIAN_POINT('Ctrl Pts',(-3.88771308285171,1.,1.11400292434429));
#52452=CARTESIAN_POINT('Ctrl Pts',(-3.89377768340344,-1.,1.11870660794603));
#52453=CARTESIAN_POINT('Ctrl Pts',(-3.89377768340344,1.,1.11870660794603));
#52454=CARTESIAN_POINT('Ctrl Pts',(-3.89982569750025,-1.,1.12344660099043));
#52455=CARTESIAN_POINT('Ctrl Pts',(-3.89982569750025,1.,1.12344660099043));
#52456=CARTESIAN_POINT('Ctrl Pts',(-3.90585753318737,-1.,1.12822258281553));
#52457=CARTESIAN_POINT('Ctrl Pts',(-3.90585753318737,1.,1.12822258281553));
#52458=CARTESIAN_POINT('Ctrl Pts',(-3.91187321145649,-1.,1.13303414693896));
#52459=CARTESIAN_POINT('Ctrl Pts',(-3.91187321145649,1.,1.13303414693896));
#52460=CARTESIAN_POINT('Ctrl Pts',(-3.91787251936827,-1.,1.13788084225554));
#52461=CARTESIAN_POINT('Ctrl Pts',(-3.91787251936827,1.,1.13788084225554));
#52462=CARTESIAN_POINT('Ctrl Pts',(-3.92385513133997,-1.,1.14276220561593));
#52463=CARTESIAN_POINT('Ctrl Pts',(-3.92385513133997,1.,1.14276220561593));
#52464=CARTESIAN_POINT('Ctrl Pts',(-3.92982073294257,-1.,1.14767779451123));
#52465=CARTESIAN_POINT('Ctrl Pts',(-3.92982073294257,1.,1.14767779451123));
#52466=CARTESIAN_POINT('Ctrl Pts',(-3.9357691705628,-1.,1.1526272271632));
#52467=CARTESIAN_POINT('Ctrl Pts',(-3.9357691705628,1.,1.1526272271632));
#52468=CARTESIAN_POINT('Ctrl Pts',(-3.94170046685203,-1.,1.15761018340956));
#52469=CARTESIAN_POINT('Ctrl Pts',(-3.94170046685203,1.,1.15761018340956));
#52470=CARTESIAN_POINT('Ctrl Pts',(-3.94761474780583,-1.,1.16262637999157));
#52471=CARTESIAN_POINT('Ctrl Pts',(-3.94761474780583,1.,1.16262637999157));
#52472=CARTESIAN_POINT('Ctrl Pts',(-3.95351219509876,-1.,1.16767555244438));
#52473=CARTESIAN_POINT('Ctrl Pts',(-3.95351219509876,1.,1.16767555244438));
#52474=CARTESIAN_POINT('Ctrl Pts',(-3.95939299213276,-1.,1.17275743590361));
#52475=CARTESIAN_POINT('Ctrl Pts',(-3.95939299213276,1.,1.17275743590361));
#52476=CARTESIAN_POINT('Ctrl Pts',(-3.96525726358159,-1.,1.17787174135592));
#52477=CARTESIAN_POINT('Ctrl Pts',(-3.96525726358159,1.,1.17787174135592));
#52478=CARTESIAN_POINT('Ctrl Pts',(-3.97110505165415,-1.,1.18301815039831));
#52479=CARTESIAN_POINT('Ctrl Pts',(-3.97110505165415,1.,1.18301815039831));
#52480=CARTESIAN_POINT('Ctrl Pts',(-3.97693634767754,-1.,1.18819633715539));
#52481=CARTESIAN_POINT('Ctrl Pts',(-3.97693634767754,1.,1.18819633715539));
#52482=CARTESIAN_POINT('Ctrl Pts',(-3.98275111052561,-1.,1.19340598349475));
#52483=CARTESIAN_POINT('Ctrl Pts',(-3.98275111052561,1.,1.19340598349475));
#52484=CARTESIAN_POINT('Ctrl Pts',(-3.98854928957189,-1.,1.19864679609566));
#52485=CARTESIAN_POINT('Ctrl Pts',(-3.98854928957189,1.,1.19864679609566));
#52486=CARTESIAN_POINT('Ctrl Pts',(-3.99433084799666,-1.,1.20391852375139));
#52487=CARTESIAN_POINT('Ctrl Pts',(-3.99433084799666,1.,1.20391852375139));
#52488=CARTESIAN_POINT('Ctrl Pts',(-4.00009577950721,-1.,1.20922097029551));
#52489=CARTESIAN_POINT('Ctrl Pts',(-4.00009577950721,1.,1.20922097029551));
#52490=CARTESIAN_POINT('Ctrl Pts',(-4.00584409522722,-1.,1.21455398918133));
#52491=CARTESIAN_POINT('Ctrl Pts',(-4.00584409522722,1.,1.21455398918133));
#52492=CARTESIAN_POINT('Ctrl Pts',(-4.01042947140789,-1.,1.21884478244403));
#52493=CARTESIAN_POINT('Ctrl Pts',(-4.01042947140789,1.,1.21884478244403));
#52494=CARTESIAN_POINT('Ctrl Pts',(-4.01386104433519,-1.,1.22207656455845));
#52495=CARTESIAN_POINT('Ctrl Pts',(-4.01386104433519,1.,1.22207656455845));
#52496=CARTESIAN_POINT('Ctrl Pts',(-4.01614544569895,-1.,1.22423716681317));
#52497=CARTESIAN_POINT('Ctrl Pts',(-4.01614544569895,1.,1.22423716681317));
#52498=CARTESIAN_POINT('Ctrl Pts',(-4.01728681790024,-1.,1.22531898815164));
#52499=CARTESIAN_POINT('Ctrl Pts',(-4.01728681790024,1.,1.22531898815164));
#52500=CARTESIAN_POINT('',(-3.62400312501199,1.,0.963899035118986));
#52501=CARTESIAN_POINT('Ctrl Pts',(-3.62400312501199,-1.,0.963899035118986));
#52502=CARTESIAN_POINT('Ctrl Pts',(-3.62400312501199,-0.666666666666667,
0.963899035118986));
#52503=CARTESIAN_POINT('Ctrl Pts',(-3.62400312501199,-0.333333333333333,
0.963899035118986));
#52504=CARTESIAN_POINT('Ctrl Pts',(-3.62400312501199,0.333333333333333,
0.963899035118986));
#52505=CARTESIAN_POINT('Ctrl Pts',(-3.62400312501199,0.666666666666667,
0.963899035118985));
#52506=CARTESIAN_POINT('Ctrl Pts',(-3.62400312501199,1.,0.963899035118985));
#52507=CARTESIAN_POINT('',(-4.01728681790024,1.,1.22531898815164));
#52508=CARTESIAN_POINT('',(-4.01728681790024,0.,1.22531898815164));
#52509=CARTESIAN_POINT('Ctrl Pts',(-3.62400312501199,1.,0.963899035118985));
#52510=CARTESIAN_POINT('Ctrl Pts',(-3.62404828878374,1.,0.963880158556713));
#52511=CARTESIAN_POINT('Ctrl Pts',(-3.62424461507455,1.,0.963861297423579));
#52512=CARTESIAN_POINT('Ctrl Pts',(-3.62489305727516,1.,0.963957782642589));
#52513=CARTESIAN_POINT('Ctrl Pts',(-3.62652618145252,1.,0.964373850166081));
#52514=CARTESIAN_POINT('Ctrl Pts',(-3.62988252139998,1.,0.965395153165716));
#52515=CARTESIAN_POINT('Ctrl Pts',(-3.6349212208096,1.,0.967052554540877));
#52516=CARTESIAN_POINT('Ctrl Pts',(-3.64113946505393,1.,0.969195124674829));
#52517=CARTESIAN_POINT('Ctrl Pts',(-3.64819756447072,1.,0.971722122060277));
#52518=CARTESIAN_POINT('Ctrl Pts',(-3.6557157673487,1.,0.974519971354138));
#52519=CARTESIAN_POINT('Ctrl Pts',(-3.66333049637403,1.,0.977478312751416));
#52520=CARTESIAN_POINT('Ctrl Pts',(-3.67074983340444,1.,0.980505922458494));
#52521=CARTESIAN_POINT('Ctrl Pts',(-3.67782408841876,1.,0.983550791470864));
#52522=CARTESIAN_POINT('Ctrl Pts',(-3.6845531792623,1.,0.986602639864285));
#52523=CARTESIAN_POINT('Ctrl Pts',(-3.69102682138955,1.,0.989676715398858));
#52524=CARTESIAN_POINT('Ctrl Pts',(-3.69738123415696,1.,0.992802218332103));
#52525=CARTESIAN_POINT('Ctrl Pts',(-3.70375282282107,1.,0.996009819772431));
#52526=CARTESIAN_POINT('Ctrl Pts',(-3.7102243971387,1.,0.999317260756344));
#52527=CARTESIAN_POINT('Ctrl Pts',(-3.71680667125047,1.,1.00272423396802));
#52528=CARTESIAN_POINT('Ctrl Pts',(-3.72346803750544,1.,1.00622000735696));
#52529=CARTESIAN_POINT('Ctrl Pts',(-3.73015276704407,1.,1.00978798539491));
#52530=CARTESIAN_POINT('Ctrl Pts',(-3.73680245055747,1.,1.01341114319906));
#52531=CARTESIAN_POINT('Ctrl Pts',(-3.74337942504993,1.,1.01707794311088));
#52532=CARTESIAN_POINT('Ctrl Pts',(-3.74987777155873,1.,1.02078510487439));
#52533=CARTESIAN_POINT('Ctrl Pts',(-3.75631037456224,1.,1.02453429444668));
#52534=CARTESIAN_POINT('Ctrl Pts',(-3.76270122291245,1.,1.02833014458184));
#52535=CARTESIAN_POINT('Ctrl Pts',(-3.76907609832516,1.,1.03217786604919));
#52536=CARTESIAN_POINT('Ctrl Pts',(-3.77545283140427,1.,1.03608074678008));
#52537=CARTESIAN_POINT('Ctrl Pts',(-3.7818353500817,1.,1.04003862055798));
#52538=CARTESIAN_POINT('Ctrl Pts',(-3.78821910787179,1.,1.04404924374422));
#52539=CARTESIAN_POINT('Ctrl Pts',(-3.79459440308786,1.,1.04810913267639));
#52540=CARTESIAN_POINT('Ctrl Pts',(-3.80095039790681,1.,1.05221457990016));
#52541=CARTESIAN_POINT('Ctrl Pts',(-3.80727913637791,1.,1.05636266918644));
#52542=CARTESIAN_POINT('Ctrl Pts',(-3.8135786611749,1.,1.06055206187299));
#52543=CARTESIAN_POINT('Ctrl Pts',(-3.81985083953012,1.,1.0647824403893));
#52544=CARTESIAN_POINT('Ctrl Pts',(-3.82609989967276,1.,1.06905413180359));
#52545=CARTESIAN_POINT('Ctrl Pts',(-3.83233071195144,1.,1.07336766633459));
#52546=CARTESIAN_POINT('Ctrl Pts',(-3.83854714117491,1.,1.07772335353858));
#52547=CARTESIAN_POINT('Ctrl Pts',(-3.8447504803063,1.,1.08212087917991));
#52548=CARTESIAN_POINT('Ctrl Pts',(-3.85094025222713,1.,1.08655950846384));
#52549=CARTESIAN_POINT('Ctrl Pts',(-3.85711487933931,1.,1.09103825516294));
#52550=CARTESIAN_POINT('Ctrl Pts',(-3.86327241021247,1.,1.09555606505013));
#52551=CARTESIAN_POINT('Ctrl Pts',(-3.86941120134849,1.,1.10011198761195));
#52552=CARTESIAN_POINT('Ctrl Pts',(-3.87553067187514,1.,1.10470536603287));
#52553=CARTESIAN_POINT('Ctrl Pts',(-3.88163105531724,1.,1.10933577224008));
#52554=CARTESIAN_POINT('Ctrl Pts',(-3.88771308285171,1.,1.11400292434429));
#52555=CARTESIAN_POINT('Ctrl Pts',(-3.89377768340344,1.,1.11870660794603));
#52556=CARTESIAN_POINT('Ctrl Pts',(-3.89982569750025,1.,1.12344660099043));
#52557=CARTESIAN_POINT('Ctrl Pts',(-3.90585753318737,1.,1.12822258281553));
#52558=CARTESIAN_POINT('Ctrl Pts',(-3.91187321145649,1.,1.13303414693896));
#52559=CARTESIAN_POINT('Ctrl Pts',(-3.91787251936827,1.,1.13788084225554));
#52560=CARTESIAN_POINT('Ctrl Pts',(-3.92385513133997,1.,1.14276220561593));
#52561=CARTESIAN_POINT('Ctrl Pts',(-3.92982073294257,1.,1.14767779451123));
#52562=CARTESIAN_POINT('Ctrl Pts',(-3.9357691705628,1.,1.1526272271632));
#52563=CARTESIAN_POINT('Ctrl Pts',(-3.94170046685203,1.,1.15761018340956));
#52564=CARTESIAN_POINT('Ctrl Pts',(-3.94761474780583,1.,1.16262637999157));
#52565=CARTESIAN_POINT('Ctrl Pts',(-3.95351219509876,1.,1.16767555244438));
#52566=CARTESIAN_POINT('Ctrl Pts',(-3.95939299213276,1.,1.17275743590361));
#52567=CARTESIAN_POINT('Ctrl Pts',(-3.96525726358159,1.,1.17787174135592));
#52568=CARTESIAN_POINT('Ctrl Pts',(-3.97110505165415,1.,1.18301815039831));
#52569=CARTESIAN_POINT('Ctrl Pts',(-3.97693634767754,1.,1.18819633715539));
#52570=CARTESIAN_POINT('Ctrl Pts',(-3.98275111052561,1.,1.19340598349475));
#52571=CARTESIAN_POINT('Ctrl Pts',(-3.98854928957189,1.,1.19864679609566));
#52572=CARTESIAN_POINT('Ctrl Pts',(-3.99433084799666,1.,1.20391852375139));
#52573=CARTESIAN_POINT('Ctrl Pts',(-4.00009577950721,1.,1.20922097029551));
#52574=CARTESIAN_POINT('Ctrl Pts',(-4.00584409522722,1.,1.21455398918133));
#52575=CARTESIAN_POINT('Ctrl Pts',(-4.01042947140789,1.,1.21884478244403));
#52576=CARTESIAN_POINT('Ctrl Pts',(-4.01386104433519,1.,1.22207656455845));
#52577=CARTESIAN_POINT('Ctrl Pts',(-4.01614544569895,1.,1.22423716681317));
#52578=CARTESIAN_POINT('Ctrl Pts',(-4.01728681790024,1.,1.22531898815164));
#52579=CARTESIAN_POINT('Origin',(-4.01728681790024,0.,1.22531898815164));
#52580=CARTESIAN_POINT('',(-3.97027773754922,1.,1.36999806084572));
#52581=CARTESIAN_POINT('Origin',(0.,0.,0.));
#52582=CARTESIAN_POINT('',(-3.66661143271648,1.,0.786422660833743));
#52583=CARTESIAN_POINT('Origin',(0.,1.,0.));
#52584=CARTESIAN_POINT('Ctrl Pts',(-3.66661143271648,1.,0.786422660833743));
#52585=CARTESIAN_POINT('Ctrl Pts',(-3.66661143271648,0.666666666666667,
0.786422660833743));
#52586=CARTESIAN_POINT('Ctrl Pts',(-3.66661143271648,0.333333333333333,
0.786422660833743));
#52587=CARTESIAN_POINT('Ctrl Pts',(-3.66661143271648,-0.333333333333333,
0.786422660833743));
#52588=CARTESIAN_POINT('Ctrl Pts',(-3.66661143271648,-0.666666666666667,
0.786422660833743));
#52589=CARTESIAN_POINT('Ctrl Pts',(-3.66661143271648,-1.,0.786422660833743));
#52590=CARTESIAN_POINT('Ctrl Pts',(-4.13571194405636,-1.,0.732042837400619));
#52591=CARTESIAN_POINT('Ctrl Pts',(-4.13571194405636,1.,0.732042837400619));
#52592=CARTESIAN_POINT('Ctrl Pts',(-4.13420383737278,-1.,0.732488575135926));
#52593=CARTESIAN_POINT('Ctrl Pts',(-4.13420383737278,1.,0.732488575135926));
#52594=CARTESIAN_POINT('Ctrl Pts',(-4.13118752796397,-1.,0.733376589325634));
#52595=CARTESIAN_POINT('Ctrl Pts',(-4.13118752796397,1.,0.733376589325634));
#52596=CARTESIAN_POINT('Ctrl Pts',(-4.12666277572794,-1.,0.734698226767512));
#52597=CARTESIAN_POINT('Ctrl Pts',(-4.12666277572794,1.,0.734698226767512));
#52598=CARTESIAN_POINT('Ctrl Pts',(-4.12062919626082,-1.,0.736439634335347));
#52599=CARTESIAN_POINT('Ctrl Pts',(-4.12062919626082,1.,0.736439634335347));
#52600=CARTESIAN_POINT('Ctrl Pts',(-4.11308626953795,-1.,0.738581708229118));
#52601=CARTESIAN_POINT('Ctrl Pts',(-4.11308626953795,1.,0.738581708229118));
#52602=CARTESIAN_POINT('Ctrl Pts',(-4.1055424175856,-1.,0.740688998555151));
#52603=CARTESIAN_POINT('Ctrl Pts',(-4.1055424175856,1.,0.740688998555151));
#52604=CARTESIAN_POINT('Ctrl Pts',(-4.09799769702712,-1.,0.742761369690017));
#52605=CARTESIAN_POINT('Ctrl Pts',(-4.09799769702712,1.,0.742761369690017));
#52606=CARTESIAN_POINT('Ctrl Pts',(-4.09045220253011,-1.,0.744798649705514));
#52607=CARTESIAN_POINT('Ctrl Pts',(-4.09045220253011,1.,0.744798649705514));
#52608=CARTESIAN_POINT('Ctrl Pts',(-4.08290608094789,-1.,0.746800631490821));
#52609=CARTESIAN_POINT('Ctrl Pts',(-4.08290608094789,1.,0.746800631490821));
#52610=CARTESIAN_POINT('Ctrl Pts',(-4.07535951055363,-1.,0.748767076679177));
#52611=CARTESIAN_POINT('Ctrl Pts',(-4.07535951055363,1.,0.748767076679177));
#52612=CARTESIAN_POINT('Ctrl Pts',(-4.06781267241886,-1.,0.750697720483175));
#52613=CARTESIAN_POINT('Ctrl Pts',(-4.06781267241886,1.,0.750697720483175));
#52614=CARTESIAN_POINT('Ctrl Pts',(-4.06026572221399,-1.,0.752592276482869));
#52615=CARTESIAN_POINT('Ctrl Pts',(-4.06026572221399,1.,0.752592276482869));
#52616=CARTESIAN_POINT('Ctrl Pts',(-4.05271876688106,-1.,0.754450441816411));
#52617=CARTESIAN_POINT('Ctrl Pts',(-4.05271876688106,1.,0.754450441816411));
#52618=CARTESIAN_POINT('Ctrl Pts',(-4.04517182654344,-1.,0.756271902370186));
#52619=CARTESIAN_POINT('Ctrl Pts',(-4.04517182654344,1.,0.756271902370186));
#52620=CARTESIAN_POINT('Ctrl Pts',(-4.03762485803468,-1.,0.758056338885553));
#52621=CARTESIAN_POINT('Ctrl Pts',(-4.03762485803468,1.,0.758056338885553));
#52622=CARTESIAN_POINT('Ctrl Pts',(-4.0300778195465,-1.,0.759803433244166));
#52623=CARTESIAN_POINT('Ctrl Pts',(-4.0300778195465,1.,0.759803433244166));
#52624=CARTESIAN_POINT('Ctrl Pts',(-4.02253072741347,-1.,0.761512875859941));
#52625=CARTESIAN_POINT('Ctrl Pts',(-4.02253072741347,1.,0.761512875859941));
#52626=CARTESIAN_POINT('Ctrl Pts',(-4.01498370680434,-1.,0.763184371182826));
#52627=CARTESIAN_POINT('Ctrl Pts',(-4.01498370680434,1.,0.763184371182826));
#52628=CARTESIAN_POINT('Ctrl Pts',(-4.00743706791366,-1.,0.764817648784946));
#52629=CARTESIAN_POINT('Ctrl Pts',(-4.00743706791366,1.,0.764817648784946));
#52630=CARTESIAN_POINT('Ctrl Pts',(-3.99989129179464,-1.,0.766412457135785));
#52631=CARTESIAN_POINT('Ctrl Pts',(-3.99989129179464,1.,0.766412457135785));
#52632=CARTESIAN_POINT('Ctrl Pts',(-3.99234687880892,-1.,0.767968531377708));
#52633=CARTESIAN_POINT('Ctrl Pts',(-3.99234687880892,1.,0.767968531377708));
#52634=CARTESIAN_POINT('Ctrl Pts',(-3.98480422348403,-1.,0.769485566245459));
#52635=CARTESIAN_POINT('Ctrl Pts',(-3.98480422348403,1.,0.769485566245459));
#52636=CARTESIAN_POINT('Ctrl Pts',(-3.97726349165507,-1.,0.770963190030503));
#52637=CARTESIAN_POINT('Ctrl Pts',(-3.97726349165507,1.,0.770963190030503));
#52638=CARTESIAN_POINT('Ctrl Pts',(-3.96972446532832,-1.,0.772400931772238));
#52639=CARTESIAN_POINT('Ctrl Pts',(-3.96972446532832,1.,0.772400931772238));
#52640=CARTESIAN_POINT('Ctrl Pts',(-3.96218649639876,-1.,0.773798212026682));
#52641=CARTESIAN_POINT('Ctrl Pts',(-3.96218649639876,1.,0.773798212026682));
#52642=CARTESIAN_POINT('Ctrl Pts',(-3.95464885452364,-1.,0.775154418039441));
#52643=CARTESIAN_POINT('Ctrl Pts',(-3.95464885452364,1.,0.775154418039441));
#52644=CARTESIAN_POINT('Ctrl Pts',(-3.94711101619471,-1.,0.77646896669796));
#52645=CARTESIAN_POINT('Ctrl Pts',(-3.94711101619471,1.,0.77646896669796));
#52646=CARTESIAN_POINT('Ctrl Pts',(-3.93957296768098,-1.,0.777741370568549));
#52647=CARTESIAN_POINT('Ctrl Pts',(-3.93957296768098,1.,0.777741370568549));
#52648=CARTESIAN_POINT('Ctrl Pts',(-3.93203552473153,-1.,0.778971308134786));
#52649=CARTESIAN_POINT('Ctrl Pts',(-3.93203552473153,1.,0.778971308134786));
#52650=CARTESIAN_POINT('Ctrl Pts',(-3.92450058323799,-1.,0.780158678615506));
#52651=CARTESIAN_POINT('Ctrl Pts',(-3.92450058323799,1.,0.780158678615506));
#52652=CARTESIAN_POINT('Ctrl Pts',(-3.9169703605466,-1.,0.781303428618343));
#52653=CARTESIAN_POINT('Ctrl Pts',(-3.9169703605466,1.,0.781303428618343));
#52654=CARTESIAN_POINT('Ctrl Pts',(-3.90944671004536,-1.,0.782405395622758));
#52655=CARTESIAN_POINT('Ctrl Pts',(-3.90944671004536,1.,0.782405395622758));
#52656=CARTESIAN_POINT('Ctrl Pts',(-3.90193039043971,-1.,0.783464141529082));
#52657=CARTESIAN_POINT('Ctrl Pts',(-3.90193039043971,1.,0.783464141529082));
#52658=CARTESIAN_POINT('Ctrl Pts',(-3.89442039235105,-1.,0.784478799358335));
#52659=CARTESIAN_POINT('Ctrl Pts',(-3.89442039235105,1.,0.784478799358335));
#52660=CARTESIAN_POINT('Ctrl Pts',(-3.88691313167399,-1.,0.785447890340723));
#52661=CARTESIAN_POINT('Ctrl Pts',(-3.88691313167399,1.,0.785447890340723));
#52662=CARTESIAN_POINT('Ctrl Pts',(-3.87940402818186,-1.,0.786369675812592));
#52663=CARTESIAN_POINT('Ctrl Pts',(-3.87940402818186,1.,0.786369675812592));
#52664=CARTESIAN_POINT('Ctrl Pts',(-3.87188916600905,-1.,0.78724252761798));
#52665=CARTESIAN_POINT('Ctrl Pts',(-3.87188916600905,1.,0.78724252761798));
#52666=CARTESIAN_POINT('Ctrl Pts',(-3.86436702561342,-1.,0.788065315093771));
#52667=CARTESIAN_POINT('Ctrl Pts',(-3.86436702561342,1.,0.788065315093771));
#52668=CARTESIAN_POINT('Ctrl Pts',(-3.85683995872536,-1.,0.788837734090688));
#52669=CARTESIAN_POINT('Ctrl Pts',(-3.85683995872536,1.,0.788837734090688));
#52670=CARTESIAN_POINT('Ctrl Pts',(-3.8493163780891,-1.,0.789560798155618));
#52671=CARTESIAN_POINT('Ctrl Pts',(-3.8493163780891,1.,0.789560798155618));
#52672=CARTESIAN_POINT('Ctrl Pts',(-3.84180762342476,-1.,0.790236124191289));
#52673=CARTESIAN_POINT('Ctrl Pts',(-3.84180762342476,1.,0.790236124191289));
#52674=CARTESIAN_POINT('Ctrl Pts',(-3.83432392054804,-1.,0.79086501270534));
#52675=CARTESIAN_POINT('Ctrl Pts',(-3.83432392054804,1.,0.79086501270534));
#52676=CARTESIAN_POINT('Ctrl Pts',(-3.82687033899799,-1.,0.791447528662381));
#52677=CARTESIAN_POINT('Ctrl Pts',(-3.82687033899799,1.,0.791447528662381));
#52678=CARTESIAN_POINT('Ctrl Pts',(-3.81944345442237,-1.,0.791981740718606));
#52679=CARTESIAN_POINT('Ctrl Pts',(-3.81944345442237,1.,0.791981740718606));
#52680=CARTESIAN_POINT('Ctrl Pts',(-3.81202588694726,-1.,0.792462483517568));
#52681=CARTESIAN_POINT('Ctrl Pts',(-3.81202588694726,1.,0.792462483517568));
#52682=CARTESIAN_POINT('Ctrl Pts',(-3.80459229925598,-1.,0.792882695234693));
#52683=CARTESIAN_POINT('Ctrl Pts',(-3.80459229925598,1.,0.792882695234693));
#52684=CARTESIAN_POINT('Ctrl Pts',(-3.79711921389862,-1.,0.7932356129732));
#52685=CARTESIAN_POINT('Ctrl Pts',(-3.79711921389862,1.,0.7932356129732));
#52686=CARTESIAN_POINT('Ctrl Pts',(-3.78959439439222,-1.,0.793516871680966));
#52687=CARTESIAN_POINT('Ctrl Pts',(-3.78959439439222,1.,0.793516871680966));
#52688=CARTESIAN_POINT('Ctrl Pts',(-3.78202460377617,-1.,0.793726235781339));
#52689=CARTESIAN_POINT('Ctrl Pts',(-3.78202460377617,1.,0.793726235781339));
#52690=CARTESIAN_POINT('Ctrl Pts',(-3.77444863801264,-1.,0.793870523787515));
#52691=CARTESIAN_POINT('Ctrl Pts',(-3.77444863801264,1.,0.793870523787515));
#52692=CARTESIAN_POINT('Ctrl Pts',(-3.76692626931184,-1.,0.793961083689141));
#52693=CARTESIAN_POINT('Ctrl Pts',(-3.76692626931184,1.,0.793961083689141));
#52694=CARTESIAN_POINT('Ctrl Pts',(-3.75951468666325,-1.,0.794008429135047));
#52695=CARTESIAN_POINT('Ctrl Pts',(-3.75951468666325,1.,0.794008429135047));
#52696=CARTESIAN_POINT('Ctrl Pts',(-3.75224692493895,-1.,0.79401734737144));
#52697=CARTESIAN_POINT('Ctrl Pts',(-3.75224692493895,1.,0.79401734737144));
#52698=CARTESIAN_POINT('Ctrl Pts',(-3.74511357728827,-1.,0.79398270045988));
#52699=CARTESIAN_POINT('Ctrl Pts',(-3.74511357728827,1.,0.79398270045988));
#52700=CARTESIAN_POINT('Ctrl Pts',(-3.73803280541576,-1.,0.79388270093679));
#52701=CARTESIAN_POINT('Ctrl Pts',(-3.73803280541576,1.,0.79388270093679));
#52702=CARTESIAN_POINT('Ctrl Pts',(-3.7308691469564,-1.,0.793682750269347));
#52703=CARTESIAN_POINT('Ctrl Pts',(-3.7308691469564,1.,0.793682750269347));
#52704=CARTESIAN_POINT('Ctrl Pts',(-3.7234879729357,-1.,0.79334702378387));
#52705=CARTESIAN_POINT('Ctrl Pts',(-3.7234879729357,1.,0.79334702378387));
#52706=CARTESIAN_POINT('Ctrl Pts',(-3.7158024239604,-1.,0.792848377370115));
#52707=CARTESIAN_POINT('Ctrl Pts',(-3.7158024239604,1.,0.792848377370115));
#52708=CARTESIAN_POINT('Ctrl Pts',(-3.70781724021879,-1.,0.792177688845967));
#52709=CARTESIAN_POINT('Ctrl Pts',(-3.70781724021879,1.,0.792177688845967));
#52710=CARTESIAN_POINT('Ctrl Pts',(-3.69968940808982,-1.,0.791356575696509));
#52711=CARTESIAN_POINT('Ctrl Pts',(-3.69968940808982,1.,0.791356575696509));
#52712=CARTESIAN_POINT('Ctrl Pts',(-3.69172044327754,-1.,0.79043628498958));
#52713=CARTESIAN_POINT('Ctrl Pts',(-3.69172044327754,1.,0.79043628498958));
#52714=CARTESIAN_POINT('Ctrl Pts',(-3.68428439784285,-1.,0.789483546065158));
#52715=CARTESIAN_POINT('Ctrl Pts',(-3.68428439784285,1.,0.789483546065158));
#52716=CARTESIAN_POINT('Ctrl Pts',(-3.67777119516438,-1.,0.788569566220662));
#52717=CARTESIAN_POINT('Ctrl Pts',(-3.67777119516438,1.,0.788569566220662));
#52718=CARTESIAN_POINT('Ctrl Pts',(-3.672529236635,-1.,0.787758799995426));
#52719=CARTESIAN_POINT('Ctrl Pts',(-3.672529236635,1.,0.787758799995426));
#52720=CARTESIAN_POINT('Ctrl Pts',(-3.66879484800625,-1.,0.787095252589507));
#52721=CARTESIAN_POINT('Ctrl Pts',(-3.66879484800625,1.,0.787095252589507));
#52722=CARTESIAN_POINT('Ctrl Pts',(-3.66710211819938,-1.,0.786698783541657));
#52723=CARTESIAN_POINT('Ctrl Pts',(-3.66710211819938,1.,0.786698783541657));
#52724=CARTESIAN_POINT('Ctrl Pts',(-3.66657784454965,-1.,0.786480236184947));
#52725=CARTESIAN_POINT('Ctrl Pts',(-3.66657784454965,1.,0.786480236184947));
#52726=CARTESIAN_POINT('Ctrl Pts',(-3.66655932661846,-1.,0.786369528183039));
#52727=CARTESIAN_POINT('Ctrl Pts',(-3.66655932661846,1.,0.786369528183039));
#52728=CARTESIAN_POINT('Ctrl Pts',(-3.66663282329846,-1.,0.786322922920599));
#52729=CARTESIAN_POINT('Ctrl Pts',(-3.66663282329846,1.,0.786322922920599));
#52730=CARTESIAN_POINT('',(-4.13571194405636,1.,0.732042837400619));
#52731=CARTESIAN_POINT('Ctrl Pts',(-4.13571194405636,1.,0.732042837400619));
#52732=CARTESIAN_POINT('Ctrl Pts',(-4.13420383737278,1.,0.732488575135926));
#52733=CARTESIAN_POINT('Ctrl Pts',(-4.13118752796397,1.,0.733376589325634));
#52734=CARTESIAN_POINT('Ctrl Pts',(-4.12666277572794,1.,0.734698226767512));
#52735=CARTESIAN_POINT('Ctrl Pts',(-4.12062919626082,1.,0.736439634335347));
#52736=CARTESIAN_POINT('Ctrl Pts',(-4.11308626953795,1.,0.738581708229118));
#52737=CARTESIAN_POINT('Ctrl Pts',(-4.1055424175856,1.,0.740688998555151));
#52738=CARTESIAN_POINT('Ctrl Pts',(-4.09799769702712,1.,0.742761369690017));
#52739=CARTESIAN_POINT('Ctrl Pts',(-4.09045220253011,1.,0.744798649705514));
#52740=CARTESIAN_POINT('Ctrl Pts',(-4.08290608094789,1.,0.746800631490821));
#52741=CARTESIAN_POINT('Ctrl Pts',(-4.07535951055363,1.,0.748767076679177));
#52742=CARTESIAN_POINT('Ctrl Pts',(-4.06781267241886,1.,0.750697720483175));
#52743=CARTESIAN_POINT('Ctrl Pts',(-4.06026572221399,1.,0.752592276482869));
#52744=CARTESIAN_POINT('Ctrl Pts',(-4.05271876688106,1.,0.754450441816411));
#52745=CARTESIAN_POINT('Ctrl Pts',(-4.04517182654344,1.,0.756271902370186));
#52746=CARTESIAN_POINT('Ctrl Pts',(-4.03762485803468,1.,0.758056338885553));
#52747=CARTESIAN_POINT('Ctrl Pts',(-4.0300778195465,1.,0.759803433244166));
#52748=CARTESIAN_POINT('Ctrl Pts',(-4.02253072741347,1.,0.761512875859941));
#52749=CARTESIAN_POINT('Ctrl Pts',(-4.01498370680434,1.,0.763184371182826));
#52750=CARTESIAN_POINT('Ctrl Pts',(-4.00743706791366,1.,0.764817648784946));
#52751=CARTESIAN_POINT('Ctrl Pts',(-3.99989129179464,1.,0.766412457135785));
#52752=CARTESIAN_POINT('Ctrl Pts',(-3.99234687880892,1.,0.767968531377708));
#52753=CARTESIAN_POINT('Ctrl Pts',(-3.98480422348403,1.,0.769485566245459));
#52754=CARTESIAN_POINT('Ctrl Pts',(-3.97726349165507,1.,0.770963190030503));
#52755=CARTESIAN_POINT('Ctrl Pts',(-3.96972446532832,1.,0.772400931772238));
#52756=CARTESIAN_POINT('Ctrl Pts',(-3.96218649639876,1.,0.773798212026682));
#52757=CARTESIAN_POINT('Ctrl Pts',(-3.95464885452364,1.,0.775154418039441));
#52758=CARTESIAN_POINT('Ctrl Pts',(-3.94711101619471,1.,0.77646896669796));
#52759=CARTESIAN_POINT('Ctrl Pts',(-3.93957296768098,1.,0.777741370568549));
#52760=CARTESIAN_POINT('Ctrl Pts',(-3.93203552473153,1.,0.778971308134786));
#52761=CARTESIAN_POINT('Ctrl Pts',(-3.92450058323799,1.,0.780158678615506));
#52762=CARTESIAN_POINT('Ctrl Pts',(-3.9169703605466,1.,0.781303428618343));
#52763=CARTESIAN_POINT('Ctrl Pts',(-3.90944671004536,1.,0.782405395622758));
#52764=CARTESIAN_POINT('Ctrl Pts',(-3.90193039043971,1.,0.783464141529082));
#52765=CARTESIAN_POINT('Ctrl Pts',(-3.89442039235105,1.,0.784478799358335));
#52766=CARTESIAN_POINT('Ctrl Pts',(-3.88691313167399,1.,0.785447890340723));
#52767=CARTESIAN_POINT('Ctrl Pts',(-3.87940402818186,1.,0.786369675812592));
#52768=CARTESIAN_POINT('Ctrl Pts',(-3.87188916600905,1.,0.78724252761798));
#52769=CARTESIAN_POINT('Ctrl Pts',(-3.86436702561342,1.,0.788065315093771));
#52770=CARTESIAN_POINT('Ctrl Pts',(-3.85683995872536,1.,0.788837734090688));
#52771=CARTESIAN_POINT('Ctrl Pts',(-3.8493163780891,1.,0.789560798155618));
#52772=CARTESIAN_POINT('Ctrl Pts',(-3.84180762342476,1.,0.790236124191289));
#52773=CARTESIAN_POINT('Ctrl Pts',(-3.83432392054804,1.,0.79086501270534));
#52774=CARTESIAN_POINT('Ctrl Pts',(-3.82687033899799,1.,0.791447528662381));
#52775=CARTESIAN_POINT('Ctrl Pts',(-3.81944345442237,1.,0.791981740718606));
#52776=CARTESIAN_POINT('Ctrl Pts',(-3.81202588694726,1.,0.792462483517568));
#52777=CARTESIAN_POINT('Ctrl Pts',(-3.80459229925598,1.,0.792882695234693));
#52778=CARTESIAN_POINT('Ctrl Pts',(-3.79711921389862,1.,0.7932356129732));
#52779=CARTESIAN_POINT('Ctrl Pts',(-3.78959439439222,1.,0.793516871680966));
#52780=CARTESIAN_POINT('Ctrl Pts',(-3.78202460377617,1.,0.793726235781339));
#52781=CARTESIAN_POINT('Ctrl Pts',(-3.77444863801264,1.,0.793870523787515));
#52782=CARTESIAN_POINT('Ctrl Pts',(-3.76692626931184,1.,0.793961083689141));
#52783=CARTESIAN_POINT('Ctrl Pts',(-3.75951468666325,1.,0.794008429135047));
#52784=CARTESIAN_POINT('Ctrl Pts',(-3.75224692493895,1.,0.79401734737144));
#52785=CARTESIAN_POINT('Ctrl Pts',(-3.74511357728827,1.,0.79398270045988));
#52786=CARTESIAN_POINT('Ctrl Pts',(-3.73803280541576,1.,0.79388270093679));
#52787=CARTESIAN_POINT('Ctrl Pts',(-3.7308691469564,1.,0.793682750269347));
#52788=CARTESIAN_POINT('Ctrl Pts',(-3.7234879729357,1.,0.79334702378387));
#52789=CARTESIAN_POINT('Ctrl Pts',(-3.7158024239604,1.,0.792848377370115));
#52790=CARTESIAN_POINT('Ctrl Pts',(-3.70781724021879,1.,0.792177688845967));
#52791=CARTESIAN_POINT('Ctrl Pts',(-3.69968940808982,1.,0.791356575696509));
#52792=CARTESIAN_POINT('Ctrl Pts',(-3.69172044327754,1.,0.79043628498958));
#52793=CARTESIAN_POINT('Ctrl Pts',(-3.68428439784285,1.,0.789483546065158));
#52794=CARTESIAN_POINT('Ctrl Pts',(-3.67777119516438,1.,0.788569566220662));
#52795=CARTESIAN_POINT('Ctrl Pts',(-3.672529236635,1.,0.787758799995426));
#52796=CARTESIAN_POINT('Ctrl Pts',(-3.66907505398769,1.,0.787145041181588));
#52797=CARTESIAN_POINT('Ctrl Pts',(-3.66743103898844,1.,0.786774337198499));
#52798=CARTESIAN_POINT('Ctrl Pts',(-3.66680946938396,1.,0.786565919559889));
#52799=CARTESIAN_POINT('Ctrl Pts',(-3.66664310415236,1.,0.786459983896781));
#52800=CARTESIAN_POINT('Ctrl Pts',(-3.66661143271648,1.,0.786422660833743));
#52801=CARTESIAN_POINT('',(-4.13571194405636,0.,0.732042837400619));
#52802=CARTESIAN_POINT('Ctrl Pts',(-3.73016218570874,-1.,0.385214314776329));
#52803=CARTESIAN_POINT('Ctrl Pts',(-3.73016218570874,1.,0.385214314776329));
#52804=CARTESIAN_POINT('Ctrl Pts',(-3.73010668803185,-1.,0.385147278814804));
#52805=CARTESIAN_POINT('Ctrl Pts',(-3.73010668803185,1.,0.385147278814804));
#52806=CARTESIAN_POINT('Ctrl Pts',(-3.73015851028729,-1.,0.385047711603887));
#52807=CARTESIAN_POINT('Ctrl Pts',(-3.73015851028729,1.,0.385047711603887));
#52808=CARTESIAN_POINT('Ctrl Pts',(-3.73072465900727,-1.,0.385001870183841));
#52809=CARTESIAN_POINT('Ctrl Pts',(-3.73072465900727,1.,0.385001870183841));
#52810=CARTESIAN_POINT('Ctrl Pts',(-3.73245705639337,-1.,0.385147887989514));
#52811=CARTESIAN_POINT('Ctrl Pts',(-3.73245705639337,1.,0.385147887989514));
#52812=CARTESIAN_POINT('Ctrl Pts',(-3.73621371845475,-1.,0.385670806454744));
#52813=CARTESIAN_POINT('Ctrl Pts',(-3.73621371845475,1.,0.385670806454744));
#52814=CARTESIAN_POINT('Ctrl Pts',(-3.74144965781088,-1.,0.386519576222035));
#52815=CARTESIAN_POINT('Ctrl Pts',(-3.74144965781088,1.,0.386519576222035));
#52816=CARTESIAN_POINT('Ctrl Pts',(-3.74792651696269,-1.,0.387663020050396));
#52817=CARTESIAN_POINT('Ctrl Pts',(-3.74792651696269,1.,0.387663020050396));
#52818=CARTESIAN_POINT('Ctrl Pts',(-3.75529302894757,-1.,0.389054775898251));
#52819=CARTESIAN_POINT('Ctrl Pts',(-3.75529302894757,1.,0.389054775898251));
#52820=CARTESIAN_POINT('Ctrl Pts',(-3.76315635032993,-1.,0.390642072979259));
#52821=CARTESIAN_POINT('Ctrl Pts',(-3.76315635032993,1.,0.390642072979259));
#52822=CARTESIAN_POINT('Ctrl Pts',(-3.77114011595892,-1.,0.392372786223346));
#52823=CARTESIAN_POINT('Ctrl Pts',(-3.77114011595892,1.,0.392372786223346));
#52824=CARTESIAN_POINT('Ctrl Pts',(-3.77894173114368,-1.,0.394202481011595));
#52825=CARTESIAN_POINT('Ctrl Pts',(-3.77894173114368,1.,0.394202481011595));
#52826=CARTESIAN_POINT('Ctrl Pts',(-3.78640521279479,-1.,0.396103205335028));
#52827=CARTESIAN_POINT('Ctrl Pts',(-3.78640521279479,1.,0.396103205335028));
#52828=CARTESIAN_POINT('Ctrl Pts',(-3.79352887163457,-1.,0.398064818684158));
#52829=CARTESIAN_POINT('Ctrl Pts',(-3.79352887163457,1.,0.398064818684158));
#52830=CARTESIAN_POINT('Ctrl Pts',(-3.80040370384659,-1.,0.400088346504726));
#52831=CARTESIAN_POINT('Ctrl Pts',(-3.80040370384659,1.,0.400088346504726));
#52832=CARTESIAN_POINT('Ctrl Pts',(-3.80716881962763,-1.,0.402181320148474));
#52833=CARTESIAN_POINT('Ctrl Pts',(-3.80716881962763,1.,0.402181320148474));
#52834=CARTESIAN_POINT('Ctrl Pts',(-3.81396374287762,-1.,0.404352694628236));
#52835=CARTESIAN_POINT('Ctrl Pts',(-3.81396374287762,1.,0.404352694628236));
#52836=CARTESIAN_POINT('Ctrl Pts',(-3.82087303913741,-1.,0.406607038258906));
#52837=CARTESIAN_POINT('Ctrl Pts',(-3.82087303913741,1.,0.406607038258906));
#52838=CARTESIAN_POINT('Ctrl Pts',(-3.82790724256397,-1.,0.408942371447377));
#52839=CARTESIAN_POINT('Ctrl Pts',(-3.82790724256397,1.,0.408942371447377));
#52840=CARTESIAN_POINT('Ctrl Pts',(-3.83503345578645,-1.,0.411353038798459));
#52841=CARTESIAN_POINT('Ctrl Pts',(-3.83503345578645,1.,0.411353038798459));
#52842=CARTESIAN_POINT('Ctrl Pts',(-3.84219403994742,-1.,0.413831367016726));
#52843=CARTESIAN_POINT('Ctrl Pts',(-3.84219403994742,1.,0.413831367016726));
#52844=CARTESIAN_POINT('Ctrl Pts',(-3.8493286415751,-1.,0.41636967805292));
#52845=CARTESIAN_POINT('Ctrl Pts',(-3.8493286415751,1.,0.41636967805292));
#52846=CARTESIAN_POINT('Ctrl Pts',(-3.85639825648031,-1.,0.418962468086809));
#52847=CARTESIAN_POINT('Ctrl Pts',(-3.85639825648031,1.,0.418962468086809));
#52848=CARTESIAN_POINT('Ctrl Pts',(-3.86339652542749,-1.,0.421607423177575));
#52849=CARTESIAN_POINT('Ctrl Pts',(-3.86339652542749,1.,0.421607423177575));
#52850=CARTESIAN_POINT('Ctrl Pts',(-3.87033643487882,-1.,0.424304173195142));
#52851=CARTESIAN_POINT('Ctrl Pts',(-3.87033643487882,1.,0.424304173195142));
#52852=CARTESIAN_POINT('Ctrl Pts',(-3.87724240306609,-1.,0.427053541173469));
#52853=CARTESIAN_POINT('Ctrl Pts',(-3.87724240306609,1.,0.427053541173469));
#52854=CARTESIAN_POINT('Ctrl Pts',(-3.88414070943334,-1.,0.429856640579733));
#52855=CARTESIAN_POINT('Ctrl Pts',(-3.88414070943334,1.,0.429856640579733));
#52856=CARTESIAN_POINT('Ctrl Pts',(-3.89104947940592,-1.,0.432713929544439));
#52857=CARTESIAN_POINT('Ctrl Pts',(-3.89104947940592,1.,0.432713929544439));
#52858=CARTESIAN_POINT('Ctrl Pts',(-3.8979725665544,-1.,0.435624629433505));
#52859=CARTESIAN_POINT('Ctrl Pts',(-3.8979725665544,1.,0.435624629433505));
#52860=CARTESIAN_POINT('Ctrl Pts',(-3.90490512938546,-1.,0.438587235458233));
#52861=CARTESIAN_POINT('Ctrl Pts',(-3.90490512938546,1.,0.438587235458233));
#52862=CARTESIAN_POINT('Ctrl Pts',(-3.91183704069146,-1.,0.441599824524047));
#52863=CARTESIAN_POINT('Ctrl Pts',(-3.91183704069146,1.,0.441599824524047));
#52864=CARTESIAN_POINT('Ctrl Pts',(-3.91875701610721,-1.,0.444660430230592));
#52865=CARTESIAN_POINT('Ctrl Pts',(-3.91875701610721,1.,0.444660430230592));
#52866=CARTESIAN_POINT('Ctrl Pts',(-3.92565674143424,-1.,0.447767416837296));
#52867=CARTESIAN_POINT('Ctrl Pts',(-3.92565674143424,1.,0.447767416837296));
#52868=CARTESIAN_POINT('Ctrl Pts',(-3.93253407403128,-1.,0.450919768356347));
#52869=CARTESIAN_POINT('Ctrl Pts',(-3.93253407403128,1.,0.450919768356347));
#52870=CARTESIAN_POINT('Ctrl Pts',(-3.93939080846298,-1.,0.454116879027576));
#52871=CARTESIAN_POINT('Ctrl Pts',(-3.93939080846298,1.,0.454116879027576));
#52872=CARTESIAN_POINT('Ctrl Pts',(-3.94623117206675,-1.,0.457358410451674));
#52873=CARTESIAN_POINT('Ctrl Pts',(-3.94623117206675,1.,0.457358410451674));
#52874=CARTESIAN_POINT('Ctrl Pts',(-3.95306005817363,-1.,0.460644124429119));
#52875=CARTESIAN_POINT('Ctrl Pts',(-3.95306005817363,1.,0.460644124429119));
#52876=CARTESIAN_POINT('Ctrl Pts',(-3.95988133243543,-1.,0.463973722115744));
#52877=CARTESIAN_POINT('Ctrl Pts',(-3.95988133243543,1.,0.463973722115744));
#52878=CARTESIAN_POINT('Ctrl Pts',(-3.96669622273946,-1.,0.467346690880671));
#52879=CARTESIAN_POINT('Ctrl Pts',(-3.96669622273946,1.,0.467346690880671));
#52880=CARTESIAN_POINT('Ctrl Pts',(-3.97350414289415,-1.,0.470762379613477));
#52881=CARTESIAN_POINT('Ctrl Pts',(-3.97350414289415,1.,0.470762379613477));
#52882=CARTESIAN_POINT('Ctrl Pts',(-3.9803033804443,-1.,0.474220061019542));
#52883=CARTESIAN_POINT('Ctrl Pts',(-3.9803033804443,1.,0.474220061019542));
#52884=CARTESIAN_POINT('Ctrl Pts',(-3.98709184306743,-1.,0.477718999122033));
#52885=CARTESIAN_POINT('Ctrl Pts',(-3.98709184306743,1.,0.477718999122033));
#52886=CARTESIAN_POINT('Ctrl Pts',(-3.99386775880655,-1.,0.481258512209638));
#52887=CARTESIAN_POINT('Ctrl Pts',(-3.99386775880655,1.,0.481258512209638));
#52888=CARTESIAN_POINT('Ctrl Pts',(-4.00063045119234,-1.,0.484838042421754));
#52889=CARTESIAN_POINT('Ctrl Pts',(-4.00063045119234,1.,0.484838042421754));
#52890=CARTESIAN_POINT('Ctrl Pts',(-4.0073800839092,-1.,0.48845713042453));
#52891=CARTESIAN_POINT('Ctrl Pts',(-4.0073800839092,1.,0.48845713042453));
#52892=CARTESIAN_POINT('Ctrl Pts',(-4.01411733503486,-1.,0.49211538341793));
#52893=CARTESIAN_POINT('Ctrl Pts',(-4.01411733503486,1.,0.49211538341793));
#52894=CARTESIAN_POINT('Ctrl Pts',(-4.02084308851813,-1.,0.495812444326223));
#52895=CARTESIAN_POINT('Ctrl Pts',(-4.02084308851813,1.,0.495812444326223));
#52896=CARTESIAN_POINT('Ctrl Pts',(-4.0275581398015,-1.,0.499547962340889));
#52897=CARTESIAN_POINT('Ctrl Pts',(-4.0275581398015,1.,0.499547962340889));
#52898=CARTESIAN_POINT('Ctrl Pts',(-4.0342628417439,-1.,0.503321556915513));
#52899=CARTESIAN_POINT('Ctrl Pts',(-4.0342628417439,1.,0.503321556915513));
#52900=CARTESIAN_POINT('Ctrl Pts',(-4.04095715149074,-1.,0.507132823288361));
#52901=CARTESIAN_POINT('Ctrl Pts',(-4.04095715149074,1.,0.507132823288361));
#52902=CARTESIAN_POINT('Ctrl Pts',(-4.04764078815591,-1.,0.510981349219173));
#52903=CARTESIAN_POINT('Ctrl Pts',(-4.04764078815591,1.,0.510981349219173));
#52904=CARTESIAN_POINT('Ctrl Pts',(-4.05431335771261,-1.,0.514866728193104));
#52905=CARTESIAN_POINT('Ctrl Pts',(-4.05431335771261,1.,0.514866728193104));
#52906=CARTESIAN_POINT('Ctrl Pts',(-4.06097448037934,-1.,0.518788572336809));
#52907=CARTESIAN_POINT('Ctrl Pts',(-4.06097448037934,1.,0.518788572336809));
#52908=CARTESIAN_POINT('Ctrl Pts',(-4.06762394471075,-1.,0.522746528602767));
#52909=CARTESIAN_POINT('Ctrl Pts',(-4.06762394471075,1.,0.522746528602767));
#52910=CARTESIAN_POINT('Ctrl Pts',(-4.07426172299496,-1.,0.526740277226999));
#52911=CARTESIAN_POINT('Ctrl Pts',(-4.07426172299496,1.,0.526740277226999));
#52912=CARTESIAN_POINT('Ctrl Pts',(-4.08088789536488,-1.,0.530769518728075));
#52913=CARTESIAN_POINT('Ctrl Pts',(-4.08088789536488,1.,0.530769518728075));
#52914=CARTESIAN_POINT('Ctrl Pts',(-4.08750259988693,-1.,0.534833963476999));
#52915=CARTESIAN_POINT('Ctrl Pts',(-4.08750259988693,1.,0.534833963476999));
#52916=CARTESIAN_POINT('Ctrl Pts',(-4.09410597627116,-1.,0.53893332117992));
#52917=CARTESIAN_POINT('Ctrl Pts',(-4.09410597627116,1.,0.53893332117992));
#52918=CARTESIAN_POINT('Ctrl Pts',(-4.10069810244473,-1.,0.543067286878457));
#52919=CARTESIAN_POINT('Ctrl Pts',(-4.10069810244473,1.,0.543067286878457));
#52920=CARTESIAN_POINT('Ctrl Pts',(-4.1072789702877,-1.,0.547235539486759));
#52921=CARTESIAN_POINT('Ctrl Pts',(-4.1072789702877,1.,0.547235539486759));
#52922=CARTESIAN_POINT('Ctrl Pts',(-4.11384852025578,-1.,0.551437758498246));
#52923=CARTESIAN_POINT('Ctrl Pts',(-4.11384852025578,1.,0.551437758498246));
#52924=CARTESIAN_POINT('Ctrl Pts',(-4.1204066619623,-1.,0.555673636130778));
#52925=CARTESIAN_POINT('Ctrl Pts',(-4.1204066619623,1.,0.555673636130778));
#52926=CARTESIAN_POINT('Ctrl Pts',(-4.12695329951859,-1.,0.559942890594628));
#52927=CARTESIAN_POINT('Ctrl Pts',(-4.12695329951859,1.,0.559942890594628));
#52928=CARTESIAN_POINT('Ctrl Pts',(-4.13348835726086,-1.,0.564245279535705));
#52929=CARTESIAN_POINT('Ctrl Pts',(-4.13348835726086,1.,0.564245279535705));
#52930=CARTESIAN_POINT('Ctrl Pts',(-4.14001179828669,-1.,0.568580610187116));
#52931=CARTESIAN_POINT('Ctrl Pts',(-4.14001179828669,1.,0.568580610187116));
#52932=CARTESIAN_POINT('Ctrl Pts',(-4.14652361065787,-1.,0.572948736066276));
#52933=CARTESIAN_POINT('Ctrl Pts',(-4.14652361065787,1.,0.572948736066276));
#52934=CARTESIAN_POINT('Ctrl Pts',(-4.1517237611974,-1.,0.576469391673916));
#52935=CARTESIAN_POINT('Ctrl Pts',(-4.1517237611974,1.,0.576469391673916));
#52936=CARTESIAN_POINT('Ctrl Pts',(-4.15561864787379,-1.,0.579124568912543));
#52937=CARTESIAN_POINT('Ctrl Pts',(-4.15561864787379,1.,0.579124568912543));
#52938=CARTESIAN_POINT('Ctrl Pts',(-4.15821291712391,-1.,0.580901211462913));
#52939=CARTESIAN_POINT('Ctrl Pts',(-4.15821291712391,1.,0.580901211462913));
#52940=CARTESIAN_POINT('Ctrl Pts',(-4.15950947128175,-1.,0.581791163835814));
#52941=CARTESIAN_POINT('Ctrl Pts',(-4.15950947128175,1.,0.581791163835814));
#52942=CARTESIAN_POINT('',(-3.73017266276632,1.,0.385112848332549));
#52943=CARTESIAN_POINT('Ctrl Pts',(-3.73017266276632,-1.,0.385112848332549));
#52944=CARTESIAN_POINT('Ctrl Pts',(-3.73017266276632,-0.666666666666667,
0.385112848332549));
#52945=CARTESIAN_POINT('Ctrl Pts',(-3.73017266276632,-0.333333333333333,
0.385112848332549));
#52946=CARTESIAN_POINT('Ctrl Pts',(-3.73017266276632,0.333333333333333,
0.385112848332549));
#52947=CARTESIAN_POINT('Ctrl Pts',(-3.73017266276632,0.666666666666667,
0.385112848332549));
#52948=CARTESIAN_POINT('Ctrl Pts',(-3.73017266276632,1.,0.385112848332549));
#52949=CARTESIAN_POINT('',(-4.15950947128175,1.,0.581791163835814));
#52950=CARTESIAN_POINT('',(-4.15950947128175,0.,0.581791163835814));
#52951=CARTESIAN_POINT('Ctrl Pts',(-3.73017266276632,1.,0.385112848332549));
#52952=CARTESIAN_POINT('Ctrl Pts',(-3.73021431755218,1.,0.385087139001609));
#52953=CARTESIAN_POINT('Ctrl Pts',(-3.73040527620929,1.,0.385037797882046));
#52954=CARTESIAN_POINT('Ctrl Pts',(-3.73106082862399,1.,0.385031656499141));
#52955=CARTESIAN_POINT('Ctrl Pts',(-3.73273893363318,1.,0.385187124633964));
#52956=CARTESIAN_POINT('Ctrl Pts',(-3.73621371845475,1.,0.385670806454744));
#52957=CARTESIAN_POINT('Ctrl Pts',(-3.74144965781088,1.,0.386519576222035));
#52958=CARTESIAN_POINT('Ctrl Pts',(-3.74792651696269,1.,0.387663020050396));
#52959=CARTESIAN_POINT('Ctrl Pts',(-3.75529302894757,1.,0.389054775898251));
#52960=CARTESIAN_POINT('Ctrl Pts',(-3.76315635032993,1.,0.390642072979259));
#52961=CARTESIAN_POINT('Ctrl Pts',(-3.77114011595892,1.,0.392372786223346));
#52962=CARTESIAN_POINT('Ctrl Pts',(-3.77894173114368,1.,0.394202481011595));
#52963=CARTESIAN_POINT('Ctrl Pts',(-3.78640521279479,1.,0.396103205335028));
#52964=CARTESIAN_POINT('Ctrl Pts',(-3.79352887163457,1.,0.398064818684158));
#52965=CARTESIAN_POINT('Ctrl Pts',(-3.80040370384659,1.,0.400088346504726));
#52966=CARTESIAN_POINT('Ctrl Pts',(-3.80716881962763,1.,0.402181320148474));
#52967=CARTESIAN_POINT('Ctrl Pts',(-3.81396374287762,1.,0.404352694628236));
#52968=CARTESIAN_POINT('Ctrl Pts',(-3.82087303913741,1.,0.406607038258906));
#52969=CARTESIAN_POINT('Ctrl Pts',(-3.82790724256397,1.,0.408942371447377));
#52970=CARTESIAN_POINT('Ctrl Pts',(-3.83503345578645,1.,0.411353038798459));
#52971=CARTESIAN_POINT('Ctrl Pts',(-3.84219403994742,1.,0.413831367016726));
#52972=CARTESIAN_POINT('Ctrl Pts',(-3.8493286415751,1.,0.41636967805292));
#52973=CARTESIAN_POINT('Ctrl Pts',(-3.85639825648031,1.,0.418962468086809));
#52974=CARTESIAN_POINT('Ctrl Pts',(-3.86339652542749,1.,0.421607423177575));
#52975=CARTESIAN_POINT('Ctrl Pts',(-3.87033643487882,1.,0.424304173195142));
#52976=CARTESIAN_POINT('Ctrl Pts',(-3.87724240306609,1.,0.427053541173469));
#52977=CARTESIAN_POINT('Ctrl Pts',(-3.88414070943334,1.,0.429856640579733));
#52978=CARTESIAN_POINT('Ctrl Pts',(-3.89104947940592,1.,0.432713929544439));
#52979=CARTESIAN_POINT('Ctrl Pts',(-3.8979725665544,1.,0.435624629433505));
#52980=CARTESIAN_POINT('Ctrl Pts',(-3.90490512938546,1.,0.438587235458233));
#52981=CARTESIAN_POINT('Ctrl Pts',(-3.91183704069146,1.,0.441599824524047));
#52982=CARTESIAN_POINT('Ctrl Pts',(-3.91875701610721,1.,0.444660430230592));
#52983=CARTESIAN_POINT('Ctrl Pts',(-3.92565674143424,1.,0.447767416837296));
#52984=CARTESIAN_POINT('Ctrl Pts',(-3.93253407403128,1.,0.450919768356347));
#52985=CARTESIAN_POINT('Ctrl Pts',(-3.93939080846298,1.,0.454116879027576));
#52986=CARTESIAN_POINT('Ctrl Pts',(-3.94623117206675,1.,0.457358410451674));
#52987=CARTESIAN_POINT('Ctrl Pts',(-3.95306005817363,1.,0.460644124429119));
#52988=CARTESIAN_POINT('Ctrl Pts',(-3.95988133243543,1.,0.463973722115744));
#52989=CARTESIAN_POINT('Ctrl Pts',(-3.96669622273946,1.,0.467346690880671));
#52990=CARTESIAN_POINT('Ctrl Pts',(-3.97350414289415,1.,0.470762379613477));
#52991=CARTESIAN_POINT('Ctrl Pts',(-3.9803033804443,1.,0.474220061019542));
#52992=CARTESIAN_POINT('Ctrl Pts',(-3.98709184306743,1.,0.477718999122033));
#52993=CARTESIAN_POINT('Ctrl Pts',(-3.99386775880655,1.,0.481258512209638));
#52994=CARTESIAN_POINT('Ctrl Pts',(-4.00063045119234,1.,0.484838042421754));
#52995=CARTESIAN_POINT('Ctrl Pts',(-4.0073800839092,1.,0.48845713042453));
#52996=CARTESIAN_POINT('Ctrl Pts',(-4.01411733503486,1.,0.49211538341793));
#52997=CARTESIAN_POINT('Ctrl Pts',(-4.02084308851813,1.,0.495812444326223));
#52998=CARTESIAN_POINT('Ctrl Pts',(-4.0275581398015,1.,0.499547962340889));
#52999=CARTESIAN_POINT('Ctrl Pts',(-4.0342628417439,1.,0.503321556915513));
#53000=CARTESIAN_POINT('Ctrl Pts',(-4.04095715149074,1.,0.507132823288361));
#53001=CARTESIAN_POINT('Ctrl Pts',(-4.04764078815591,1.,0.510981349219173));
#53002=CARTESIAN_POINT('Ctrl Pts',(-4.05431335771261,1.,0.514866728193104));
#53003=CARTESIAN_POINT('Ctrl Pts',(-4.06097448037934,1.,0.518788572336809));
#53004=CARTESIAN_POINT('Ctrl Pts',(-4.06762394471075,1.,0.522746528602767));
#53005=CARTESIAN_POINT('Ctrl Pts',(-4.07426172299496,1.,0.526740277226999));
#53006=CARTESIAN_POINT('Ctrl Pts',(-4.08088789536488,1.,0.530769518728075));
#53007=CARTESIAN_POINT('Ctrl Pts',(-4.08750259988693,1.,0.534833963476999));
#53008=CARTESIAN_POINT('Ctrl Pts',(-4.09410597627116,1.,0.53893332117992));
#53009=CARTESIAN_POINT('Ctrl Pts',(-4.10069810244473,1.,0.543067286878457));
#53010=CARTESIAN_POINT('Ctrl Pts',(-4.1072789702877,1.,0.547235539486759));
#53011=CARTESIAN_POINT('Ctrl Pts',(-4.11384852025578,1.,0.551437758498246));
#53012=CARTESIAN_POINT('Ctrl Pts',(-4.1204066619623,1.,0.555673636130778));
#53013=CARTESIAN_POINT('Ctrl Pts',(-4.12695329951859,1.,0.559942890594628));
#53014=CARTESIAN_POINT('Ctrl Pts',(-4.13348835726086,1.,0.564245279535705));
#53015=CARTESIAN_POINT('Ctrl Pts',(-4.14001179828669,1.,0.568580610187116));
#53016=CARTESIAN_POINT('Ctrl Pts',(-4.14652361065787,1.,0.572948736066276));
#53017=CARTESIAN_POINT('Ctrl Pts',(-4.1517237611974,1.,0.576469391673916));
#53018=CARTESIAN_POINT('Ctrl Pts',(-4.15561864787379,1.,0.579124568912543));
#53019=CARTESIAN_POINT('Ctrl Pts',(-4.15821291712391,1.,0.580901211462913));
#53020=CARTESIAN_POINT('Ctrl Pts',(-4.15950947128175,1.,0.581791163835814));
#53021=CARTESIAN_POINT('Origin',(-4.15950947128175,0.,0.581791163835814));
#53022=CARTESIAN_POINT('',(-4.13571194405636,1.,0.732042837400619));
#53023=CARTESIAN_POINT('Origin',(0.,0.,0.));
#53024=CARTESIAN_POINT('',(-3.74449296982994,1.,0.203156094897896));
#53025=CARTESIAN_POINT('Origin',(0.,1.,0.));
#53026=CARTESIAN_POINT('Ctrl Pts',(-3.74449296982994,1.,0.203156094897896));
#53027=CARTESIAN_POINT('Ctrl Pts',(-3.74449296982994,0.666666666666667,
0.203156094897896));
#53028=CARTESIAN_POINT('Ctrl Pts',(-3.74449296982994,0.333333333333333,
0.203156094897896));
#53029=CARTESIAN_POINT('Ctrl Pts',(-3.74449296982994,-0.333333333333333,
0.203156094897896));
#53030=CARTESIAN_POINT('Ctrl Pts',(-3.74449296982994,-0.666666666666667,
0.203156094897896));
#53031=CARTESIAN_POINT('Ctrl Pts',(-3.74449296982994,-1.,0.203156094897896));
#53032=CARTESIAN_POINT('Ctrl Pts',(-4.19931119685982,-1.,0.0760622897878236));
#53033=CARTESIAN_POINT('Ctrl Pts',(-4.19931119685982,1.,0.0760622897878236));
#53034=CARTESIAN_POINT('Ctrl Pts',(-4.19789138621624,-1.,0.0767384596142195));
#53035=CARTESIAN_POINT('Ctrl Pts',(-4.19789138621624,1.,0.0767384596142195));
#53036=CARTESIAN_POINT('Ctrl Pts',(-4.19505112860624,-1.,0.0780873956244402));
#53037=CARTESIAN_POINT('Ctrl Pts',(-4.19505112860624,1.,0.0780873956244402));
#53038=CARTESIAN_POINT('Ctrl Pts',(-4.19078883322483,-1.,0.0801005887117603));
#53039=CARTESIAN_POINT('Ctrl Pts',(-4.19078883322483,1.,0.0801005887117603));
#53040=CARTESIAN_POINT('Ctrl Pts',(-4.1851019532944,-1.,0.082764416438951));
#53041=CARTESIAN_POINT('Ctrl Pts',(-4.1851019532944,1.,0.082764416438951));
#53042=CARTESIAN_POINT('Ctrl Pts',(-4.17798698669991,-1.,0.0860600915552515));
#53043=CARTESIAN_POINT('Ctrl Pts',(-4.17798698669991,1.,0.0860600915552515));
#53044=CARTESIAN_POINT('Ctrl Pts',(-4.17086566491823,-1.,0.0893215560850327));
#53045=CARTESIAN_POINT('Ctrl Pts',(-4.17086566491823,1.,0.0893215560850327));
#53046=CARTESIAN_POINT('Ctrl Pts',(-4.16373802265942,-1.,0.092548667216769));
#53047=CARTESIAN_POINT('Ctrl Pts',(-4.16373802265942,1.,0.092548667216769));
#53048=CARTESIAN_POINT('Ctrl Pts',(-4.15660412653006,-1.,0.0957412403297067));
#53049=CARTESIAN_POINT('Ctrl Pts',(-4.15660412653006,1.,0.0957412403297067));
#53050=CARTESIAN_POINT('Ctrl Pts',(-4.1494640891762,-1.,0.0988990478899811));
#53051=CARTESIAN_POINT('Ctrl Pts',(-4.1494640891762,1.,0.0988990478899811));
#53052=CARTESIAN_POINT('Ctrl Pts',(-4.14231804938737,-1.,0.102021826577454));
#53053=CARTESIAN_POINT('Ctrl Pts',(-4.14231804938737,1.,0.102021826577454));
#53054=CARTESIAN_POINT('Ctrl Pts',(-4.13516614458396,-1.,0.105109286538864));
#53055=CARTESIAN_POINT('Ctrl Pts',(-4.13516614458396,1.,0.105109286538864));
#53056=CARTESIAN_POINT('Ctrl Pts',(-4.12800848371386,-1.,0.10816112052835));
#53057=CARTESIAN_POINT('Ctrl Pts',(-4.12800848371386,1.,0.10816112052835));
#53058=CARTESIAN_POINT('Ctrl Pts',(-4.12084512502444,-1.,0.111177012683377));
#53059=CARTESIAN_POINT('Ctrl Pts',(-4.12084512502444,1.,0.111177012683377));
#53060=CARTESIAN_POINT('Ctrl Pts',(-4.11367603925313,-1.,0.114156649609601));
#53061=CARTESIAN_POINT('Ctrl Pts',(-4.11367603925313,1.,0.114156649609601));
#53062=CARTESIAN_POINT('Ctrl Pts',(-4.10650113382187,-1.,0.117099722731704));
#53063=CARTESIAN_POINT('Ctrl Pts',(-4.10650113382187,1.,0.117099722731704));
#53064=CARTESIAN_POINT('Ctrl Pts',(-4.09932031767243,-1.,0.120005924388162));
#53065=CARTESIAN_POINT('Ctrl Pts',(-4.09932031767243,1.,0.120005924388162));
#53066=CARTESIAN_POINT('Ctrl Pts',(-4.09213355850836,-1.,0.122874946249119));
#53067=CARTESIAN_POINT('Ctrl Pts',(-4.09213355850836,1.,0.122874946249119));
#53068=CARTESIAN_POINT('Ctrl Pts',(-4.08494093372315,-1.,0.125706476822529));
#53069=CARTESIAN_POINT('Ctrl Pts',(-4.08494093372315,1.,0.125706476822529));
#53070=CARTESIAN_POINT('Ctrl Pts',(-4.07774270738809,-1.,0.128500200484814));
#53071=CARTESIAN_POINT('Ctrl Pts',(-4.07774270738809,1.,0.128500200484814));
#53072=CARTESIAN_POINT('Ctrl Pts',(-4.07053931528579,-1.,0.131255793548914));
#53073=CARTESIAN_POINT('Ctrl Pts',(-4.07053931528579,1.,0.131255793548914));
#53074=CARTESIAN_POINT('Ctrl Pts',(-4.06333121018476,-1.,0.133972916144225));
#53075=CARTESIAN_POINT('Ctrl Pts',(-4.06333121018476,1.,0.133972916144225));
#53076=CARTESIAN_POINT('Ctrl Pts',(-4.05611873400122,-1.,0.136651205046111));
#53077=CARTESIAN_POINT('Ctrl Pts',(-4.05611873400122,1.,0.136651205046111));
#53078=CARTESIAN_POINT('Ctrl Pts',(-4.04890199238056,-1.,0.139290267180059));
#53079=CARTESIAN_POINT('Ctrl Pts',(-4.04890199238056,1.,0.139290267180059));
#53080=CARTESIAN_POINT('Ctrl Pts',(-4.04168069633842,-1.,0.141889671485508));
#53081=CARTESIAN_POINT('Ctrl Pts',(-4.04168069633842,1.,0.141889671485508));
#53082=CARTESIAN_POINT('Ctrl Pts',(-4.03445411510403,-1.,0.144448947038352));
#53083=CARTESIAN_POINT('Ctrl Pts',(-4.03445411510403,1.,0.144448947038352));
#53084=CARTESIAN_POINT('Ctrl Pts',(-4.02722143147048,-1.,0.146967602878998));
#53085=CARTESIAN_POINT('Ctrl Pts',(-4.02722143147048,1.,0.146967602878998));
#53086=CARTESIAN_POINT('Ctrl Pts',(-4.01998203715588,-1.,0.149445144968707));
#53087=CARTESIAN_POINT('Ctrl Pts',(-4.01998203715588,1.,0.149445144968707));
#53088=CARTESIAN_POINT('Ctrl Pts',(-4.01273584234684,-1.,0.151881094022909));
#53089=CARTESIAN_POINT('Ctrl Pts',(-4.01273584234684,1.,0.151881094022909));
#53090=CARTESIAN_POINT('Ctrl Pts',(-4.00548360245297,-1.,0.15427500487231));
#53091=CARTESIAN_POINT('Ctrl Pts',(-4.00548360245297,1.,0.15427500487231));
#53092=CARTESIAN_POINT('Ctrl Pts',(-3.99822717425869,-1.,0.156626481393735));
#53093=CARTESIAN_POINT('Ctrl Pts',(-3.99822717425869,1.,0.156626481393735));
#53094=CARTESIAN_POINT('Ctrl Pts',(-3.99096873945862,-1.,0.158935123982796));
#53095=CARTESIAN_POINT('Ctrl Pts',(-3.99096873945862,1.,0.158935123982796));
#53096=CARTESIAN_POINT('Ctrl Pts',(-3.98371010319866,-1.,0.161200482186087));
#53097=CARTESIAN_POINT('Ctrl Pts',(-3.98371010319866,1.,0.161200482186087));
#53098=CARTESIAN_POINT('Ctrl Pts',(-3.97645194630944,-1.,0.163422004609999));
#53099=CARTESIAN_POINT('Ctrl Pts',(-3.97645194630944,1.,0.163422004609999));
#53100=CARTESIAN_POINT('Ctrl Pts',(-3.9691931362141,-1.,0.165598992851097));
#53101=CARTESIAN_POINT('Ctrl Pts',(-3.9691931362141,1.,0.165598992851097));
#53102=CARTESIAN_POINT('Ctrl Pts',(-3.96192990160296,-1.,0.167730547023312));
#53103=CARTESIAN_POINT('Ctrl Pts',(-3.96192990160296,1.,0.167730547023312));
#53104=CARTESIAN_POINT('Ctrl Pts',(-3.95465744665263,-1.,0.16981566637413));
#53105=CARTESIAN_POINT('Ctrl Pts',(-3.95465744665263,1.,0.16981566637413));
#53106=CARTESIAN_POINT('Ctrl Pts',(-3.94737164900861,-1.,0.171853355369233));
#53107=CARTESIAN_POINT('Ctrl Pts',(-3.94737164900861,1.,0.171853355369233));
#53108=CARTESIAN_POINT('Ctrl Pts',(-3.94007083096214,-1.,0.173842734974607));
#53109=CARTESIAN_POINT('Ctrl Pts',(-3.94007083096214,1.,0.173842734974607));
#53110=CARTESIAN_POINT('Ctrl Pts',(-3.93275726771049,-1.,0.175783136893872));
#53111=CARTESIAN_POINT('Ctrl Pts',(-3.93275726771049,1.,0.175783136893872));
#53112=CARTESIAN_POINT('Ctrl Pts',(-3.92543942697672,-1.,0.177674246152328));
#53113=CARTESIAN_POINT('Ctrl Pts',(-3.92543942697672,1.,0.177674246152328));
#53114=CARTESIAN_POINT('Ctrl Pts',(-3.91812876180948,-1.,0.179515885822894));
#53115=CARTESIAN_POINT('Ctrl Pts',(-3.91812876180948,1.,0.179515885822894));
#53116=CARTESIAN_POINT('Ctrl Pts',(-3.91083557557193,-1.,0.181307740731796));
#53117=CARTESIAN_POINT('Ctrl Pts',(-3.91083557557193,1.,0.181307740731796));
#53118=CARTESIAN_POINT('Ctrl Pts',(-3.90356488555138,-1.,0.183049081993193));
#53119=CARTESIAN_POINT('Ctrl Pts',(-3.90356488555138,1.,0.183049081993193));
#53120=CARTESIAN_POINT('Ctrl Pts',(-3.89631300742633,-1.,0.184738537728035));
#53121=CARTESIAN_POINT('Ctrl Pts',(-3.89631300742633,1.,0.184738537728035));
#53122=CARTESIAN_POINT('Ctrl Pts',(-3.88906196725817,-1.,0.186373724985263));
#53123=CARTESIAN_POINT('Ctrl Pts',(-3.88906196725817,1.,0.186373724985263));
#53124=CARTESIAN_POINT('Ctrl Pts',(-3.88178563496187,-1.,0.187951632512663));
#53125=CARTESIAN_POINT('Ctrl Pts',(-3.88178563496187,1.,0.187951632512663));
#53126=CARTESIAN_POINT('Ctrl Pts',(-3.87445976418377,-1.,0.189469253358254));
#53127=CARTESIAN_POINT('Ctrl Pts',(-3.87445976418377,1.,0.189469253358254));
#53128=CARTESIAN_POINT('Ctrl Pts',(-3.8670715862477,-1.,0.190924190418613));
#53129=CARTESIAN_POINT('Ctrl Pts',(-3.8670715862477,1.,0.190924190418613));
#53130=CARTESIAN_POINT('Ctrl Pts',(-3.85962774407652,-1.,0.192315153044979));
#53131=CARTESIAN_POINT('Ctrl Pts',(-3.85962774407652,1.,0.192315153044979));
#53132=CARTESIAN_POINT('Ctrl Pts',(-3.85216762264019,-1.,0.193642806777747));
#53133=CARTESIAN_POINT('Ctrl Pts',(-3.85216762264019,1.,0.193642806777747));
#53134=CARTESIAN_POINT('Ctrl Pts',(-3.84475203347052,-1.,0.194909009460254));
#53135=CARTESIAN_POINT('Ctrl Pts',(-3.84475203347052,1.,0.194909009460254));
#53136=CARTESIAN_POINT('Ctrl Pts',(-3.83743910616265,-1.,0.196115198971889));
#53137=CARTESIAN_POINT('Ctrl Pts',(-3.83743910616265,1.,0.196115198971889));
#53138=CARTESIAN_POINT('Ctrl Pts',(-3.83026221776488,-1.,0.197260935827375));
#53139=CARTESIAN_POINT('Ctrl Pts',(-3.83026221776488,1.,0.197260935827375));
#53140=CARTESIAN_POINT('Ctrl Pts',(-3.82321127348981,-1.,0.19834261690047));
#53141=CARTESIAN_POINT('Ctrl Pts',(-3.82321127348981,1.,0.19834261690047));
#53142=CARTESIAN_POINT('Ctrl Pts',(-3.81620203429702,-1.,0.199351525297396));
#53143=CARTESIAN_POINT('Ctrl Pts',(-3.81620203429702,1.,0.199351525297396));
#53144=CARTESIAN_POINT('Ctrl Pts',(-3.80909529318501,-1.,0.20027467943329));
#53145=CARTESIAN_POINT('Ctrl Pts',(-3.80909529318501,1.,0.20027467943329));
#53146=CARTESIAN_POINT('Ctrl Pts',(-3.80175247447171,-1.,0.201097756307252));
#53147=CARTESIAN_POINT('Ctrl Pts',(-3.80175247447171,1.,0.201097756307252));
#53148=CARTESIAN_POINT('Ctrl Pts',(-3.79408354187274,-1.,0.201807533800799));
#53149=CARTESIAN_POINT('Ctrl Pts',(-3.79408354187274,1.,0.201807533800799));
#53150=CARTESIAN_POINT('Ctrl Pts',(-3.78609175019317,-1.,0.202394260512193));
#53151=CARTESIAN_POINT('Ctrl Pts',(-3.78609175019317,1.,0.202394260512193));
#53152=CARTESIAN_POINT('Ctrl Pts',(-3.77793553476879,-1.,0.202854729699196));
#53153=CARTESIAN_POINT('Ctrl Pts',(-3.77793553476879,1.,0.202854729699196));
#53154=CARTESIAN_POINT('Ctrl Pts',(-3.76992071595267,-1.,0.203192390045337));
#53155=CARTESIAN_POINT('Ctrl Pts',(-3.76992071595267,1.,0.203192390045337));
#53156=CARTESIAN_POINT('Ctrl Pts',(-3.76242717937273,-1.,0.203414634707646));
#53157=CARTESIAN_POINT('Ctrl Pts',(-3.76242717937273,1.,0.203414634707646));
#53158=CARTESIAN_POINT('Ctrl Pts',(-3.75585118707924,-1.,0.203530796848403));
#53159=CARTESIAN_POINT('Ctrl Pts',(-3.75585118707924,1.,0.203530796848403));
#53160=CARTESIAN_POINT('Ctrl Pts',(-3.75054693397716,-1.,0.203550035479097));
#53161=CARTESIAN_POINT('Ctrl Pts',(-3.75054693397716,1.,0.203550035479097));
#53162=CARTESIAN_POINT('Ctrl Pts',(-3.74675472018582,-1.,0.203478844530229));
#53163=CARTESIAN_POINT('Ctrl Pts',(-3.74675472018582,1.,0.203478844530229));
#53164=CARTESIAN_POINT('Ctrl Pts',(-3.7450208092684,-1.,0.203352057956055));
#53165=CARTESIAN_POINT('Ctrl Pts',(-3.7450208092684,1.,0.203352057956055));
#53166=CARTESIAN_POINT('Ctrl Pts',(-3.74446880195845,-1.,0.203218215747894));
#53167=CARTESIAN_POINT('Ctrl Pts',(-3.74446880195845,1.,0.203218215747894));
#53168=CARTESIAN_POINT('Ctrl Pts',(-3.74443319346666,-1.,0.20311176758786));
#53169=CARTESIAN_POINT('Ctrl Pts',(-3.74443319346666,1.,0.20311176758786));
#53170=CARTESIAN_POINT('Ctrl Pts',(-3.74449849461127,-1.,0.203054238699719));
#53171=CARTESIAN_POINT('Ctrl Pts',(-3.74449849461127,1.,0.203054238699719));
#53172=CARTESIAN_POINT('',(-4.19931119685982,1.,0.0760622897878236));
#53173=CARTESIAN_POINT('Ctrl Pts',(-4.19931119685982,1.,0.0760622897878236));
#53174=CARTESIAN_POINT('Ctrl Pts',(-4.19789138621624,1.,0.0767384596142195));
#53175=CARTESIAN_POINT('Ctrl Pts',(-4.19505112860624,1.,0.0780873956244402));
#53176=CARTESIAN_POINT('Ctrl Pts',(-4.19078883322483,1.,0.0801005887117603));
#53177=CARTESIAN_POINT('Ctrl Pts',(-4.1851019532944,1.,0.082764416438951));
#53178=CARTESIAN_POINT('Ctrl Pts',(-4.17798698669991,1.,0.0860600915552515));
#53179=CARTESIAN_POINT('Ctrl Pts',(-4.17086566491823,1.,0.0893215560850327));
#53180=CARTESIAN_POINT('Ctrl Pts',(-4.16373802265942,1.,0.092548667216769));
#53181=CARTESIAN_POINT('Ctrl Pts',(-4.15660412653006,1.,0.0957412403297067));
#53182=CARTESIAN_POINT('Ctrl Pts',(-4.1494640891762,1.,0.0988990478899811));
#53183=CARTESIAN_POINT('Ctrl Pts',(-4.14231804938737,1.,0.102021826577454));
#53184=CARTESIAN_POINT('Ctrl Pts',(-4.13516614458396,1.,0.105109286538864));
#53185=CARTESIAN_POINT('Ctrl Pts',(-4.12800848371386,1.,0.10816112052835));
#53186=CARTESIAN_POINT('Ctrl Pts',(-4.12084512502444,1.,0.111177012683377));
#53187=CARTESIAN_POINT('Ctrl Pts',(-4.11367603925313,1.,0.114156649609601));
#53188=CARTESIAN_POINT('Ctrl Pts',(-4.10650113382187,1.,0.117099722731704));
#53189=CARTESIAN_POINT('Ctrl Pts',(-4.09932031767243,1.,0.120005924388162));
#53190=CARTESIAN_POINT('Ctrl Pts',(-4.09213355850836,1.,0.122874946249119));
#53191=CARTESIAN_POINT('Ctrl Pts',(-4.08494093372315,1.,0.125706476822529));
#53192=CARTESIAN_POINT('Ctrl Pts',(-4.07774270738809,1.,0.128500200484814));
#53193=CARTESIAN_POINT('Ctrl Pts',(-4.07053931528579,1.,0.131255793548914));
#53194=CARTESIAN_POINT('Ctrl Pts',(-4.06333121018476,1.,0.133972916144225));
#53195=CARTESIAN_POINT('Ctrl Pts',(-4.05611873400122,1.,0.136651205046111));
#53196=CARTESIAN_POINT('Ctrl Pts',(-4.04890199238056,1.,0.139290267180059));
#53197=CARTESIAN_POINT('Ctrl Pts',(-4.04168069633842,1.,0.141889671485508));
#53198=CARTESIAN_POINT('Ctrl Pts',(-4.03445411510403,1.,0.144448947038352));
#53199=CARTESIAN_POINT('Ctrl Pts',(-4.02722143147048,1.,0.146967602878998));
#53200=CARTESIAN_POINT('Ctrl Pts',(-4.01998203715588,1.,0.149445144968707));
#53201=CARTESIAN_POINT('Ctrl Pts',(-4.01273584234684,1.,0.151881094022909));
#53202=CARTESIAN_POINT('Ctrl Pts',(-4.00548360245297,1.,0.15427500487231));
#53203=CARTESIAN_POINT('Ctrl Pts',(-3.99822717425869,1.,0.156626481393735));
#53204=CARTESIAN_POINT('Ctrl Pts',(-3.99096873945862,1.,0.158935123982796));
#53205=CARTESIAN_POINT('Ctrl Pts',(-3.98371010319866,1.,0.161200482186087));
#53206=CARTESIAN_POINT('Ctrl Pts',(-3.97645194630944,1.,0.163422004609999));
#53207=CARTESIAN_POINT('Ctrl Pts',(-3.9691931362141,1.,0.165598992851097));
#53208=CARTESIAN_POINT('Ctrl Pts',(-3.96192990160296,1.,0.167730547023312));
#53209=CARTESIAN_POINT('Ctrl Pts',(-3.95465744665263,1.,0.16981566637413));
#53210=CARTESIAN_POINT('Ctrl Pts',(-3.94737164900861,1.,0.171853355369233));
#53211=CARTESIAN_POINT('Ctrl Pts',(-3.94007083096214,1.,0.173842734974607));
#53212=CARTESIAN_POINT('Ctrl Pts',(-3.93275726771049,1.,0.175783136893872));
#53213=CARTESIAN_POINT('Ctrl Pts',(-3.92543942697672,1.,0.177674246152328));
#53214=CARTESIAN_POINT('Ctrl Pts',(-3.91812876180948,1.,0.179515885822894));
#53215=CARTESIAN_POINT('Ctrl Pts',(-3.91083557557193,1.,0.181307740731796));
#53216=CARTESIAN_POINT('Ctrl Pts',(-3.90356488555138,1.,0.183049081993193));
#53217=CARTESIAN_POINT('Ctrl Pts',(-3.89631300742633,1.,0.184738537728035));
#53218=CARTESIAN_POINT('Ctrl Pts',(-3.88906196725817,1.,0.186373724985263));
#53219=CARTESIAN_POINT('Ctrl Pts',(-3.88178563496187,1.,0.187951632512663));
#53220=CARTESIAN_POINT('Ctrl Pts',(-3.87445976418377,1.,0.189469253358254));
#53221=CARTESIAN_POINT('Ctrl Pts',(-3.8670715862477,1.,0.190924190418613));
#53222=CARTESIAN_POINT('Ctrl Pts',(-3.85962774407652,1.,0.192315153044979));
#53223=CARTESIAN_POINT('Ctrl Pts',(-3.85216762264019,1.,0.193642806777747));
#53224=CARTESIAN_POINT('Ctrl Pts',(-3.84475203347052,1.,0.194909009460254));
#53225=CARTESIAN_POINT('Ctrl Pts',(-3.83743910616265,1.,0.196115198971889));
#53226=CARTESIAN_POINT('Ctrl Pts',(-3.83026221776488,1.,0.197260935827375));
#53227=CARTESIAN_POINT('Ctrl Pts',(-3.82321127348981,1.,0.19834261690047));
#53228=CARTESIAN_POINT('Ctrl Pts',(-3.81620203429702,1.,0.199351525297396));
#53229=CARTESIAN_POINT('Ctrl Pts',(-3.80909529318501,1.,0.20027467943329));
#53230=CARTESIAN_POINT('Ctrl Pts',(-3.80175247447171,1.,0.201097756307252));
#53231=CARTESIAN_POINT('Ctrl Pts',(-3.79408354187274,1.,0.201807533800799));
#53232=CARTESIAN_POINT('Ctrl Pts',(-3.78609175019317,1.,0.202394260512193));
#53233=CARTESIAN_POINT('Ctrl Pts',(-3.77793553476879,1.,0.202854729699196));
#53234=CARTESIAN_POINT('Ctrl Pts',(-3.76992071595267,1.,0.203192390045337));
#53235=CARTESIAN_POINT('Ctrl Pts',(-3.76242717937273,1.,0.203414634707646));
#53236=CARTESIAN_POINT('Ctrl Pts',(-3.75585118707924,1.,0.203530796848403));
#53237=CARTESIAN_POINT('Ctrl Pts',(-3.75054693397716,1.,0.203550035479097));
#53238=CARTESIAN_POINT('Ctrl Pts',(-3.74703926501843,1.,0.203484186269314));
#53239=CARTESIAN_POINT('Ctrl Pts',(-3.74535749969262,1.,0.203375226874331));
#53240=CARTESIAN_POINT('Ctrl Pts',(-3.74471097893961,1.,0.203266610111264));
#53241=CARTESIAN_POINT('Ctrl Pts',(-3.74453008995129,1.,0.203188003947965));
#53242=CARTESIAN_POINT('Ctrl Pts',(-3.74449296982994,1.,0.203156094897896));
#53243=CARTESIAN_POINT('',(-4.19931119685982,0.,0.0760622897878236));
#53244=CARTESIAN_POINT('Ctrl Pts',(-3.74449849461127,-1.,-0.20305423869972));
#53245=CARTESIAN_POINT('Ctrl Pts',(-3.74449849461127,1.,-0.20305423869972));
#53246=CARTESIAN_POINT('Ctrl Pts',(-3.7444331934681,-1.,-0.203111767587923));
#53247=CARTESIAN_POINT('Ctrl Pts',(-3.7444331934681,1.,-0.203111767587923));
#53248=CARTESIAN_POINT('Ctrl Pts',(-3.7444688019622,-1.,-0.203218215748059));
#53249=CARTESIAN_POINT('Ctrl Pts',(-3.7444688019622,1.,-0.203218215748059));
#53250=CARTESIAN_POINT('Ctrl Pts',(-3.74502080927395,-1.,-0.203352057956297));
#53251=CARTESIAN_POINT('Ctrl Pts',(-3.74502080927395,1.,-0.203352057956297));
#53252=CARTESIAN_POINT('Ctrl Pts',(-3.7467547201908,-1.,-0.203478844530447));
#53253=CARTESIAN_POINT('Ctrl Pts',(-3.7467547201908,1.,-0.203478844530447));
#53254=CARTESIAN_POINT('Ctrl Pts',(-3.75054693397875,-1.,-0.203550035479166));
#53255=CARTESIAN_POINT('Ctrl Pts',(-3.75054693397875,1.,-0.203550035479166));
#53256=CARTESIAN_POINT('Ctrl Pts',(-3.75585118707734,-1.,-0.203530796848322));
#53257=CARTESIAN_POINT('Ctrl Pts',(-3.75585118707734,1.,-0.203530796848322));
#53258=CARTESIAN_POINT('Ctrl Pts',(-3.76242717936885,-1.,-0.203414634707478));
#53259=CARTESIAN_POINT('Ctrl Pts',(-3.76242717936885,1.,-0.203414634707478));
#53260=CARTESIAN_POINT('Ctrl Pts',(-3.7699207159487,-1.,-0.203192390045164));
#53261=CARTESIAN_POINT('Ctrl Pts',(-3.7699207159487,1.,-0.203192390045164));
#53262=CARTESIAN_POINT('Ctrl Pts',(-3.77793553476614,-1.,-0.202854729699081));
#53263=CARTESIAN_POINT('Ctrl Pts',(-3.77793553476614,1.,-0.202854729699081));
#53264=CARTESIAN_POINT('Ctrl Pts',(-3.78609175019242,-1.,-0.20239426051216));
#53265=CARTESIAN_POINT('Ctrl Pts',(-3.78609175019242,1.,-0.20239426051216));
#53266=CARTESIAN_POINT('Ctrl Pts',(-3.7940835418736,-1.,-0.201807533800837));
#53267=CARTESIAN_POINT('Ctrl Pts',(-3.7940835418736,1.,-0.201807533800837));
#53268=CARTESIAN_POINT('Ctrl Pts',(-3.80175247447337,-1.,-0.201097756307326));
#53269=CARTESIAN_POINT('Ctrl Pts',(-3.80175247447337,1.,-0.201097756307326));
#53270=CARTESIAN_POINT('Ctrl Pts',(-3.80909529318669,-1.,-0.200274679433364));
#53271=CARTESIAN_POINT('Ctrl Pts',(-3.80909529318669,1.,-0.200274679433364));
#53272=CARTESIAN_POINT('Ctrl Pts',(-3.81620203429815,-1.,-0.199351525297447));
#53273=CARTESIAN_POINT('Ctrl Pts',(-3.81620203429815,1.,-0.199351525297447));
#53274=CARTESIAN_POINT('Ctrl Pts',(-3.82321127349016,-1.,-0.198342616900486));
#53275=CARTESIAN_POINT('Ctrl Pts',(-3.82321127349016,1.,-0.198342616900486));
#53276=CARTESIAN_POINT('Ctrl Pts',(-3.83026221776456,-1.,-0.197260935827361));
#53277=CARTESIAN_POINT('Ctrl Pts',(-3.83026221776456,1.,-0.197260935827361));
#53278=CARTESIAN_POINT('Ctrl Pts',(-3.83743910616195,-1.,-0.196115198971859));
#53279=CARTESIAN_POINT('Ctrl Pts',(-3.83743910616195,1.,-0.196115198971859));
#53280=CARTESIAN_POINT('Ctrl Pts',(-3.84475203346977,-1.,-0.194909009460221));
#53281=CARTESIAN_POINT('Ctrl Pts',(-3.84475203346977,1.,-0.194909009460221));
#53282=CARTESIAN_POINT('Ctrl Pts',(-3.85216762263966,-1.,-0.193642806777723));
#53283=CARTESIAN_POINT('Ctrl Pts',(-3.85216762263966,1.,-0.193642806777723));
#53284=CARTESIAN_POINT('Ctrl Pts',(-3.85962774407633,-1.,-0.192315153044971));
#53285=CARTESIAN_POINT('Ctrl Pts',(-3.85962774407633,1.,-0.192315153044971));
#53286=CARTESIAN_POINT('Ctrl Pts',(-3.86707158624783,-1.,-0.19092419041862));
#53287=CARTESIAN_POINT('Ctrl Pts',(-3.86707158624783,1.,-0.19092419041862));
#53288=CARTESIAN_POINT('Ctrl Pts',(-3.87445976418412,-1.,-0.189469253358272));
#53289=CARTESIAN_POINT('Ctrl Pts',(-3.87445976418412,1.,-0.189469253358272));
#53290=CARTESIAN_POINT('Ctrl Pts',(-3.88178563496228,-1.,-0.187951632512685));
#53291=CARTESIAN_POINT('Ctrl Pts',(-3.88178563496228,1.,-0.187951632512685));
#53292=CARTESIAN_POINT('Ctrl Pts',(-3.88906196725848,-1.,-0.18637372498528));
#53293=CARTESIAN_POINT('Ctrl Pts',(-3.88906196725848,1.,-0.18637372498528));
#53294=CARTESIAN_POINT('Ctrl Pts',(-3.89631300742646,-1.,-0.184738537728043));
#53295=CARTESIAN_POINT('Ctrl Pts',(-3.89631300742646,1.,-0.184738537728043));
#53296=CARTESIAN_POINT('Ctrl Pts',(-3.90356488555132,-1.,-0.183049081993191));
#53297=CARTESIAN_POINT('Ctrl Pts',(-3.90356488555132,1.,-0.183049081993191));
#53298=CARTESIAN_POINT('Ctrl Pts',(-3.91083557557175,-1.,-0.181307740731786));
#53299=CARTESIAN_POINT('Ctrl Pts',(-3.91083557557175,1.,-0.181307740731786));
#53300=CARTESIAN_POINT('Ctrl Pts',(-3.91812876180926,-1.,-0.179515885822882));
#53301=CARTESIAN_POINT('Ctrl Pts',(-3.91812876180926,1.,-0.179515885822882));
#53302=CARTESIAN_POINT('Ctrl Pts',(-3.92543942697655,-1.,-0.177674246152317));
#53303=CARTESIAN_POINT('Ctrl Pts',(-3.92543942697655,1.,-0.177674246152317));
#53304=CARTESIAN_POINT('Ctrl Pts',(-3.93275726771042,-1.,-0.175783136893868));
#53305=CARTESIAN_POINT('Ctrl Pts',(-3.93275726771042,1.,-0.175783136893868));
#53306=CARTESIAN_POINT('Ctrl Pts',(-3.94007083096217,-1.,-0.17384273497461));
#53307=CARTESIAN_POINT('Ctrl Pts',(-3.94007083096217,1.,-0.17384273497461));
#53308=CARTESIAN_POINT('Ctrl Pts',(-3.94737164900868,-1.,-0.17185335536924));
#53309=CARTESIAN_POINT('Ctrl Pts',(-3.94737164900868,1.,-0.17185335536924));
#53310=CARTESIAN_POINT('Ctrl Pts',(-3.95465744665268,-1.,-0.169815666374139));
#53311=CARTESIAN_POINT('Ctrl Pts',(-3.95465744665268,1.,-0.169815666374139));
#53312=CARTESIAN_POINT('Ctrl Pts',(-3.96192990160296,-1.,-0.167730547023319));
#53313=CARTESIAN_POINT('Ctrl Pts',(-3.96192990160296,1.,-0.167730547023319));
#53314=CARTESIAN_POINT('Ctrl Pts',(-3.96919313621407,-1.,-0.165598992851102));
#53315=CARTESIAN_POINT('Ctrl Pts',(-3.96919313621407,1.,-0.165598992851102));
#53316=CARTESIAN_POINT('Ctrl Pts',(-3.97645194630943,-1.,-0.163422004609999));
#53317=CARTESIAN_POINT('Ctrl Pts',(-3.97645194630943,1.,-0.163422004609999));
#53318=CARTESIAN_POINT('Ctrl Pts',(-3.98371010319872,-1.,-0.161200482186085));
#53319=CARTESIAN_POINT('Ctrl Pts',(-3.98371010319872,1.,-0.161200482186085));
#53320=CARTESIAN_POINT('Ctrl Pts',(-3.99096873945878,-1.,-0.158935123982793));
#53321=CARTESIAN_POINT('Ctrl Pts',(-3.99096873945878,1.,-0.158935123982793));
#53322=CARTESIAN_POINT('Ctrl Pts',(-3.99822717425893,-1.,-0.156626481393734));
#53323=CARTESIAN_POINT('Ctrl Pts',(-3.99822717425893,1.,-0.156626481393734));
#53324=CARTESIAN_POINT('Ctrl Pts',(-4.00548360245319,-1.,-0.154275004872311));
#53325=CARTESIAN_POINT('Ctrl Pts',(-4.00548360245319,1.,-0.154275004872311));
#53326=CARTESIAN_POINT('Ctrl Pts',(-4.01273584234689,-1.,-0.151881094022911));
#53327=CARTESIAN_POINT('Ctrl Pts',(-4.01273584234689,1.,-0.151881094022911));
#53328=CARTESIAN_POINT('Ctrl Pts',(-4.01998203715564,-1.,-0.149445144968707));
#53329=CARTESIAN_POINT('Ctrl Pts',(-4.01998203715564,1.,-0.149445144968707));
#53330=CARTESIAN_POINT('Ctrl Pts',(-4.02722143146994,-1.,-0.146967602878994));
#53331=CARTESIAN_POINT('Ctrl Pts',(-4.02722143146994,1.,-0.146967602878994));
#53332=CARTESIAN_POINT('Ctrl Pts',(-4.03445411510333,-1.,-0.144448947038345));
#53333=CARTESIAN_POINT('Ctrl Pts',(-4.03445411510333,1.,-0.144448947038345));
#53334=CARTESIAN_POINT('Ctrl Pts',(-4.04168069633781,-1.,-0.1418896714855));
#53335=CARTESIAN_POINT('Ctrl Pts',(-4.04168069633781,1.,-0.1418896714855));
#53336=CARTESIAN_POINT('Ctrl Pts',(-4.04890199238036,-1.,-0.139290267180057));
#53337=CARTESIAN_POINT('Ctrl Pts',(-4.04890199238036,1.,-0.139290267180057));
#53338=CARTESIAN_POINT('Ctrl Pts',(-4.05611873400172,-1.,-0.136651205046119));
#53339=CARTESIAN_POINT('Ctrl Pts',(-4.05611873400172,1.,-0.136651205046119));
#53340=CARTESIAN_POINT('Ctrl Pts',(-4.06333121018596,-1.,-0.133972916144245));
#53341=CARTESIAN_POINT('Ctrl Pts',(-4.06333121018596,1.,-0.133972916144245));
#53342=CARTESIAN_POINT('Ctrl Pts',(-4.0705393152874,-1.,-0.13125579354894));
#53343=CARTESIAN_POINT('Ctrl Pts',(-4.0705393152874,1.,-0.13125579354894));
#53344=CARTESIAN_POINT('Ctrl Pts',(-4.07774270738954,-1.,-0.128500200484838));
#53345=CARTESIAN_POINT('Ctrl Pts',(-4.07774270738954,1.,-0.128500200484838));
#53346=CARTESIAN_POINT('Ctrl Pts',(-4.08494093372377,-1.,-0.12570647682254));
#53347=CARTESIAN_POINT('Ctrl Pts',(-4.08494093372377,1.,-0.12570647682254));
#53348=CARTESIAN_POINT('Ctrl Pts',(-4.09213355850756,-1.,-0.122874946249107));
#53349=CARTESIAN_POINT('Ctrl Pts',(-4.09213355850756,1.,-0.122874946249107));
#53350=CARTESIAN_POINT('Ctrl Pts',(-4.09932031767002,-1.,-0.120005924388124));
#53351=CARTESIAN_POINT('Ctrl Pts',(-4.09932031767002,1.,-0.120005924388124));
#53352=CARTESIAN_POINT('Ctrl Pts',(-4.10650113381833,-1.,-0.117099722731648));
#53353=CARTESIAN_POINT('Ctrl Pts',(-4.10650113381833,1.,-0.117099722731648));
#53354=CARTESIAN_POINT('Ctrl Pts',(-4.11367603924961,-1.,-0.114156649609546));
#53355=CARTESIAN_POINT('Ctrl Pts',(-4.11367603924961,1.,-0.114156649609546));
#53356=CARTESIAN_POINT('Ctrl Pts',(-4.1208451250225,-1.,-0.111177012683347));
#53357=CARTESIAN_POINT('Ctrl Pts',(-4.1208451250225,1.,-0.111177012683347));
#53358=CARTESIAN_POINT('Ctrl Pts',(-4.12800848371504,-1.,-0.108161120528369));
#53359=CARTESIAN_POINT('Ctrl Pts',(-4.12800848371504,1.,-0.108161120528369));
#53360=CARTESIAN_POINT('Ctrl Pts',(-4.13516614458895,-1.,-0.105109286538945));
#53361=CARTESIAN_POINT('Ctrl Pts',(-4.13516614458895,1.,-0.105109286538945));
#53362=CARTESIAN_POINT('Ctrl Pts',(-4.14231804939538,-1.,-0.102021826577584));
#53363=CARTESIAN_POINT('Ctrl Pts',(-4.14231804939538,1.,-0.102021826577584));
#53364=CARTESIAN_POINT('Ctrl Pts',(-4.14946408918485,-1.,-0.0988990478901226));
#53365=CARTESIAN_POINT('Ctrl Pts',(-4.14946408918485,1.,-0.0988990478901226));
#53366=CARTESIAN_POINT('Ctrl Pts',(-4.15660412653577,-1.,-0.0957412403298007));
#53367=CARTESIAN_POINT('Ctrl Pts',(-4.15660412653577,1.,-0.0957412403298007));
#53368=CARTESIAN_POINT('Ctrl Pts',(-4.16373802265839,-1.,-0.0925486672167531));
#53369=CARTESIAN_POINT('Ctrl Pts',(-4.16373802265839,1.,-0.0925486672167531));
#53370=CARTESIAN_POINT('Ctrl Pts',(-4.17086566490794,-1.,-0.0893215560848649));
#53371=CARTESIAN_POINT('Ctrl Pts',(-4.17086566490794,1.,-0.0893215560848649));
#53372=CARTESIAN_POINT('Ctrl Pts',(-4.17798698668094,-1.,-0.0860600915549397));
#53373=CARTESIAN_POINT('Ctrl Pts',(-4.17798698668094,1.,-0.0860600915549397));
#53374=CARTESIAN_POINT('Ctrl Pts',(-4.18510195327123,-1.,-0.0827644164385679));
#53375=CARTESIAN_POINT('Ctrl Pts',(-4.18510195327123,1.,-0.0827644164385679));
#53376=CARTESIAN_POINT('Ctrl Pts',(-4.19078883320504,-1.,-0.080100588711432));
#53377=CARTESIAN_POINT('Ctrl Pts',(-4.19078883320504,1.,-0.080100588711432));
#53378=CARTESIAN_POINT('Ctrl Pts',(-4.19505112859416,-1.,-0.0780873956242397));
#53379=CARTESIAN_POINT('Ctrl Pts',(-4.19505112859416,1.,-0.0780873956242397));
#53380=CARTESIAN_POINT('Ctrl Pts',(-4.1978913862118,-1.,-0.0767384596141464));
#53381=CARTESIAN_POINT('Ctrl Pts',(-4.1978913862118,1.,-0.0767384596141464));
#53382=CARTESIAN_POINT('Ctrl Pts',(-4.19931119685982,-1.,-0.0760622897878246));
#53383=CARTESIAN_POINT('Ctrl Pts',(-4.19931119685982,1.,-0.0760622897878246));
#53384=CARTESIAN_POINT('',(-3.74449296983004,1.,-0.2031560948961));
#53385=CARTESIAN_POINT('Ctrl Pts',(-3.74449296983004,-1.,-0.203156094896101));
#53386=CARTESIAN_POINT('Ctrl Pts',(-3.74449296983004,-0.666666666666667,
-0.203156094896101));
#53387=CARTESIAN_POINT('Ctrl Pts',(-3.74449296983004,-0.333333333333333,
-0.203156094896101));
#53388=CARTESIAN_POINT('Ctrl Pts',(-3.74449296983004,0.333333333333333,
-0.203156094896101));
#53389=CARTESIAN_POINT('Ctrl Pts',(-3.74449296983004,0.666666666666667,
-0.203156094896101));
#53390=CARTESIAN_POINT('Ctrl Pts',(-3.74449296983004,1.,-0.203156094896101));
#53391=CARTESIAN_POINT('',(-4.19931119685982,1.,-0.0760622897878246));
#53392=CARTESIAN_POINT('',(-4.19931119685982,0.,-0.0760622897878246));
#53393=CARTESIAN_POINT('Ctrl Pts',(-3.74449296983004,1.,-0.203156094896101));
#53394=CARTESIAN_POINT('Ctrl Pts',(-3.74453008995092,1.,-0.203188003946657));
#53395=CARTESIAN_POINT('Ctrl Pts',(-3.74471097893844,1.,-0.203266610110531));
#53396=CARTESIAN_POINT('Ctrl Pts',(-3.74535749969115,1.,-0.203375226874121));
#53397=CARTESIAN_POINT('Ctrl Pts',(-3.74703926501752,1.,-0.203484186269415));
#53398=CARTESIAN_POINT('Ctrl Pts',(-3.75054693397875,1.,-0.203550035479166));
#53399=CARTESIAN_POINT('Ctrl Pts',(-3.75585118707734,1.,-0.203530796848322));
#53400=CARTESIAN_POINT('Ctrl Pts',(-3.76242717936885,1.,-0.203414634707478));
#53401=CARTESIAN_POINT('Ctrl Pts',(-3.7699207159487,1.,-0.203192390045164));
#53402=CARTESIAN_POINT('Ctrl Pts',(-3.77793553476614,1.,-0.202854729699081));
#53403=CARTESIAN_POINT('Ctrl Pts',(-3.78609175019242,1.,-0.20239426051216));
#53404=CARTESIAN_POINT('Ctrl Pts',(-3.7940835418736,1.,-0.201807533800837));
#53405=CARTESIAN_POINT('Ctrl Pts',(-3.80175247447337,1.,-0.201097756307326));
#53406=CARTESIAN_POINT('Ctrl Pts',(-3.80909529318669,1.,-0.200274679433364));
#53407=CARTESIAN_POINT('Ctrl Pts',(-3.81620203429815,1.,-0.199351525297447));
#53408=CARTESIAN_POINT('Ctrl Pts',(-3.82321127349016,1.,-0.198342616900486));
#53409=CARTESIAN_POINT('Ctrl Pts',(-3.83026221776456,1.,-0.197260935827361));
#53410=CARTESIAN_POINT('Ctrl Pts',(-3.83743910616195,1.,-0.196115198971859));
#53411=CARTESIAN_POINT('Ctrl Pts',(-3.84475203346977,1.,-0.194909009460221));
#53412=CARTESIAN_POINT('Ctrl Pts',(-3.85216762263966,1.,-0.193642806777723));
#53413=CARTESIAN_POINT('Ctrl Pts',(-3.85962774407633,1.,-0.192315153044971));
#53414=CARTESIAN_POINT('Ctrl Pts',(-3.86707158624783,1.,-0.19092419041862));
#53415=CARTESIAN_POINT('Ctrl Pts',(-3.87445976418412,1.,-0.189469253358272));
#53416=CARTESIAN_POINT('Ctrl Pts',(-3.88178563496228,1.,-0.187951632512685));
#53417=CARTESIAN_POINT('Ctrl Pts',(-3.88906196725848,1.,-0.18637372498528));
#53418=CARTESIAN_POINT('Ctrl Pts',(-3.89631300742646,1.,-0.184738537728043));
#53419=CARTESIAN_POINT('Ctrl Pts',(-3.90356488555132,1.,-0.183049081993191));
#53420=CARTESIAN_POINT('Ctrl Pts',(-3.91083557557175,1.,-0.181307740731786));
#53421=CARTESIAN_POINT('Ctrl Pts',(-3.91812876180926,1.,-0.179515885822882));
#53422=CARTESIAN_POINT('Ctrl Pts',(-3.92543942697655,1.,-0.177674246152317));
#53423=CARTESIAN_POINT('Ctrl Pts',(-3.93275726771042,1.,-0.175783136893868));
#53424=CARTESIAN_POINT('Ctrl Pts',(-3.94007083096217,1.,-0.17384273497461));
#53425=CARTESIAN_POINT('Ctrl Pts',(-3.94737164900868,1.,-0.17185335536924));
#53426=CARTESIAN_POINT('Ctrl Pts',(-3.95465744665268,1.,-0.169815666374139));
#53427=CARTESIAN_POINT('Ctrl Pts',(-3.96192990160296,1.,-0.167730547023319));
#53428=CARTESIAN_POINT('Ctrl Pts',(-3.96919313621407,1.,-0.165598992851102));
#53429=CARTESIAN_POINT('Ctrl Pts',(-3.97645194630943,1.,-0.163422004609999));
#53430=CARTESIAN_POINT('Ctrl Pts',(-3.98371010319872,1.,-0.161200482186085));
#53431=CARTESIAN_POINT('Ctrl Pts',(-3.99096873945878,1.,-0.158935123982793));
#53432=CARTESIAN_POINT('Ctrl Pts',(-3.99822717425893,1.,-0.156626481393734));
#53433=CARTESIAN_POINT('Ctrl Pts',(-4.00548360245319,1.,-0.154275004872311));
#53434=CARTESIAN_POINT('Ctrl Pts',(-4.01273584234689,1.,-0.151881094022911));
#53435=CARTESIAN_POINT('Ctrl Pts',(-4.01998203715564,1.,-0.149445144968707));
#53436=CARTESIAN_POINT('Ctrl Pts',(-4.02722143146994,1.,-0.146967602878994));
#53437=CARTESIAN_POINT('Ctrl Pts',(-4.03445411510333,1.,-0.144448947038345));
#53438=CARTESIAN_POINT('Ctrl Pts',(-4.04168069633781,1.,-0.1418896714855));
#53439=CARTESIAN_POINT('Ctrl Pts',(-4.04890199238036,1.,-0.139290267180057));
#53440=CARTESIAN_POINT('Ctrl Pts',(-4.05611873400172,1.,-0.136651205046119));
#53441=CARTESIAN_POINT('Ctrl Pts',(-4.06333121018596,1.,-0.133972916144245));
#53442=CARTESIAN_POINT('Ctrl Pts',(-4.0705393152874,1.,-0.13125579354894));
#53443=CARTESIAN_POINT('Ctrl Pts',(-4.07774270738954,1.,-0.128500200484838));
#53444=CARTESIAN_POINT('Ctrl Pts',(-4.08494093372377,1.,-0.12570647682254));
#53445=CARTESIAN_POINT('Ctrl Pts',(-4.09213355850756,1.,-0.122874946249107));
#53446=CARTESIAN_POINT('Ctrl Pts',(-4.09932031767002,1.,-0.120005924388124));
#53447=CARTESIAN_POINT('Ctrl Pts',(-4.10650113381833,1.,-0.117099722731648));
#53448=CARTESIAN_POINT('Ctrl Pts',(-4.11367603924961,1.,-0.114156649609546));
#53449=CARTESIAN_POINT('Ctrl Pts',(-4.1208451250225,1.,-0.111177012683347));
#53450=CARTESIAN_POINT('Ctrl Pts',(-4.12800848371504,1.,-0.108161120528369));
#53451=CARTESIAN_POINT('Ctrl Pts',(-4.13516614458895,1.,-0.105109286538945));
#53452=CARTESIAN_POINT('Ctrl Pts',(-4.14231804939538,1.,-0.102021826577584));
#53453=CARTESIAN_POINT('Ctrl Pts',(-4.14946408918485,1.,-0.0988990478901226));
#53454=CARTESIAN_POINT('Ctrl Pts',(-4.15660412653577,1.,-0.0957412403298007));
#53455=CARTESIAN_POINT('Ctrl Pts',(-4.16373802265839,1.,-0.0925486672167531));
#53456=CARTESIAN_POINT('Ctrl Pts',(-4.17086566490794,1.,-0.0893215560848649));
#53457=CARTESIAN_POINT('Ctrl Pts',(-4.17798698668094,1.,-0.0860600915549397));
#53458=CARTESIAN_POINT('Ctrl Pts',(-4.18510195327123,1.,-0.0827644164385679));
#53459=CARTESIAN_POINT('Ctrl Pts',(-4.19078883320504,1.,-0.080100588711432));
#53460=CARTESIAN_POINT('Ctrl Pts',(-4.19505112859416,1.,-0.0780873956242397));
#53461=CARTESIAN_POINT('Ctrl Pts',(-4.1978913862118,1.,-0.0767384596141464));
#53462=CARTESIAN_POINT('Ctrl Pts',(-4.19931119685982,1.,-0.0760622897878246));
#53463=CARTESIAN_POINT('Origin',(-4.19931119685982,0.,-0.0760622897878246));
#53464=CARTESIAN_POINT('',(-4.19931119685982,1.,0.0760622897878236));
#53465=CARTESIAN_POINT('Origin',(0.,0.,0.));
#53466=CARTESIAN_POINT('',(-3.73017266276651,1.,-0.385112848330761));
#53467=CARTESIAN_POINT('Origin',(0.,1.,0.));
#53468=CARTESIAN_POINT('Ctrl Pts',(-3.73017266276651,1.,-0.385112848330762));
#53469=CARTESIAN_POINT('Ctrl Pts',(-3.73017266276651,0.666666666666667,
-0.385112848330762));
#53470=CARTESIAN_POINT('Ctrl Pts',(-3.73017266276651,0.333333333333333,
-0.385112848330762));
#53471=CARTESIAN_POINT('Ctrl Pts',(-3.73017266276651,-0.333333333333333,
-0.385112848330762));
#53472=CARTESIAN_POINT('Ctrl Pts',(-3.73017266276651,-0.666666666666667,
-0.385112848330762));
#53473=CARTESIAN_POINT('Ctrl Pts',(-3.73017266276651,-1.,-0.385112848330762));
#53474=CARTESIAN_POINT('Ctrl Pts',(-4.15950947128175,-1.,-0.581791163835815));
#53475=CARTESIAN_POINT('Ctrl Pts',(-4.15950947128175,1.,-0.581791163835815));
#53476=CARTESIAN_POINT('Ctrl Pts',(-4.1582129171283,-1.,-0.580901211463535));
#53477=CARTESIAN_POINT('Ctrl Pts',(-4.1582129171283,1.,-0.580901211463535));
#53478=CARTESIAN_POINT('Ctrl Pts',(-4.15561864788576,-1.,-0.579124568914235));
#53479=CARTESIAN_POINT('Ctrl Pts',(-4.15561864788576,1.,-0.579124568914235));
#53480=CARTESIAN_POINT('Ctrl Pts',(-4.151723761217,-1.,-0.576469391676688));
#53481=CARTESIAN_POINT('Ctrl Pts',(-4.151723761217,1.,-0.576469391676688));
#53482=CARTESIAN_POINT('Ctrl Pts',(-4.14652361068081,-1.,-0.572948736069522));
#53483=CARTESIAN_POINT('Ctrl Pts',(-4.14652361068081,1.,-0.572948736069522));
#53484=CARTESIAN_POINT('Ctrl Pts',(-4.14001179830547,-1.,-0.568580610189774));
#53485=CARTESIAN_POINT('Ctrl Pts',(-4.14001179830547,1.,-0.568580610189774));
#53486=CARTESIAN_POINT('Ctrl Pts',(-4.13348835727104,-1.,-0.564245279537148));
#53487=CARTESIAN_POINT('Ctrl Pts',(-4.13348835727104,1.,-0.564245279537148));
#53488=CARTESIAN_POINT('Ctrl Pts',(-4.12695329951961,-1.,-0.559942890594773));
#53489=CARTESIAN_POINT('Ctrl Pts',(-4.12695329951961,1.,-0.559942890594773));
#53490=CARTESIAN_POINT('Ctrl Pts',(-4.12040666195664,-1.,-0.555673636129977));
#53491=CARTESIAN_POINT('Ctrl Pts',(-4.12040666195664,1.,-0.555673636129977));
#53492=CARTESIAN_POINT('Ctrl Pts',(-4.11384852024721,-1.,-0.551437758497032));
#53493=CARTESIAN_POINT('Ctrl Pts',(-4.11384852024721,1.,-0.551437758497032));
#53494=CARTESIAN_POINT('Ctrl Pts',(-4.10727897027977,-1.,-0.547235539485637));
#53495=CARTESIAN_POINT('Ctrl Pts',(-4.10727897027977,1.,-0.547235539485637));
#53496=CARTESIAN_POINT('Ctrl Pts',(-4.10069810243979,-1.,-0.543067286877757));
#53497=CARTESIAN_POINT('Ctrl Pts',(-4.10069810243979,1.,-0.543067286877757));
#53498=CARTESIAN_POINT('Ctrl Pts',(-4.09410597627,-1.,-0.538933321179756));
#53499=CARTESIAN_POINT('Ctrl Pts',(-4.09410597627,1.,-0.538933321179756));
#53500=CARTESIAN_POINT('Ctrl Pts',(-4.08750259988885,-1.,-0.534833963477273));
#53501=CARTESIAN_POINT('Ctrl Pts',(-4.08750259988885,1.,-0.534833963477273));
#53502=CARTESIAN_POINT('Ctrl Pts',(-4.08088789536836,-1.,-0.530769518728571));
#53503=CARTESIAN_POINT('Ctrl Pts',(-4.08088789536836,1.,-0.530769518728571));
#53504=CARTESIAN_POINT('Ctrl Pts',(-4.07426172299847,-1.,-0.526740277227498));
#53505=CARTESIAN_POINT('Ctrl Pts',(-4.07426172299847,1.,-0.526740277227498));
#53506=CARTESIAN_POINT('Ctrl Pts',(-4.06762394471314,-1.,-0.522746528603107));
#53507=CARTESIAN_POINT('Ctrl Pts',(-4.06762394471314,1.,-0.522746528603107));
#53508=CARTESIAN_POINT('Ctrl Pts',(-4.06097448038013,-1.,-0.518788572336923));
#53509=CARTESIAN_POINT('Ctrl Pts',(-4.06097448038013,1.,-0.518788572336923));
#53510=CARTESIAN_POINT('Ctrl Pts',(-4.05431335771199,-1.,-0.514866728193017));
#53511=CARTESIAN_POINT('Ctrl Pts',(-4.05431335771199,1.,-0.514866728193017));
#53512=CARTESIAN_POINT('Ctrl Pts',(-4.04764078815447,-1.,-0.51098134921897));
#53513=CARTESIAN_POINT('Ctrl Pts',(-4.04764078815447,1.,-0.51098134921897));
#53514=CARTESIAN_POINT('Ctrl Pts',(-4.04095715148915,-1.,-0.507132823288136));
#53515=CARTESIAN_POINT('Ctrl Pts',(-4.04095715148915,1.,-0.507132823288136));
#53516=CARTESIAN_POINT('Ctrl Pts',(-4.03426284174272,-1.,-0.503321556915346));
#53517=CARTESIAN_POINT('Ctrl Pts',(-4.03426284174272,1.,-0.503321556915346));
#53518=CARTESIAN_POINT('Ctrl Pts',(-4.02755813980101,-1.,-0.499547962340821));
#53519=CARTESIAN_POINT('Ctrl Pts',(-4.02755813980101,1.,-0.499547962340821));
#53520=CARTESIAN_POINT('Ctrl Pts',(-4.02084308851832,-1.,-0.495812444326251));
#53521=CARTESIAN_POINT('Ctrl Pts',(-4.02084308851832,1.,-0.495812444326251));
#53522=CARTESIAN_POINT('Ctrl Pts',(-4.01411733503546,-1.,-0.492115383418018));
#53523=CARTESIAN_POINT('Ctrl Pts',(-4.01411733503546,1.,-0.492115383418018));
#53524=CARTESIAN_POINT('Ctrl Pts',(-4.0073800839099,-1.,-0.488457130424633));
#53525=CARTESIAN_POINT('Ctrl Pts',(-4.0073800839099,1.,-0.488457130424633));
#53526=CARTESIAN_POINT('Ctrl Pts',(-4.00063045119288,-1.,-0.484838042421835));
#53527=CARTESIAN_POINT('Ctrl Pts',(-4.00063045119288,1.,-0.484838042421835));
#53528=CARTESIAN_POINT('Ctrl Pts',(-3.99386775880679,-1.,-0.481258512209675));
#53529=CARTESIAN_POINT('Ctrl Pts',(-3.99386775880679,1.,-0.481258512209675));
#53530=CARTESIAN_POINT('Ctrl Pts',(-3.98709184306738,-1.,-0.477718999122027));
#53531=CARTESIAN_POINT('Ctrl Pts',(-3.98709184306738,1.,-0.477718999122027));
#53532=CARTESIAN_POINT('Ctrl Pts',(-3.98030338044409,-1.,-0.47422006101951));
#53533=CARTESIAN_POINT('Ctrl Pts',(-3.98030338044409,1.,-0.47422006101951));
#53534=CARTESIAN_POINT('Ctrl Pts',(-3.97350414289392,-1.,-0.470762379613439));
#53535=CARTESIAN_POINT('Ctrl Pts',(-3.97350414289392,1.,-0.470762379613439));
#53536=CARTESIAN_POINT('Ctrl Pts',(-3.9666962227393,-1.,-0.467346690880643));
#53537=CARTESIAN_POINT('Ctrl Pts',(-3.9666962227393,1.,-0.467346690880643));
#53538=CARTESIAN_POINT('Ctrl Pts',(-3.95988133243538,-1.,-0.463973722115733));
#53539=CARTESIAN_POINT('Ctrl Pts',(-3.95988133243538,1.,-0.463973722115733));
#53540=CARTESIAN_POINT('Ctrl Pts',(-3.95306005817364,-1.,-0.460644124429121));
#53541=CARTESIAN_POINT('Ctrl Pts',(-3.95306005817364,1.,-0.460644124429121));
#53542=CARTESIAN_POINT('Ctrl Pts',(-3.94623117206678,-1.,-0.457358410451683));
#53543=CARTESIAN_POINT('Ctrl Pts',(-3.94623117206678,1.,-0.457358410451683));
#53544=CARTESIAN_POINT('Ctrl Pts',(-3.93939080846298,-1.,-0.454116879027584));
#53545=CARTESIAN_POINT('Ctrl Pts',(-3.93939080846298,1.,-0.454116879027584));
#53546=CARTESIAN_POINT('Ctrl Pts',(-3.93253407403123,-1.,-0.450919768356348));
#53547=CARTESIAN_POINT('Ctrl Pts',(-3.93253407403123,1.,-0.450919768356348));
#53548=CARTESIAN_POINT('Ctrl Pts',(-3.92565674143416,-1.,-0.447767416837292));
#53549=CARTESIAN_POINT('Ctrl Pts',(-3.92565674143416,1.,-0.447767416837292));
#53550=CARTESIAN_POINT('Ctrl Pts',(-3.91875701610719,-1.,-0.444660430230591));
#53551=CARTESIAN_POINT('Ctrl Pts',(-3.91875701610719,1.,-0.444660430230591));
#53552=CARTESIAN_POINT('Ctrl Pts',(-3.91183704069153,-1.,-0.441599824524054));
#53553=CARTESIAN_POINT('Ctrl Pts',(-3.91183704069153,1.,-0.441599824524054));
#53554=CARTESIAN_POINT('Ctrl Pts',(-3.90490512938563,-1.,-0.438587235458249));
#53555=CARTESIAN_POINT('Ctrl Pts',(-3.90490512938563,1.,-0.438587235458249));
#53556=CARTESIAN_POINT('Ctrl Pts',(-3.89797256655462,-1.,-0.435624629433527));
#53557=CARTESIAN_POINT('Ctrl Pts',(-3.89797256655462,1.,-0.435624629433527));
#53558=CARTESIAN_POINT('Ctrl Pts',(-3.89104947940611,-1.,-0.432713929544458));
#53559=CARTESIAN_POINT('Ctrl Pts',(-3.89104947940611,1.,-0.432713929544458));
#53560=CARTESIAN_POINT('Ctrl Pts',(-3.88414070943341,-1.,-0.429856640579741));
#53561=CARTESIAN_POINT('Ctrl Pts',(-3.88414070943341,1.,-0.429856640579741));
#53562=CARTESIAN_POINT('Ctrl Pts',(-3.87724240306597,-1.,-0.427053541173457));
#53563=CARTESIAN_POINT('Ctrl Pts',(-3.87724240306597,1.,-0.427053541173457));
#53564=CARTESIAN_POINT('Ctrl Pts',(-3.87033643487851,-1.,-0.424304173195111));
#53565=CARTESIAN_POINT('Ctrl Pts',(-3.87033643487851,1.,-0.424304173195111));
#53566=CARTESIAN_POINT('Ctrl Pts',(-3.86339652542709,-1.,-0.421607423177534));
#53567=CARTESIAN_POINT('Ctrl Pts',(-3.86339652542709,1.,-0.421607423177534));
#53568=CARTESIAN_POINT('Ctrl Pts',(-3.85639825647996,-1.,-0.418962468086773));
#53569=CARTESIAN_POINT('Ctrl Pts',(-3.85639825647996,1.,-0.418962468086773));
#53570=CARTESIAN_POINT('Ctrl Pts',(-3.84932864157497,-1.,-0.416369678052907));
#53571=CARTESIAN_POINT('Ctrl Pts',(-3.84932864157497,1.,-0.416369678052907));
#53572=CARTESIAN_POINT('Ctrl Pts',(-3.84219403994762,-1.,-0.413831367016748));
#53573=CARTESIAN_POINT('Ctrl Pts',(-3.84219403994762,1.,-0.413831367016748));
#53574=CARTESIAN_POINT('Ctrl Pts',(-3.83503345578698,-1.,-0.411353038798518));
#53575=CARTESIAN_POINT('Ctrl Pts',(-3.83503345578698,1.,-0.411353038798518));
#53576=CARTESIAN_POINT('Ctrl Pts',(-3.82790724256471,-1.,-0.40894237144746));
#53577=CARTESIAN_POINT('Ctrl Pts',(-3.82790724256471,1.,-0.40894237144746));
#53578=CARTESIAN_POINT('Ctrl Pts',(-3.8208730391381,-1.,-0.406607038258985));
#53579=CARTESIAN_POINT('Ctrl Pts',(-3.8208730391381,1.,-0.406607038258985));
#53580=CARTESIAN_POINT('Ctrl Pts',(-3.81396374287793,-1.,-0.404352694628273));
#53581=CARTESIAN_POINT('Ctrl Pts',(-3.81396374287793,1.,-0.404352694628273));
#53582=CARTESIAN_POINT('Ctrl Pts',(-3.80716881962728,-1.,-0.402181320148436));
#53583=CARTESIAN_POINT('Ctrl Pts',(-3.80716881962728,1.,-0.402181320148436));
#53584=CARTESIAN_POINT('Ctrl Pts',(-3.80040370384546,-1.,-0.4000883465046));
#53585=CARTESIAN_POINT('Ctrl Pts',(-3.80040370384546,1.,-0.4000883465046));
#53586=CARTESIAN_POINT('Ctrl Pts',(-3.7935288716329,-1.,-0.398064818683969));
#53587=CARTESIAN_POINT('Ctrl Pts',(-3.7935288716329,1.,-0.398064818683969));
#53588=CARTESIAN_POINT('Ctrl Pts',(-3.78640521279313,-1.,-0.396103205334841));
#53589=CARTESIAN_POINT('Ctrl Pts',(-3.78640521279313,1.,-0.396103205334841));
#53590=CARTESIAN_POINT('Ctrl Pts',(-3.77894173114283,-1.,-0.394202481011499));
#53591=CARTESIAN_POINT('Ctrl Pts',(-3.77894173114283,1.,-0.394202481011499));
#53592=CARTESIAN_POINT('Ctrl Pts',(-3.77114011595967,-1.,-0.392372786223432));
#53593=CARTESIAN_POINT('Ctrl Pts',(-3.77114011595967,1.,-0.392372786223432));
#53594=CARTESIAN_POINT('Ctrl Pts',(-3.76315635033257,-1.,-0.39064207297956));
#53595=CARTESIAN_POINT('Ctrl Pts',(-3.76315635033257,1.,-0.39064207297956));
#53596=CARTESIAN_POINT('Ctrl Pts',(-3.75529302895152,-1.,-0.389054775898702));
#53597=CARTESIAN_POINT('Ctrl Pts',(-3.75529302895152,1.,-0.389054775898702));
#53598=CARTESIAN_POINT('Ctrl Pts',(-3.74792651696654,-1.,-0.387663020050836));
#53599=CARTESIAN_POINT('Ctrl Pts',(-3.74792651696654,1.,-0.387663020050836));
#53600=CARTESIAN_POINT('Ctrl Pts',(-3.74144965781276,-1.,-0.386519576222251));
#53601=CARTESIAN_POINT('Ctrl Pts',(-3.74144965781276,1.,-0.386519576222251));
#53602=CARTESIAN_POINT('Ctrl Pts',(-3.73621371845318,-1.,-0.385670806454566));
#53603=CARTESIAN_POINT('Ctrl Pts',(-3.73621371845318,1.,-0.385670806454566));
#53604=CARTESIAN_POINT('Ctrl Pts',(-3.73245705638843,-1.,-0.385147887988951));
#53605=CARTESIAN_POINT('Ctrl Pts',(-3.73245705638843,1.,-0.385147887988951));
#53606=CARTESIAN_POINT('Ctrl Pts',(-3.73072465900175,-1.,-0.385001870183213));
#53607=CARTESIAN_POINT('Ctrl Pts',(-3.73072465900175,1.,-0.385001870183213));
#53608=CARTESIAN_POINT('Ctrl Pts',(-3.73015851028356,-1.,-0.385047711603462));
#53609=CARTESIAN_POINT('Ctrl Pts',(-3.73015851028356,1.,-0.385047711603462));
#53610=CARTESIAN_POINT('Ctrl Pts',(-3.73010668803042,-1.,-0.385147278814642));
#53611=CARTESIAN_POINT('Ctrl Pts',(-3.73010668803042,1.,-0.385147278814642));
#53612=CARTESIAN_POINT('Ctrl Pts',(-3.73016218570874,-1.,-0.38521431477633));
#53613=CARTESIAN_POINT('Ctrl Pts',(-3.73016218570874,1.,-0.38521431477633));
#53614=CARTESIAN_POINT('',(-4.15950947128175,1.,-0.581791163835815));
#53615=CARTESIAN_POINT('Ctrl Pts',(-4.15950947128175,1.,-0.581791163835815));
#53616=CARTESIAN_POINT('Ctrl Pts',(-4.1582129171283,1.,-0.580901211463535));
#53617=CARTESIAN_POINT('Ctrl Pts',(-4.15561864788576,1.,-0.579124568914235));
#53618=CARTESIAN_POINT('Ctrl Pts',(-4.151723761217,1.,-0.576469391676688));
#53619=CARTESIAN_POINT('Ctrl Pts',(-4.14652361068081,1.,-0.572948736069522));
#53620=CARTESIAN_POINT('Ctrl Pts',(-4.14001179830547,1.,-0.568580610189774));
#53621=CARTESIAN_POINT('Ctrl Pts',(-4.13348835727104,1.,-0.564245279537148));
#53622=CARTESIAN_POINT('Ctrl Pts',(-4.12695329951961,1.,-0.559942890594773));
#53623=CARTESIAN_POINT('Ctrl Pts',(-4.12040666195664,1.,-0.555673636129977));
#53624=CARTESIAN_POINT('Ctrl Pts',(-4.11384852024721,1.,-0.551437758497032));
#53625=CARTESIAN_POINT('Ctrl Pts',(-4.10727897027977,1.,-0.547235539485637));
#53626=CARTESIAN_POINT('Ctrl Pts',(-4.10069810243979,1.,-0.543067286877757));
#53627=CARTESIAN_POINT('Ctrl Pts',(-4.09410597627,1.,-0.538933321179756));
#53628=CARTESIAN_POINT('Ctrl Pts',(-4.08750259988885,1.,-0.534833963477273));
#53629=CARTESIAN_POINT('Ctrl Pts',(-4.08088789536836,1.,-0.530769518728571));
#53630=CARTESIAN_POINT('Ctrl Pts',(-4.07426172299847,1.,-0.526740277227498));
#53631=CARTESIAN_POINT('Ctrl Pts',(-4.06762394471314,1.,-0.522746528603107));
#53632=CARTESIAN_POINT('Ctrl Pts',(-4.06097448038013,1.,-0.518788572336923));
#53633=CARTESIAN_POINT('Ctrl Pts',(-4.05431335771199,1.,-0.514866728193017));
#53634=CARTESIAN_POINT('Ctrl Pts',(-4.04764078815447,1.,-0.51098134921897));
#53635=CARTESIAN_POINT('Ctrl Pts',(-4.04095715148915,1.,-0.507132823288136));
#53636=CARTESIAN_POINT('Ctrl Pts',(-4.03426284174272,1.,-0.503321556915346));
#53637=CARTESIAN_POINT('Ctrl Pts',(-4.02755813980101,1.,-0.499547962340821));
#53638=CARTESIAN_POINT('Ctrl Pts',(-4.02084308851832,1.,-0.495812444326251));
#53639=CARTESIAN_POINT('Ctrl Pts',(-4.01411733503546,1.,-0.492115383418018));
#53640=CARTESIAN_POINT('Ctrl Pts',(-4.0073800839099,1.,-0.488457130424633));
#53641=CARTESIAN_POINT('Ctrl Pts',(-4.00063045119288,1.,-0.484838042421835));
#53642=CARTESIAN_POINT('Ctrl Pts',(-3.99386775880679,1.,-0.481258512209675));
#53643=CARTESIAN_POINT('Ctrl Pts',(-3.98709184306738,1.,-0.477718999122027));
#53644=CARTESIAN_POINT('Ctrl Pts',(-3.98030338044409,1.,-0.47422006101951));
#53645=CARTESIAN_POINT('Ctrl Pts',(-3.97350414289392,1.,-0.470762379613439));
#53646=CARTESIAN_POINT('Ctrl Pts',(-3.9666962227393,1.,-0.467346690880643));
#53647=CARTESIAN_POINT('Ctrl Pts',(-3.95988133243538,1.,-0.463973722115733));
#53648=CARTESIAN_POINT('Ctrl Pts',(-3.95306005817364,1.,-0.460644124429121));
#53649=CARTESIAN_POINT('Ctrl Pts',(-3.94623117206678,1.,-0.457358410451683));
#53650=CARTESIAN_POINT('Ctrl Pts',(-3.93939080846298,1.,-0.454116879027584));
#53651=CARTESIAN_POINT('Ctrl Pts',(-3.93253407403123,1.,-0.450919768356348));
#53652=CARTESIAN_POINT('Ctrl Pts',(-3.92565674143416,1.,-0.447767416837292));
#53653=CARTESIAN_POINT('Ctrl Pts',(-3.91875701610719,1.,-0.444660430230591));
#53654=CARTESIAN_POINT('Ctrl Pts',(-3.91183704069153,1.,-0.441599824524054));
#53655=CARTESIAN_POINT('Ctrl Pts',(-3.90490512938563,1.,-0.438587235458249));
#53656=CARTESIAN_POINT('Ctrl Pts',(-3.89797256655462,1.,-0.435624629433527));
#53657=CARTESIAN_POINT('Ctrl Pts',(-3.89104947940611,1.,-0.432713929544458));
#53658=CARTESIAN_POINT('Ctrl Pts',(-3.88414070943341,1.,-0.429856640579741));
#53659=CARTESIAN_POINT('Ctrl Pts',(-3.87724240306597,1.,-0.427053541173457));
#53660=CARTESIAN_POINT('Ctrl Pts',(-3.87033643487851,1.,-0.424304173195111));
#53661=CARTESIAN_POINT('Ctrl Pts',(-3.86339652542709,1.,-0.421607423177534));
#53662=CARTESIAN_POINT('Ctrl Pts',(-3.85639825647996,1.,-0.418962468086773));
#53663=CARTESIAN_POINT('Ctrl Pts',(-3.84932864157497,1.,-0.416369678052907));
#53664=CARTESIAN_POINT('Ctrl Pts',(-3.84219403994762,1.,-0.413831367016748));
#53665=CARTESIAN_POINT('Ctrl Pts',(-3.83503345578698,1.,-0.411353038798518));
#53666=CARTESIAN_POINT('Ctrl Pts',(-3.82790724256471,1.,-0.40894237144746));
#53667=CARTESIAN_POINT('Ctrl Pts',(-3.8208730391381,1.,-0.406607038258985));
#53668=CARTESIAN_POINT('Ctrl Pts',(-3.81396374287793,1.,-0.404352694628273));
#53669=CARTESIAN_POINT('Ctrl Pts',(-3.80716881962728,1.,-0.402181320148436));
#53670=CARTESIAN_POINT('Ctrl Pts',(-3.80040370384546,1.,-0.4000883465046));
#53671=CARTESIAN_POINT('Ctrl Pts',(-3.7935288716329,1.,-0.398064818683969));
#53672=CARTESIAN_POINT('Ctrl Pts',(-3.78640521279313,1.,-0.396103205334841));
#53673=CARTESIAN_POINT('Ctrl Pts',(-3.77894173114283,1.,-0.394202481011499));
#53674=CARTESIAN_POINT('Ctrl Pts',(-3.77114011595967,1.,-0.392372786223432));
#53675=CARTESIAN_POINT('Ctrl Pts',(-3.76315635033257,1.,-0.39064207297956));
#53676=CARTESIAN_POINT('Ctrl Pts',(-3.75529302895152,1.,-0.389054775898702));
#53677=CARTESIAN_POINT('Ctrl Pts',(-3.74792651696654,1.,-0.387663020050836));
#53678=CARTESIAN_POINT('Ctrl Pts',(-3.74144965781276,1.,-0.386519576222251));
#53679=CARTESIAN_POINT('Ctrl Pts',(-3.73621371845318,1.,-0.385670806454566));
#53680=CARTESIAN_POINT('Ctrl Pts',(-3.73273893363406,1.,-0.385187124634206));
#53681=CARTESIAN_POINT('Ctrl Pts',(-3.73106082862548,1.,-0.385031656499164));
#53682=CARTESIAN_POINT('Ctrl Pts',(-3.73040527621055,1.,-0.385037797881504));
#53683=CARTESIAN_POINT('Ctrl Pts',(-3.73021431755274,1.,-0.385087139000374));
#53684=CARTESIAN_POINT('Ctrl Pts',(-3.73017266276651,1.,-0.385112848330762));
#53685=CARTESIAN_POINT('',(-4.15950947128175,0.,-0.581791163835815));
#53686=CARTESIAN_POINT('Ctrl Pts',(-3.66663282329846,-1.,-0.7863229229206));
#53687=CARTESIAN_POINT('Ctrl Pts',(-3.66663282329846,1.,-0.7863229229206));
#53688=CARTESIAN_POINT('Ctrl Pts',(-3.66655932661986,-1.,-0.786369528183326));
#53689=CARTESIAN_POINT('Ctrl Pts',(-3.66655932661986,1.,-0.786369528183326));
#53690=CARTESIAN_POINT('Ctrl Pts',(-3.66657784455334,-1.,-0.786480236185696));
#53691=CARTESIAN_POINT('Ctrl Pts',(-3.66657784455334,1.,-0.786480236185696));
#53692=CARTESIAN_POINT('Ctrl Pts',(-3.66710211820482,-1.,-0.786698783542764));
#53693=CARTESIAN_POINT('Ctrl Pts',(-3.66710211820482,1.,-0.786698783542764));
#53694=CARTESIAN_POINT('Ctrl Pts',(-3.66879484801113,-1.,-0.787095252590501));
#53695=CARTESIAN_POINT('Ctrl Pts',(-3.66879484801113,1.,-0.787095252590501));
#53696=CARTESIAN_POINT('Ctrl Pts',(-3.67252923663655,-1.,-0.787758799995742));
#53697=CARTESIAN_POINT('Ctrl Pts',(-3.67252923663655,1.,-0.787758799995742));
#53698=CARTESIAN_POINT('Ctrl Pts',(-3.67777119516252,-1.,-0.788569566220285));
#53699=CARTESIAN_POINT('Ctrl Pts',(-3.67777119516252,1.,-0.788569566220285));
#53700=CARTESIAN_POINT('Ctrl Pts',(-3.68428439783905,-1.,-0.789483546064387));
#53701=CARTESIAN_POINT('Ctrl Pts',(-3.68428439783905,1.,-0.789483546064387));
#53702=CARTESIAN_POINT('Ctrl Pts',(-3.69172044327364,-1.,-0.790436284988787));
#53703=CARTESIAN_POINT('Ctrl Pts',(-3.69172044327364,1.,-0.790436284988787));
#53704=CARTESIAN_POINT('Ctrl Pts',(-3.69968940808721,-1.,-0.79135657569598));
#53705=CARTESIAN_POINT('Ctrl Pts',(-3.69968940808721,1.,-0.79135657569598));
#53706=CARTESIAN_POINT('Ctrl Pts',(-3.70781724021806,-1.,-0.792177688845818));
#53707=CARTESIAN_POINT('Ctrl Pts',(-3.70781724021806,1.,-0.792177688845818));
#53708=CARTESIAN_POINT('Ctrl Pts',(-3.71580242396124,-1.,-0.792848377370287));
#53709=CARTESIAN_POINT('Ctrl Pts',(-3.71580242396124,1.,-0.792848377370287));
#53710=CARTESIAN_POINT('Ctrl Pts',(-3.72348797293734,-1.,-0.793347023784205));
#53711=CARTESIAN_POINT('Ctrl Pts',(-3.72348797293734,1.,-0.793347023784205));
#53712=CARTESIAN_POINT('Ctrl Pts',(-3.73086914695805,-1.,-0.793682750269684));
#53713=CARTESIAN_POINT('Ctrl Pts',(-3.73086914695805,1.,-0.793682750269684));
#53714=CARTESIAN_POINT('Ctrl Pts',(-3.73803280541687,-1.,-0.793882700937017));
#53715=CARTESIAN_POINT('Ctrl Pts',(-3.73803280541687,1.,-0.793882700937017));
#53716=CARTESIAN_POINT('Ctrl Pts',(-3.74511357728861,-1.,-0.793982700459952));
#53717=CARTESIAN_POINT('Ctrl Pts',(-3.74511357728861,1.,-0.793982700459952));
#53718=CARTESIAN_POINT('Ctrl Pts',(-3.75224692493864,-1.,-0.794017347371377));
#53719=CARTESIAN_POINT('Ctrl Pts',(-3.75224692493864,1.,-0.794017347371377));
#53720=CARTESIAN_POINT('Ctrl Pts',(-3.75951468666257,-1.,-0.794008429134907));
#53721=CARTESIAN_POINT('Ctrl Pts',(-3.75951468666257,1.,-0.794008429134907));
#53722=CARTESIAN_POINT('Ctrl Pts',(-3.76692626931111,-1.,-0.793961083688991));
#53723=CARTESIAN_POINT('Ctrl Pts',(-3.76692626931111,1.,-0.793961083688991));
#53724=CARTESIAN_POINT('Ctrl Pts',(-3.77444863801212,-1.,-0.793870523787408));
#53725=CARTESIAN_POINT('Ctrl Pts',(-3.77444863801212,1.,-0.793870523787408));
#53726=CARTESIAN_POINT('Ctrl Pts',(-3.78202460377598,-1.,-0.7937262357813));
#53727=CARTESIAN_POINT('Ctrl Pts',(-3.78202460377598,1.,-0.7937262357813));
#53728=CARTESIAN_POINT('Ctrl Pts',(-3.78959439439235,-1.,-0.793516871680993));
#53729=CARTESIAN_POINT('Ctrl Pts',(-3.78959439439235,1.,-0.793516871680993));
#53730=CARTESIAN_POINT('Ctrl Pts',(-3.79711921389897,-1.,-0.793235612973273));
#53731=CARTESIAN_POINT('Ctrl Pts',(-3.79711921389897,1.,-0.793235612973273));
#53732=CARTESIAN_POINT('Ctrl Pts',(-3.80459229925637,-1.,-0.792882695234778));
#53733=CARTESIAN_POINT('Ctrl Pts',(-3.80459229925637,1.,-0.792882695234778));
#53734=CARTESIAN_POINT('Ctrl Pts',(-3.81202588694756,-1.,-0.792462483517634));
#53735=CARTESIAN_POINT('Ctrl Pts',(-3.81202588694756,1.,-0.792462483517634));
#53736=CARTESIAN_POINT('Ctrl Pts',(-3.81944345442249,-1.,-0.791981740718635));
#53737=CARTESIAN_POINT('Ctrl Pts',(-3.81944345442249,1.,-0.791981740718635));
#53738=CARTESIAN_POINT('Ctrl Pts',(-3.82687033899792,-1.,-0.791447528662369));
#53739=CARTESIAN_POINT('Ctrl Pts',(-3.82687033899792,1.,-0.791447528662369));
#53740=CARTESIAN_POINT('Ctrl Pts',(-3.83432392054786,-1.,-0.790865012705301));
#53741=CARTESIAN_POINT('Ctrl Pts',(-3.83432392054786,1.,-0.790865012705301));
#53742=CARTESIAN_POINT('Ctrl Pts',(-3.84180762342454,-1.,-0.790236124191242));
#53743=CARTESIAN_POINT('Ctrl Pts',(-3.84180762342454,1.,-0.790236124191242));
#53744=CARTESIAN_POINT('Ctrl Pts',(-3.84931637808894,-1.,-0.789560798155582));
#53745=CARTESIAN_POINT('Ctrl Pts',(-3.84931637808894,1.,-0.789560798155582));
#53746=CARTESIAN_POINT('Ctrl Pts',(-3.85683995872529,-1.,-0.788837734090672));
#53747=CARTESIAN_POINT('Ctrl Pts',(-3.85683995872529,1.,-0.788837734090672));
#53748=CARTESIAN_POINT('Ctrl Pts',(-3.86436702561345,-1.,-0.788065315093777));
#53749=CARTESIAN_POINT('Ctrl Pts',(-3.86436702561345,1.,-0.788065315093777));
#53750=CARTESIAN_POINT('Ctrl Pts',(-3.87188916600912,-1.,-0.787242527617999));
#53751=CARTESIAN_POINT('Ctrl Pts',(-3.87188916600912,1.,-0.787242527617999));
#53752=CARTESIAN_POINT('Ctrl Pts',(-3.8794040281819,-1.,-0.786369675812608));
#53753=CARTESIAN_POINT('Ctrl Pts',(-3.8794040281819,1.,-0.786369675812608));
#53754=CARTESIAN_POINT('Ctrl Pts',(-3.88691313167398,-1.,-0.78544789034073));
#53755=CARTESIAN_POINT('Ctrl Pts',(-3.88691313167398,1.,-0.78544789034073));
#53756=CARTESIAN_POINT('Ctrl Pts',(-3.89442039235103,-1.,-0.784478799358336));
#53757=CARTESIAN_POINT('Ctrl Pts',(-3.89442039235103,1.,-0.784478799358336));
#53758=CARTESIAN_POINT('Ctrl Pts',(-3.9019303904397,-1.,-0.783464141529081));
#53759=CARTESIAN_POINT('Ctrl Pts',(-3.9019303904397,1.,-0.783464141529081));
#53760=CARTESIAN_POINT('Ctrl Pts',(-3.90944671004542,-1.,-0.782405395622764));
#53761=CARTESIAN_POINT('Ctrl Pts',(-3.90944671004542,1.,-0.782405395622764));
#53762=CARTESIAN_POINT('Ctrl Pts',(-3.91697036054676,-1.,-0.781303428618366));
#53763=CARTESIAN_POINT('Ctrl Pts',(-3.91697036054676,1.,-0.781303428618366));
#53764=CARTESIAN_POINT('Ctrl Pts',(-3.92450058323823,-1.,-0.780158678615542));
#53765=CARTESIAN_POINT('Ctrl Pts',(-3.92450058323823,1.,-0.780158678615542));
#53766=CARTESIAN_POINT('Ctrl Pts',(-3.93203552473174,-1.,-0.778971308134821));
#53767=CARTESIAN_POINT('Ctrl Pts',(-3.93203552473174,1.,-0.778971308134821));
#53768=CARTESIAN_POINT('Ctrl Pts',(-3.93957296768103,-1.,-0.777741370568558));
#53769=CARTESIAN_POINT('Ctrl Pts',(-3.93957296768103,1.,-0.777741370568558));
#53770=CARTESIAN_POINT('Ctrl Pts',(-3.94711101619447,-1.,-0.776468966697921));
#53771=CARTESIAN_POINT('Ctrl Pts',(-3.94711101619447,1.,-0.776468966697921));
#53772=CARTESIAN_POINT('Ctrl Pts',(-3.9546488545231,-1.,-0.775154418039351));
#53773=CARTESIAN_POINT('Ctrl Pts',(-3.9546488545231,1.,-0.775154418039351));
#53774=CARTESIAN_POINT('Ctrl Pts',(-3.96218649639807,-1.,-0.773798212026565));
#53775=CARTESIAN_POINT('Ctrl Pts',(-3.96218649639807,1.,-0.773798212026565));
#53776=CARTESIAN_POINT('Ctrl Pts',(-3.96972446532772,-1.,-0.772400931772136));
#53777=CARTESIAN_POINT('Ctrl Pts',(-3.96972446532772,1.,-0.772400931772136));
#53778=CARTESIAN_POINT('Ctrl Pts',(-3.97726349165488,-1.,-0.770963190030471));
#53779=CARTESIAN_POINT('Ctrl Pts',(-3.97726349165488,1.,-0.770963190030471));
#53780=CARTESIAN_POINT('Ctrl Pts',(-3.98480422348451,-1.,-0.769485566245544));
#53781=CARTESIAN_POINT('Ctrl Pts',(-3.98480422348451,1.,-0.769485566245544));
#53782=CARTESIAN_POINT('Ctrl Pts',(-3.9923468788101,-1.,-0.767968531377915));
#53783=CARTESIAN_POINT('Ctrl Pts',(-3.9923468788101,1.,-0.767968531377915));
#53784=CARTESIAN_POINT('Ctrl Pts',(-3.99989129179622,-1.,-0.766412457136064));
#53785=CARTESIAN_POINT('Ctrl Pts',(-3.99989129179622,1.,-0.766412457136064));
#53786=CARTESIAN_POINT('Ctrl Pts',(-4.00743706791509,-1.,-0.764817648785197));
#53787=CARTESIAN_POINT('Ctrl Pts',(-4.00743706791509,1.,-0.764817648785197));
#53788=CARTESIAN_POINT('Ctrl Pts',(-4.01498370680496,-1.,-0.763184371182935));
#53789=CARTESIAN_POINT('Ctrl Pts',(-4.01498370680496,1.,-0.763184371182935));
#53790=CARTESIAN_POINT('Ctrl Pts',(-4.02253072741268,-1.,-0.761512875859804));
#53791=CARTESIAN_POINT('Ctrl Pts',(-4.02253072741268,1.,-0.761512875859804));
#53792=CARTESIAN_POINT('Ctrl Pts',(-4.03007781954412,-1.,-0.759803433243752));
#53793=CARTESIAN_POINT('Ctrl Pts',(-4.03007781954412,1.,-0.759803433243752));
#53794=CARTESIAN_POINT('Ctrl Pts',(-4.03762485803119,-1.,-0.758056338884944));
#53795=CARTESIAN_POINT('Ctrl Pts',(-4.03762485803119,1.,-0.758056338884944));
#53796=CARTESIAN_POINT('Ctrl Pts',(-4.04517182653997,-1.,-0.756271902369581));
#53797=CARTESIAN_POINT('Ctrl Pts',(-4.04517182653997,1.,-0.756271902369581));
#53798=CARTESIAN_POINT('Ctrl Pts',(-4.05271876687915,-1.,-0.754450441816078));
#53799=CARTESIAN_POINT('Ctrl Pts',(-4.05271876687915,1.,-0.754450441816078));
#53800=CARTESIAN_POINT('Ctrl Pts',(-4.06026572221515,-1.,-0.752592276483072));
#53801=CARTESIAN_POINT('Ctrl Pts',(-4.06026572221515,1.,-0.752592276483072));
#53802=CARTESIAN_POINT('Ctrl Pts',(-4.06781267242378,-1.,-0.750697720484036));
#53803=CARTESIAN_POINT('Ctrl Pts',(-4.06781267242378,1.,-0.750697720484036));
#53804=CARTESIAN_POINT('Ctrl Pts',(-4.07535951056152,-1.,-0.748767076680557));
#53805=CARTESIAN_POINT('Ctrl Pts',(-4.07535951056152,1.,-0.748767076680557));
#53806=CARTESIAN_POINT('Ctrl Pts',(-4.08290608095642,-1.,-0.746800631492315));
#53807=CARTESIAN_POINT('Ctrl Pts',(-4.08290608095642,1.,-0.746800631492315));
#53808=CARTESIAN_POINT('Ctrl Pts',(-4.09045220253573,-1.,-0.7447986497065));
#53809=CARTESIAN_POINT('Ctrl Pts',(-4.09045220253573,1.,-0.7447986497065));
#53810=CARTESIAN_POINT('Ctrl Pts',(-4.09799769702611,-1.,-0.742761369689841));
#53811=CARTESIAN_POINT('Ctrl Pts',(-4.09799769702611,1.,-0.742761369689841));
#53812=CARTESIAN_POINT('Ctrl Pts',(-4.10554241757547,-1.,-0.740688998553377));
#53813=CARTESIAN_POINT('Ctrl Pts',(-4.10554241757547,1.,-0.740688998553377));
#53814=CARTESIAN_POINT('Ctrl Pts',(-4.11308626951927,-1.,-0.738581708225844));
#53815=CARTESIAN_POINT('Ctrl Pts',(-4.11308626951927,1.,-0.738581708225844));
#53816=CARTESIAN_POINT('Ctrl Pts',(-4.120629196238,-1.,-0.736439634331345));
#53817=CARTESIAN_POINT('Ctrl Pts',(-4.120629196238,1.,-0.736439634331345));
#53818=CARTESIAN_POINT('Ctrl Pts',(-4.12666277570844,-1.,-0.734698226764092));
#53819=CARTESIAN_POINT('Ctrl Pts',(-4.12666277570844,1.,-0.734698226764092));
#53820=CARTESIAN_POINT('Ctrl Pts',(-4.13118752795207,-1.,-0.733376589323546));
#53821=CARTESIAN_POINT('Ctrl Pts',(-4.13118752795207,1.,-0.733376589323546));
#53822=CARTESIAN_POINT('Ctrl Pts',(-4.1342038373684,-1.,-0.732488575135159));
#53823=CARTESIAN_POINT('Ctrl Pts',(-4.1342038373684,1.,-0.732488575135159));
#53824=CARTESIAN_POINT('Ctrl Pts',(-4.13571194405636,-1.,-0.73204283740062));
#53825=CARTESIAN_POINT('Ctrl Pts',(-4.13571194405636,1.,-0.73204283740062));
#53826=CARTESIAN_POINT('',(-3.66661143271685,1.,-0.786422660831985));
#53827=CARTESIAN_POINT('Ctrl Pts',(-3.66661143271685,-1.,-0.786422660831985));
#53828=CARTESIAN_POINT('Ctrl Pts',(-3.66661143271685,-0.666666666666667,
-0.786422660831985));
#53829=CARTESIAN_POINT('Ctrl Pts',(-3.66661143271685,-0.333333333333333,
-0.786422660831985));
#53830=CARTESIAN_POINT('Ctrl Pts',(-3.66661143271685,0.333333333333333,
-0.786422660831985));
#53831=CARTESIAN_POINT('Ctrl Pts',(-3.66661143271685,0.666666666666667,
-0.786422660831985));
#53832=CARTESIAN_POINT('Ctrl Pts',(-3.66661143271685,1.,-0.786422660831985));
#53833=CARTESIAN_POINT('',(-4.13571194405636,1.,-0.73204283740062));
#53834=CARTESIAN_POINT('',(-4.13571194405636,0.,-0.73204283740062));
#53835=CARTESIAN_POINT('Ctrl Pts',(-3.66661143271685,1.,-0.786422660831985));
#53836=CARTESIAN_POINT('Ctrl Pts',(-3.6666431041522,1.,-0.786459983895432));
#53837=CARTESIAN_POINT('Ctrl Pts',(-3.66680946938292,1.,-0.786565919558984));
#53838=CARTESIAN_POINT('Ctrl Pts',(-3.66743103898702,1.,-0.786774337198062));
#53839=CARTESIAN_POINT('Ctrl Pts',(-3.66907505398677,1.,-0.787145041181545));
#53840=CARTESIAN_POINT('Ctrl Pts',(-3.67252923663655,1.,-0.787758799995742));
#53841=CARTESIAN_POINT('Ctrl Pts',(-3.67777119516252,1.,-0.788569566220285));
#53842=CARTESIAN_POINT('Ctrl Pts',(-3.68428439783905,1.,-0.789483546064387));
#53843=CARTESIAN_POINT('Ctrl Pts',(-3.69172044327364,1.,-0.790436284988787));
#53844=CARTESIAN_POINT('Ctrl Pts',(-3.69968940808721,1.,-0.79135657569598));
#53845=CARTESIAN_POINT('Ctrl Pts',(-3.70781724021806,1.,-0.792177688845818));
#53846=CARTESIAN_POINT('Ctrl Pts',(-3.71580242396124,1.,-0.792848377370287));
#53847=CARTESIAN_POINT('Ctrl Pts',(-3.72348797293734,1.,-0.793347023784205));
#53848=CARTESIAN_POINT('Ctrl Pts',(-3.73086914695805,1.,-0.793682750269684));
#53849=CARTESIAN_POINT('Ctrl Pts',(-3.73803280541687,1.,-0.793882700937017));
#53850=CARTESIAN_POINT('Ctrl Pts',(-3.74511357728861,1.,-0.793982700459952));
#53851=CARTESIAN_POINT('Ctrl Pts',(-3.75224692493864,1.,-0.794017347371377));
#53852=CARTESIAN_POINT('Ctrl Pts',(-3.75951468666257,1.,-0.794008429134907));
#53853=CARTESIAN_POINT('Ctrl Pts',(-3.76692626931111,1.,-0.793961083688991));
#53854=CARTESIAN_POINT('Ctrl Pts',(-3.77444863801212,1.,-0.793870523787408));
#53855=CARTESIAN_POINT('Ctrl Pts',(-3.78202460377598,1.,-0.7937262357813));
#53856=CARTESIAN_POINT('Ctrl Pts',(-3.78959439439235,1.,-0.793516871680993));
#53857=CARTESIAN_POINT('Ctrl Pts',(-3.79711921389897,1.,-0.793235612973273));
#53858=CARTESIAN_POINT('Ctrl Pts',(-3.80459229925637,1.,-0.792882695234778));
#53859=CARTESIAN_POINT('Ctrl Pts',(-3.81202588694756,1.,-0.792462483517634));
#53860=CARTESIAN_POINT('Ctrl Pts',(-3.81944345442249,1.,-0.791981740718635));
#53861=CARTESIAN_POINT('Ctrl Pts',(-3.82687033899792,1.,-0.791447528662369));
#53862=CARTESIAN_POINT('Ctrl Pts',(-3.83432392054786,1.,-0.790865012705301));
#53863=CARTESIAN_POINT('Ctrl Pts',(-3.84180762342454,1.,-0.790236124191242));
#53864=CARTESIAN_POINT('Ctrl Pts',(-3.84931637808894,1.,-0.789560798155582));
#53865=CARTESIAN_POINT('Ctrl Pts',(-3.85683995872529,1.,-0.788837734090672));
#53866=CARTESIAN_POINT('Ctrl Pts',(-3.86436702561345,1.,-0.788065315093777));
#53867=CARTESIAN_POINT('Ctrl Pts',(-3.87188916600912,1.,-0.787242527617999));
#53868=CARTESIAN_POINT('Ctrl Pts',(-3.8794040281819,1.,-0.786369675812608));
#53869=CARTESIAN_POINT('Ctrl Pts',(-3.88691313167398,1.,-0.78544789034073));
#53870=CARTESIAN_POINT('Ctrl Pts',(-3.89442039235103,1.,-0.784478799358336));
#53871=CARTESIAN_POINT('Ctrl Pts',(-3.9019303904397,1.,-0.783464141529081));
#53872=CARTESIAN_POINT('Ctrl Pts',(-3.90944671004542,1.,-0.782405395622764));
#53873=CARTESIAN_POINT('Ctrl Pts',(-3.91697036054676,1.,-0.781303428618366));
#53874=CARTESIAN_POINT('Ctrl Pts',(-3.92450058323823,1.,-0.780158678615542));
#53875=CARTESIAN_POINT('Ctrl Pts',(-3.93203552473174,1.,-0.778971308134821));
#53876=CARTESIAN_POINT('Ctrl Pts',(-3.93957296768103,1.,-0.777741370568558));
#53877=CARTESIAN_POINT('Ctrl Pts',(-3.94711101619447,1.,-0.776468966697921));
#53878=CARTESIAN_POINT('Ctrl Pts',(-3.9546488545231,1.,-0.775154418039351));
#53879=CARTESIAN_POINT('Ctrl Pts',(-3.96218649639807,1.,-0.773798212026565));
#53880=CARTESIAN_POINT('Ctrl Pts',(-3.96972446532772,1.,-0.772400931772136));
#53881=CARTESIAN_POINT('Ctrl Pts',(-3.97726349165488,1.,-0.770963190030471));
#53882=CARTESIAN_POINT('Ctrl Pts',(-3.98480422348451,1.,-0.769485566245544));
#53883=CARTESIAN_POINT('Ctrl Pts',(-3.9923468788101,1.,-0.767968531377915));
#53884=CARTESIAN_POINT('Ctrl Pts',(-3.99989129179622,1.,-0.766412457136064));
#53885=CARTESIAN_POINT('Ctrl Pts',(-4.00743706791509,1.,-0.764817648785197));
#53886=CARTESIAN_POINT('Ctrl Pts',(-4.01498370680496,1.,-0.763184371182935));
#53887=CARTESIAN_POINT('Ctrl Pts',(-4.02253072741268,1.,-0.761512875859804));
#53888=CARTESIAN_POINT('Ctrl Pts',(-4.03007781954412,1.,-0.759803433243752));
#53889=CARTESIAN_POINT('Ctrl Pts',(-4.03762485803119,1.,-0.758056338884944));
#53890=CARTESIAN_POINT('Ctrl Pts',(-4.04517182653997,1.,-0.756271902369581));
#53891=CARTESIAN_POINT('Ctrl Pts',(-4.05271876687915,1.,-0.754450441816078));
#53892=CARTESIAN_POINT('Ctrl Pts',(-4.06026572221515,1.,-0.752592276483072));
#53893=CARTESIAN_POINT('Ctrl Pts',(-4.06781267242378,1.,-0.750697720484036));
#53894=CARTESIAN_POINT('Ctrl Pts',(-4.07535951056152,1.,-0.748767076680557));
#53895=CARTESIAN_POINT('Ctrl Pts',(-4.08290608095642,1.,-0.746800631492315));
#53896=CARTESIAN_POINT('Ctrl Pts',(-4.09045220253573,1.,-0.7447986497065));
#53897=CARTESIAN_POINT('Ctrl Pts',(-4.09799769702611,1.,-0.742761369689841));
#53898=CARTESIAN_POINT('Ctrl Pts',(-4.10554241757547,1.,-0.740688998553377));
#53899=CARTESIAN_POINT('Ctrl Pts',(-4.11308626951927,1.,-0.738581708225844));
#53900=CARTESIAN_POINT('Ctrl Pts',(-4.120629196238,1.,-0.736439634331345));
#53901=CARTESIAN_POINT('Ctrl Pts',(-4.12666277570844,1.,-0.734698226764092));
#53902=CARTESIAN_POINT('Ctrl Pts',(-4.13118752795207,1.,-0.733376589323546));
#53903=CARTESIAN_POINT('Ctrl Pts',(-4.1342038373684,1.,-0.732488575135159));
#53904=CARTESIAN_POINT('Ctrl Pts',(-4.13571194405636,1.,-0.73204283740062));
#53905=CARTESIAN_POINT('Origin',(-4.13571194405636,0.,-0.73204283740062));
#53906=CARTESIAN_POINT('',(-4.15950947128175,1.,-0.581791163835815));
#53907=CARTESIAN_POINT('Origin',(0.,0.,0.));
#53908=CARTESIAN_POINT('',(-3.62400312501245,1.,-0.963899035117248));
#53909=CARTESIAN_POINT('Origin',(0.,1.,0.));
#53910=CARTESIAN_POINT('Ctrl Pts',(-3.62400312501245,1.,-0.963899035117249));
#53911=CARTESIAN_POINT('Ctrl Pts',(-3.62400312501245,0.666666666666667,
-0.963899035117249));
#53912=CARTESIAN_POINT('Ctrl Pts',(-3.62400312501245,0.333333333333333,
-0.963899035117249));
#53913=CARTESIAN_POINT('Ctrl Pts',(-3.62400312501245,-0.333333333333333,
-0.963899035117249));
#53914=CARTESIAN_POINT('Ctrl Pts',(-3.62400312501246,-0.666666666666667,
-0.963899035117249));
#53915=CARTESIAN_POINT('Ctrl Pts',(-3.62400312501246,-1.,-0.963899035117249));
#53916=CARTESIAN_POINT('Ctrl Pts',(-4.01728681790024,-1.,-1.22531898815164));
#53917=CARTESIAN_POINT('Ctrl Pts',(-4.01728681790024,1.,-1.22531898815164));
#53918=CARTESIAN_POINT('Ctrl Pts',(-4.0161454457032,-1.,-1.22423716681447));
#53919=CARTESIAN_POINT('Ctrl Pts',(-4.0161454457032,1.,-1.22423716681447));
#53920=CARTESIAN_POINT('Ctrl Pts',(-4.01386104434674,-1.,-1.22207656456199));
#53921=CARTESIAN_POINT('Ctrl Pts',(-4.01386104434674,1.,-1.22207656456199));
#53922=CARTESIAN_POINT('Ctrl Pts',(-4.01042947142681,-1.,-1.21884478244983));
#53923=CARTESIAN_POINT('Ctrl Pts',(-4.01042947142681,1.,-1.21884478244983));
#53924=CARTESIAN_POINT('Ctrl Pts',(-4.00584409524937,-1.,-1.21455398918813));
#53925=CARTESIAN_POINT('Ctrl Pts',(-4.00584409524937,1.,-1.21455398918813));
#53926=CARTESIAN_POINT('Ctrl Pts',(-4.00009577952534,-1.,-1.20922097030107));
#53927=CARTESIAN_POINT('Ctrl Pts',(-4.00009577952534,1.,-1.20922097030107));
#53928=CARTESIAN_POINT('Ctrl Pts',(-3.99433084800649,-1.,-1.2039185237544));
#53929=CARTESIAN_POINT('Ctrl Pts',(-3.99433084800649,1.,-1.2039185237544));
#53930=CARTESIAN_POINT('Ctrl Pts',(-3.98854928957287,-1.,-1.19864679609596));
#53931=CARTESIAN_POINT('Ctrl Pts',(-3.98854928957287,1.,-1.19864679609596));
#53932=CARTESIAN_POINT('Ctrl Pts',(-3.98275111052015,-1.,-1.19340598349307));
#53933=CARTESIAN_POINT('Ctrl Pts',(-3.98275111052015,1.,-1.19340598349307));
#53934=CARTESIAN_POINT('Ctrl Pts',(-3.97693634766926,-1.,-1.18819633715285));
#53935=CARTESIAN_POINT('Ctrl Pts',(-3.97693634766926,1.,-1.18819633715285));
#53936=CARTESIAN_POINT('Ctrl Pts',(-3.9711050516465,-1.,-1.18301815039596));
#53937=CARTESIAN_POINT('Ctrl Pts',(-3.9711050516465,1.,-1.18301815039596));
#53938=CARTESIAN_POINT('Ctrl Pts',(-3.96525726357682,-1.,-1.17787174135445));
#53939=CARTESIAN_POINT('Ctrl Pts',(-3.96525726357682,1.,-1.17787174135445));
#53940=CARTESIAN_POINT('Ctrl Pts',(-3.95939299213164,-1.,-1.17275743590327));
#53941=CARTESIAN_POINT('Ctrl Pts',(-3.95939299213164,1.,-1.17275743590327));
#53942=CARTESIAN_POINT('Ctrl Pts',(-3.95351219510062,-1.,-1.16767555244495));
#53943=CARTESIAN_POINT('Ctrl Pts',(-3.95351219510062,1.,-1.16767555244495));
#53944=CARTESIAN_POINT('Ctrl Pts',(-3.9476147478092,-1.,-1.16262637999261));
#53945=CARTESIAN_POINT('Ctrl Pts',(-3.9476147478092,1.,-1.16262637999261));
#53946=CARTESIAN_POINT('Ctrl Pts',(-3.94170046685542,-1.,-1.1576101834106));
#53947=CARTESIAN_POINT('Ctrl Pts',(-3.94170046685542,1.,-1.1576101834106));
#53948=CARTESIAN_POINT('Ctrl Pts',(-3.9357691705651,-1.,-1.1526272271639));
#53949=CARTESIAN_POINT('Ctrl Pts',(-3.9357691705651,1.,-1.1526272271639));
#53950=CARTESIAN_POINT('Ctrl Pts',(-3.92982073294334,-1.,-1.14767779451147));
#53951=CARTESIAN_POINT('Ctrl Pts',(-3.92982073294334,1.,-1.14767779451147));
#53952=CARTESIAN_POINT('Ctrl Pts',(-3.92385513133937,-1.,-1.14276220561575));
#53953=CARTESIAN_POINT('Ctrl Pts',(-3.92385513133937,1.,-1.14276220561575));
#53954=CARTESIAN_POINT('Ctrl Pts',(-3.91787251936688,-1.,-1.13788084225511));
#53955=CARTESIAN_POINT('Ctrl Pts',(-3.91787251936688,1.,-1.13788084225511));
#53956=CARTESIAN_POINT('Ctrl Pts',(-3.91187321145495,-1.,-1.13303414693849));
#53957=CARTESIAN_POINT('Ctrl Pts',(-3.91187321145495,1.,-1.13303414693849));
#53958=CARTESIAN_POINT('Ctrl Pts',(-3.90585753318622,-1.,-1.12822258281518));
#53959=CARTESIAN_POINT('Ctrl Pts',(-3.90585753318622,1.,-1.12822258281518));
#53960=CARTESIAN_POINT('Ctrl Pts',(-3.89982569749978,-1.,-1.12344660099029));
#53961=CARTESIAN_POINT('Ctrl Pts',(-3.89982569749978,1.,-1.12344660099029));
#53962=CARTESIAN_POINT('Ctrl Pts',(-3.89377768340362,-1.,-1.11870660794609));
#53963=CARTESIAN_POINT('Ctrl Pts',(-3.89377768340362,1.,-1.11870660794609));
#53964=CARTESIAN_POINT('Ctrl Pts',(-3.88771308285229,-1.,-1.11400292434447));
#53965=CARTESIAN_POINT('Ctrl Pts',(-3.88771308285229,1.,-1.11400292434447));
#53966=CARTESIAN_POINT('Ctrl Pts',(-3.88163105531791,-1.,-1.10933577224029));
#53967=CARTESIAN_POINT('Ctrl Pts',(-3.88163105531791,1.,-1.10933577224029));
#53968=CARTESIAN_POINT('Ctrl Pts',(-3.87553067187566,-1.,-1.10470536603303));
#53969=CARTESIAN_POINT('Ctrl Pts',(-3.87553067187566,1.,-1.10470536603303));
#53970=CARTESIAN_POINT('Ctrl Pts',(-3.86941120134872,-1.,-1.10011198761202));
#53971=CARTESIAN_POINT('Ctrl Pts',(-3.86941120134872,1.,-1.10011198761202));
#53972=CARTESIAN_POINT('Ctrl Pts',(-3.86327241021242,-1.,-1.09555606505012));
#53973=CARTESIAN_POINT('Ctrl Pts',(-3.86327241021242,1.,-1.09555606505012));
#53974=CARTESIAN_POINT('Ctrl Pts',(-3.85711487933911,-1.,-1.09103825516288));
#53975=CARTESIAN_POINT('Ctrl Pts',(-3.85711487933911,1.,-1.09103825516288));
#53976=CARTESIAN_POINT('Ctrl Pts',(-3.8509402522269,-1.,-1.08655950846377));
#53977=CARTESIAN_POINT('Ctrl Pts',(-3.8509402522269,1.,-1.08655950846377));
#53978=CARTESIAN_POINT('Ctrl Pts',(-3.84475048030615,-1.,-1.08212087917986));
#53979=CARTESIAN_POINT('Ctrl Pts',(-3.84475048030615,1.,-1.08212087917986));
#53980=CARTESIAN_POINT('Ctrl Pts',(-3.83854714117486,-1.,-1.07772335353856));
#53981=CARTESIAN_POINT('Ctrl Pts',(-3.83854714117486,1.,-1.07772335353856));
#53982=CARTESIAN_POINT('Ctrl Pts',(-3.83233071195145,-1.,-1.0733676663346));
#53983=CARTESIAN_POINT('Ctrl Pts',(-3.83233071195145,1.,-1.0733676663346));
#53984=CARTESIAN_POINT('Ctrl Pts',(-3.82609989967278,-1.,-1.0690541318036));
#53985=CARTESIAN_POINT('Ctrl Pts',(-3.82609989967278,1.,-1.0690541318036));
#53986=CARTESIAN_POINT('Ctrl Pts',(-3.81985083953012,-1.,-1.06478244038931));
#53987=CARTESIAN_POINT('Ctrl Pts',(-3.81985083953012,1.,-1.06478244038931));
#53988=CARTESIAN_POINT('Ctrl Pts',(-3.81357866117485,-1.,-1.06055206187298));
#53989=CARTESIAN_POINT('Ctrl Pts',(-3.81357866117485,1.,-1.06055206187298));
#53990=CARTESIAN_POINT('Ctrl Pts',(-3.80727913637784,-1.,-1.05636266918643));
#53991=CARTESIAN_POINT('Ctrl Pts',(-3.80727913637784,1.,-1.05636266918643));
#53992=CARTESIAN_POINT('Ctrl Pts',(-3.80095039790678,-1.,-1.05221457990015));
#53993=CARTESIAN_POINT('Ctrl Pts',(-3.80095039790678,1.,-1.05221457990015));
#53994=CARTESIAN_POINT('Ctrl Pts',(-3.79459440308793,-1.,-1.04810913267641));
#53995=CARTESIAN_POINT('Ctrl Pts',(-3.79459440308793,1.,-1.04810913267641));
#53996=CARTESIAN_POINT('Ctrl Pts',(-3.78821910787195,-1.,-1.04404924374426));
#53997=CARTESIAN_POINT('Ctrl Pts',(-3.78821910787195,1.,-1.04404924374426));
#53998=CARTESIAN_POINT('Ctrl Pts',(-3.78183535008192,-1.,-1.04003862055804));
#53999=CARTESIAN_POINT('Ctrl Pts',(-3.78183535008192,1.,-1.04003862055804));
#54000=CARTESIAN_POINT('Ctrl Pts',(-3.77545283140445,-1.,-1.03608074678013));
#54001=CARTESIAN_POINT('Ctrl Pts',(-3.77545283140445,1.,-1.03608074678013));
#54002=CARTESIAN_POINT('Ctrl Pts',(-3.76907609832522,-1.,-1.0321778660492));
#54003=CARTESIAN_POINT('Ctrl Pts',(-3.76907609832522,1.,-1.0321778660492));
#54004=CARTESIAN_POINT('Ctrl Pts',(-3.76270122291232,-1.,-1.02833014458181));
#54005=CARTESIAN_POINT('Ctrl Pts',(-3.76270122291232,1.,-1.02833014458181));
#54006=CARTESIAN_POINT('Ctrl Pts',(-3.75631037456194,-1.,-1.0245342944466));
#54007=CARTESIAN_POINT('Ctrl Pts',(-3.75631037456194,1.,-1.0245342944466));
#54008=CARTESIAN_POINT('Ctrl Pts',(-3.74987777155834,-1.,-1.02078510487428));
#54009=CARTESIAN_POINT('Ctrl Pts',(-3.74987777155834,1.,-1.02078510487428));
#54010=CARTESIAN_POINT('Ctrl Pts',(-3.74337942504959,-1.,-1.01707794311079));
#54011=CARTESIAN_POINT('Ctrl Pts',(-3.74337942504959,1.,-1.01707794311079));
#54012=CARTESIAN_POINT('Ctrl Pts',(-3.73680245055734,-1.,-1.01341114319903));
#54013=CARTESIAN_POINT('Ctrl Pts',(-3.73680245055734,1.,-1.01341114319903));
#54014=CARTESIAN_POINT('Ctrl Pts',(-3.73015276704426,-1.,-1.00978798539496));
#54015=CARTESIAN_POINT('Ctrl Pts',(-3.73015276704426,1.,-1.00978798539496));
#54016=CARTESIAN_POINT('Ctrl Pts',(-3.72346803750595,-1.,-1.0062200073571));
#54017=CARTESIAN_POINT('Ctrl Pts',(-3.72346803750595,1.,-1.0062200073571));
#54018=CARTESIAN_POINT('Ctrl Pts',(-3.71680667125118,-1.,-1.00272423396822));
#54019=CARTESIAN_POINT('Ctrl Pts',(-3.71680667125118,1.,-1.00272423396822));
#54020=CARTESIAN_POINT('Ctrl Pts',(-3.71022439713938,-1.,-0.99931726075653));
#54021=CARTESIAN_POINT('Ctrl Pts',(-3.71022439713938,1.,-0.99931726075653));
#54022=CARTESIAN_POINT('Ctrl Pts',(-3.70375282282138,-1.,-0.996009819772518));
#54023=CARTESIAN_POINT('Ctrl Pts',(-3.70375282282138,1.,-0.996009819772518));
#54024=CARTESIAN_POINT('Ctrl Pts',(-3.69738123415662,-1.,-0.99280221833201));
#54025=CARTESIAN_POINT('Ctrl Pts',(-3.69738123415662,1.,-0.99280221833201));
#54026=CARTESIAN_POINT('Ctrl Pts',(-3.69102682138846,-1.,-0.989676715398558));
#54027=CARTESIAN_POINT('Ctrl Pts',(-3.69102682138846,1.,-0.989676715398558));
#54028=CARTESIAN_POINT('Ctrl Pts',(-3.68455317926068,-1.,-0.986602639863837));
#54029=CARTESIAN_POINT('Ctrl Pts',(-3.68455317926068,1.,-0.986602639863837));
#54030=CARTESIAN_POINT('Ctrl Pts',(-3.67782408841715,-1.,-0.983550791470419));
#54031=CARTESIAN_POINT('Ctrl Pts',(-3.67782408841715,1.,-0.983550791470419));
#54032=CARTESIAN_POINT('Ctrl Pts',(-3.67074983340361,-1.,-0.980505922458267));
#54033=CARTESIAN_POINT('Ctrl Pts',(-3.67074983340361,1.,-0.980505922458267));
#54034=CARTESIAN_POINT('Ctrl Pts',(-3.66333049637475,-1.,-0.977478312751618));
#54035=CARTESIAN_POINT('Ctrl Pts',(-3.66333049637475,1.,-0.977478312751618));
#54036=CARTESIAN_POINT('Ctrl Pts',(-3.65571576735126,-1.,-0.974519971354848));
#54037=CARTESIAN_POINT('Ctrl Pts',(-3.65571576735126,1.,-0.974519971354848));
#54038=CARTESIAN_POINT('Ctrl Pts',(-3.64819756447455,-1.,-0.971722122061341));
#54039=CARTESIAN_POINT('Ctrl Pts',(-3.64819756447455,1.,-0.971722122061341));
#54040=CARTESIAN_POINT('Ctrl Pts',(-3.64113946505766,-1.,-0.969195124675865));
#54041=CARTESIAN_POINT('Ctrl Pts',(-3.64113946505766,1.,-0.969195124675865));
#54042=CARTESIAN_POINT('Ctrl Pts',(-3.63492122081143,-1.,-0.967052554541385));
#54043=CARTESIAN_POINT('Ctrl Pts',(-3.63492122081143,1.,-0.967052554541385));
#54044=CARTESIAN_POINT('Ctrl Pts',(-3.62988252139846,-1.,-0.965395153165293));
#54045=CARTESIAN_POINT('Ctrl Pts',(-3.62988252139846,1.,-0.965395153165293));
#54046=CARTESIAN_POINT('Ctrl Pts',(-3.62625391254797,-1.,-0.964291001273287));
#54047=CARTESIAN_POINT('Ctrl Pts',(-3.62625391254797,1.,-0.964291001273287));
#54048=CARTESIAN_POINT('Ctrl Pts',(-3.6245656860652,-1.,-0.963875774530619));
#54049=CARTESIAN_POINT('Ctrl Pts',(-3.6245656860652,1.,-0.963875774530619));
#54050=CARTESIAN_POINT('Ctrl Pts',(-3.62399933639914,-1.,-0.963832486395051));
#54051=CARTESIAN_POINT('Ctrl Pts',(-3.62399933639914,1.,-0.963832486395051));
#54052=CARTESIAN_POINT('Ctrl Pts',(-3.62393257642052,-1.,-0.963922720982193));
#54053=CARTESIAN_POINT('Ctrl Pts',(-3.62393257642052,1.,-0.963922720982193));
#54054=CARTESIAN_POINT('Ctrl Pts',(-3.62397690409552,-1.,-0.963997613369571));
#54055=CARTESIAN_POINT('Ctrl Pts',(-3.62397690409552,1.,-0.963997613369571));
#54056=CARTESIAN_POINT('',(-4.01728681790024,1.,-1.22531898815164));
#54057=CARTESIAN_POINT('Ctrl Pts',(-4.01728681790024,1.,-1.22531898815164));
#54058=CARTESIAN_POINT('Ctrl Pts',(-4.0161454457032,1.,-1.22423716681447));
#54059=CARTESIAN_POINT('Ctrl Pts',(-4.01386104434674,1.,-1.22207656456199));
#54060=CARTESIAN_POINT('Ctrl Pts',(-4.01042947142681,1.,-1.21884478244983));
#54061=CARTESIAN_POINT('Ctrl Pts',(-4.00584409524937,1.,-1.21455398918813));
#54062=CARTESIAN_POINT('Ctrl Pts',(-4.00009577952534,1.,-1.20922097030107));
#54063=CARTESIAN_POINT('Ctrl Pts',(-3.99433084800649,1.,-1.2039185237544));
#54064=CARTESIAN_POINT('Ctrl Pts',(-3.98854928957287,1.,-1.19864679609596));
#54065=CARTESIAN_POINT('Ctrl Pts',(-3.98275111052015,1.,-1.19340598349307));
#54066=CARTESIAN_POINT('Ctrl Pts',(-3.97693634766926,1.,-1.18819633715285));
#54067=CARTESIAN_POINT('Ctrl Pts',(-3.9711050516465,1.,-1.18301815039596));
#54068=CARTESIAN_POINT('Ctrl Pts',(-3.96525726357682,1.,-1.17787174135445));
#54069=CARTESIAN_POINT('Ctrl Pts',(-3.95939299213164,1.,-1.17275743590327));
#54070=CARTESIAN_POINT('Ctrl Pts',(-3.95351219510062,1.,-1.16767555244495));
#54071=CARTESIAN_POINT('Ctrl Pts',(-3.9476147478092,1.,-1.16262637999261));
#54072=CARTESIAN_POINT('Ctrl Pts',(-3.94170046685542,1.,-1.1576101834106));
#54073=CARTESIAN_POINT('Ctrl Pts',(-3.9357691705651,1.,-1.1526272271639));
#54074=CARTESIAN_POINT('Ctrl Pts',(-3.92982073294334,1.,-1.14767779451147));
#54075=CARTESIAN_POINT('Ctrl Pts',(-3.92385513133937,1.,-1.14276220561575));
#54076=CARTESIAN_POINT('Ctrl Pts',(-3.91787251936688,1.,-1.13788084225511));
#54077=CARTESIAN_POINT('Ctrl Pts',(-3.91187321145495,1.,-1.13303414693849));
#54078=CARTESIAN_POINT('Ctrl Pts',(-3.90585753318622,1.,-1.12822258281518));
#54079=CARTESIAN_POINT('Ctrl Pts',(-3.89982569749978,1.,-1.12344660099029));
#54080=CARTESIAN_POINT('Ctrl Pts',(-3.89377768340362,1.,-1.11870660794609));
#54081=CARTESIAN_POINT('Ctrl Pts',(-3.88771308285229,1.,-1.11400292434447));
#54082=CARTESIAN_POINT('Ctrl Pts',(-3.88163105531791,1.,-1.10933577224029));
#54083=CARTESIAN_POINT('Ctrl Pts',(-3.87553067187566,1.,-1.10470536603303));
#54084=CARTESIAN_POINT('Ctrl Pts',(-3.86941120134872,1.,-1.10011198761202));
#54085=CARTESIAN_POINT('Ctrl Pts',(-3.86327241021242,1.,-1.09555606505012));
#54086=CARTESIAN_POINT('Ctrl Pts',(-3.85711487933911,1.,-1.09103825516288));
#54087=CARTESIAN_POINT('Ctrl Pts',(-3.8509402522269,1.,-1.08655950846377));
#54088=CARTESIAN_POINT('Ctrl Pts',(-3.84475048030615,1.,-1.08212087917986));
#54089=CARTESIAN_POINT('Ctrl Pts',(-3.83854714117486,1.,-1.07772335353856));
#54090=CARTESIAN_POINT('Ctrl Pts',(-3.83233071195145,1.,-1.0733676663346));
#54091=CARTESIAN_POINT('Ctrl Pts',(-3.82609989967278,1.,-1.0690541318036));
#54092=CARTESIAN_POINT('Ctrl Pts',(-3.81985083953012,1.,-1.06478244038931));
#54093=CARTESIAN_POINT('Ctrl Pts',(-3.81357866117485,1.,-1.06055206187298));
#54094=CARTESIAN_POINT('Ctrl Pts',(-3.80727913637784,1.,-1.05636266918643));
#54095=CARTESIAN_POINT('Ctrl Pts',(-3.80095039790678,1.,-1.05221457990015));
#54096=CARTESIAN_POINT('Ctrl Pts',(-3.79459440308793,1.,-1.04810913267641));
#54097=CARTESIAN_POINT('Ctrl Pts',(-3.78821910787195,1.,-1.04404924374426));
#54098=CARTESIAN_POINT('Ctrl Pts',(-3.78183535008192,1.,-1.04003862055804));
#54099=CARTESIAN_POINT('Ctrl Pts',(-3.77545283140445,1.,-1.03608074678013));
#54100=CARTESIAN_POINT('Ctrl Pts',(-3.76907609832522,1.,-1.0321778660492));
#54101=CARTESIAN_POINT('Ctrl Pts',(-3.76270122291232,1.,-1.02833014458181));
#54102=CARTESIAN_POINT('Ctrl Pts',(-3.75631037456194,1.,-1.0245342944466));
#54103=CARTESIAN_POINT('Ctrl Pts',(-3.74987777155834,1.,-1.02078510487428));
#54104=CARTESIAN_POINT('Ctrl Pts',(-3.74337942504959,1.,-1.01707794311079));
#54105=CARTESIAN_POINT('Ctrl Pts',(-3.73680245055734,1.,-1.01341114319903));
#54106=CARTESIAN_POINT('Ctrl Pts',(-3.73015276704426,1.,-1.00978798539496));
#54107=CARTESIAN_POINT('Ctrl Pts',(-3.72346803750595,1.,-1.0062200073571));
#54108=CARTESIAN_POINT('Ctrl Pts',(-3.71680667125118,1.,-1.00272423396822));
#54109=CARTESIAN_POINT('Ctrl Pts',(-3.71022439713938,1.,-0.99931726075653));
#54110=CARTESIAN_POINT('Ctrl Pts',(-3.70375282282138,1.,-0.996009819772518));
#54111=CARTESIAN_POINT('Ctrl Pts',(-3.69738123415662,1.,-0.99280221833201));
#54112=CARTESIAN_POINT('Ctrl Pts',(-3.69102682138846,1.,-0.989676715398558));
#54113=CARTESIAN_POINT('Ctrl Pts',(-3.68455317926068,1.,-0.986602639863837));
#54114=CARTESIAN_POINT('Ctrl Pts',(-3.67782408841715,1.,-0.983550791470419));
#54115=CARTESIAN_POINT('Ctrl Pts',(-3.67074983340361,1.,-0.980505922458267));
#54116=CARTESIAN_POINT('Ctrl Pts',(-3.66333049637475,1.,-0.977478312751618));
#54117=CARTESIAN_POINT('Ctrl Pts',(-3.65571576735126,1.,-0.974519971354848));
#54118=CARTESIAN_POINT('Ctrl Pts',(-3.64819756447455,1.,-0.971722122061341));
#54119=CARTESIAN_POINT('Ctrl Pts',(-3.64113946505766,1.,-0.969195124675865));
#54120=CARTESIAN_POINT('Ctrl Pts',(-3.63492122081143,1.,-0.967052554541385));
#54121=CARTESIAN_POINT('Ctrl Pts',(-3.62988252139846,1.,-0.965395153165293));
#54122=CARTESIAN_POINT('Ctrl Pts',(-3.62652618145335,1.,-0.964373850166458));
#54123=CARTESIAN_POINT('Ctrl Pts',(-3.62489305727662,1.,-0.963957782642843));
#54124=CARTESIAN_POINT('Ctrl Pts',(-3.62424461507588,1.,-0.963861297423241));
#54125=CARTESIAN_POINT('Ctrl Pts',(-3.6240482887845,1.,-0.963880158555582));
#54126=CARTESIAN_POINT('Ctrl Pts',(-3.62400312501245,1.,-0.963899035117249));
#54127=CARTESIAN_POINT('',(-4.01728681790024,0.,-1.22531898815164));
#54128=CARTESIAN_POINT('Ctrl Pts',(-3.49848248301936,-1.,-1.35022972712301));
#54129=CARTESIAN_POINT('Ctrl Pts',(-3.49848248301936,1.,-1.35022972712301));
#54130=CARTESIAN_POINT('Ctrl Pts',(-3.4984026005375,-1.,-1.35026426118402));
#54131=CARTESIAN_POINT('Ctrl Pts',(-3.4984026005375,1.,-1.35026426118402));
#54132=CARTESIAN_POINT('Ctrl Pts',(-3.49840357193736,-1.,-1.35037650303019));
#54133=CARTESIAN_POINT('Ctrl Pts',(-3.49840357193736,1.,-1.35037650303019));
#54134=CARTESIAN_POINT('Ctrl Pts',(-3.49888720257132,-1.,-1.35067437417483));
#54135=CARTESIAN_POINT('Ctrl Pts',(-3.49888720257132,1.,-1.35067437417483));
#54136=CARTESIAN_POINT('Ctrl Pts',(-3.5004970706414,-1.,-1.3513307633124));
#54137=CARTESIAN_POINT('Ctrl Pts',(-3.5004970706414,1.,-1.3513307633124));
#54138=CARTESIAN_POINT('Ctrl Pts',(-3.50408168106261,-1.,-1.35257032843486));
#54139=CARTESIAN_POINT('Ctrl Pts',(-3.50408168106261,1.,-1.35257032843486));
#54140=CARTESIAN_POINT('Ctrl Pts',(-3.50913227059999,-1.,-1.35419113575956));
#54141=CARTESIAN_POINT('Ctrl Pts',(-3.50913227059999,1.,-1.35419113575956));
#54142=CARTESIAN_POINT('Ctrl Pts',(-3.51542230699556,-1.,-1.35611275237152));
#54143=CARTESIAN_POINT('Ctrl Pts',(-3.51542230699556,1.,-1.35611275237152));
#54144=CARTESIAN_POINT('Ctrl Pts',(-3.52261776116748,-1.,-1.35821701528836));
#54145=CARTESIAN_POINT('Ctrl Pts',(-3.52261776116748,1.,-1.35821701528836));
#54146=CARTESIAN_POINT('Ctrl Pts',(-3.530344649616,-1.,-1.36037259643734));
#54147=CARTESIAN_POINT('Ctrl Pts',(-3.530344649616,1.,-1.36037259643734));
#54148=CARTESIAN_POINT('Ctrl Pts',(-3.53824396424961,-1.,-1.36245507339307));
#54149=CARTESIAN_POINT('Ctrl Pts',(-3.53824396424961,1.,-1.36245507339307));
#54150=CARTESIAN_POINT('Ctrl Pts',(-3.54602591832973,-1.,-1.36436666257597));
#54151=CARTESIAN_POINT('Ctrl Pts',(-3.54602591832973,1.,-1.36436666257597));
#54152=CARTESIAN_POINT('Ctrl Pts',(-3.55353883995949,-1.,-1.3660614545677));
#54153=CARTESIAN_POINT('Ctrl Pts',(-3.55353883995949,1.,-1.3660614545677));
#54154=CARTESIAN_POINT('Ctrl Pts',(-3.56077662028649,-1.,-1.36754771771233));
#54155=CARTESIAN_POINT('Ctrl Pts',(-3.56077662028649,1.,-1.36754771771233));
#54156=CARTESIAN_POINT('Ctrl Pts',(-3.5678208030466,-1.,-1.36886584973389));
#54157=CARTESIAN_POINT('Ctrl Pts',(-3.5678208030466,1.,-1.36886584973389));
#54158=CARTESIAN_POINT('Ctrl Pts',(-3.57479875549486,-1.,-1.37007229485659));
#54159=CARTESIAN_POINT('Ctrl Pts',(-3.57479875549486,1.,-1.37007229485659));
#54160=CARTESIAN_POINT('Ctrl Pts',(-3.58183885982715,-1.,-1.37122241663062));
#54161=CARTESIAN_POINT('Ctrl Pts',(-3.58183885982715,1.,-1.37122241663062));
#54162=CARTESIAN_POINT('Ctrl Pts',(-3.58901853846365,-1.,-1.37235053660976));
#54163=CARTESIAN_POINT('Ctrl Pts',(-3.58901853846365,1.,-1.37235053660976));
#54164=CARTESIAN_POINT('Ctrl Pts',(-3.59634627869048,-1.,-1.37346320103157));
#54165=CARTESIAN_POINT('Ctrl Pts',(-3.59634627869048,1.,-1.37346320103157));
#54166=CARTESIAN_POINT('Ctrl Pts',(-3.60379020123988,-1.,-1.37455051379623));
#54167=CARTESIAN_POINT('Ctrl Pts',(-3.60379020123988,1.,-1.37455051379623));
#54168=CARTESIAN_POINT('Ctrl Pts',(-3.61129546591064,-1.,-1.37559314436634));
#54169=CARTESIAN_POINT('Ctrl Pts',(-3.61129546591064,1.,-1.37559314436634));
#54170=CARTESIAN_POINT('Ctrl Pts',(-3.6188048116042,-1.,-1.37657053403107));
#54171=CARTESIAN_POINT('Ctrl Pts',(-3.6188048116042,1.,-1.37657053403107));
#54172=CARTESIAN_POINT('Ctrl Pts',(-3.62628098665145,-1.,-1.37746987919881));
#54173=CARTESIAN_POINT('Ctrl Pts',(-3.62628098665145,1.,-1.37746987919881));
#54174=CARTESIAN_POINT('Ctrl Pts',(-3.63371727442486,-1.,-1.37829035457339));
#54175=CARTESIAN_POINT('Ctrl Pts',(-3.63371727442486,1.,-1.37829035457339));
#54176=CARTESIAN_POINT('Ctrl Pts',(-3.64112507791141,-1.,-1.37903818567359));
#54177=CARTESIAN_POINT('Ctrl Pts',(-3.64112507791141,1.,-1.37903818567359));
#54178=CARTESIAN_POINT('Ctrl Pts',(-3.64852652756456,-1.,-1.37972372481603));
#54179=CARTESIAN_POINT('Ctrl Pts',(-3.64852652756456,1.,-1.37972372481603));
#54180=CARTESIAN_POINT('Ctrl Pts',(-3.6559455440439,-1.,-1.38035791051212));
#54181=CARTESIAN_POINT('Ctrl Pts',(-3.6559455440439,1.,-1.38035791051212));
#54182=CARTESIAN_POINT('Ctrl Pts',(-3.66339848520857,-1.,-1.38094856333552));
#54183=CARTESIAN_POINT('Ctrl Pts',(-3.66339848520857,1.,-1.38094856333552));
#54184=CARTESIAN_POINT('Ctrl Pts',(-3.67088843112262,-1.,-1.38149812653868));
#54185=CARTESIAN_POINT('Ctrl Pts',(-3.67088843112262,1.,-1.38149812653868));
#54186=CARTESIAN_POINT('Ctrl Pts',(-3.67841038482414,-1.,-1.3820057429062));
#54187=CARTESIAN_POINT('Ctrl Pts',(-3.67841038482414,1.,-1.3820057429062));
#54188=CARTESIAN_POINT('Ctrl Pts',(-3.68595444983837,-1.,-1.38246852827182));
#54189=CARTESIAN_POINT('Ctrl Pts',(-3.68595444983837,1.,-1.38246852827182));
#54190=CARTESIAN_POINT('Ctrl Pts',(-3.69350967899526,-1.,-1.3828831117165));
#54191=CARTESIAN_POINT('Ctrl Pts',(-3.69350967899526,1.,-1.3828831117165));
#54192=CARTESIAN_POINT('Ctrl Pts',(-3.701067921679,-1.,-1.38324717612865));
#54193=CARTESIAN_POINT('Ctrl Pts',(-3.701067921679,1.,-1.38324717612865));
#54194=CARTESIAN_POINT('Ctrl Pts',(-3.70862680753347,-1.,-1.38356065402124));
#54195=CARTESIAN_POINT('Ctrl Pts',(-3.70862680753347,1.,-1.38356065402124));
#54196=CARTESIAN_POINT('Ctrl Pts',(-3.7161876605181,-1.,-1.38382489984586));
#54197=CARTESIAN_POINT('Ctrl Pts',(-3.7161876605181,1.,-1.38382489984586));
#54198=CARTESIAN_POINT('Ctrl Pts',(-3.72375409358803,-1.,-1.3840421342895));
#54199=CARTESIAN_POINT('Ctrl Pts',(-3.72375409358803,1.,-1.3840421342895));
#54200=CARTESIAN_POINT('Ctrl Pts',(-3.73133035859282,-1.,-1.38421479111531));
#54201=CARTESIAN_POINT('Ctrl Pts',(-3.73133035859282,1.,-1.38421479111531));
#54202=CARTESIAN_POINT('Ctrl Pts',(-3.73891976418104,-1.,-1.38434489156458));
#54203=CARTESIAN_POINT('Ctrl Pts',(-3.73891976418104,1.,-1.38434489156458));
#54204=CARTESIAN_POINT('Ctrl Pts',(-3.74652317167876,-1.,-1.38443344984394));
#54205=CARTESIAN_POINT('Ctrl Pts',(-3.74652317167876,1.,-1.38443344984394));
#54206=CARTESIAN_POINT('Ctrl Pts',(-3.7541397631875,-1.,-1.38448077997163));
#54207=CARTESIAN_POINT('Ctrl Pts',(-3.7541397631875,1.,-1.38448077997163));
#54208=CARTESIAN_POINT('Ctrl Pts',(-3.76176768271367,-1.,-1.3844867525335));
#54209=CARTESIAN_POINT('Ctrl Pts',(-3.76176768271367,1.,-1.3844867525335));
#54210=CARTESIAN_POINT('Ctrl Pts',(-3.76940473185779,-1.,-1.38445107339518));
#54211=CARTESIAN_POINT('Ctrl Pts',(-3.76940473185779,1.,-1.38445107339518));
#54212=CARTESIAN_POINT('Ctrl Pts',(-3.77704902230418,-1.,-1.38437354551428));
#54213=CARTESIAN_POINT('Ctrl Pts',(-3.77704902230418,1.,-1.38437354551428));
#54214=CARTESIAN_POINT('Ctrl Pts',(-3.78469969805082,-1.,-1.38425435883756));
#54215=CARTESIAN_POINT('Ctrl Pts',(-3.78469969805082,1.,-1.38425435883756));
#54216=CARTESIAN_POINT('Ctrl Pts',(-3.79235669640841,-1.,-1.38409399694566));
#54217=CARTESIAN_POINT('Ctrl Pts',(-3.79235669640841,1.,-1.38409399694566));
#54218=CARTESIAN_POINT('Ctrl Pts',(-3.80002044322111,-1.,-1.38389311766682));
#54219=CARTESIAN_POINT('Ctrl Pts',(-3.80002044322111,1.,-1.38389311766682));
#54220=CARTESIAN_POINT('Ctrl Pts',(-3.80769156398411,-1.,-1.3836524404622));
#54221=CARTESIAN_POINT('Ctrl Pts',(-3.80769156398411,1.,-1.3836524404622));
#54222=CARTESIAN_POINT('Ctrl Pts',(-3.81537060817811,-1.,-1.38337263902782));
#54223=CARTESIAN_POINT('Ctrl Pts',(-3.81537060817811,1.,-1.38337263902782));
#54224=CARTESIAN_POINT('Ctrl Pts',(-3.82305771743829,-1.,-1.38305421262763));
#54225=CARTESIAN_POINT('Ctrl Pts',(-3.82305771743829,1.,-1.38305421262763));
#54226=CARTESIAN_POINT('Ctrl Pts',(-3.8307526698229,-1.,-1.38269750245138));
#54227=CARTESIAN_POINT('Ctrl Pts',(-3.8307526698229,1.,-1.38269750245138));
#54228=CARTESIAN_POINT('Ctrl Pts',(-3.83845502790746,-1.,-1.38230274828821));
#54229=CARTESIAN_POINT('Ctrl Pts',(-3.83845502790746,1.,-1.38230274828821));
#54230=CARTESIAN_POINT('Ctrl Pts',(-3.84616425605764,-1.,-1.38187013346109));
#54231=CARTESIAN_POINT('Ctrl Pts',(-3.84616425605764,1.,-1.38187013346109));
#54232=CARTESIAN_POINT('Ctrl Pts',(-3.85387983979481,-1.,-1.38139983115049));
#54233=CARTESIAN_POINT('Ctrl Pts',(-3.85387983979481,1.,-1.38139983115049));
#54234=CARTESIAN_POINT('Ctrl Pts',(-3.86160143043959,-1.,-1.38089205992989));
#54235=CARTESIAN_POINT('Ctrl Pts',(-3.86160143043959,1.,-1.38089205992989));
#54236=CARTESIAN_POINT('Ctrl Pts',(-3.86932885813068,-1.,-1.38034709213014));
#54237=CARTESIAN_POINT('Ctrl Pts',(-3.86932885813068,1.,-1.38034709213014));
#54238=CARTESIAN_POINT('Ctrl Pts',(-3.87706205830532,-1.,-1.37976523097073));
#54239=CARTESIAN_POINT('Ctrl Pts',(-3.87706205830532,1.,-1.37976523097073));
#54240=CARTESIAN_POINT('Ctrl Pts',(-3.88480102249277,-1.,-1.37914679719383));
#54241=CARTESIAN_POINT('Ctrl Pts',(-3.88480102249277,1.,-1.37914679719383));
#54242=CARTESIAN_POINT('Ctrl Pts',(-3.89254574338496,-1.,-1.3784921128802));
#54243=CARTESIAN_POINT('Ctrl Pts',(-3.89254574338496,1.,-1.3784921128802));
#54244=CARTESIAN_POINT('Ctrl Pts',(-3.90029615196727,-1.,-1.37780148512792));
#54245=CARTESIAN_POINT('Ctrl Pts',(-3.90029615196727,1.,-1.37780148512792));
#54246=CARTESIAN_POINT('Ctrl Pts',(-3.90805209523486,-1.,-1.3770751963402));
#54247=CARTESIAN_POINT('Ctrl Pts',(-3.90805209523486,1.,-1.3770751963402));
#54248=CARTESIAN_POINT('Ctrl Pts',(-3.91581337462644,-1.,-1.37631350505797));
#54249=CARTESIAN_POINT('Ctrl Pts',(-3.91581337462644,1.,-1.37631350505797));
#54250=CARTESIAN_POINT('Ctrl Pts',(-3.92357976987672,-1.,-1.37551664448242));
#54251=CARTESIAN_POINT('Ctrl Pts',(-3.92357976987672,1.,-1.37551664448242));
#54252=CARTESIAN_POINT('Ctrl Pts',(-3.93135106761844,-1.,-1.37468482215751));
#54253=CARTESIAN_POINT('Ctrl Pts',(-3.93135106761844,1.,-1.37468482215751));
#54254=CARTESIAN_POINT('Ctrl Pts',(-3.93912709040818,-1.,-1.37381821967165));
#54255=CARTESIAN_POINT('Ctrl Pts',(-3.93912709040818,1.,-1.37381821967165));
#54256=CARTESIAN_POINT('Ctrl Pts',(-3.94690771785133,-1.,-1.37291699202807));
#54257=CARTESIAN_POINT('Ctrl Pts',(-3.94690771785133,1.,-1.37291699202807));
#54258=CARTESIAN_POINT('Ctrl Pts',(-3.95469287280914,-1.,-1.37198126432386));
#54259=CARTESIAN_POINT('Ctrl Pts',(-3.95469287280914,1.,-1.37198126432386));
#54260=CARTESIAN_POINT('Ctrl Pts',(-3.96092458506535,-1.,-1.3712051561502));
#54261=CARTESIAN_POINT('Ctrl Pts',(-3.96092458506535,1.,-1.3712051561502));
#54262=CARTESIAN_POINT('Ctrl Pts',(-3.96560037974645,-1.,-1.37060761745635));
#54263=CARTESIAN_POINT('Ctrl Pts',(-3.96560037974645,1.,-1.37060761745635));
#54264=CARTESIAN_POINT('Ctrl Pts',(-3.9687184694131,-1.,-1.37020239094614));
#54265=CARTESIAN_POINT('Ctrl Pts',(-3.9687184694131,1.,-1.37020239094614));
#54266=CARTESIAN_POINT('Ctrl Pts',(-3.97027773754922,-1.,-1.36999806084572));
#54267=CARTESIAN_POINT('Ctrl Pts',(-3.97027773754922,1.,-1.36999806084572));
#54268=CARTESIAN_POINT('',(-3.4984457533445,1.,-1.35032489087101));
#54269=CARTESIAN_POINT('Ctrl Pts',(-3.4984457533445,-1.,-1.35032489087101));
#54270=CARTESIAN_POINT('Ctrl Pts',(-3.4984457533445,-0.666666666666667,
-1.35032489087101));
#54271=CARTESIAN_POINT('Ctrl Pts',(-3.4984457533445,-0.333333333333333,
-1.35032489087101));
#54272=CARTESIAN_POINT('Ctrl Pts',(-3.4984457533445,0.333333333333333,-1.35032489087101));
#54273=CARTESIAN_POINT('Ctrl Pts',(-3.4984457533445,0.666666666666667,-1.35032489087101));
#54274=CARTESIAN_POINT('Ctrl Pts',(-3.4984457533445,1.,-1.35032489087101));
#54275=CARTESIAN_POINT('',(-3.97027773754922,1.,-1.36999806084572));
#54276=CARTESIAN_POINT('',(-3.97027773754922,0.,-1.36999806084572));
#54277=CARTESIAN_POINT('Ctrl Pts',(-3.4984457533445,1.,-1.35032489087101));
#54278=CARTESIAN_POINT('Ctrl Pts',(-3.49847119623846,1.,-1.35036670892966));
#54279=CARTESIAN_POINT('Ctrl Pts',(-3.49861894124827,1.,-1.35049736560527));
#54280=CARTESIAN_POINT('Ctrl Pts',(-3.49920025459723,1.,-1.35080045218587));
#54281=CARTESIAN_POINT('Ctrl Pts',(-3.5007660381649,1.,-1.35142377279517));
#54282=CARTESIAN_POINT('Ctrl Pts',(-3.50408168106261,1.,-1.35257032843486));
#54283=CARTESIAN_POINT('Ctrl Pts',(-3.50913227059999,1.,-1.35419113575956));
#54284=CARTESIAN_POINT('Ctrl Pts',(-3.51542230699556,1.,-1.35611275237152));
#54285=CARTESIAN_POINT('Ctrl Pts',(-3.52261776116748,1.,-1.35821701528836));
#54286=CARTESIAN_POINT('Ctrl Pts',(-3.530344649616,1.,-1.36037259643734));
#54287=CARTESIAN_POINT('Ctrl Pts',(-3.53824396424961,1.,-1.36245507339307));
#54288=CARTESIAN_POINT('Ctrl Pts',(-3.54602591832973,1.,-1.36436666257597));
#54289=CARTESIAN_POINT('Ctrl Pts',(-3.55353883995949,1.,-1.3660614545677));
#54290=CARTESIAN_POINT('Ctrl Pts',(-3.56077662028649,1.,-1.36754771771233));
#54291=CARTESIAN_POINT('Ctrl Pts',(-3.5678208030466,1.,-1.36886584973389));
#54292=CARTESIAN_POINT('Ctrl Pts',(-3.57479875549486,1.,-1.37007229485659));
#54293=CARTESIAN_POINT('Ctrl Pts',(-3.58183885982715,1.,-1.37122241663062));
#54294=CARTESIAN_POINT('Ctrl Pts',(-3.58901853846365,1.,-1.37235053660976));
#54295=CARTESIAN_POINT('Ctrl Pts',(-3.59634627869048,1.,-1.37346320103157));
#54296=CARTESIAN_POINT('Ctrl Pts',(-3.60379020123988,1.,-1.37455051379623));
#54297=CARTESIAN_POINT('Ctrl Pts',(-3.61129546591064,1.,-1.37559314436634));
#54298=CARTESIAN_POINT('Ctrl Pts',(-3.6188048116042,1.,-1.37657053403107));
#54299=CARTESIAN_POINT('Ctrl Pts',(-3.62628098665145,1.,-1.37746987919881));
#54300=CARTESIAN_POINT('Ctrl Pts',(-3.63371727442486,1.,-1.37829035457339));
#54301=CARTESIAN_POINT('Ctrl Pts',(-3.64112507791141,1.,-1.37903818567359));
#54302=CARTESIAN_POINT('Ctrl Pts',(-3.64852652756456,1.,-1.37972372481603));
#54303=CARTESIAN_POINT('Ctrl Pts',(-3.6559455440439,1.,-1.38035791051212));
#54304=CARTESIAN_POINT('Ctrl Pts',(-3.66339848520857,1.,-1.38094856333552));
#54305=CARTESIAN_POINT('Ctrl Pts',(-3.67088843112262,1.,-1.38149812653868));
#54306=CARTESIAN_POINT('Ctrl Pts',(-3.67841038482414,1.,-1.3820057429062));
#54307=CARTESIAN_POINT('Ctrl Pts',(-3.68595444983837,1.,-1.38246852827182));
#54308=CARTESIAN_POINT('Ctrl Pts',(-3.69350967899526,1.,-1.3828831117165));
#54309=CARTESIAN_POINT('Ctrl Pts',(-3.701067921679,1.,-1.38324717612865));
#54310=CARTESIAN_POINT('Ctrl Pts',(-3.70862680753347,1.,-1.38356065402124));
#54311=CARTESIAN_POINT('Ctrl Pts',(-3.7161876605181,1.,-1.38382489984586));
#54312=CARTESIAN_POINT('Ctrl Pts',(-3.72375409358803,1.,-1.3840421342895));
#54313=CARTESIAN_POINT('Ctrl Pts',(-3.73133035859282,1.,-1.38421479111531));
#54314=CARTESIAN_POINT('Ctrl Pts',(-3.73891976418104,1.,-1.38434489156458));
#54315=CARTESIAN_POINT('Ctrl Pts',(-3.74652317167876,1.,-1.38443344984394));
#54316=CARTESIAN_POINT('Ctrl Pts',(-3.7541397631875,1.,-1.38448077997163));
#54317=CARTESIAN_POINT('Ctrl Pts',(-3.76176768271367,1.,-1.3844867525335));
#54318=CARTESIAN_POINT('Ctrl Pts',(-3.76940473185779,1.,-1.38445107339518));
#54319=CARTESIAN_POINT('Ctrl Pts',(-3.77704902230418,1.,-1.38437354551428));
#54320=CARTESIAN_POINT('Ctrl Pts',(-3.78469969805082,1.,-1.38425435883756));
#54321=CARTESIAN_POINT('Ctrl Pts',(-3.79235669640841,1.,-1.38409399694566));
#54322=CARTESIAN_POINT('Ctrl Pts',(-3.80002044322111,1.,-1.38389311766682));
#54323=CARTESIAN_POINT('Ctrl Pts',(-3.80769156398411,1.,-1.3836524404622));
#54324=CARTESIAN_POINT('Ctrl Pts',(-3.81537060817811,1.,-1.38337263902782));
#54325=CARTESIAN_POINT('Ctrl Pts',(-3.82305771743829,1.,-1.38305421262763));
#54326=CARTESIAN_POINT('Ctrl Pts',(-3.8307526698229,1.,-1.38269750245138));
#54327=CARTESIAN_POINT('Ctrl Pts',(-3.83845502790746,1.,-1.38230274828821));
#54328=CARTESIAN_POINT('Ctrl Pts',(-3.84616425605764,1.,-1.38187013346109));
#54329=CARTESIAN_POINT('Ctrl Pts',(-3.85387983979481,1.,-1.38139983115049));
#54330=CARTESIAN_POINT('Ctrl Pts',(-3.86160143043959,1.,-1.38089205992989));
#54331=CARTESIAN_POINT('Ctrl Pts',(-3.86932885813068,1.,-1.38034709213014));
#54332=CARTESIAN_POINT('Ctrl Pts',(-3.87706205830532,1.,-1.37976523097073));
#54333=CARTESIAN_POINT('Ctrl Pts',(-3.88480102249277,1.,-1.37914679719383));
#54334=CARTESIAN_POINT('Ctrl Pts',(-3.89254574338496,1.,-1.3784921128802));
#54335=CARTESIAN_POINT('Ctrl Pts',(-3.90029615196727,1.,-1.37780148512792));
#54336=CARTESIAN_POINT('Ctrl Pts',(-3.90805209523486,1.,-1.3770751963402));
#54337=CARTESIAN_POINT('Ctrl Pts',(-3.91581337462644,1.,-1.37631350505797));
#54338=CARTESIAN_POINT('Ctrl Pts',(-3.92357976987672,1.,-1.37551664448242));
#54339=CARTESIAN_POINT('Ctrl Pts',(-3.93135106761844,1.,-1.37468482215751));
#54340=CARTESIAN_POINT('Ctrl Pts',(-3.93912709040818,1.,-1.37381821967165));
#54341=CARTESIAN_POINT('Ctrl Pts',(-3.94690771785133,1.,-1.37291699202807));
#54342=CARTESIAN_POINT('Ctrl Pts',(-3.95469287280914,1.,-1.37198126432386));
#54343=CARTESIAN_POINT('Ctrl Pts',(-3.96092458506535,1.,-1.3712051561502));
#54344=CARTESIAN_POINT('Ctrl Pts',(-3.96560037974645,1.,-1.37060761745635));
#54345=CARTESIAN_POINT('Ctrl Pts',(-3.9687184694131,1.,-1.37020239094614));
#54346=CARTESIAN_POINT('Ctrl Pts',(-3.97027773754922,1.,-1.36999806084572));
#54347=CARTESIAN_POINT('Origin',(-3.97027773754922,0.,-1.36999806084572));
#54348=CARTESIAN_POINT('',(-4.01728681790024,1.,-1.22531898815164));
#54349=CARTESIAN_POINT('Origin',(0.,0.,0.));
#54350=CARTESIAN_POINT('',(-3.42859860294378,1.,-1.51895082866166));
#54351=CARTESIAN_POINT('Origin',(0.,1.,0.));
#54352=CARTESIAN_POINT('Ctrl Pts',(-3.42859860294378,1.,-1.51895082866166));
#54353=CARTESIAN_POINT('Ctrl Pts',(-3.42859860294378,0.666666666666667,
-1.51895082866166));
#54354=CARTESIAN_POINT('Ctrl Pts',(-3.42859860294378,0.333333333333333,
-1.51895082866166));
#54355=CARTESIAN_POINT('Ctrl Pts',(-3.42859860294378,-0.333333333333333,
-1.51895082866166));
#54356=CARTESIAN_POINT('Ctrl Pts',(-3.42859860294378,-0.666666666666667,
-1.51895082866166));
#54357=CARTESIAN_POINT('Ctrl Pts',(-3.42859860294378,-1.,-1.51895082866166));
#54358=CARTESIAN_POINT('Ctrl Pts',(-3.77614523045147,-1.,-1.83867539237861));
#54359=CARTESIAN_POINT('Ctrl Pts',(-3.77614523045147,1.,-1.83867539237861));
#54360=CARTESIAN_POINT('Ctrl Pts',(-3.77518714458232,-1.,-1.83742834010821));
#54361=CARTESIAN_POINT('Ctrl Pts',(-3.77518714458232,1.,-1.83742834010821));
#54362=CARTESIAN_POINT('Ctrl Pts',(-3.77326886065484,-1.,-1.83493697935064));
#54363=CARTESIAN_POINT('Ctrl Pts',(-3.77326886065484,1.,-1.83493697935064));
#54364=CARTESIAN_POINT('Ctrl Pts',(-3.77038509819777,-1.,-1.83120816956515));
#54365=CARTESIAN_POINT('Ctrl Pts',(-3.77038509819777,1.,-1.83120816956515));
#54366=CARTESIAN_POINT('Ctrl Pts',(-3.76652740355856,-1.,-1.82625289221933));
#54367=CARTESIAN_POINT('Ctrl Pts',(-3.76652740355856,1.,-1.82625289221933));
#54368=CARTESIAN_POINT('Ctrl Pts',(-3.76168412709652,-1.,-1.82008629694924));
#54369=CARTESIAN_POINT('Ctrl Pts',(-3.76168412709652,1.,-1.82008629694924));
#54370=CARTESIAN_POINT('Ctrl Pts',(-3.75681965683995,-1.,-1.81394729834032));
#54371=CARTESIAN_POINT('Ctrl Pts',(-3.75681965683995,1.,-1.81394729834032));
#54372=CARTESIAN_POINT('Ctrl Pts',(-3.75193395888069,-1.,-1.80783603939662));
#54373=CARTESIAN_POINT('Ctrl Pts',(-3.75193395888069,1.,-1.80783603939662));
#54374=CARTESIAN_POINT('Ctrl Pts',(-3.74702700874954,-1.,-1.80175271485519));
#54375=CARTESIAN_POINT('Ctrl Pts',(-3.74702700874954,1.,-1.80175271485519));
#54376=CARTESIAN_POINT('Ctrl Pts',(-3.74209880351667,-1.,-1.79569757859041));
#54377=CARTESIAN_POINT('Ctrl Pts',(-3.74209880351667,1.,-1.79569757859041));
#54378=CARTESIAN_POINT('Ctrl Pts',(-3.73714934729962,-1.,-1.78967092823139));
#54379=CARTESIAN_POINT('Ctrl Pts',(-3.73714934729962,1.,-1.78967092823139));
#54380=CARTESIAN_POINT('Ctrl Pts',(-3.73217863095022,-1.,-1.78367308442682));
#54381=CARTESIAN_POINT('Ctrl Pts',(-3.73217863095022,1.,-1.78367308442682));
#54382=CARTESIAN_POINT('Ctrl Pts',(-3.72718661205504,-1.,-1.77770437039606));
#54383=CARTESIAN_POINT('Ctrl Pts',(-3.72718661205504,1.,-1.77770437039606));
#54384=CARTESIAN_POINT('Ctrl Pts',(-3.72217319911429,-1.,-1.77176509401846));
#54385=CARTESIAN_POINT('Ctrl Pts',(-3.72217319911429,1.,-1.77176509401846));
#54386=CARTESIAN_POINT('Ctrl Pts',(-3.71713822377675,-1.,-1.76585552124549));
#54387=CARTESIAN_POINT('Ctrl Pts',(-3.71713822377675,1.,-1.76585552124549));
#54388=CARTESIAN_POINT('Ctrl Pts',(-3.71208146346454,-1.,-1.75997588499021));
#54389=CARTESIAN_POINT('Ctrl Pts',(-3.71208146346454,1.,-1.75997588499021));
#54390=CARTESIAN_POINT('Ctrl Pts',(-3.70700269736876,-1.,-1.75412641804148));
#54391=CARTESIAN_POINT('Ctrl Pts',(-3.70700269736876,1.,-1.75412641804148));
#54392=CARTESIAN_POINT('Ctrl Pts',(-3.70190175673422,-1.,-1.74830738046092));
#54393=CARTESIAN_POINT('Ctrl Pts',(-3.70190175673422,1.,-1.74830738046092));
#54394=CARTESIAN_POINT('Ctrl Pts',(-3.6967785691046,-1.,-1.74251908492589));
#54395=CARTESIAN_POINT('Ctrl Pts',(-3.6967785691046,1.,-1.74251908492589));
#54396=CARTESIAN_POINT('Ctrl Pts',(-3.69163322647906,-1.,-1.73676193254493));
#54397=CARTESIAN_POINT('Ctrl Pts',(-3.69163322647906,1.,-1.73676193254493));
#54398=CARTESIAN_POINT('Ctrl Pts',(-3.68646597019188,-1.,-1.73103640956647));
#54399=CARTESIAN_POINT('Ctrl Pts',(-3.68646597019188,1.,-1.73103640956647));
#54400=CARTESIAN_POINT('Ctrl Pts',(-3.68127704936472,-1.,-1.72534302437003));
#54401=CARTESIAN_POINT('Ctrl Pts',(-3.68127704936472,1.,-1.72534302437003));
#54402=CARTESIAN_POINT('Ctrl Pts',(-3.67606660374665,-1.,-1.71968225581787));
#54403=CARTESIAN_POINT('Ctrl Pts',(-3.67606660374665,1.,-1.71968225581787));
#54404=CARTESIAN_POINT('Ctrl Pts',(-3.67083454901629,-1.,-1.71405450210392));
#54405=CARTESIAN_POINT('Ctrl Pts',(-3.67083454901629,1.,-1.71405450210392));
#54406=CARTESIAN_POINT('Ctrl Pts',(-3.6655804319893,-1.,-1.70846001610983));
#54407=CARTESIAN_POINT('Ctrl Pts',(-3.6655804319893,1.,-1.70846001610983));
#54408=CARTESIAN_POINT('Ctrl Pts',(-3.6603033877491,-1.,-1.70289888566904));
#54409=CARTESIAN_POINT('Ctrl Pts',(-3.6603033877491,1.,-1.70289888566904));
#54410=CARTESIAN_POINT('Ctrl Pts',(-3.65500246526798,-1.,-1.69737117722558));
#54411=CARTESIAN_POINT('Ctrl Pts',(-3.65500246526798,1.,-1.69737117722558));
#54412=CARTESIAN_POINT('Ctrl Pts',(-3.64967689827393,-1.,-1.691877054817));
#54413=CARTESIAN_POINT('Ctrl Pts',(-3.64967689827393,1.,-1.691877054817));
#54414=CARTESIAN_POINT('Ctrl Pts',(-3.64432638915199,-1.,-1.68641690471455));
#54415=CARTESIAN_POINT('Ctrl Pts',(-3.64432638915199,1.,-1.68641690471455));
#54416=CARTESIAN_POINT('Ctrl Pts',(-3.63895140887443,-1.,-1.68099146651577));
#54417=CARTESIAN_POINT('Ctrl Pts',(-3.63895140887443,1.,-1.68099146651577));
#54418=CARTESIAN_POINT('Ctrl Pts',(-3.63355343201211,-1.,-1.67560193613145));
#54419=CARTESIAN_POINT('Ctrl Pts',(-3.63355343201211,1.,-1.67560193613145));
#54420=CARTESIAN_POINT('Ctrl Pts',(-3.62813422105257,-1.,-1.67024966008037));
#54421=CARTESIAN_POINT('Ctrl Pts',(-3.62813422105257,1.,-1.67024966008037));
#54422=CARTESIAN_POINT('Ctrl Pts',(-3.62269517989104,-1.,-1.66493585923853));
#54423=CARTESIAN_POINT('Ctrl Pts',(-3.62269517989104,1.,-1.66493585923853));
#54424=CARTESIAN_POINT('Ctrl Pts',(-3.61723666482457,-1.,-1.65966133399186));
#54425=CARTESIAN_POINT('Ctrl Pts',(-3.61723666482457,1.,-1.65966133399186));
#54426=CARTESIAN_POINT('Ctrl Pts',(-3.61175734965129,-1.,-1.65442619244327));
#54427=CARTESIAN_POINT('Ctrl Pts',(-3.61175734965129,1.,-1.65442619244327));
#54428=CARTESIAN_POINT('Ctrl Pts',(-3.60625346556992,-1.,-1.64922952425833));
#54429=CARTESIAN_POINT('Ctrl Pts',(-3.60625346556992,1.,-1.64922952425833));
#54430=CARTESIAN_POINT('Ctrl Pts',(-3.6007202851384,-1.,-1.6440700438558));
#54431=CARTESIAN_POINT('Ctrl Pts',(-3.6007202851384,1.,-1.6440700438558));
#54432=CARTESIAN_POINT('Ctrl Pts',(-3.59515368334887,-1.,-1.63894676675349));
#54433=CARTESIAN_POINT('Ctrl Pts',(-3.59515368334887,1.,-1.63894676675349));
#54434=CARTESIAN_POINT('Ctrl Pts',(-3.58955176627876,-1.,-1.63385971451259));
#54435=CARTESIAN_POINT('Ctrl Pts',(-3.58955176627876,1.,-1.63385971451259));
#54436=CARTESIAN_POINT('Ctrl Pts',(-3.5839162577435,-1.,-1.62881051550748));
#54437=CARTESIAN_POINT('Ctrl Pts',(-3.5839162577435,1.,-1.62881051550748));
#54438=CARTESIAN_POINT('Ctrl Pts',(-3.57825455954405,-1.,-1.62380329464851));
#54439=CARTESIAN_POINT('Ctrl Pts',(-3.57825455954405,1.,-1.62380329464851));
#54440=CARTESIAN_POINT('Ctrl Pts',(-3.57257679609826,-1.,-1.61884340915412));
#54441=CARTESIAN_POINT('Ctrl Pts',(-3.57257679609826,1.,-1.61884340915412));
#54442=CARTESIAN_POINT('Ctrl Pts',(-3.56689200468404,-1.,-1.61393581747522));
#54443=CARTESIAN_POINT('Ctrl Pts',(-3.56689200468404,1.,-1.61393581747522));
#54444=CARTESIAN_POINT('Ctrl Pts',(-3.56120432482986,-1.,-1.60908344685459));
#54445=CARTESIAN_POINT('Ctrl Pts',(-3.56120432482986,1.,-1.60908344685459));
#54446=CARTESIAN_POINT('Ctrl Pts',(-3.55550985096117,-1.,-1.60428584699848));
#54447=CARTESIAN_POINT('Ctrl Pts',(-3.55550985096117,1.,-1.60428584699848));
#54448=CARTESIAN_POINT('Ctrl Pts',(-3.54979148634426,-1.,-1.59953698113444));
#54449=CARTESIAN_POINT('Ctrl Pts',(-3.54979148634426,1.,-1.59953698113444));
#54450=CARTESIAN_POINT('Ctrl Pts',(-3.544024581823,-1.,-1.5948276694975));
#54451=CARTESIAN_POINT('Ctrl Pts',(-3.544024581823,1.,-1.5948276694975));
#54452=CARTESIAN_POINT('Ctrl Pts',(-3.53818616861045,-1.,-1.59014958368725));
#54453=CARTESIAN_POINT('Ctrl Pts',(-3.53818616861045,1.,-1.59014958368725));
#54454=CARTESIAN_POINT('Ctrl Pts',(-3.53226378147068,-1.,-1.58549906268083));
#54455=CARTESIAN_POINT('Ctrl Pts',(-3.53226378147068,1.,-1.58549906268083));
#54456=CARTESIAN_POINT('Ctrl Pts',(-3.52626275334899,-1.,-1.58088027227856));
#54457=CARTESIAN_POINT('Ctrl Pts',(-3.52626275334899,1.,-1.58088027227856));
#54458=CARTESIAN_POINT('Ctrl Pts',(-3.52021847865961,-1.,-1.5763104998818));
#54459=CARTESIAN_POINT('Ctrl Pts',(-3.52021847865961,1.,-1.5763104998818));
#54460=CARTESIAN_POINT('Ctrl Pts',(-3.51418598431733,-1.,-1.57181569799774));
#54461=CARTESIAN_POINT('Ctrl Pts',(-3.51418598431733,1.,-1.57181569799774));
#54462=CARTESIAN_POINT('Ctrl Pts',(-3.50821771695427,-1.,-1.56742097575041));
#54463=CARTESIAN_POINT('Ctrl Pts',(-3.50821771695427,1.,-1.56742097575041));
#54464=CARTESIAN_POINT('Ctrl Pts',(-3.50234321621607,-1.,-1.56314187758689));
#54465=CARTESIAN_POINT('Ctrl Pts',(-3.50234321621607,1.,-1.56314187758689));
#54466=CARTESIAN_POINT('Ctrl Pts',(-3.49655185179623,-1.,-1.55897703097859));
#54467=CARTESIAN_POINT('Ctrl Pts',(-3.49655185179623,1.,-1.55897703097859));
#54468=CARTESIAN_POINT('Ctrl Pts',(-3.49076460877317,-1.,-1.5548959590107));
#54469=CARTESIAN_POINT('Ctrl Pts',(-3.49076460877317,1.,-1.5548959590107));
#54470=CARTESIAN_POINT('Ctrl Pts',(-3.48485155928414,-1.,-1.55084702970382));
#54471=CARTESIAN_POINT('Ctrl Pts',(-3.48485155928414,1.,-1.55084702970382));
#54472=CARTESIAN_POINT('Ctrl Pts',(-3.47868272898599,-1.,-1.54678009290206));
#54473=CARTESIAN_POINT('Ctrl Pts',(-3.47868272898599,1.,-1.54678009290206));
#54474=CARTESIAN_POINT('Ctrl Pts',(-3.47217189224576,-1.,-1.54266605398152));
#54475=CARTESIAN_POINT('Ctrl Pts',(-3.47217189224576,1.,-1.54266605398152));
#54476=CARTESIAN_POINT('Ctrl Pts',(-3.46531752207222,-1.,-1.53851507915533));
#54477=CARTESIAN_POINT('Ctrl Pts',(-3.46531752207222,1.,-1.53851507915533));
#54478=CARTESIAN_POINT('Ctrl Pts',(-3.45825932955273,-1.,-1.53440195378902));
#54479=CARTESIAN_POINT('Ctrl Pts',(-3.45825932955273,1.,-1.53440195378902));
#54480=CARTESIAN_POINT('Ctrl Pts',(-3.45127136828667,-1.,-1.530462444618));
#54481=CARTESIAN_POINT('Ctrl Pts',(-3.45127136828667,1.,-1.530462444618));
#54482=CARTESIAN_POINT('Ctrl Pts',(-3.44469547527,-1.,-1.52686242875717));
#54483=CARTESIAN_POINT('Ctrl Pts',(-3.44469547527,1.,-1.52686242875717));
#54484=CARTESIAN_POINT('Ctrl Pts',(-3.43888895974182,-1.,-1.52377348950429));
#54485=CARTESIAN_POINT('Ctrl Pts',(-3.43888895974182,1.,-1.52377348950429));
#54486=CARTESIAN_POINT('Ctrl Pts',(-3.43417156977749,-1.,-1.52134826724227));
#54487=CARTESIAN_POINT('Ctrl Pts',(-3.43417156977749,1.,-1.52134826724227));
#54488=CARTESIAN_POINT('Ctrl Pts',(-3.43076036253384,-1.,-1.51969006980792));
#54489=CARTESIAN_POINT('Ctrl Pts',(-3.43076036253384,1.,-1.51969006980792));
#54490=CARTESIAN_POINT('Ctrl Pts',(-3.42915787669388,-1.,-1.51901585838879));
#54491=CARTESIAN_POINT('Ctrl Pts',(-3.42915787669388,1.,-1.51901585838879));
#54492=CARTESIAN_POINT('Ctrl Pts',(-3.42860527148835,-1.,-1.51888450659497));
#54493=CARTESIAN_POINT('Ctrl Pts',(-3.42860527148835,1.,-1.51888450659497));
#54494=CARTESIAN_POINT('Ctrl Pts',(-3.42852521763648,-1.,-1.51896318668306));
#54495=CARTESIAN_POINT('Ctrl Pts',(-3.42852521763648,1.,-1.51896318668306));
#54496=CARTESIAN_POINT('Ctrl Pts',(-3.42855728381368,-1.,-1.519044091397));
#54497=CARTESIAN_POINT('Ctrl Pts',(-3.42855728381368,1.,-1.519044091397));
#54498=CARTESIAN_POINT('',(-3.77614523045147,1.,-1.83867539237861));
#54499=CARTESIAN_POINT('Ctrl Pts',(-3.77614523045147,1.,-1.83867539237861));
#54500=CARTESIAN_POINT('Ctrl Pts',(-3.77518714458232,1.,-1.83742834010821));
#54501=CARTESIAN_POINT('Ctrl Pts',(-3.77326886065484,1.,-1.83493697935064));
#54502=CARTESIAN_POINT('Ctrl Pts',(-3.77038509819777,1.,-1.83120816956515));
#54503=CARTESIAN_POINT('Ctrl Pts',(-3.76652740355856,1.,-1.82625289221933));
#54504=CARTESIAN_POINT('Ctrl Pts',(-3.76168412709652,1.,-1.82008629694924));
#54505=CARTESIAN_POINT('Ctrl Pts',(-3.75681965683995,1.,-1.81394729834032));
#54506=CARTESIAN_POINT('Ctrl Pts',(-3.75193395888069,1.,-1.80783603939662));
#54507=CARTESIAN_POINT('Ctrl Pts',(-3.74702700874954,1.,-1.80175271485519));
#54508=CARTESIAN_POINT('Ctrl Pts',(-3.74209880351667,1.,-1.79569757859041));
#54509=CARTESIAN_POINT('Ctrl Pts',(-3.73714934729962,1.,-1.78967092823139));
#54510=CARTESIAN_POINT('Ctrl Pts',(-3.73217863095022,1.,-1.78367308442682));
#54511=CARTESIAN_POINT('Ctrl Pts',(-3.72718661205504,1.,-1.77770437039606));
#54512=CARTESIAN_POINT('Ctrl Pts',(-3.72217319911429,1.,-1.77176509401846));
#54513=CARTESIAN_POINT('Ctrl Pts',(-3.71713822377675,1.,-1.76585552124549));
#54514=CARTESIAN_POINT('Ctrl Pts',(-3.71208146346454,1.,-1.75997588499021));
#54515=CARTESIAN_POINT('Ctrl Pts',(-3.70700269736876,1.,-1.75412641804148));
#54516=CARTESIAN_POINT('Ctrl Pts',(-3.70190175673422,1.,-1.74830738046092));
#54517=CARTESIAN_POINT('Ctrl Pts',(-3.6967785691046,1.,-1.74251908492589));
#54518=CARTESIAN_POINT('Ctrl Pts',(-3.69163322647906,1.,-1.73676193254493));
#54519=CARTESIAN_POINT('Ctrl Pts',(-3.68646597019188,1.,-1.73103640956647));
#54520=CARTESIAN_POINT('Ctrl Pts',(-3.68127704936472,1.,-1.72534302437003));
#54521=CARTESIAN_POINT('Ctrl Pts',(-3.67606660374665,1.,-1.71968225581787));
#54522=CARTESIAN_POINT('Ctrl Pts',(-3.67083454901629,1.,-1.71405450210392));
#54523=CARTESIAN_POINT('Ctrl Pts',(-3.6655804319893,1.,-1.70846001610983));
#54524=CARTESIAN_POINT('Ctrl Pts',(-3.6603033877491,1.,-1.70289888566904));
#54525=CARTESIAN_POINT('Ctrl Pts',(-3.65500246526798,1.,-1.69737117722558));
#54526=CARTESIAN_POINT('Ctrl Pts',(-3.64967689827393,1.,-1.691877054817));
#54527=CARTESIAN_POINT('Ctrl Pts',(-3.64432638915199,1.,-1.68641690471455));
#54528=CARTESIAN_POINT('Ctrl Pts',(-3.63895140887443,1.,-1.68099146651577));
#54529=CARTESIAN_POINT('Ctrl Pts',(-3.63355343201211,1.,-1.67560193613145));
#54530=CARTESIAN_POINT('Ctrl Pts',(-3.62813422105257,1.,-1.67024966008037));
#54531=CARTESIAN_POINT('Ctrl Pts',(-3.62269517989104,1.,-1.66493585923853));
#54532=CARTESIAN_POINT('Ctrl Pts',(-3.61723666482457,1.,-1.65966133399186));
#54533=CARTESIAN_POINT('Ctrl Pts',(-3.61175734965129,1.,-1.65442619244327));
#54534=CARTESIAN_POINT('Ctrl Pts',(-3.60625346556992,1.,-1.64922952425833));
#54535=CARTESIAN_POINT('Ctrl Pts',(-3.6007202851384,1.,-1.6440700438558));
#54536=CARTESIAN_POINT('Ctrl Pts',(-3.59515368334887,1.,-1.63894676675349));
#54537=CARTESIAN_POINT('Ctrl Pts',(-3.58955176627876,1.,-1.63385971451259));
#54538=CARTESIAN_POINT('Ctrl Pts',(-3.5839162577435,1.,-1.62881051550748));
#54539=CARTESIAN_POINT('Ctrl Pts',(-3.57825455954405,1.,-1.62380329464851));
#54540=CARTESIAN_POINT('Ctrl Pts',(-3.57257679609826,1.,-1.61884340915412));
#54541=CARTESIAN_POINT('Ctrl Pts',(-3.56689200468404,1.,-1.61393581747522));
#54542=CARTESIAN_POINT('Ctrl Pts',(-3.56120432482986,1.,-1.60908344685459));
#54543=CARTESIAN_POINT('Ctrl Pts',(-3.55550985096117,1.,-1.60428584699848));
#54544=CARTESIAN_POINT('Ctrl Pts',(-3.54979148634426,1.,-1.59953698113444));
#54545=CARTESIAN_POINT('Ctrl Pts',(-3.544024581823,1.,-1.5948276694975));
#54546=CARTESIAN_POINT('Ctrl Pts',(-3.53818616861045,1.,-1.59014958368725));
#54547=CARTESIAN_POINT('Ctrl Pts',(-3.53226378147068,1.,-1.58549906268083));
#54548=CARTESIAN_POINT('Ctrl Pts',(-3.52626275334899,1.,-1.58088027227856));
#54549=CARTESIAN_POINT('Ctrl Pts',(-3.52021847865961,1.,-1.5763104998818));
#54550=CARTESIAN_POINT('Ctrl Pts',(-3.51418598431733,1.,-1.57181569799774));
#54551=CARTESIAN_POINT('Ctrl Pts',(-3.50821771695427,1.,-1.56742097575041));
#54552=CARTESIAN_POINT('Ctrl Pts',(-3.50234321621607,1.,-1.56314187758689));
#54553=CARTESIAN_POINT('Ctrl Pts',(-3.49655185179623,1.,-1.55897703097859));
#54554=CARTESIAN_POINT('Ctrl Pts',(-3.49076460877317,1.,-1.5548959590107));
#54555=CARTESIAN_POINT('Ctrl Pts',(-3.48485155928414,1.,-1.55084702970382));
#54556=CARTESIAN_POINT('Ctrl Pts',(-3.47868272898599,1.,-1.54678009290206));
#54557=CARTESIAN_POINT('Ctrl Pts',(-3.47217189224576,1.,-1.54266605398152));
#54558=CARTESIAN_POINT('Ctrl Pts',(-3.46531752207222,1.,-1.53851507915533));
#54559=CARTESIAN_POINT('Ctrl Pts',(-3.45825932955273,1.,-1.53440195378902));
#54560=CARTESIAN_POINT('Ctrl Pts',(-3.45127136828667,1.,-1.530462444618));
#54561=CARTESIAN_POINT('Ctrl Pts',(-3.44469547527,1.,-1.52686242875717));
#54562=CARTESIAN_POINT('Ctrl Pts',(-3.43888895974182,1.,-1.52377348950429));
#54563=CARTESIAN_POINT('Ctrl Pts',(-3.43417156977749,1.,-1.52134826724227));
#54564=CARTESIAN_POINT('Ctrl Pts',(-3.43101631893491,1.,-1.5198144909343));
#54565=CARTESIAN_POINT('Ctrl Pts',(-3.42946838852728,1.,-1.51914806898539));
#54566=CARTESIAN_POINT('Ctrl Pts',(-3.42884302333978,1.,-1.51895133295017));
#54567=CARTESIAN_POINT('Ctrl Pts',(-3.42864616361967,1.,-1.51893924967231));
#54568=CARTESIAN_POINT('Ctrl Pts',(-3.42859860294378,1.,-1.51895082866166));
#54569=CARTESIAN_POINT('',(-3.77614523045147,0.,-1.83867539237861));
#54570=CARTESIAN_POINT('Ctrl Pts',(-3.24418789321065,-1.,-1.8808893942881));
#54571=CARTESIAN_POINT('Ctrl Pts',(-3.24418789321065,1.,-1.8808893942881));
#54572=CARTESIAN_POINT('Ctrl Pts',(-3.24410359189733,-1.,-1.8809110068042));
#54573=CARTESIAN_POINT('Ctrl Pts',(-3.24410359189733,1.,-1.8809110068042));
#54574=CARTESIAN_POINT('Ctrl Pts',(-3.24408699284449,-1.,-1.8810220187274));
#54575=CARTESIAN_POINT('Ctrl Pts',(-3.24408699284449,1.,-1.8810220187274));
#54576=CARTESIAN_POINT('Ctrl Pts',(-3.24451807186964,-1.,-1.88139187908347));
#54577=CARTESIAN_POINT('Ctrl Pts',(-3.24451807186964,1.,-1.88139187908347));
#54578=CARTESIAN_POINT('Ctrl Pts',(-3.24600543790876,-1.,-1.88229202583187));
#54579=CARTESIAN_POINT('Ctrl Pts',(-3.24600543790876,1.,-1.88229202583187));
#54580=CARTESIAN_POINT('Ctrl Pts',(-3.24935200512055,-1.,-1.88407708646435));
#54581=CARTESIAN_POINT('Ctrl Pts',(-3.24935200512055,1.,-1.88407708646435));
#54582=CARTESIAN_POINT('Ctrl Pts',(-3.25408686339298,-1.,-1.88646802523372));
#54583=CARTESIAN_POINT('Ctrl Pts',(-3.25408686339298,1.,-1.88646802523372));
#54584=CARTESIAN_POINT('Ctrl Pts',(-3.2599988519361,-1.,-1.88934996203508));
#54585=CARTESIAN_POINT('Ctrl Pts',(-3.2599988519361,1.,-1.88934996203508));
#54586=CARTESIAN_POINT('Ctrl Pts',(-3.2667765388833,-1.,-1.89255393500769));
#54587=CARTESIAN_POINT('Ctrl Pts',(-3.2667765388833,1.,-1.89255393500769));
#54588=CARTESIAN_POINT('Ctrl Pts',(-3.27407108932908,-1.,-1.89589172903662));
#54589=CARTESIAN_POINT('Ctrl Pts',(-3.27407108932908,1.,-1.89589172903662));
#54590=CARTESIAN_POINT('Ctrl Pts',(-3.28154737912287,-1.,-1.89918429230424));
#54591=CARTESIAN_POINT('Ctrl Pts',(-3.28154737912287,1.,-1.89918429230424));
#54592=CARTESIAN_POINT('Ctrl Pts',(-3.28893448600364,-1.,-1.9022897124757));
#54593=CARTESIAN_POINT('Ctrl Pts',(-3.28893448600364,1.,-1.9022897124757));
#54594=CARTESIAN_POINT('Ctrl Pts',(-3.29608978722258,-1.,-1.9051389186417));
#54595=CARTESIAN_POINT('Ctrl Pts',(-3.29608978722258,1.,-1.9051389186417));
#54596=CARTESIAN_POINT('Ctrl Pts',(-3.30300595568341,-1.,-1.90773912171424));
#54597=CARTESIAN_POINT('Ctrl Pts',(-3.30300595568341,1.,-1.90773912171424));
#54598=CARTESIAN_POINT('Ctrl Pts',(-3.30975721158694,-1.,-1.91014297830502));
#54599=CARTESIAN_POINT('Ctrl Pts',(-3.30975721158694,1.,-1.91014297830502));
#54600=CARTESIAN_POINT('Ctrl Pts',(-3.31646052426395,-1.,-1.91242616234459));
#54601=CARTESIAN_POINT('Ctrl Pts',(-3.31646052426395,1.,-1.91242616234459));
#54602=CARTESIAN_POINT('Ctrl Pts',(-3.32323403454507,-1.,-1.91466343916612));
#54603=CARTESIAN_POINT('Ctrl Pts',(-3.32323403454507,1.,-1.91466343916612));
#54604=CARTESIAN_POINT('Ctrl Pts',(-3.33014884257812,-1.,-1.91690081930297));
#54605=CARTESIAN_POINT('Ctrl Pts',(-3.33014884257812,1.,-1.91690081930297));
#54606=CARTESIAN_POINT('Ctrl Pts',(-3.33721230709948,-1.,-1.91914609610173));
#54607=CARTESIAN_POINT('Ctrl Pts',(-3.33721230709948,1.,-1.91914609610173));
#54608=CARTESIAN_POINT('Ctrl Pts',(-3.34439448941915,-1.,-1.92138450828378));
#54609=CARTESIAN_POINT('Ctrl Pts',(-3.34439448941915,1.,-1.92138450828378));
#54610=CARTESIAN_POINT('Ctrl Pts',(-3.35164424847206,-1.,-1.92358838440518));
#54611=CARTESIAN_POINT('Ctrl Pts',(-3.35164424847206,1.,-1.92358838440518));
#54612=CARTESIAN_POINT('Ctrl Pts',(-3.35890824422976,-1.,-1.92572846125763));
#54613=CARTESIAN_POINT('Ctrl Pts',(-3.35890824422976,1.,-1.92572846125763));
#54614=CARTESIAN_POINT('Ctrl Pts',(-3.36615168657597,-1.,-1.92778626543803));
#54615=CARTESIAN_POINT('Ctrl Pts',(-3.36615168657597,1.,-1.92778626543803));
#54616=CARTESIAN_POINT('Ctrl Pts',(-3.37336807068078,-1.,-1.92975993109897));
#54617=CARTESIAN_POINT('Ctrl Pts',(-3.37336807068078,1.,-1.92975993109897));
#54618=CARTESIAN_POINT('Ctrl Pts',(-3.38056768525577,-1.,-1.93165739093292));
#54619=CARTESIAN_POINT('Ctrl Pts',(-3.38056768525577,1.,-1.93165739093292));
#54620=CARTESIAN_POINT('Ctrl Pts',(-3.38777076883267,-1.,-1.93349233176794));
#54621=CARTESIAN_POINT('Ctrl Pts',(-3.38777076883267,1.,-1.93349233176794));
#54622=CARTESIAN_POINT('Ctrl Pts',(-3.39499923640789,-1.,-1.93527929945982));
#54623=CARTESIAN_POINT('Ctrl Pts',(-3.39499923640789,1.,-1.93527929945982));
#54624=CARTESIAN_POINT('Ctrl Pts',(-3.40226802104093,-1.,-1.93702857723089));
#54625=CARTESIAN_POINT('Ctrl Pts',(-3.40226802104093,1.,-1.93702857723089));
#54626=CARTESIAN_POINT('Ctrl Pts',(-3.40957978266622,-1.,-1.93874306008132));
#54627=CARTESIAN_POINT('Ctrl Pts',(-3.40957978266622,1.,-1.93874306008132));
#54628=CARTESIAN_POINT('Ctrl Pts',(-3.41692971994082,-1.,-1.94042111965237));
#54629=CARTESIAN_POINT('Ctrl Pts',(-3.41692971994082,1.,-1.94042111965237));
#54630=CARTESIAN_POINT('Ctrl Pts',(-3.42430850941497,-1.,-1.94205835913692));
#54631=CARTESIAN_POINT('Ctrl Pts',(-3.42430850941497,1.,-1.94205835913692));
#54632=CARTESIAN_POINT('Ctrl Pts',(-3.43170586602436,-1.,-1.94364973660285));
#54633=CARTESIAN_POINT('Ctrl Pts',(-3.43170586602436,1.,-1.94364973660285));
#54634=CARTESIAN_POINT('Ctrl Pts',(-3.43911410197693,-1.,-1.94519168842883));
#54635=CARTESIAN_POINT('Ctrl Pts',(-3.43911410197693,1.,-1.94519168842883));
#54636=CARTESIAN_POINT('Ctrl Pts',(-3.44653088665685,-1.,-1.94668377715332));
#54637=CARTESIAN_POINT('Ctrl Pts',(-3.44653088665685,1.,-1.94668377715332));
#54638=CARTESIAN_POINT('Ctrl Pts',(-3.45395731584051,-1.,-1.94812754766524));
#54639=CARTESIAN_POINT('Ctrl Pts',(-3.45395731584051,1.,-1.94812754766524));
#54640=CARTESIAN_POINT('Ctrl Pts',(-3.46139661060959,-1.,-1.94952575850196));
#54641=CARTESIAN_POINT('Ctrl Pts',(-3.46139661060959,1.,-1.94952575850196));
#54642=CARTESIAN_POINT('Ctrl Pts',(-3.4688525897419,-1.,-1.95088147859876));
#54643=CARTESIAN_POINT('Ctrl Pts',(-3.4688525897419,1.,-1.95088147859876));
#54644=CARTESIAN_POINT('Ctrl Pts',(-3.47632820495926,-1.,-1.95219722189878));
#54645=CARTESIAN_POINT('Ctrl Pts',(-3.47632820495926,1.,-1.95219722189878));
#54646=CARTESIAN_POINT('Ctrl Pts',(-3.48382414832648,-1.,-1.95347412486316));
#54647=CARTESIAN_POINT('Ctrl Pts',(-3.48382414832648,1.,-1.95347412486316));
#54648=CARTESIAN_POINT('Ctrl Pts',(-3.49133956289154,-1.,-1.95471236969653));
#54649=CARTESIAN_POINT('Ctrl Pts',(-3.49133956289154,1.,-1.95471236969653));
#54650=CARTESIAN_POINT('Ctrl Pts',(-3.49887263575602,-1.,-1.9559115382367));
#54651=CARTESIAN_POINT('Ctrl Pts',(-3.49887263575602,1.,-1.9559115382367));
#54652=CARTESIAN_POINT('Ctrl Pts',(-3.50642124159913,-1.,-1.95707099606513));
#54653=CARTESIAN_POINT('Ctrl Pts',(-3.50642124159913,1.,-1.95707099606513));
#54654=CARTESIAN_POINT('Ctrl Pts',(-3.51398354617772,-1.,-1.95819025316768));
#54655=CARTESIAN_POINT('Ctrl Pts',(-3.51398354617772,1.,-1.95819025316768));
#54656=CARTESIAN_POINT('Ctrl Pts',(-3.52155867431438,-1.,-1.95926936324436));
#54657=CARTESIAN_POINT('Ctrl Pts',(-3.52155867431438,1.,-1.95926936324436));
#54658=CARTESIAN_POINT('Ctrl Pts',(-3.52914648844289,-1.,-1.96030879411534));
#54659=CARTESIAN_POINT('Ctrl Pts',(-3.52914648844289,1.,-1.96030879411534));
#54660=CARTESIAN_POINT('Ctrl Pts',(-3.53674730625759,-1.,-1.96130926212661));
#54661=CARTESIAN_POINT('Ctrl Pts',(-3.53674730625759,1.,-1.96130926212661));
#54662=CARTESIAN_POINT('Ctrl Pts',(-3.54436163300425,-1.,-1.96227157573058));
#54663=CARTESIAN_POINT('Ctrl Pts',(-3.54436163300425,1.,-1.96227157573058));
#54664=CARTESIAN_POINT('Ctrl Pts',(-3.55198990600929,-1.,-1.96319648628667));
#54665=CARTESIAN_POINT('Ctrl Pts',(-3.55198990600929,1.,-1.96319648628667));
#54666=CARTESIAN_POINT('Ctrl Pts',(-3.55963218706201,-1.,-1.96408450906868));
#54667=CARTESIAN_POINT('Ctrl Pts',(-3.55963218706201,1.,-1.96408450906868));
#54668=CARTESIAN_POINT('Ctrl Pts',(-3.56728820357933,-1.,-1.96493594634643));
#54669=CARTESIAN_POINT('Ctrl Pts',(-3.56728820357933,1.,-1.96493594634643));
#54670=CARTESIAN_POINT('Ctrl Pts',(-3.57495748601088,-1.,-1.96575096652857));
#54671=CARTESIAN_POINT('Ctrl Pts',(-3.57495748601088,1.,-1.96575096652857));
#54672=CARTESIAN_POINT('Ctrl Pts',(-3.58263947663884,-1.,-1.9665296668894));
#54673=CARTESIAN_POINT('Ctrl Pts',(-3.58263947663884,1.,-1.9665296668894));
#54674=CARTESIAN_POINT('Ctrl Pts',(-3.5903336402273,-1.,-1.96727213799507));
#54675=CARTESIAN_POINT('Ctrl Pts',(-3.5903336402273,1.,-1.96727213799507));
#54676=CARTESIAN_POINT('Ctrl Pts',(-3.59803959819725,-1.,-1.96797854118257));
#54677=CARTESIAN_POINT('Ctrl Pts',(-3.59803959819725,1.,-1.96797854118257));
#54678=CARTESIAN_POINT('Ctrl Pts',(-3.60575714017676,-1.,-1.96864911885775));
#54679=CARTESIAN_POINT('Ctrl Pts',(-3.60575714017676,1.,-1.96864911885775));
#54680=CARTESIAN_POINT('Ctrl Pts',(-3.61348615496393,-1.,-1.96928416040712));
#54681=CARTESIAN_POINT('Ctrl Pts',(-3.61348615496393,1.,-1.96928416040712));
#54682=CARTESIAN_POINT('Ctrl Pts',(-3.62122658401722,-1.,-1.96988398129888));
#54683=CARTESIAN_POINT('Ctrl Pts',(-3.62122658401722,1.,-1.96988398129888));
#54684=CARTESIAN_POINT('Ctrl Pts',(-3.62897836973397,-1.,-1.97044889850518));
#54685=CARTESIAN_POINT('Ctrl Pts',(-3.62897836973397,1.,-1.97044889850518));
#54686=CARTESIAN_POINT('Ctrl Pts',(-3.63674139590853,-1.,-1.97097920454698));
#54687=CARTESIAN_POINT('Ctrl Pts',(-3.63674139590853,1.,-1.97097920454698));
#54688=CARTESIAN_POINT('Ctrl Pts',(-3.64451546724221,-1.,-1.97147515441539));
#54689=CARTESIAN_POINT('Ctrl Pts',(-3.64451546724221,1.,-1.97147515441539));
#54690=CARTESIAN_POINT('Ctrl Pts',(-3.65230034717364,-1.,-1.97193697240645));
#54691=CARTESIAN_POINT('Ctrl Pts',(-3.65230034717364,1.,-1.97193697240645));
#54692=CARTESIAN_POINT('Ctrl Pts',(-3.66009578166865,-1.,-1.97236485439317));
#54693=CARTESIAN_POINT('Ctrl Pts',(-3.66009578166865,1.,-1.97236485439317));
#54694=CARTESIAN_POINT('Ctrl Pts',(-3.66790152751984,-1.,-1.9727589719863));
#54695=CARTESIAN_POINT('Ctrl Pts',(-3.66790152751984,1.,-1.9727589719863));
#54696=CARTESIAN_POINT('Ctrl Pts',(-3.67571738106175,-1.,-1.97311947678035));
#54697=CARTESIAN_POINT('Ctrl Pts',(-3.67571738106175,1.,-1.97311947678035));
#54698=CARTESIAN_POINT('Ctrl Pts',(-3.68354319913416,-1.,-1.9734465030363));
#54699=CARTESIAN_POINT('Ctrl Pts',(-3.68354319913416,1.,-1.9734465030363));
#54700=CARTESIAN_POINT('Ctrl Pts',(-3.69137888597855,-1.,-1.97374016224397));
#54701=CARTESIAN_POINT('Ctrl Pts',(-3.69137888597855,1.,-1.97374016224397));
#54702=CARTESIAN_POINT('Ctrl Pts',(-3.69765528558292,-1.,-1.97394846382288));
#54703=CARTESIAN_POINT('Ctrl Pts',(-3.69765528558292,1.,-1.97394846382288));
#54704=CARTESIAN_POINT('Ctrl Pts',(-3.70236698911837,-1.,-1.97408973726149));
#54705=CARTESIAN_POINT('Ctrl Pts',(-3.70236698911837,1.,-1.97408973726149));
#54706=CARTESIAN_POINT('Ctrl Pts',(-3.7055100813194,-1.,-1.974177276451));
#54707=CARTESIAN_POINT('Ctrl Pts',(-3.7055100813194,1.,-1.974177276451));
#54708=CARTESIAN_POINT('Ctrl Pts',(-3.70708211654725,-1.,-1.97421938526992));
#54709=CARTESIAN_POINT('Ctrl Pts',(-3.70708211654725,1.,-1.97421938526992));
#54710=CARTESIAN_POINT('',(-3.24413672884902,1.,-1.88097764062542));
#54711=CARTESIAN_POINT('Ctrl Pts',(-3.24413672884902,-1.,-1.88097764062542));
#54712=CARTESIAN_POINT('Ctrl Pts',(-3.24413672884902,-0.666666666666667,
-1.88097764062542));
#54713=CARTESIAN_POINT('Ctrl Pts',(-3.24413672884902,-0.333333333333333,
-1.88097764062542));
#54714=CARTESIAN_POINT('Ctrl Pts',(-3.24413672884902,0.333333333333333,
-1.88097764062542));
#54715=CARTESIAN_POINT('Ctrl Pts',(-3.24413672884902,0.666666666666667,
-1.88097764062542));
#54716=CARTESIAN_POINT('Ctrl Pts',(-3.24413672884902,1.,-1.88097764062542));
#54717=CARTESIAN_POINT('',(-3.70708211654725,1.,-1.97421938526992));
#54718=CARTESIAN_POINT('',(-3.70708211654725,0.,-1.97421938526992));
#54719=CARTESIAN_POINT('Ctrl Pts',(-3.24413672884902,1.,-1.88097764062542));
#54720=CARTESIAN_POINT('Ctrl Pts',(-3.24415531671311,1.,-1.88102292397987));
#54721=CARTESIAN_POINT('Ctrl Pts',(-3.24428080352952,1.,-1.88117508446657));
#54722=CARTESIAN_POINT('Ctrl Pts',(-3.24480754675942,1.,-1.88156537699118));
#54723=CARTESIAN_POINT('Ctrl Pts',(-3.24625654410705,1.,-1.88242596600422));
#54724=CARTESIAN_POINT('Ctrl Pts',(-3.24935200512055,1.,-1.88407708646435));
#54725=CARTESIAN_POINT('Ctrl Pts',(-3.25408686339298,1.,-1.88646802523372));
#54726=CARTESIAN_POINT('Ctrl Pts',(-3.2599988519361,1.,-1.88934996203508));
#54727=CARTESIAN_POINT('Ctrl Pts',(-3.2667765388833,1.,-1.89255393500769));
#54728=CARTESIAN_POINT('Ctrl Pts',(-3.27407108932908,1.,-1.89589172903662));
#54729=CARTESIAN_POINT('Ctrl Pts',(-3.28154737912287,1.,-1.89918429230424));
#54730=CARTESIAN_POINT('Ctrl Pts',(-3.28893448600364,1.,-1.9022897124757));
#54731=CARTESIAN_POINT('Ctrl Pts',(-3.29608978722258,1.,-1.9051389186417));
#54732=CARTESIAN_POINT('Ctrl Pts',(-3.30300595568341,1.,-1.90773912171424));
#54733=CARTESIAN_POINT('Ctrl Pts',(-3.30975721158694,1.,-1.91014297830502));
#54734=CARTESIAN_POINT('Ctrl Pts',(-3.31646052426395,1.,-1.91242616234459));
#54735=CARTESIAN_POINT('Ctrl Pts',(-3.32323403454507,1.,-1.91466343916612));
#54736=CARTESIAN_POINT('Ctrl Pts',(-3.33014884257812,1.,-1.91690081930297));
#54737=CARTESIAN_POINT('Ctrl Pts',(-3.33721230709948,1.,-1.91914609610173));
#54738=CARTESIAN_POINT('Ctrl Pts',(-3.34439448941915,1.,-1.92138450828378));
#54739=CARTESIAN_POINT('Ctrl Pts',(-3.35164424847206,1.,-1.92358838440518));
#54740=CARTESIAN_POINT('Ctrl Pts',(-3.35890824422976,1.,-1.92572846125763));
#54741=CARTESIAN_POINT('Ctrl Pts',(-3.36615168657597,1.,-1.92778626543803));
#54742=CARTESIAN_POINT('Ctrl Pts',(-3.37336807068078,1.,-1.92975993109897));
#54743=CARTESIAN_POINT('Ctrl Pts',(-3.38056768525577,1.,-1.93165739093292));
#54744=CARTESIAN_POINT('Ctrl Pts',(-3.38777076883267,1.,-1.93349233176794));
#54745=CARTESIAN_POINT('Ctrl Pts',(-3.39499923640789,1.,-1.93527929945982));
#54746=CARTESIAN_POINT('Ctrl Pts',(-3.40226802104093,1.,-1.93702857723089));
#54747=CARTESIAN_POINT('Ctrl Pts',(-3.40957978266622,1.,-1.93874306008132));
#54748=CARTESIAN_POINT('Ctrl Pts',(-3.41692971994082,1.,-1.94042111965237));
#54749=CARTESIAN_POINT('Ctrl Pts',(-3.42430850941497,1.,-1.94205835913692));
#54750=CARTESIAN_POINT('Ctrl Pts',(-3.43170586602436,1.,-1.94364973660285));
#54751=CARTESIAN_POINT('Ctrl Pts',(-3.43911410197693,1.,-1.94519168842883));
#54752=CARTESIAN_POINT('Ctrl Pts',(-3.44653088665685,1.,-1.94668377715332));
#54753=CARTESIAN_POINT('Ctrl Pts',(-3.45395731584051,1.,-1.94812754766524));
#54754=CARTESIAN_POINT('Ctrl Pts',(-3.46139661060959,1.,-1.94952575850196));
#54755=CARTESIAN_POINT('Ctrl Pts',(-3.4688525897419,1.,-1.95088147859876));
#54756=CARTESIAN_POINT('Ctrl Pts',(-3.47632820495926,1.,-1.95219722189878));
#54757=CARTESIAN_POINT('Ctrl Pts',(-3.48382414832648,1.,-1.95347412486316));
#54758=CARTESIAN_POINT('Ctrl Pts',(-3.49133956289154,1.,-1.95471236969653));
#54759=CARTESIAN_POINT('Ctrl Pts',(-3.49887263575602,1.,-1.9559115382367));
#54760=CARTESIAN_POINT('Ctrl Pts',(-3.50642124159913,1.,-1.95707099606513));
#54761=CARTESIAN_POINT('Ctrl Pts',(-3.51398354617772,1.,-1.95819025316768));
#54762=CARTESIAN_POINT('Ctrl Pts',(-3.52155867431438,1.,-1.95926936324436));
#54763=CARTESIAN_POINT('Ctrl Pts',(-3.52914648844289,1.,-1.96030879411534));
#54764=CARTESIAN_POINT('Ctrl Pts',(-3.53674730625759,1.,-1.96130926212661));
#54765=CARTESIAN_POINT('Ctrl Pts',(-3.54436163300425,1.,-1.96227157573058));
#54766=CARTESIAN_POINT('Ctrl Pts',(-3.55198990600929,1.,-1.96319648628667));
#54767=CARTESIAN_POINT('Ctrl Pts',(-3.55963218706201,1.,-1.96408450906868));
#54768=CARTESIAN_POINT('Ctrl Pts',(-3.56728820357933,1.,-1.96493594634643));
#54769=CARTESIAN_POINT('Ctrl Pts',(-3.57495748601088,1.,-1.96575096652857));
#54770=CARTESIAN_POINT('Ctrl Pts',(-3.58263947663884,1.,-1.9665296668894));
#54771=CARTESIAN_POINT('Ctrl Pts',(-3.5903336402273,1.,-1.96727213799507));
#54772=CARTESIAN_POINT('Ctrl Pts',(-3.59803959819725,1.,-1.96797854118257));
#54773=CARTESIAN_POINT('Ctrl Pts',(-3.60575714017676,1.,-1.96864911885775));
#54774=CARTESIAN_POINT('Ctrl Pts',(-3.61348615496393,1.,-1.96928416040712));
#54775=CARTESIAN_POINT('Ctrl Pts',(-3.62122658401722,1.,-1.96988398129888));
#54776=CARTESIAN_POINT('Ctrl Pts',(-3.62897836973397,1.,-1.97044889850518));
#54777=CARTESIAN_POINT('Ctrl Pts',(-3.63674139590853,1.,-1.97097920454698));
#54778=CARTESIAN_POINT('Ctrl Pts',(-3.64451546724221,1.,-1.97147515441539));
#54779=CARTESIAN_POINT('Ctrl Pts',(-3.65230034717364,1.,-1.97193697240645));
#54780=CARTESIAN_POINT('Ctrl Pts',(-3.66009578166865,1.,-1.97236485439317));
#54781=CARTESIAN_POINT('Ctrl Pts',(-3.66790152751984,1.,-1.9727589719863));
#54782=CARTESIAN_POINT('Ctrl Pts',(-3.67571738106175,1.,-1.97311947678035));
#54783=CARTESIAN_POINT('Ctrl Pts',(-3.68354319913416,1.,-1.9734465030363));
#54784=CARTESIAN_POINT('Ctrl Pts',(-3.69137888597855,1.,-1.97374016224397));
#54785=CARTESIAN_POINT('Ctrl Pts',(-3.69765528558292,1.,-1.97394846382288));
#54786=CARTESIAN_POINT('Ctrl Pts',(-3.70236698911837,1.,-1.97408973726149));
#54787=CARTESIAN_POINT('Ctrl Pts',(-3.7055100813194,1.,-1.974177276451));
#54788=CARTESIAN_POINT('Ctrl Pts',(-3.70708211654725,1.,-1.97421938526992));
#54789=CARTESIAN_POINT('Origin',(-3.70708211654725,0.,-1.97421938526992));
#54790=CARTESIAN_POINT('',(-3.77614523045147,1.,-1.83867539237861));
#54791=CARTESIAN_POINT('Origin',(0.,0.,0.));
#54792=CARTESIAN_POINT('',(-3.14877060440425,1.,-2.03660101169564));
#54793=CARTESIAN_POINT('Origin',(0.,1.,0.));
#54794=CARTESIAN_POINT('Ctrl Pts',(-3.14877060440425,1.,-2.03660101169564));
#54795=CARTESIAN_POINT('Ctrl Pts',(-3.14877060440425,0.666666666666667,
-2.03660101169564));
#54796=CARTESIAN_POINT('Ctrl Pts',(-3.14877060440425,0.333333333333333,
-2.03660101169564));
#54797=CARTESIAN_POINT('Ctrl Pts',(-3.14877060440425,-0.333333333333333,
-2.03660101169564));
#54798=CARTESIAN_POINT('Ctrl Pts',(-3.14877060440425,-0.666666666666667,
-2.03660101169564));
#54799=CARTESIAN_POINT('Ctrl Pts',(-3.14877060440425,-1.,-2.03660101169564));
#54800=CARTESIAN_POINT('Ctrl Pts',(-3.44202241512147,-1.,-2.40675750623143));
#54801=CARTESIAN_POINT('Ctrl Pts',(-3.44202241512147,1.,-2.40675750623143));
#54802=CARTESIAN_POINT('Ctrl Pts',(-3.44127120683402,-1.,-2.40537592959345));
#54803=CARTESIAN_POINT('Ctrl Pts',(-3.44127120683402,1.,-2.40537592959345));
#54804=CARTESIAN_POINT('Ctrl Pts',(-3.43976627485223,-1.,-2.40261515590099));
#54805=CARTESIAN_POINT('Ctrl Pts',(-3.43976627485223,1.,-2.40261515590099));
#54806=CARTESIAN_POINT('Ctrl Pts',(-3.43750133066036,-1.,-2.39848113411429));
#54807=CARTESIAN_POINT('Ctrl Pts',(-3.43750133066036,1.,-2.39848113411429));
#54808=CARTESIAN_POINT('Ctrl Pts',(-3.43446630680436,-1.,-2.39298338805823));
#54809=CARTESIAN_POINT('Ctrl Pts',(-3.43446630680436,1.,-2.39298338805823));
#54810=CARTESIAN_POINT('Ctrl Pts',(-3.43064732714472,-1.,-2.38613505844641));
#54811=CARTESIAN_POINT('Ctrl Pts',(-3.43064732714472,1.,-2.38613505844641));
#54812=CARTESIAN_POINT('Ctrl Pts',(-3.42680309755241,-1.,-2.37931067029517));
#54813=CARTESIAN_POINT('Ctrl Pts',(-3.42680309755241,1.,-2.37931067029517));
#54814=CARTESIAN_POINT('Ctrl Pts',(-3.42293356216595,-1.,-2.37251035954351));
#54815=CARTESIAN_POINT('Ctrl Pts',(-3.42293356216595,1.,-2.37251035954351));
#54816=CARTESIAN_POINT('Ctrl Pts',(-3.41903866635384,-1.,-2.36573431470314));
#54817=CARTESIAN_POINT('Ctrl Pts',(-3.41903866635384,1.,-2.36573431470314));
#54818=CARTESIAN_POINT('Ctrl Pts',(-3.4151183675076,-1.,-2.35898278606449));
#54819=CARTESIAN_POINT('Ctrl Pts',(-3.4151183675076,1.,-2.35898278606449));
#54820=CARTESIAN_POINT('Ctrl Pts',(-3.41117262313464,-1.,-2.35225606823649));
#54821=CARTESIAN_POINT('Ctrl Pts',(-3.41117262313464,1.,-2.35225606823649));
#54822=CARTESIAN_POINT('Ctrl Pts',(-3.40720137403888,-1.,-2.34555447648901));
#54823=CARTESIAN_POINT('Ctrl Pts',(-3.40720137403888,1.,-2.34555447648901));
#54824=CARTESIAN_POINT('Ctrl Pts',(-3.40320452776646,-1.,-2.33887832342715));
#54825=CARTESIAN_POINT('Ctrl Pts',(-3.40320452776646,1.,-2.33887832342715));
#54826=CARTESIAN_POINT('Ctrl Pts',(-3.39918194578115,-1.,-2.33222789882601));
#54827=CARTESIAN_POINT('Ctrl Pts',(-3.39918194578115,1.,-2.33222789882601));
#54828=CARTESIAN_POINT('Ctrl Pts',(-3.39513342020045,-1.,-2.32560343902683));
#54829=CARTESIAN_POINT('Ctrl Pts',(-3.39513342020045,1.,-2.32560343902683));
#54830=CARTESIAN_POINT('Ctrl Pts',(-3.39105869475112,-1.,-2.31900513925627));
#54831=CARTESIAN_POINT('Ctrl Pts',(-3.39105869475112,1.,-2.31900513925627));
#54832=CARTESIAN_POINT('Ctrl Pts',(-3.38695751492659,-1.,-2.31243319489505));
#54833=CARTESIAN_POINT('Ctrl Pts',(-3.38695751492659,1.,-2.31243319489505));
#54834=CARTESIAN_POINT('Ctrl Pts',(-3.38282967336676,-1.,-2.30588783640389));
#54835=CARTESIAN_POINT('Ctrl Pts',(-3.38282967336676,1.,-2.30588783640389));
#54836=CARTESIAN_POINT('Ctrl Pts',(-3.37867504959382,-1.,-2.29936936127588));
#54837=CARTESIAN_POINT('Ctrl Pts',(-3.37867504959382,1.,-2.29936936127588));
#54838=CARTESIAN_POINT('Ctrl Pts',(-3.37449367172707,-1.,-2.2928781800731));
#54839=CARTESIAN_POINT('Ctrl Pts',(-3.37449367172707,1.,-2.2928781800731));
#54840=CARTESIAN_POINT('Ctrl Pts',(-3.37028570206357,-1.,-2.28641481081045));
#54841=CARTESIAN_POINT('Ctrl Pts',(-3.37028570206357,1.,-2.28641481081045));
#54842=CARTESIAN_POINT('Ctrl Pts',(-3.36605130712978,-1.,-2.27997979457968));
#54843=CARTESIAN_POINT('Ctrl Pts',(-3.36605130712978,1.,-2.27997979457968));
#54844=CARTESIAN_POINT('Ctrl Pts',(-3.36179055004369,-1.,-2.27357362620902));
#54845=CARTESIAN_POINT('Ctrl Pts',(-3.36179055004369,1.,-2.27357362620902));
#54846=CARTESIAN_POINT('Ctrl Pts',(-3.35750328523077,-1.,-2.26719668579921));
#54847=CARTESIAN_POINT('Ctrl Pts',(-3.35750328523077,1.,-2.26719668579921));
#54848=CARTESIAN_POINT('Ctrl Pts',(-3.35318902552676,-1.,-2.26084915222484));
#54849=CARTESIAN_POINT('Ctrl Pts',(-3.35318902552676,1.,-2.26084915222484));
#54850=CARTESIAN_POINT('Ctrl Pts',(-3.34884690292342,-1.,-2.25453097693524));
#54851=CARTESIAN_POINT('Ctrl Pts',(-3.34884690292342,1.,-2.25453097693524));
#54852=CARTESIAN_POINT('Ctrl Pts',(-3.34447596770768,-1.,-2.24824207678288));
#54853=CARTESIAN_POINT('Ctrl Pts',(-3.34447596770768,1.,-2.24824207678288));
#54854=CARTESIAN_POINT('Ctrl Pts',(-3.34007543738044,-1.,-2.24198249391437));
#54855=CARTESIAN_POINT('Ctrl Pts',(-3.34007543738044,1.,-2.24198249391437));
#54856=CARTESIAN_POINT('Ctrl Pts',(-3.33564495756478,-1.,-2.2357525632881));
#54857=CARTESIAN_POINT('Ctrl Pts',(-3.33564495756478,1.,-2.2357525632881));
#54858=CARTESIAN_POINT('Ctrl Pts',(-3.33118487773593,-1.,-2.22955308907221));
#54859=CARTESIAN_POINT('Ctrl Pts',(-3.33118487773593,1.,-2.22955308907221));
#54860=CARTESIAN_POINT('Ctrl Pts',(-3.32669646722871,-1.,-2.22338548312758));
#54861=CARTESIAN_POINT('Ctrl Pts',(-3.32669646722871,1.,-2.22338548312758));
#54862=CARTESIAN_POINT('Ctrl Pts',(-3.32218125618955,-1.,-2.21725135110889));
#54863=CARTESIAN_POINT('Ctrl Pts',(-3.32218125618955,1.,-2.21725135110889));
#54864=CARTESIAN_POINT('Ctrl Pts',(-3.31764044024231,-1.,-2.21115211847872));
#54865=CARTESIAN_POINT('Ctrl Pts',(-3.31764044024231,1.,-2.21115211847872));
#54866=CARTESIAN_POINT('Ctrl Pts',(-3.3130742460895,-1.,-2.20508863150608));
#54867=CARTESIAN_POINT('Ctrl Pts',(-3.3130742460895,1.,-2.20508863150608));
#54868=CARTESIAN_POINT('Ctrl Pts',(-3.30848134694596,-1.,-2.19906078949924));
#54869=CARTESIAN_POINT('Ctrl Pts',(-3.30848134694596,1.,-2.19906078949924));
#54870=CARTESIAN_POINT('Ctrl Pts',(-3.30385816281831,-1.,-2.19306710376112));
#54871=CARTESIAN_POINT('Ctrl Pts',(-3.30385816281831,1.,-2.19306710376112));
#54872=CARTESIAN_POINT('Ctrl Pts',(-3.29920022557635,-1.,-2.18710556500325));
#54873=CARTESIAN_POINT('Ctrl Pts',(-3.29920022557635,1.,-2.18710556500325));
#54874=CARTESIAN_POINT('Ctrl Pts',(-3.29450361500484,-1.,-2.18117455557062));
#54875=CARTESIAN_POINT('Ctrl Pts',(-3.29450361500484,1.,-2.18117455557062));
#54876=CARTESIAN_POINT('Ctrl Pts',(-3.28976645712566,-1.,-2.17527380048422));
#54877=CARTESIAN_POINT('Ctrl Pts',(-3.28976645712566,1.,-2.17527380048422));
#54878=CARTESIAN_POINT('Ctrl Pts',(-3.2849901997973,-1.,-2.16940517773459));
#54879=CARTESIAN_POINT('Ctrl Pts',(-3.2849901997973,1.,-2.16940517773459));
#54880=CARTESIAN_POINT('Ctrl Pts',(-3.28018150841414,-1.,-2.16357391934434));
#54881=CARTESIAN_POINT('Ctrl Pts',(-3.28018150841414,1.,-2.16357391934434));
#54882=CARTESIAN_POINT('Ctrl Pts',(-3.27534954469206,-1.,-2.15778690038359));
#54883=CARTESIAN_POINT('Ctrl Pts',(-3.27534954469206,1.,-2.15778690038359));
#54884=CARTESIAN_POINT('Ctrl Pts',(-3.27050245897244,-1.,-2.15205043199818));
#54885=CARTESIAN_POINT('Ctrl Pts',(-3.27050245897244,1.,-2.15205043199818));
#54886=CARTESIAN_POINT('Ctrl Pts',(-3.26564388189764,-1.,-2.14636805295663));
#54887=CARTESIAN_POINT('Ctrl Pts',(-3.26564388189764,1.,-2.14636805295663));
#54888=CARTESIAN_POINT('Ctrl Pts',(-3.26077002641868,-1.,-2.14073870754257));
#54889=CARTESIAN_POINT('Ctrl Pts',(-3.26077002641868,1.,-2.14073870754257));
#54890=CARTESIAN_POINT('Ctrl Pts',(-3.25586495065027,-1.,-2.13515375878786));
#54891=CARTESIAN_POINT('Ctrl Pts',(-3.25586495065027,1.,-2.13515375878786));
#54892=CARTESIAN_POINT('Ctrl Pts',(-3.25090574493994,-1.,-2.1296002839681));
#54893=CARTESIAN_POINT('Ctrl Pts',(-3.25090574493994,1.,-2.1296002839681));
#54894=CARTESIAN_POINT('Ctrl Pts',(-3.24587102613347,-1.,-2.12406646410943));
#54895=CARTESIAN_POINT('Ctrl Pts',(-3.24587102613347,1.,-2.12406646410943));
#54896=CARTESIAN_POINT('Ctrl Pts',(-3.24074905517282,-1.,-2.11854673326972));
#54897=CARTESIAN_POINT('Ctrl Pts',(-3.24074905517282,1.,-2.11854673326972));
#54898=CARTESIAN_POINT('Ctrl Pts',(-3.23554444767115,-1.,-2.11304604021784));
#54899=CARTESIAN_POINT('Ctrl Pts',(-3.23554444767115,1.,-2.11304604021784));
#54900=CARTESIAN_POINT('Ctrl Pts',(-3.23028945793334,-1.,-2.1075869964248));
#54901=CARTESIAN_POINT('Ctrl Pts',(-3.23028945793334,1.,-2.1075869964248));
#54902=CARTESIAN_POINT('Ctrl Pts',(-3.22503437553496,-1.,-2.10220384298533));
#54903=CARTESIAN_POINT('Ctrl Pts',(-3.22503437553496,1.,-2.10220384298533));
#54904=CARTESIAN_POINT('Ctrl Pts',(-3.21982707347067,-1.,-2.09692958434933));
#54905=CARTESIAN_POINT('Ctrl Pts',(-3.21982707347067,1.,-2.09692958434933));
#54906=CARTESIAN_POINT('Ctrl Pts',(-3.2146942960168,-1.,-2.0917841946046));
#54907=CARTESIAN_POINT('Ctrl Pts',(-3.2146942960168,1.,-2.0917841946046));
#54908=CARTESIAN_POINT('Ctrl Pts',(-3.20962575845433,-1.,-2.08676465517435));
#54909=CARTESIAN_POINT('Ctrl Pts',(-3.20962575845433,1.,-2.08676465517435));
#54910=CARTESIAN_POINT('Ctrl Pts',(-3.20454818630635,-1.,-2.08182850370816));
#54911=CARTESIAN_POINT('Ctrl Pts',(-3.20454818630635,1.,-2.08182850370816));
#54912=CARTESIAN_POINT('Ctrl Pts',(-3.19934132835879,-1.,-2.0769044187063));
#54913=CARTESIAN_POINT('Ctrl Pts',(-3.19934132835879,1.,-2.0769044187063));
#54914=CARTESIAN_POINT('Ctrl Pts',(-3.19388465568113,-1.,-2.07192253497765));
#54915=CARTESIAN_POINT('Ctrl Pts',(-3.19388465568113,1.,-2.07192253497765));
#54916=CARTESIAN_POINT('Ctrl Pts',(-3.18809755562297,-1.,-2.06684062744065));
#54917=CARTESIAN_POINT('Ctrl Pts',(-3.18809755562297,1.,-2.06684062744065));
#54918=CARTESIAN_POINT('Ctrl Pts',(-3.18197692964677,-1.,-2.06166849827143));
#54919=CARTESIAN_POINT('Ctrl Pts',(-3.18197692964677,1.,-2.06166849827143));
#54920=CARTESIAN_POINT('Ctrl Pts',(-3.17564906975592,-1.,-2.05650186773279));
#54921=CARTESIAN_POINT('Ctrl Pts',(-3.17564906975592,1.,-2.05650186773279));
#54922=CARTESIAN_POINT('Ctrl Pts',(-3.16936341689859,-1.,-2.05151770247452));
#54923=CARTESIAN_POINT('Ctrl Pts',(-3.16936341689859,1.,-2.05151770247452));
#54924=CARTESIAN_POINT('Ctrl Pts',(-3.16343165059235,-1.,-2.0469333124766));
#54925=CARTESIAN_POINT('Ctrl Pts',(-3.16343165059235,1.,-2.0469333124766));
#54926=CARTESIAN_POINT('Ctrl Pts',(-3.15817983946525,-1.,-2.04297406404132));
#54927=CARTESIAN_POINT('Ctrl Pts',(-3.15817983946525,1.,-2.04297406404132));
#54928=CARTESIAN_POINT('Ctrl Pts',(-3.1538999167466,-1.,-2.03984073791432));
#54929=CARTESIAN_POINT('Ctrl Pts',(-3.1538999167466,1.,-2.03984073791432));
#54930=CARTESIAN_POINT('Ctrl Pts',(-3.15079010635326,-1.,-2.03766932526171));
#54931=CARTESIAN_POINT('Ctrl Pts',(-3.15079010635326,1.,-2.03766932526171));
#54932=CARTESIAN_POINT('Ctrl Pts',(-3.14931281967585,-1.,-2.03675273048882));
#54933=CARTESIAN_POINT('Ctrl Pts',(-3.14931281967585,1.,-2.03675273048882));
#54934=CARTESIAN_POINT('Ctrl Pts',(-3.14878756590499,-1.,-2.03653654935384));
#54935=CARTESIAN_POINT('Ctrl Pts',(-3.14878756590499,1.,-2.03653654935384));
#54936=CARTESIAN_POINT('Ctrl Pts',(-3.14869618937138,-1.,-2.036601737578));
#54937=CARTESIAN_POINT('Ctrl Pts',(-3.14869618937138,1.,-2.036601737578));
#54938=CARTESIAN_POINT('Ctrl Pts',(-3.1487152044751,-1.,-2.03668666247593));
#54939=CARTESIAN_POINT('Ctrl Pts',(-3.1487152044751,1.,-2.03668666247593));
#54940=CARTESIAN_POINT('',(-3.44202241512147,1.,-2.40675750623143));
#54941=CARTESIAN_POINT('Ctrl Pts',(-3.44202241512147,1.,-2.40675750623143));
#54942=CARTESIAN_POINT('Ctrl Pts',(-3.44127120683402,1.,-2.40537592959345));
#54943=CARTESIAN_POINT('Ctrl Pts',(-3.43976627485223,1.,-2.40261515590099));
#54944=CARTESIAN_POINT('Ctrl Pts',(-3.43750133066036,1.,-2.39848113411429));
#54945=CARTESIAN_POINT('Ctrl Pts',(-3.43446630680436,1.,-2.39298338805823));
#54946=CARTESIAN_POINT('Ctrl Pts',(-3.43064732714472,1.,-2.38613505844641));
#54947=CARTESIAN_POINT('Ctrl Pts',(-3.42680309755241,1.,-2.37931067029517));
#54948=CARTESIAN_POINT('Ctrl Pts',(-3.42293356216595,1.,-2.37251035954351));
#54949=CARTESIAN_POINT('Ctrl Pts',(-3.41903866635384,1.,-2.36573431470314));
#54950=CARTESIAN_POINT('Ctrl Pts',(-3.4151183675076,1.,-2.35898278606449));
#54951=CARTESIAN_POINT('Ctrl Pts',(-3.41117262313464,1.,-2.35225606823649));
#54952=CARTESIAN_POINT('Ctrl Pts',(-3.40720137403888,1.,-2.34555447648901));
#54953=CARTESIAN_POINT('Ctrl Pts',(-3.40320452776646,1.,-2.33887832342715));
#54954=CARTESIAN_POINT('Ctrl Pts',(-3.39918194578115,1.,-2.33222789882601));
#54955=CARTESIAN_POINT('Ctrl Pts',(-3.39513342020045,1.,-2.32560343902683));
#54956=CARTESIAN_POINT('Ctrl Pts',(-3.39105869475112,1.,-2.31900513925627));
#54957=CARTESIAN_POINT('Ctrl Pts',(-3.38695751492659,1.,-2.31243319489505));
#54958=CARTESIAN_POINT('Ctrl Pts',(-3.38282967336676,1.,-2.30588783640389));
#54959=CARTESIAN_POINT('Ctrl Pts',(-3.37867504959382,1.,-2.29936936127588));
#54960=CARTESIAN_POINT('Ctrl Pts',(-3.37449367172707,1.,-2.2928781800731));
#54961=CARTESIAN_POINT('Ctrl Pts',(-3.37028570206357,1.,-2.28641481081045));
#54962=CARTESIAN_POINT('Ctrl Pts',(-3.36605130712978,1.,-2.27997979457968));
#54963=CARTESIAN_POINT('Ctrl Pts',(-3.36179055004369,1.,-2.27357362620902));
#54964=CARTESIAN_POINT('Ctrl Pts',(-3.35750328523077,1.,-2.26719668579921));
#54965=CARTESIAN_POINT('Ctrl Pts',(-3.35318902552676,1.,-2.26084915222484));
#54966=CARTESIAN_POINT('Ctrl Pts',(-3.34884690292342,1.,-2.25453097693524));
#54967=CARTESIAN_POINT('Ctrl Pts',(-3.34447596770768,1.,-2.24824207678288));
#54968=CARTESIAN_POINT('Ctrl Pts',(-3.34007543738044,1.,-2.24198249391437));
#54969=CARTESIAN_POINT('Ctrl Pts',(-3.33564495756478,1.,-2.2357525632881));
#54970=CARTESIAN_POINT('Ctrl Pts',(-3.33118487773593,1.,-2.22955308907221));
#54971=CARTESIAN_POINT('Ctrl Pts',(-3.32669646722871,1.,-2.22338548312758));
#54972=CARTESIAN_POINT('Ctrl Pts',(-3.32218125618955,1.,-2.21725135110889));
#54973=CARTESIAN_POINT('Ctrl Pts',(-3.31764044024231,1.,-2.21115211847872));
#54974=CARTESIAN_POINT('Ctrl Pts',(-3.3130742460895,1.,-2.20508863150608));
#54975=CARTESIAN_POINT('Ctrl Pts',(-3.30848134694596,1.,-2.19906078949924));
#54976=CARTESIAN_POINT('Ctrl Pts',(-3.30385816281831,1.,-2.19306710376112));
#54977=CARTESIAN_POINT('Ctrl Pts',(-3.29920022557635,1.,-2.18710556500325));
#54978=CARTESIAN_POINT('Ctrl Pts',(-3.29450361500484,1.,-2.18117455557062));
#54979=CARTESIAN_POINT('Ctrl Pts',(-3.28976645712566,1.,-2.17527380048422));
#54980=CARTESIAN_POINT('Ctrl Pts',(-3.2849901997973,1.,-2.16940517773459));
#54981=CARTESIAN_POINT('Ctrl Pts',(-3.28018150841414,1.,-2.16357391934434));
#54982=CARTESIAN_POINT('Ctrl Pts',(-3.27534954469206,1.,-2.15778690038359));
#54983=CARTESIAN_POINT('Ctrl Pts',(-3.27050245897244,1.,-2.15205043199818));
#54984=CARTESIAN_POINT('Ctrl Pts',(-3.26564388189764,1.,-2.14636805295663));
#54985=CARTESIAN_POINT('Ctrl Pts',(-3.26077002641868,1.,-2.14073870754257));
#54986=CARTESIAN_POINT('Ctrl Pts',(-3.25586495065027,1.,-2.13515375878786));
#54987=CARTESIAN_POINT('Ctrl Pts',(-3.25090574493994,1.,-2.1296002839681));
#54988=CARTESIAN_POINT('Ctrl Pts',(-3.24587102613347,1.,-2.12406646410943));
#54989=CARTESIAN_POINT('Ctrl Pts',(-3.24074905517282,1.,-2.11854673326972));
#54990=CARTESIAN_POINT('Ctrl Pts',(-3.23554444767115,1.,-2.11304604021784));
#54991=CARTESIAN_POINT('Ctrl Pts',(-3.23028945793334,1.,-2.1075869964248));
#54992=CARTESIAN_POINT('Ctrl Pts',(-3.22503437553496,1.,-2.10220384298533));
#54993=CARTESIAN_POINT('Ctrl Pts',(-3.21982707347067,1.,-2.09692958434933));
#54994=CARTESIAN_POINT('Ctrl Pts',(-3.2146942960168,1.,-2.0917841946046));
#54995=CARTESIAN_POINT('Ctrl Pts',(-3.20962575845433,1.,-2.08676465517435));
#54996=CARTESIAN_POINT('Ctrl Pts',(-3.20454818630635,1.,-2.08182850370816));
#54997=CARTESIAN_POINT('Ctrl Pts',(-3.19934132835879,1.,-2.0769044187063));
#54998=CARTESIAN_POINT('Ctrl Pts',(-3.19388465568113,1.,-2.07192253497765));
#54999=CARTESIAN_POINT('Ctrl Pts',(-3.18809755562297,1.,-2.06684062744065));
#55000=CARTESIAN_POINT('Ctrl Pts',(-3.18197692964677,1.,-2.06166849827143));
#55001=CARTESIAN_POINT('Ctrl Pts',(-3.17564906975592,1.,-2.05650186773279));
#55002=CARTESIAN_POINT('Ctrl Pts',(-3.16936341689859,1.,-2.05151770247452));
#55003=CARTESIAN_POINT('Ctrl Pts',(-3.16343165059235,1.,-2.0469333124766));
#55004=CARTESIAN_POINT('Ctrl Pts',(-3.15817983946525,1.,-2.04297406404132));
#55005=CARTESIAN_POINT('Ctrl Pts',(-3.1538999167466,1.,-2.03984073791432));
#55006=CARTESIAN_POINT('Ctrl Pts',(-3.15102344775396,1.,-2.03783225496023));
#55007=CARTESIAN_POINT('Ctrl Pts',(-3.14959882629936,1.,-2.03693188810614));
#55008=CARTESIAN_POINT('Ctrl Pts',(-3.14901193669147,1.,-2.03663974554941));
#55009=CARTESIAN_POINT('Ctrl Pts',(-3.1488193908823,1.,-2.03659701539175));
#55010=CARTESIAN_POINT('Ctrl Pts',(-3.14877060440425,1.,-2.03660101169564));
#55011=CARTESIAN_POINT('',(-3.44202241512147,0.,-2.40675750623143));
#55012=CARTESIAN_POINT('Ctrl Pts',(-2.91001063062876,-1.,-2.36523532225181));
#55013=CARTESIAN_POINT('Ctrl Pts',(-2.91001063062876,1.,-2.36523532225181));
#55014=CARTESIAN_POINT('Ctrl Pts',(-2.90992398626211,-1.,-2.36524348105112));
#55015=CARTESIAN_POINT('Ctrl Pts',(-2.90992398626211,1.,-2.36524348105112));
#55016=CARTESIAN_POINT('Ctrl Pts',(-2.90989022548032,-1.,-2.36535052956938));
#55017=CARTESIAN_POINT('Ctrl Pts',(-2.90989022548032,1.,-2.36535052956938));
#55018=CARTESIAN_POINT('Ctrl Pts',(-2.91025813830041,-1.,-2.36578327194741));
#55019=CARTESIAN_POINT('Ctrl Pts',(-2.91025813830041,1.,-2.36578327194741));
#55020=CARTESIAN_POINT('Ctrl Pts',(-2.9115863784204,-1.,-2.36690501170627));
#55021=CARTESIAN_POINT('Ctrl Pts',(-2.9115863784204,1.,-2.36690501170627));
#55022=CARTESIAN_POINT('Ctrl Pts',(-2.9146124988314,-1.,-2.36919161373173));
#55023=CARTESIAN_POINT('Ctrl Pts',(-2.9146124988314,1.,-2.36919161373173));
#55024=CARTESIAN_POINT('Ctrl Pts',(-2.91891503791411,-1.,-2.37229381109821));
#55025=CARTESIAN_POINT('Ctrl Pts',(-2.91891503791411,1.,-2.37229381109821));
#55026=CARTESIAN_POINT('Ctrl Pts',(-2.92430340582608,-1.,-2.3760651052403));
#55027=CARTESIAN_POINT('Ctrl Pts',(-2.92430340582608,1.,-2.3760651052403));
#55028=CARTESIAN_POINT('Ctrl Pts',(-2.93049643640206,-1.,-2.38028989582073));
#55029=CARTESIAN_POINT('Ctrl Pts',(-2.93049643640206,1.,-2.38028989582073));
#55030=CARTESIAN_POINT('Ctrl Pts',(-2.93717903280391,-1.,-2.38472771516311));
#55031=CARTESIAN_POINT('Ctrl Pts',(-2.93717903280391,1.,-2.38472771516311));
#55032=CARTESIAN_POINT('Ctrl Pts',(-2.94404820669076,-1.,-2.38914929090759));
#55033=CARTESIAN_POINT('Ctrl Pts',(-2.94404820669076,1.,-2.38914929090759));
#55034=CARTESIAN_POINT('Ctrl Pts',(-2.95085857128439,-1.,-2.39337207631667));
#55035=CARTESIAN_POINT('Ctrl Pts',(-2.95085857128439,1.,-2.39337207631667));
#55036=CARTESIAN_POINT('Ctrl Pts',(-2.95748006482942,-1.,-2.39730553974517));
#55037=CARTESIAN_POINT('Ctrl Pts',(-2.95748006482942,1.,-2.39730553974517));
#55038=CARTESIAN_POINT('Ctrl Pts',(-2.96390432240312,-1.,-2.4009556571164));
#55039=CARTESIAN_POINT('Ctrl Pts',(-2.96390432240312,1.,-2.4009556571164));
#55040=CARTESIAN_POINT('Ctrl Pts',(-2.9701964131236,-1.,-2.40438604734919));
#55041=CARTESIAN_POINT('Ctrl Pts',(-2.9701964131236,1.,-2.40438604734919));
#55042=CARTESIAN_POINT('Ctrl Pts',(-2.97646002822422,-1.,-2.40768975073713));
#55043=CARTESIAN_POINT('Ctrl Pts',(-2.97646002822422,1.,-2.40768975073713));
#55044=CARTESIAN_POINT('Ctrl Pts',(-2.98280015815107,-1.,-2.41095909342571));
#55045=CARTESIAN_POINT('Ctrl Pts',(-2.98280015815107,1.,-2.41095909342571));
#55046=CARTESIAN_POINT('Ctrl Pts',(-2.98927983005796,-1.,-2.41425064199586));
#55047=CARTESIAN_POINT('Ctrl Pts',(-2.98927983005796,1.,-2.41425064199586));
#55048=CARTESIAN_POINT('Ctrl Pts',(-2.99590509293503,-1.,-2.41757324500514));
#55049=CARTESIAN_POINT('Ctrl Pts',(-2.99590509293503,1.,-2.41757324500514));
#55050=CARTESIAN_POINT('Ctrl Pts',(-3.00264868585996,-1.,-2.42090763946779));
#55051=CARTESIAN_POINT('Ctrl Pts',(-3.00264868585996,1.,-2.42090763946779));
#55052=CARTESIAN_POINT('Ctrl Pts',(-3.00946442616658,-1.,-2.42421849439613));
#55053=CARTESIAN_POINT('Ctrl Pts',(-3.00946442616658,1.,-2.42421849439613));
#55054=CARTESIAN_POINT('Ctrl Pts',(-3.01630420830504,-1.,-2.42746856264168));
#55055=CARTESIAN_POINT('Ctrl Pts',(-3.01630420830504,1.,-2.42746856264168));
#55056=CARTESIAN_POINT('Ctrl Pts',(-3.02313656036004,-1.,-2.43063415586637));
#55057=CARTESIAN_POINT('Ctrl Pts',(-3.02313656036004,1.,-2.43063415586637));
#55058=CARTESIAN_POINT('Ctrl Pts',(-3.02995534946978,-1.,-2.43371241361488));
#55059=CARTESIAN_POINT('Ctrl Pts',(-3.02995534946978,1.,-2.43371241361488));
#55060=CARTESIAN_POINT('Ctrl Pts',(-3.03676949672821,-1.,-2.43671278042414));
#55061=CARTESIAN_POINT('Ctrl Pts',(-3.03676949672821,1.,-2.43671278042414));
#55062=CARTESIAN_POINT('Ctrl Pts',(-3.04359685040555,-1.,-2.43965194061857));
#55063=CARTESIAN_POINT('Ctrl Pts',(-3.04359685040555,1.,-2.43965194061857));
#55064=CARTESIAN_POINT('Ctrl Pts',(-3.05045678021504,-1.,-2.44254768923105));
#55065=CARTESIAN_POINT('Ctrl Pts',(-3.05045678021504,1.,-2.44254768923105));
#55066=CARTESIAN_POINT('Ctrl Pts',(-3.05736242671506,-1.,-2.44541251892556));
#55067=CARTESIAN_POINT('Ctrl Pts',(-3.05736242671506,1.,-2.44541251892556));
#55068=CARTESIAN_POINT('Ctrl Pts',(-3.06431596421405,-1.,-2.44824970516544));
#55069=CARTESIAN_POINT('Ctrl Pts',(-3.06431596421405,1.,-2.44824970516544));
#55070=CARTESIAN_POINT('Ctrl Pts',(-3.07131290521297,-1.,-2.45105688854422));
#55071=CARTESIAN_POINT('Ctrl Pts',(-3.07131290521297,1.,-2.45105688854422));
#55072=CARTESIAN_POINT('Ctrl Pts',(-3.07834472886139,-1.,-2.4538282678779));
#55073=CARTESIAN_POINT('Ctrl Pts',(-3.07834472886139,1.,-2.4538282678779));
#55074=CARTESIAN_POINT('Ctrl Pts',(-3.08540206545315,-1.,-2.45655725437039));
#55075=CARTESIAN_POINT('Ctrl Pts',(-3.08540206545315,1.,-2.45655725437039));
#55076=CARTESIAN_POINT('Ctrl Pts',(-3.09247787931887,-1.,-2.4592391256388));
#55077=CARTESIAN_POINT('Ctrl Pts',(-3.09247787931887,1.,-2.4592391256388));
#55078=CARTESIAN_POINT('Ctrl Pts',(-3.09956993697052,-1.,-2.46187308501884));
#55079=CARTESIAN_POINT('Ctrl Pts',(-3.09956993697052,1.,-2.46187308501884));
#55080=CARTESIAN_POINT('Ctrl Pts',(-3.1066790790198,-1.,-2.46446082979646));
#55081=CARTESIAN_POINT('Ctrl Pts',(-3.1066790790198,1.,-2.46446082979646));
#55082=CARTESIAN_POINT('Ctrl Pts',(-3.11380805536122,-1.,-2.46700558843506));
#55083=CARTESIAN_POINT('Ctrl Pts',(-3.11380805536122,1.,-2.46700558843506));
#55084=CARTESIAN_POINT('Ctrl Pts',(-3.12096015766983,-1.,-2.46951098947469));
#55085=CARTESIAN_POINT('Ctrl Pts',(-3.12096015766983,1.,-2.46951098947469));
#55086=CARTESIAN_POINT('Ctrl Pts',(-3.12813790805952,-1.,-2.47197997765871));
#55087=CARTESIAN_POINT('Ctrl Pts',(-3.12813790805952,1.,-2.47197997765871));
#55088=CARTESIAN_POINT('Ctrl Pts',(-3.13534181229295,-1.,-2.47441378371932));
#55089=CARTESIAN_POINT('Ctrl Pts',(-3.13534181229295,1.,-2.47441378371932));
#55090=CARTESIAN_POINT('Ctrl Pts',(-3.1425709954655,-1.,-2.47681245356109));
#55091=CARTESIAN_POINT('Ctrl Pts',(-3.1425709954655,1.,-2.47681245356109));
#55092=CARTESIAN_POINT('Ctrl Pts',(-3.14982373241352,-1.,-2.47917529057029));
#55093=CARTESIAN_POINT('Ctrl Pts',(-3.14982373241352,1.,-2.47917529057029));
#55094=CARTESIAN_POINT('Ctrl Pts',(-3.15709802322739,-1.,-2.48150133566571));
#55095=CARTESIAN_POINT('Ctrl Pts',(-3.15709802322739,1.,-2.48150133566571));
#55096=CARTESIAN_POINT('Ctrl Pts',(-3.16439213290161,-1.,-2.48378981792725));
#55097=CARTESIAN_POINT('Ctrl Pts',(-3.16439213290161,1.,-2.48378981792725));
#55098=CARTESIAN_POINT('Ctrl Pts',(-3.17170518863313,-1.,-2.48604065348587));
#55099=CARTESIAN_POINT('Ctrl Pts',(-3.17170518863313,1.,-2.48604065348587));
#55100=CARTESIAN_POINT('Ctrl Pts',(-3.17903698136622,-1.,-2.48825428288201));
#55101=CARTESIAN_POINT('Ctrl Pts',(-3.17903698136622,1.,-2.48825428288201));
#55102=CARTESIAN_POINT('Ctrl Pts',(-3.18638771282266,-1.,-2.49043146334059));
#55103=CARTESIAN_POINT('Ctrl Pts',(-3.18638771282266,1.,-2.49043146334059));
#55104=CARTESIAN_POINT('Ctrl Pts',(-3.19375775555798,-1.,-2.49257307239848));
#55105=CARTESIAN_POINT('Ctrl Pts',(-3.19375775555798,1.,-2.49257307239848));
#55106=CARTESIAN_POINT('Ctrl Pts',(-3.20114742397588,-1.,-2.49467992057755));
#55107=CARTESIAN_POINT('Ctrl Pts',(-3.20114742397588,1.,-2.49467992057755));
#55108=CARTESIAN_POINT('Ctrl Pts',(-3.20855669849836,-1.,-2.4967525264737));
#55109=CARTESIAN_POINT('Ctrl Pts',(-3.20855669849836,1.,-2.4967525264737));
#55110=CARTESIAN_POINT('Ctrl Pts',(-3.21598526261286,-1.,-2.4987911459939));
#55111=CARTESIAN_POINT('Ctrl Pts',(-3.21598526261286,1.,-2.4987911459939));
#55112=CARTESIAN_POINT('Ctrl Pts',(-3.22343262620503,-1.,-2.50079587201957));
#55113=CARTESIAN_POINT('Ctrl Pts',(-3.22343262620503,1.,-2.50079587201957));
#55114=CARTESIAN_POINT('Ctrl Pts',(-3.23089822320646,-1.,-2.50276671338111));
#55115=CARTESIAN_POINT('Ctrl Pts',(-3.23089822320646,1.,-2.50276671338111));
#55116=CARTESIAN_POINT('Ctrl Pts',(-3.23838151080319,-1.,-2.5047036758003));
#55117=CARTESIAN_POINT('Ctrl Pts',(-3.23838151080319,1.,-2.5047036758003));
#55118=CARTESIAN_POINT('Ctrl Pts',(-3.24588208983849,-1.,-2.506606859405));
#55119=CARTESIAN_POINT('Ctrl Pts',(-3.24588208983849,1.,-2.506606859405));
#55120=CARTESIAN_POINT('Ctrl Pts',(-3.25339971460982,-1.,-2.50847647070723));
#55121=CARTESIAN_POINT('Ctrl Pts',(-3.25339971460982,1.,-2.50847647070723));
#55122=CARTESIAN_POINT('Ctrl Pts',(-3.26093423001434,-1.,-2.51031277813486));
#55123=CARTESIAN_POINT('Ctrl Pts',(-3.26093423001434,1.,-2.51031277813486));
#55124=CARTESIAN_POINT('Ctrl Pts',(-3.26848552888115,-1.,-2.51211608411423));
#55125=CARTESIAN_POINT('Ctrl Pts',(-3.26848552888115,1.,-2.51211608411423));
#55126=CARTESIAN_POINT('Ctrl Pts',(-3.27605350473142,-1.,-2.513886692704));
#55127=CARTESIAN_POINT('Ctrl Pts',(-3.27605350473142,1.,-2.513886692704));
#55128=CARTESIAN_POINT('Ctrl Pts',(-3.28363799702982,-1.,-2.51562487464514));
#55129=CARTESIAN_POINT('Ctrl Pts',(-3.28363799702982,1.,-2.51562487464514));
#55130=CARTESIAN_POINT('Ctrl Pts',(-3.2912387729927,-1.,-2.51733085123797));
#55131=CARTESIAN_POINT('Ctrl Pts',(-3.2912387729927,1.,-2.51733085123797));
#55132=CARTESIAN_POINT('Ctrl Pts',(-3.29885556388352,-1.,-2.51900480701069));
#55133=CARTESIAN_POINT('Ctrl Pts',(-3.29885556388352,1.,-2.51900480701069));
#55134=CARTESIAN_POINT('Ctrl Pts',(-3.30648808815442,-1.,-2.52064689568511));
#55135=CARTESIAN_POINT('Ctrl Pts',(-3.30648808815442,1.,-2.52064689568511));
#55136=CARTESIAN_POINT('Ctrl Pts',(-3.31413607874645,-1.,-2.52225724871313));
#55137=CARTESIAN_POINT('Ctrl Pts',(-3.31413607874645,1.,-2.52225724871313));
#55138=CARTESIAN_POINT('Ctrl Pts',(-3.32179931078699,-1.,-2.5238359839626));
#55139=CARTESIAN_POINT('Ctrl Pts',(-3.32179931078699,1.,-2.5238359839626));
#55140=CARTESIAN_POINT('Ctrl Pts',(-3.32947762187533,-1.,-2.52538321164634));
#55141=CARTESIAN_POINT('Ctrl Pts',(-3.32947762187533,1.,-2.52538321164634));
#55142=CARTESIAN_POINT('Ctrl Pts',(-3.33717089999103,-1.,-2.52689902690158));
#55143=CARTESIAN_POINT('Ctrl Pts',(-3.33717089999103,1.,-2.52689902690158));
#55144=CARTESIAN_POINT('Ctrl Pts',(-3.34333744115511,-1.,-2.52808660915689));
#55145=CARTESIAN_POINT('Ctrl Pts',(-3.34333744115511,1.,-2.52808660915689));
#55146=CARTESIAN_POINT('Ctrl Pts',(-3.34796903576663,-1.,-2.52896321610703));
#55147=CARTESIAN_POINT('Ctrl Pts',(-3.34796903576663,1.,-2.52896321610703));
#55148=CARTESIAN_POINT('Ctrl Pts',(-3.35105973714071,-1.,-2.5295413654909));
#55149=CARTESIAN_POINT('Ctrl Pts',(-3.35105973714071,1.,-2.5295413654909));
#55150=CARTESIAN_POINT('Ctrl Pts',(-3.35260583073571,-1.,-2.52982887637028));
#55151=CARTESIAN_POINT('Ctrl Pts',(-3.35260583073571,1.,-2.52982887637028));
#55152=CARTESIAN_POINT('',(-2.90994629141676,1.,-2.36531447826073));
#55153=CARTESIAN_POINT('Ctrl Pts',(-2.90994629141676,-1.,-2.36531447826074));
#55154=CARTESIAN_POINT('Ctrl Pts',(-2.90994629141676,-0.666666666666667,
-2.36531447826074));
#55155=CARTESIAN_POINT('Ctrl Pts',(-2.90994629141676,-0.333333333333333,
-2.36531447826074));
#55156=CARTESIAN_POINT('Ctrl Pts',(-2.90994629141676,0.333333333333333,
-2.36531447826074));
#55157=CARTESIAN_POINT('Ctrl Pts',(-2.90994629141676,0.666666666666667,
-2.36531447826074));
#55158=CARTESIAN_POINT('Ctrl Pts',(-2.90994629141676,1.,-2.36531447826074));
#55159=CARTESIAN_POINT('',(-3.35260583073571,1.,-2.52982887637028));
#55160=CARTESIAN_POINT('',(-3.35260583073571,0.,-2.52982887637028));
#55161=CARTESIAN_POINT('Ctrl Pts',(-2.90994629141676,1.,-2.36531447826073));
#55162=CARTESIAN_POINT('Ctrl Pts',(-2.90995756655606,1.,-2.36536211188453));
#55163=CARTESIAN_POINT('Ctrl Pts',(-2.91005770527719,1.,-2.36553202948613));
#55164=CARTESIAN_POINT('Ctrl Pts',(-2.91051690822156,1.,-2.36599991765749));
#55165=CARTESIAN_POINT('Ctrl Pts',(-2.91181344022549,1.,-2.36707658451664));
#55166=CARTESIAN_POINT('Ctrl Pts',(-2.9146124988314,1.,-2.36919161373173));
#55167=CARTESIAN_POINT('Ctrl Pts',(-2.91891503791411,1.,-2.37229381109821));
#55168=CARTESIAN_POINT('Ctrl Pts',(-2.92430340582608,1.,-2.3760651052403));
#55169=CARTESIAN_POINT('Ctrl Pts',(-2.93049643640206,1.,-2.38028989582073));
#55170=CARTESIAN_POINT('Ctrl Pts',(-2.93717903280391,1.,-2.38472771516311));
#55171=CARTESIAN_POINT('Ctrl Pts',(-2.94404820669076,1.,-2.38914929090759));
#55172=CARTESIAN_POINT('Ctrl Pts',(-2.95085857128439,1.,-2.39337207631667));
#55173=CARTESIAN_POINT('Ctrl Pts',(-2.95748006482942,1.,-2.39730553974517));
#55174=CARTESIAN_POINT('Ctrl Pts',(-2.96390432240312,1.,-2.4009556571164));
#55175=CARTESIAN_POINT('Ctrl Pts',(-2.9701964131236,1.,-2.40438604734919));
#55176=CARTESIAN_POINT('Ctrl Pts',(-2.97646002822422,1.,-2.40768975073713));
#55177=CARTESIAN_POINT('Ctrl Pts',(-2.98280015815107,1.,-2.41095909342571));
#55178=CARTESIAN_POINT('Ctrl Pts',(-2.98927983005796,1.,-2.41425064199586));
#55179=CARTESIAN_POINT('Ctrl Pts',(-2.99590509293503,1.,-2.41757324500514));
#55180=CARTESIAN_POINT('Ctrl Pts',(-3.00264868585996,1.,-2.42090763946779));
#55181=CARTESIAN_POINT('Ctrl Pts',(-3.00946442616658,1.,-2.42421849439613));
#55182=CARTESIAN_POINT('Ctrl Pts',(-3.01630420830504,1.,-2.42746856264168));
#55183=CARTESIAN_POINT('Ctrl Pts',(-3.02313656036004,1.,-2.43063415586637));
#55184=CARTESIAN_POINT('Ctrl Pts',(-3.02995534946978,1.,-2.43371241361488));
#55185=CARTESIAN_POINT('Ctrl Pts',(-3.03676949672821,1.,-2.43671278042414));
#55186=CARTESIAN_POINT('Ctrl Pts',(-3.04359685040555,1.,-2.43965194061857));
#55187=CARTESIAN_POINT('Ctrl Pts',(-3.05045678021504,1.,-2.44254768923105));
#55188=CARTESIAN_POINT('Ctrl Pts',(-3.05736242671506,1.,-2.44541251892556));
#55189=CARTESIAN_POINT('Ctrl Pts',(-3.06431596421405,1.,-2.44824970516544));
#55190=CARTESIAN_POINT('Ctrl Pts',(-3.07131290521297,1.,-2.45105688854422));
#55191=CARTESIAN_POINT('Ctrl Pts',(-3.07834472886139,1.,-2.4538282678779));
#55192=CARTESIAN_POINT('Ctrl Pts',(-3.08540206545315,1.,-2.45655725437039));
#55193=CARTESIAN_POINT('Ctrl Pts',(-3.09247787931887,1.,-2.4592391256388));
#55194=CARTESIAN_POINT('Ctrl Pts',(-3.09956993697052,1.,-2.46187308501884));
#55195=CARTESIAN_POINT('Ctrl Pts',(-3.1066790790198,1.,-2.46446082979646));
#55196=CARTESIAN_POINT('Ctrl Pts',(-3.11380805536122,1.,-2.46700558843506));
#55197=CARTESIAN_POINT('Ctrl Pts',(-3.12096015766983,1.,-2.46951098947469));
#55198=CARTESIAN_POINT('Ctrl Pts',(-3.12813790805952,1.,-2.47197997765871));
#55199=CARTESIAN_POINT('Ctrl Pts',(-3.13534181229295,1.,-2.47441378371932));
#55200=CARTESIAN_POINT('Ctrl Pts',(-3.1425709954655,1.,-2.47681245356109));
#55201=CARTESIAN_POINT('Ctrl Pts',(-3.14982373241352,1.,-2.47917529057029));
#55202=CARTESIAN_POINT('Ctrl Pts',(-3.15709802322739,1.,-2.48150133566571));
#55203=CARTESIAN_POINT('Ctrl Pts',(-3.16439213290161,1.,-2.48378981792725));
#55204=CARTESIAN_POINT('Ctrl Pts',(-3.17170518863313,1.,-2.48604065348587));
#55205=CARTESIAN_POINT('Ctrl Pts',(-3.17903698136622,1.,-2.48825428288201));
#55206=CARTESIAN_POINT('Ctrl Pts',(-3.18638771282266,1.,-2.49043146334059));
#55207=CARTESIAN_POINT('Ctrl Pts',(-3.19375775555798,1.,-2.49257307239848));
#55208=CARTESIAN_POINT('Ctrl Pts',(-3.20114742397588,1.,-2.49467992057755));
#55209=CARTESIAN_POINT('Ctrl Pts',(-3.20855669849836,1.,-2.4967525264737));
#55210=CARTESIAN_POINT('Ctrl Pts',(-3.21598526261286,1.,-2.4987911459939));
#55211=CARTESIAN_POINT('Ctrl Pts',(-3.22343262620503,1.,-2.50079587201957));
#55212=CARTESIAN_POINT('Ctrl Pts',(-3.23089822320646,1.,-2.50276671338111));
#55213=CARTESIAN_POINT('Ctrl Pts',(-3.23838151080319,1.,-2.5047036758003));
#55214=CARTESIAN_POINT('Ctrl Pts',(-3.24588208983849,1.,-2.506606859405));
#55215=CARTESIAN_POINT('Ctrl Pts',(-3.25339971460982,1.,-2.50847647070723));
#55216=CARTESIAN_POINT('Ctrl Pts',(-3.26093423001434,1.,-2.51031277813486));
#55217=CARTESIAN_POINT('Ctrl Pts',(-3.26848552888115,1.,-2.51211608411423));
#55218=CARTESIAN_POINT('Ctrl Pts',(-3.27605350473142,1.,-2.513886692704));
#55219=CARTESIAN_POINT('Ctrl Pts',(-3.28363799702982,1.,-2.51562487464514));
#55220=CARTESIAN_POINT('Ctrl Pts',(-3.2912387729927,1.,-2.51733085123797));
#55221=CARTESIAN_POINT('Ctrl Pts',(-3.29885556388352,1.,-2.51900480701069));
#55222=CARTESIAN_POINT('Ctrl Pts',(-3.30648808815442,1.,-2.52064689568511));
#55223=CARTESIAN_POINT('Ctrl Pts',(-3.31413607874645,1.,-2.52225724871313));
#55224=CARTESIAN_POINT('Ctrl Pts',(-3.32179931078699,1.,-2.5238359839626));
#55225=CARTESIAN_POINT('Ctrl Pts',(-3.32947762187533,1.,-2.52538321164634));
#55226=CARTESIAN_POINT('Ctrl Pts',(-3.33717089999103,1.,-2.52689902690158));
#55227=CARTESIAN_POINT('Ctrl Pts',(-3.34333744115511,1.,-2.52808660915689));
#55228=CARTESIAN_POINT('Ctrl Pts',(-3.34796903576663,1.,-2.52896321610703));
#55229=CARTESIAN_POINT('Ctrl Pts',(-3.35105973714071,1.,-2.5295413654909));
#55230=CARTESIAN_POINT('Ctrl Pts',(-3.35260583073571,1.,-2.52982887637028));
#55231=CARTESIAN_POINT('Origin',(-3.35260583073571,0.,-2.52982887637028));
#55232=CARTESIAN_POINT('',(-3.44202241512147,1.,-2.40675750623143));
#55233=CARTESIAN_POINT('Origin',(0.,0.,0.));
#55234=CARTESIAN_POINT('',(-2.79140942341378,1.,-2.50410331873042));
#55235=CARTESIAN_POINT('Origin',(0.,1.,0.));
#55236=CARTESIAN_POINT('Ctrl Pts',(-2.79140942341378,1.,-2.50410331873042));
#55237=CARTESIAN_POINT('Ctrl Pts',(-2.79140942341378,0.666666666666667,
-2.50410331873042));
#55238=CARTESIAN_POINT('Ctrl Pts',(-2.79140942341378,0.333333333333333,
-2.50410331873042));
#55239=CARTESIAN_POINT('Ctrl Pts',(-2.79140942341378,-0.333333333333333,
-2.50410331873042));
#55240=CARTESIAN_POINT('Ctrl Pts',(-2.79140942341378,-0.666666666666667,
-2.50410331873042));
#55241=CARTESIAN_POINT('Ctrl Pts',(-2.79140942341378,-1.,-2.50410331873042));
#55242=CARTESIAN_POINT('Ctrl Pts',(-3.02314558451372,-1.,-2.91557726271063));
#55243=CARTESIAN_POINT('Ctrl Pts',(-3.02314558451372,1.,-2.91557726271063));
#55244=CARTESIAN_POINT('Ctrl Pts',(-3.02261975104912,-1.,-2.91409518070707));
#55245=CARTESIAN_POINT('Ctrl Pts',(-3.02261975104912,1.,-2.91409518070707));
#55246=CARTESIAN_POINT('Ctrl Pts',(-3.02156522743299,-1.,-2.91113297349052));
#55247=CARTESIAN_POINT('Ctrl Pts',(-3.02156522743299,1.,-2.91113297349052));
#55248=CARTESIAN_POINT('Ctrl Pts',(-3.01997487194926,-1.,-2.90669553303902));
#55249=CARTESIAN_POINT('Ctrl Pts',(-3.01997487194926,1.,-2.90669553303902));
#55250=CARTESIAN_POINT('Ctrl Pts',(-3.01783725123646,-1.,-2.90079069102661));
#55251=CARTESIAN_POINT('Ctrl Pts',(-3.01783725123646,1.,-2.90079069102661));
#55252=CARTESIAN_POINT('Ctrl Pts',(-3.01513660433291,-1.,-2.8934292556764));
#55253=CARTESIAN_POINT('Ctrl Pts',(-3.01513660433291,1.,-2.8934292556764));
#55254=CARTESIAN_POINT('Ctrl Pts',(-3.01240727309568,-1.,-2.88608751706796));
#55255=CARTESIAN_POINT('Ctrl Pts',(-3.01240727309568,1.,-2.88608751706796));
#55256=CARTESIAN_POINT('Ctrl Pts',(-3.0096491810855,-1.,-2.87876560072799));
#55257=CARTESIAN_POINT('Ctrl Pts',(-3.0096491810855,1.,-2.87876560072799));
#55258=CARTESIAN_POINT('Ctrl Pts',(-3.00686224485374,-1.,-2.87146368430104));
#55259=CARTESIAN_POINT('Ctrl Pts',(-3.00686224485374,1.,-2.87146368430104));
#55260=CARTESIAN_POINT('Ctrl Pts',(-3.00404638316245,-1.,-2.86418200833065));
#55261=CARTESIAN_POINT('Ctrl Pts',(-3.00404638316245,1.,-2.86418200833065));
#55262=CARTESIAN_POINT('Ctrl Pts',(-3.0012015079552,-1.,-2.85692085715129));
#55263=CARTESIAN_POINT('Ctrl Pts',(-3.0012015079552,1.,-2.85692085715129));
#55264=CARTESIAN_POINT('Ctrl Pts',(-2.99832751144566,-1.,-2.84968053289104));
#55265=CARTESIAN_POINT('Ctrl Pts',(-2.99832751144566,1.,-2.84968053289104));
#55266=CARTESIAN_POINT('Ctrl Pts',(-2.995424253416,-1.,-2.84246132984334));
#55267=CARTESIAN_POINT('Ctrl Pts',(-2.995424253416,1.,-2.84246132984334));
#55268=CARTESIAN_POINT('Ctrl Pts',(-2.99249155170479,-1.,-2.83526351254383));
#55269=CARTESIAN_POINT('Ctrl Pts',(-2.99249155170479,1.,-2.83526351254383));
#55270=CARTESIAN_POINT('Ctrl Pts',(-2.98952916401699,-1.,-2.82808728190402));
#55271=CARTESIAN_POINT('Ctrl Pts',(-2.98952916401699,1.,-2.82808728190402));
#55272=CARTESIAN_POINT('Ctrl Pts',(-2.98653680669434,-1.,-2.82093279065704));
#55273=CARTESIAN_POINT('Ctrl Pts',(-2.98653680669434,1.,-2.82093279065704));
#55274=CARTESIAN_POINT('Ctrl Pts',(-2.9835141977994,-1.,-2.81380019196454));
#55275=CARTESIAN_POINT('Ctrl Pts',(-2.9835141977994,1.,-2.81380019196454));
#55276=CARTESIAN_POINT('Ctrl Pts',(-2.98046109647299,-1.,-2.80668968101162));
#55277=CARTESIAN_POINT('Ctrl Pts',(-2.98046109647299,1.,-2.80668968101162));
#55278=CARTESIAN_POINT('Ctrl Pts',(-2.97737733718242,-1.,-2.79960153278186));
#55279=CARTESIAN_POINT('Ctrl Pts',(-2.97737733718242,1.,-2.79960153278186));
#55280=CARTESIAN_POINT('Ctrl Pts',(-2.97426288347475,-1.,-2.79253615718147));
#55281=CARTESIAN_POINT('Ctrl Pts',(-2.97426288347475,1.,-2.79253615718147));
#55282=CARTESIAN_POINT('Ctrl Pts',(-2.97111781461349,-1.,-2.78549409123657));
#55283=CARTESIAN_POINT('Ctrl Pts',(-2.97111781461349,1.,-2.78549409123657));
#55284=CARTESIAN_POINT('Ctrl Pts',(-2.9679422104295,-1.,-2.77847589542767));
#55285=CARTESIAN_POINT('Ctrl Pts',(-2.9679422104295,1.,-2.77847589542767));
#55286=CARTESIAN_POINT('Ctrl Pts',(-2.96473605585548,-1.,-2.77148206836464));
#55287=CARTESIAN_POINT('Ctrl Pts',(-2.96473605585548,1.,-2.77148206836464));
#55288=CARTESIAN_POINT('Ctrl Pts',(-2.96149914764832,-1.,-2.76451296269571));
#55289=CARTESIAN_POINT('Ctrl Pts',(-2.96149914764832,1.,-2.76451296269571));
#55290=CARTESIAN_POINT('Ctrl Pts',(-2.9582309766594,-1.,-2.75756867888393));
#55291=CARTESIAN_POINT('Ctrl Pts',(-2.9582309766594,1.,-2.75756867888393));
#55292=CARTESIAN_POINT('Ctrl Pts',(-2.95493069316211,-1.,-2.75064903318996));
#55293=CARTESIAN_POINT('Ctrl Pts',(-2.95493069316211,1.,-2.75064903318996));
#55294=CARTESIAN_POINT('Ctrl Pts',(-2.95159737214305,-1.,-2.7437537949221));
#55295=CARTESIAN_POINT('Ctrl Pts',(-2.95159737214305,1.,-2.7437537949221));
#55296=CARTESIAN_POINT('Ctrl Pts',(-2.94823023414381,-1.,-2.73688288329825));
#55297=CARTESIAN_POINT('Ctrl Pts',(-2.94823023414381,1.,-2.73688288329825));
#55298=CARTESIAN_POINT('Ctrl Pts',(-2.94482887675139,-1.,-2.73003657371613));
#55299=CARTESIAN_POINT('Ctrl Pts',(-2.94482887675139,1.,-2.73003657371613));
#55300=CARTESIAN_POINT('Ctrl Pts',(-2.94139351933882,-1.,-2.72321571511322));
#55301=CARTESIAN_POINT('Ctrl Pts',(-2.94139351933882,1.,-2.72321571511322));
#55302=CARTESIAN_POINT('Ctrl Pts',(-2.93792519474955,-1.,-2.71642190053575));
#55303=CARTESIAN_POINT('Ctrl Pts',(-2.93792519474955,1.,-2.71642190053575));
#55304=CARTESIAN_POINT('Ctrl Pts',(-2.93442516311168,-1.,-2.70965695523776));
#55305=CARTESIAN_POINT('Ctrl Pts',(-2.93442516311168,1.,-2.70965695523776));
#55306=CARTESIAN_POINT('Ctrl Pts',(-2.93089438233746,-1.,-2.70292247416881));
#55307=CARTESIAN_POINT('Ctrl Pts',(-2.93089438233746,1.,-2.70292247416881));
#55308=CARTESIAN_POINT('Ctrl Pts',(-2.92733294395268,-1.,-2.69621932864302));
#55309=CARTESIAN_POINT('Ctrl Pts',(-2.92733294395268,1.,-2.69621932864302));
#55310=CARTESIAN_POINT('Ctrl Pts',(-2.92373955325876,-1.,-2.68954721165342));
#55311=CARTESIAN_POINT('Ctrl Pts',(-2.92373955325876,1.,-2.68954721165342));
#55312=CARTESIAN_POINT('Ctrl Pts',(-2.92011090722152,-1.,-2.68290409279689));
#55313=CARTESIAN_POINT('Ctrl Pts',(-2.92011090722152,1.,-2.68290409279689));
#55314=CARTESIAN_POINT('Ctrl Pts',(-2.91644290704281,-1.,-2.67628728855309));
#55315=CARTESIAN_POINT('Ctrl Pts',(-2.91644290704281,1.,-2.67628728855309));
#55316=CARTESIAN_POINT('Ctrl Pts',(-2.91273193382876,-1.,-2.66969458792627));
#55317=CARTESIAN_POINT('Ctrl Pts',(-2.91273193382876,1.,-2.66969458792627));
#55318=CARTESIAN_POINT('Ctrl Pts',(-2.90897617968921,-1.,-2.66312542616808));
#55319=CARTESIAN_POINT('Ctrl Pts',(-2.90897617968921,1.,-2.66312542616808));
#55320=CARTESIAN_POINT('Ctrl Pts',(-2.90517678087467,-1.,-2.65658188464287));
#55321=CARTESIAN_POINT('Ctrl Pts',(-2.90517678087467,1.,-2.65658188464287));
#55322=CARTESIAN_POINT('Ctrl Pts',(-2.90133950224879,-1.,-2.65007017365576));
#55323=CARTESIAN_POINT('Ctrl Pts',(-2.90133950224879,1.,-2.65007017365576));
#55324=CARTESIAN_POINT('Ctrl Pts',(-2.89747231723361,-1.,-2.64359851684146));
#55325=CARTESIAN_POINT('Ctrl Pts',(-2.89747231723361,1.,-2.64359851684146));
#55326=CARTESIAN_POINT('Ctrl Pts',(-2.89358228854557,-1.,-2.63717442263944));
#55327=CARTESIAN_POINT('Ctrl Pts',(-2.89358228854557,1.,-2.63717442263944));
#55328=CARTESIAN_POINT('Ctrl Pts',(-2.88967244854243,-1.,-2.63080195420771));
#55329=CARTESIAN_POINT('Ctrl Pts',(-2.88967244854243,1.,-2.63080195420771));
#55330=CARTESIAN_POINT('Ctrl Pts',(-2.88573922195049,-1.,-2.62447947640253));
#55331=CARTESIAN_POINT('Ctrl Pts',(-2.88573922195049,1.,-2.62447947640253));
#55332=CARTESIAN_POINT('Ctrl Pts',(-2.88176821427502,-1.,-2.61819596473087));
#55333=CARTESIAN_POINT('Ctrl Pts',(-2.88176821427502,1.,-2.61819596473087));
#55334=CARTESIAN_POINT('Ctrl Pts',(-2.87773881947885,-1.,-2.61193507170928));
#55335=CARTESIAN_POINT('Ctrl Pts',(-2.87773881947885,1.,-2.61193507170928));
#55336=CARTESIAN_POINT('Ctrl Pts',(-2.87363176656475,-1.,-2.6056817788128));
#55337=CARTESIAN_POINT('Ctrl Pts',(-2.87363176656475,1.,-2.6056817788128));
#55338=CARTESIAN_POINT('Ctrl Pts',(-2.86943633170712,-1.,-2.59942875223202));
#55339=CARTESIAN_POINT('Ctrl Pts',(-2.86943633170712,1.,-2.59942875223202));
#55340=CARTESIAN_POINT('Ctrl Pts',(-2.86515629953528,-1.,-2.59318160184921));
#55341=CARTESIAN_POINT('Ctrl Pts',(-2.86515629953528,1.,-2.59318160184921));
#55342=CARTESIAN_POINT('Ctrl Pts',(-2.86081999003668,-1.,-2.5869677064356));
#55343=CARTESIAN_POINT('Ctrl Pts',(-2.86081999003668,1.,-2.5869677064356));
#55344=CARTESIAN_POINT('Ctrl Pts',(-2.85647171715147,-1.,-2.58082875254407));
#55345=CARTESIAN_POINT('Ctrl Pts',(-2.85647171715147,1.,-2.58082875254407));
#55346=CARTESIAN_POINT('Ctrl Pts',(-2.85215360144483,-1.,-2.57480482727128));
#55347=CARTESIAN_POINT('Ctrl Pts',(-2.85215360144483,1.,-2.57480482727128));
#55348=CARTESIAN_POINT('Ctrl Pts',(-2.84788893329091,-1.,-2.56891984251743));
#55349=CARTESIAN_POINT('Ctrl Pts',(-2.84788893329091,1.,-2.56891984251743));
#55350=CARTESIAN_POINT('Ctrl Pts',(-2.84366802680211,-1.,-2.56316920798489));
#55351=CARTESIAN_POINT('Ctrl Pts',(-2.84366802680211,1.,-2.56316920798489));
#55352=CARTESIAN_POINT('Ctrl Pts',(-2.83942515220699,-1.,-2.55749952145165));
#55353=CARTESIAN_POINT('Ctrl Pts',(-2.83942515220699,1.,-2.55749952145165));
#55354=CARTESIAN_POINT('Ctrl Pts',(-2.83505269592412,-1.,-2.55182152806964));
#55355=CARTESIAN_POINT('Ctrl Pts',(-2.83505269592412,1.,-2.55182152806964));
#55356=CARTESIAN_POINT('Ctrl Pts',(-2.83044254225794,-1.,-2.54604736792542));
#55357=CARTESIAN_POINT('Ctrl Pts',(-2.83044254225794,1.,-2.54604736792542));
#55358=CARTESIAN_POINT('Ctrl Pts',(-2.82552167649157,-1.,-2.54012272520141));
#55359=CARTESIAN_POINT('Ctrl Pts',(-2.82552167649157,1.,-2.54012272520141));
#55360=CARTESIAN_POINT('Ctrl Pts',(-2.82028550483744,-1.,-2.53405679667463));
#55361=CARTESIAN_POINT('Ctrl Pts',(-2.82028550483744,1.,-2.53405679667463));
#55362=CARTESIAN_POINT('Ctrl Pts',(-2.8148437904867,-1.,-2.52796388055457));
#55363=CARTESIAN_POINT('Ctrl Pts',(-2.8148437904867,1.,-2.52796388055457));
#55364=CARTESIAN_POINT('Ctrl Pts',(-2.80941521967234,-1.,-2.52205778589922));
#55365=CARTESIAN_POINT('Ctrl Pts',(-2.80941521967234,1.,-2.52205778589922));
#55366=CARTESIAN_POINT('Ctrl Pts',(-2.80427363984939,-1.,-2.51660190466067));
#55367=CARTESIAN_POINT('Ctrl Pts',(-2.80427363984939,1.,-2.51660190466067));
#55368=CARTESIAN_POINT('Ctrl Pts',(-2.79970585014308,-1.,-2.51186983687947));
#55369=CARTESIAN_POINT('Ctrl Pts',(-2.79970585014308,1.,-2.51186983687947));
#55370=CARTESIAN_POINT('Ctrl Pts',(-2.7959687805717,-1.,-2.50810555977564));
#55371=CARTESIAN_POINT('Ctrl Pts',(-2.7959687805717,1.,-2.50810555977564));
#55372=CARTESIAN_POINT('Ctrl Pts',(-2.79323694088143,-1.,-2.50547439929077));
#55373=CARTESIAN_POINT('Ctrl Pts',(-2.79323694088143,1.,-2.50547439929077));
#55374=CARTESIAN_POINT('Ctrl Pts',(-2.79192122906739,-1.,-2.50433799076945));
#55375=CARTESIAN_POINT('Ctrl Pts',(-2.79192122906739,1.,-2.50433799076945));
#55376=CARTESIAN_POINT('Ctrl Pts',(-2.79143626022225,-1.,-2.50404230339032));
#55377=CARTESIAN_POINT('Ctrl Pts',(-2.79143626022225,1.,-2.50404230339032));
#55378=CARTESIAN_POINT('Ctrl Pts',(-2.79133581100044,-1.,-2.50409239460011));
#55379=CARTESIAN_POINT('Ctrl Pts',(-2.79133581100044,1.,-2.50409239460011));
#55380=CARTESIAN_POINT('Ctrl Pts',(-2.79134130681569,-1.,-2.50417924854921));
#55381=CARTESIAN_POINT('Ctrl Pts',(-2.79134130681569,1.,-2.50417924854921));
#55382=CARTESIAN_POINT('',(-3.02314558451372,1.,-2.91557726271063));
#55383=CARTESIAN_POINT('Ctrl Pts',(-3.02314558451372,1.,-2.91557726271063));
#55384=CARTESIAN_POINT('Ctrl Pts',(-3.02261975104912,1.,-2.91409518070707));
#55385=CARTESIAN_POINT('Ctrl Pts',(-3.02156522743299,1.,-2.91113297349052));
#55386=CARTESIAN_POINT('Ctrl Pts',(-3.01997487194926,1.,-2.90669553303902));
#55387=CARTESIAN_POINT('Ctrl Pts',(-3.01783725123646,1.,-2.90079069102661));
#55388=CARTESIAN_POINT('Ctrl Pts',(-3.01513660433291,1.,-2.8934292556764));
#55389=CARTESIAN_POINT('Ctrl Pts',(-3.01240727309568,1.,-2.88608751706796));
#55390=CARTESIAN_POINT('Ctrl Pts',(-3.0096491810855,1.,-2.87876560072799));
#55391=CARTESIAN_POINT('Ctrl Pts',(-3.00686224485374,1.,-2.87146368430104));
#55392=CARTESIAN_POINT('Ctrl Pts',(-3.00404638316245,1.,-2.86418200833065));
#55393=CARTESIAN_POINT('Ctrl Pts',(-3.0012015079552,1.,-2.85692085715129));
#55394=CARTESIAN_POINT('Ctrl Pts',(-2.99832751144566,1.,-2.84968053289104));
#55395=CARTESIAN_POINT('Ctrl Pts',(-2.995424253416,1.,-2.84246132984334));
#55396=CARTESIAN_POINT('Ctrl Pts',(-2.99249155170479,1.,-2.83526351254383));
#55397=CARTESIAN_POINT('Ctrl Pts',(-2.98952916401699,1.,-2.82808728190402));
#55398=CARTESIAN_POINT('Ctrl Pts',(-2.98653680669434,1.,-2.82093279065704));
#55399=CARTESIAN_POINT('Ctrl Pts',(-2.9835141977994,1.,-2.81380019196454));
#55400=CARTESIAN_POINT('Ctrl Pts',(-2.98046109647299,1.,-2.80668968101162));
#55401=CARTESIAN_POINT('Ctrl Pts',(-2.97737733718242,1.,-2.79960153278186));
#55402=CARTESIAN_POINT('Ctrl Pts',(-2.97426288347475,1.,-2.79253615718147));
#55403=CARTESIAN_POINT('Ctrl Pts',(-2.97111781461349,1.,-2.78549409123657));
#55404=CARTESIAN_POINT('Ctrl Pts',(-2.9679422104295,1.,-2.77847589542767));
#55405=CARTESIAN_POINT('Ctrl Pts',(-2.96473605585548,1.,-2.77148206836464));
#55406=CARTESIAN_POINT('Ctrl Pts',(-2.96149914764832,1.,-2.76451296269571));
#55407=CARTESIAN_POINT('Ctrl Pts',(-2.9582309766594,1.,-2.75756867888393));
#55408=CARTESIAN_POINT('Ctrl Pts',(-2.95493069316211,1.,-2.75064903318996));
#55409=CARTESIAN_POINT('Ctrl Pts',(-2.95159737214305,1.,-2.7437537949221));
#55410=CARTESIAN_POINT('Ctrl Pts',(-2.94823023414381,1.,-2.73688288329825));
#55411=CARTESIAN_POINT('Ctrl Pts',(-2.94482887675139,1.,-2.73003657371613));
#55412=CARTESIAN_POINT('Ctrl Pts',(-2.94139351933882,1.,-2.72321571511322));
#55413=CARTESIAN_POINT('Ctrl Pts',(-2.93792519474955,1.,-2.71642190053575));
#55414=CARTESIAN_POINT('Ctrl Pts',(-2.93442516311168,1.,-2.70965695523776));
#55415=CARTESIAN_POINT('Ctrl Pts',(-2.93089438233746,1.,-2.70292247416881));
#55416=CARTESIAN_POINT('Ctrl Pts',(-2.92733294395268,1.,-2.69621932864302));
#55417=CARTESIAN_POINT('Ctrl Pts',(-2.92373955325876,1.,-2.68954721165342));
#55418=CARTESIAN_POINT('Ctrl Pts',(-2.92011090722152,1.,-2.68290409279689));
#55419=CARTESIAN_POINT('Ctrl Pts',(-2.91644290704281,1.,-2.67628728855309));
#55420=CARTESIAN_POINT('Ctrl Pts',(-2.91273193382876,1.,-2.66969458792627));
#55421=CARTESIAN_POINT('Ctrl Pts',(-2.90897617968921,1.,-2.66312542616808));
#55422=CARTESIAN_POINT('Ctrl Pts',(-2.90517678087467,1.,-2.65658188464287));
#55423=CARTESIAN_POINT('Ctrl Pts',(-2.90133950224879,1.,-2.65007017365576));
#55424=CARTESIAN_POINT('Ctrl Pts',(-2.89747231723361,1.,-2.64359851684146));
#55425=CARTESIAN_POINT('Ctrl Pts',(-2.89358228854557,1.,-2.63717442263944));
#55426=CARTESIAN_POINT('Ctrl Pts',(-2.88967244854243,1.,-2.63080195420771));
#55427=CARTESIAN_POINT('Ctrl Pts',(-2.88573922195049,1.,-2.62447947640253));
#55428=CARTESIAN_POINT('Ctrl Pts',(-2.88176821427502,1.,-2.61819596473087));
#55429=CARTESIAN_POINT('Ctrl Pts',(-2.87773881947885,1.,-2.61193507170928));
#55430=CARTESIAN_POINT('Ctrl Pts',(-2.87363176656475,1.,-2.6056817788128));
#55431=CARTESIAN_POINT('Ctrl Pts',(-2.86943633170712,1.,-2.59942875223202));
#55432=CARTESIAN_POINT('Ctrl Pts',(-2.86515629953528,1.,-2.59318160184921));
#55433=CARTESIAN_POINT('Ctrl Pts',(-2.86081999003668,1.,-2.5869677064356));
#55434=CARTESIAN_POINT('Ctrl Pts',(-2.85647171715147,1.,-2.58082875254407));
#55435=CARTESIAN_POINT('Ctrl Pts',(-2.85215360144483,1.,-2.57480482727128));
#55436=CARTESIAN_POINT('Ctrl Pts',(-2.84788893329091,1.,-2.56891984251743));
#55437=CARTESIAN_POINT('Ctrl Pts',(-2.84366802680211,1.,-2.56316920798489));
#55438=CARTESIAN_POINT('Ctrl Pts',(-2.83942515220699,1.,-2.55749952145165));
#55439=CARTESIAN_POINT('Ctrl Pts',(-2.83505269592412,1.,-2.55182152806964));
#55440=CARTESIAN_POINT('Ctrl Pts',(-2.83044254225794,1.,-2.54604736792542));
#55441=CARTESIAN_POINT('Ctrl Pts',(-2.82552167649157,1.,-2.54012272520141));
#55442=CARTESIAN_POINT('Ctrl Pts',(-2.82028550483744,1.,-2.53405679667463));
#55443=CARTESIAN_POINT('Ctrl Pts',(-2.8148437904867,1.,-2.52796388055457));
#55444=CARTESIAN_POINT('Ctrl Pts',(-2.80941521967234,1.,-2.52205778589922));
#55445=CARTESIAN_POINT('Ctrl Pts',(-2.80427363984939,1.,-2.51660190466067));
#55446=CARTESIAN_POINT('Ctrl Pts',(-2.79970585014308,1.,-2.51186983687947));
#55447=CARTESIAN_POINT('Ctrl Pts',(-2.7959687805717,1.,-2.50810555977564));
#55448=CARTESIAN_POINT('Ctrl Pts',(-2.79344192164204,1.,-2.50567182569153));
#55449=CARTESIAN_POINT('Ctrl Pts',(-2.79217568804874,1.,-2.50455968395235));
#55450=CARTESIAN_POINT('Ctrl Pts',(-2.79164172519039,1.,-2.50417932839344));
#55451=CARTESIAN_POINT('Ctrl Pts',(-2.79145823440899,1.,-2.50410700351427));
#55452=CARTESIAN_POINT('Ctrl Pts',(-2.79140942341378,1.,-2.50410331873043));
#55453=CARTESIAN_POINT('',(-3.02314558451372,0.,-2.91557726271063));
#55454=CARTESIAN_POINT('Ctrl Pts',(-2.50417924854921,-1.,-2.79134130681569));
#55455=CARTESIAN_POINT('Ctrl Pts',(-2.50417924854921,1.,-2.79134130681569));
#55456=CARTESIAN_POINT('Ctrl Pts',(-2.50409239460108,-1.,-2.7913358110015));
#55457=CARTESIAN_POINT('Ctrl Pts',(-2.50409239460108,1.,-2.7913358110015));
#55458=CARTESIAN_POINT('Ctrl Pts',(-2.50404230339286,-1.,-2.79143626022503));
#55459=CARTESIAN_POINT('Ctrl Pts',(-2.50404230339286,1.,-2.79143626022503));
#55460=CARTESIAN_POINT('Ctrl Pts',(-2.5043379907732,-1.,-2.79192122907148));
#55461=CARTESIAN_POINT('Ctrl Pts',(-2.5043379907732,1.,-2.79192122907148));
#55462=CARTESIAN_POINT('Ctrl Pts',(-2.50547439929414,-1.,-2.7932369408851));
#55463=CARTESIAN_POINT('Ctrl Pts',(-2.50547439929414,1.,-2.7932369408851));
#55464=CARTESIAN_POINT('Ctrl Pts',(-2.50810555977671,-1.,-2.79596878057287));
#55465=CARTESIAN_POINT('Ctrl Pts',(-2.50810555977671,1.,-2.79596878057287));
#55466=CARTESIAN_POINT('Ctrl Pts',(-2.51186983687818,-1.,-2.79970585014168));
#55467=CARTESIAN_POINT('Ctrl Pts',(-2.51186983687818,1.,-2.79970585014168));
#55468=CARTESIAN_POINT('Ctrl Pts',(-2.51660190465805,-1.,-2.80427363984653));
#55469=CARTESIAN_POINT('Ctrl Pts',(-2.51660190465805,1.,-2.80427363984653));
#55470=CARTESIAN_POINT('Ctrl Pts',(-2.52205778589653,-1.,-2.80941521966941));
#55471=CARTESIAN_POINT('Ctrl Pts',(-2.52205778589653,1.,-2.80941521966941));
#55472=CARTESIAN_POINT('Ctrl Pts',(-2.52796388055278,-1.,-2.81484379048475));
#55473=CARTESIAN_POINT('Ctrl Pts',(-2.52796388055278,1.,-2.81484379048475));
#55474=CARTESIAN_POINT('Ctrl Pts',(-2.53405679667412,-1.,-2.82028550483689));
#55475=CARTESIAN_POINT('Ctrl Pts',(-2.53405679667412,1.,-2.82028550483689));
#55476=CARTESIAN_POINT('Ctrl Pts',(-2.54012272520199,-1.,-2.8255216764922));
#55477=CARTESIAN_POINT('Ctrl Pts',(-2.54012272520199,1.,-2.8255216764922));
#55478=CARTESIAN_POINT('Ctrl Pts',(-2.54604736792655,-1.,-2.83044254225917));
#55479=CARTESIAN_POINT('Ctrl Pts',(-2.54604736792655,1.,-2.83044254225917));
#55480=CARTESIAN_POINT('Ctrl Pts',(-2.55182152807077,-1.,-2.83505269592536));
#55481=CARTESIAN_POINT('Ctrl Pts',(-2.55182152807077,1.,-2.83505269592536));
#55482=CARTESIAN_POINT('Ctrl Pts',(-2.55749952145241,-1.,-2.83942515220782));
#55483=CARTESIAN_POINT('Ctrl Pts',(-2.55749952145241,1.,-2.83942515220782));
#55484=CARTESIAN_POINT('Ctrl Pts',(-2.56316920798513,-1.,-2.84366802680237));
#55485=CARTESIAN_POINT('Ctrl Pts',(-2.56316920798513,1.,-2.84366802680237));
#55486=CARTESIAN_POINT('Ctrl Pts',(-2.56891984251721,-1.,-2.84788893329067));
#55487=CARTESIAN_POINT('Ctrl Pts',(-2.56891984251721,1.,-2.84788893329067));
#55488=CARTESIAN_POINT('Ctrl Pts',(-2.57480482727081,-1.,-2.85215360144431));
#55489=CARTESIAN_POINT('Ctrl Pts',(-2.57480482727081,1.,-2.85215360144431));
#55490=CARTESIAN_POINT('Ctrl Pts',(-2.58082875254357,-1.,-2.85647171715092));
#55491=CARTESIAN_POINT('Ctrl Pts',(-2.58082875254357,1.,-2.85647171715092));
#55492=CARTESIAN_POINT('Ctrl Pts',(-2.58696770643524,-1.,-2.86081999003629));
#55493=CARTESIAN_POINT('Ctrl Pts',(-2.58696770643524,1.,-2.86081999003629));
#55494=CARTESIAN_POINT('Ctrl Pts',(-2.59318160184908,-1.,-2.86515629953513));
#55495=CARTESIAN_POINT('Ctrl Pts',(-2.59318160184908,1.,-2.86515629953513));
#55496=CARTESIAN_POINT('Ctrl Pts',(-2.5994287522321,-1.,-2.86943633170722));
#55497=CARTESIAN_POINT('Ctrl Pts',(-2.5994287522321,1.,-2.86943633170722));
#55498=CARTESIAN_POINT('Ctrl Pts',(-2.60568177881303,-1.,-2.87363176656501));
#55499=CARTESIAN_POINT('Ctrl Pts',(-2.60568177881303,1.,-2.87363176656501));
#55500=CARTESIAN_POINT('Ctrl Pts',(-2.61193507170955,-1.,-2.87773881947915));
#55501=CARTESIAN_POINT('Ctrl Pts',(-2.61193507170955,1.,-2.87773881947915));
#55502=CARTESIAN_POINT('Ctrl Pts',(-2.61819596473108,-1.,-2.88176821427525));
#55503=CARTESIAN_POINT('Ctrl Pts',(-2.61819596473108,1.,-2.88176821427525));
#55504=CARTESIAN_POINT('Ctrl Pts',(-2.62447947640262,-1.,-2.88573922195059));
#55505=CARTESIAN_POINT('Ctrl Pts',(-2.62447947640262,1.,-2.88573922195059));
#55506=CARTESIAN_POINT('Ctrl Pts',(-2.63080195420767,-1.,-2.88967244854239));
#55507=CARTESIAN_POINT('Ctrl Pts',(-2.63080195420767,1.,-2.88967244854239));
#55508=CARTESIAN_POINT('Ctrl Pts',(-2.63717442263932,-1.,-2.89358228854544));
#55509=CARTESIAN_POINT('Ctrl Pts',(-2.63717442263932,1.,-2.89358228854544));
#55510=CARTESIAN_POINT('Ctrl Pts',(-2.64359851684131,-1.,-2.89747231723345));
#55511=CARTESIAN_POINT('Ctrl Pts',(-2.64359851684131,1.,-2.89747231723345));
#55512=CARTESIAN_POINT('Ctrl Pts',(-2.65007017365564,-1.,-2.90133950224867));
#55513=CARTESIAN_POINT('Ctrl Pts',(-2.65007017365564,1.,-2.90133950224867));
#55514=CARTESIAN_POINT('Ctrl Pts',(-2.65658188464282,-1.,-2.90517678087461));
#55515=CARTESIAN_POINT('Ctrl Pts',(-2.65658188464282,1.,-2.90517678087461));
#55516=CARTESIAN_POINT('Ctrl Pts',(-2.6631254261681,-1.,-2.90897617968923));
#55517=CARTESIAN_POINT('Ctrl Pts',(-2.6631254261681,1.,-2.90897617968923));
#55518=CARTESIAN_POINT('Ctrl Pts',(-2.66969458792631,-1.,-2.91273193382882));
#55519=CARTESIAN_POINT('Ctrl Pts',(-2.66969458792631,1.,-2.91273193382882));
#55520=CARTESIAN_POINT('Ctrl Pts',(-2.67628728855312,-1.,-2.91644290704285));
#55521=CARTESIAN_POINT('Ctrl Pts',(-2.67628728855312,1.,-2.91644290704285));
#55522=CARTESIAN_POINT('Ctrl Pts',(-2.68290409279688,-1.,-2.92011090722152));
#55523=CARTESIAN_POINT('Ctrl Pts',(-2.68290409279688,1.,-2.92011090722152));
#55524=CARTESIAN_POINT('Ctrl Pts',(-2.68954721165339,-1.,-2.92373955325875));
#55525=CARTESIAN_POINT('Ctrl Pts',(-2.68954721165339,1.,-2.92373955325875));
#55526=CARTESIAN_POINT('Ctrl Pts',(-2.69621932864301,-1.,-2.92733294395267));
#55527=CARTESIAN_POINT('Ctrl Pts',(-2.69621932864301,1.,-2.92733294395267));
#55528=CARTESIAN_POINT('Ctrl Pts',(-2.70292247416885,-1.,-2.93089438233749));
#55529=CARTESIAN_POINT('Ctrl Pts',(-2.70292247416885,1.,-2.93089438233749));
#55530=CARTESIAN_POINT('Ctrl Pts',(-2.70965695523787,-1.,-2.93442516311179));
#55531=CARTESIAN_POINT('Ctrl Pts',(-2.70965695523787,1.,-2.93442516311179));
#55532=CARTESIAN_POINT('Ctrl Pts',(-2.71642190053592,-1.,-2.93792519474972));
#55533=CARTESIAN_POINT('Ctrl Pts',(-2.71642190053592,1.,-2.93792519474972));
#55534=CARTESIAN_POINT('Ctrl Pts',(-2.72321571511337,-1.,-2.94139351933897));
#55535=CARTESIAN_POINT('Ctrl Pts',(-2.72321571511337,1.,-2.94139351933897));
#55536=CARTESIAN_POINT('Ctrl Pts',(-2.73003657371617,-1.,-2.94482887675143));
#55537=CARTESIAN_POINT('Ctrl Pts',(-2.73003657371617,1.,-2.94482887675143));
#55538=CARTESIAN_POINT('Ctrl Pts',(-2.73688288329808,-1.,-2.94823023414364));
#55539=CARTESIAN_POINT('Ctrl Pts',(-2.73688288329808,1.,-2.94823023414364));
#55540=CARTESIAN_POINT('Ctrl Pts',(-2.74375379492172,-1.,-2.95159737214266));
#55541=CARTESIAN_POINT('Ctrl Pts',(-2.74375379492172,1.,-2.95159737214266));
#55542=CARTESIAN_POINT('Ctrl Pts',(-2.75064903318947,-1.,-2.95493069316161));
#55543=CARTESIAN_POINT('Ctrl Pts',(-2.75064903318947,1.,-2.95493069316161));
#55544=CARTESIAN_POINT('Ctrl Pts',(-2.7575686788835,-1.,-2.95823097665896));
#55545=CARTESIAN_POINT('Ctrl Pts',(-2.7575686788835,1.,-2.95823097665896));
#55546=CARTESIAN_POINT('Ctrl Pts',(-2.76451296269557,-1.,-2.96149914764818));
#55547=CARTESIAN_POINT('Ctrl Pts',(-2.76451296269557,1.,-2.96149914764818));
#55548=CARTESIAN_POINT('Ctrl Pts',(-2.77148206836498,-1.,-2.96473605585583));
#55549=CARTESIAN_POINT('Ctrl Pts',(-2.77148206836498,1.,-2.96473605585583));
#55550=CARTESIAN_POINT('Ctrl Pts',(-2.7784758954285,-1.,-2.96794221043036));
#55551=CARTESIAN_POINT('Ctrl Pts',(-2.7784758954285,1.,-2.96794221043036));
#55552=CARTESIAN_POINT('Ctrl Pts',(-2.78549409123769,-1.,-2.97111781461465));
#55553=CARTESIAN_POINT('Ctrl Pts',(-2.78549409123769,1.,-2.97111781461465));
#55554=CARTESIAN_POINT('Ctrl Pts',(-2.79253615718248,-1.,-2.9742628834758));
#55555=CARTESIAN_POINT('Ctrl Pts',(-2.79253615718248,1.,-2.9742628834758));
#55556=CARTESIAN_POINT('Ctrl Pts',(-2.7996015327823,-1.,-2.97737733718287));
#55557=CARTESIAN_POINT('Ctrl Pts',(-2.7996015327823,1.,-2.97737733718287));
#55558=CARTESIAN_POINT('Ctrl Pts',(-2.80668968101106,-1.,-2.98046109647241));
#55559=CARTESIAN_POINT('Ctrl Pts',(-2.80668968101106,1.,-2.98046109647241));
#55560=CARTESIAN_POINT('Ctrl Pts',(-2.81380019196286,-1.,-2.98351419779767));
#55561=CARTESIAN_POINT('Ctrl Pts',(-2.81380019196286,1.,-2.98351419779767));
#55562=CARTESIAN_POINT('Ctrl Pts',(-2.82093279065457,-1.,-2.9865368066918));
#55563=CARTESIAN_POINT('Ctrl Pts',(-2.82093279065457,1.,-2.9865368066918));
#55564=CARTESIAN_POINT('Ctrl Pts',(-2.82808728190157,-1.,-2.98952916401446));
#55565=CARTESIAN_POINT('Ctrl Pts',(-2.82808728190157,1.,-2.98952916401446));
#55566=CARTESIAN_POINT('Ctrl Pts',(-2.83526351254248,-1.,-2.99249155170339));
#55567=CARTESIAN_POINT('Ctrl Pts',(-2.83526351254248,1.,-2.99249155170339));
#55568=CARTESIAN_POINT('Ctrl Pts',(-2.84246132984415,-1.,-2.99542425341685));
#55569=CARTESIAN_POINT('Ctrl Pts',(-2.84246132984415,1.,-2.99542425341685));
#55570=CARTESIAN_POINT('Ctrl Pts',(-2.84968053289451,-1.,-2.99832751144925));
#55571=CARTESIAN_POINT('Ctrl Pts',(-2.84968053289451,1.,-2.99832751144925));
#55572=CARTESIAN_POINT('Ctrl Pts',(-2.85692085715686,-1.,-3.00120150796095));
#55573=CARTESIAN_POINT('Ctrl Pts',(-2.85692085715686,1.,-3.00120150796095));
#55574=CARTESIAN_POINT('Ctrl Pts',(-2.86418200833667,-1.,-3.00404638316867));
#55575=CARTESIAN_POINT('Ctrl Pts',(-2.86418200833667,1.,-3.00404638316867));
#55576=CARTESIAN_POINT('Ctrl Pts',(-2.87146368430502,-1.,-3.00686224485784));
#55577=CARTESIAN_POINT('Ctrl Pts',(-2.87146368430502,1.,-3.00686224485784));
#55578=CARTESIAN_POINT('Ctrl Pts',(-2.87876560072727,-1.,-3.00964918108476));
#55579=CARTESIAN_POINT('Ctrl Pts',(-2.87876560072727,1.,-3.00964918108476));
#55580=CARTESIAN_POINT('Ctrl Pts',(-2.8860875170608,-1.,-3.01240727308829));
#55581=CARTESIAN_POINT('Ctrl Pts',(-2.8860875170608,1.,-3.01240727308829));
#55582=CARTESIAN_POINT('Ctrl Pts',(-2.89342925566321,-1.,-3.01513660431928));
#55583=CARTESIAN_POINT('Ctrl Pts',(-2.89342925566321,1.,-3.01513660431928));
#55584=CARTESIAN_POINT('Ctrl Pts',(-2.9007906910105,-1.,-3.01783725121981));
#55585=CARTESIAN_POINT('Ctrl Pts',(-2.9007906910105,1.,-3.01783725121981));
#55586=CARTESIAN_POINT('Ctrl Pts',(-2.90669553302526,-1.,-3.01997487193503));
#55587=CARTESIAN_POINT('Ctrl Pts',(-2.90669553302526,1.,-3.01997487193503));
#55588=CARTESIAN_POINT('Ctrl Pts',(-2.91113297348212,-1.,-3.02156522742431));
#55589=CARTESIAN_POINT('Ctrl Pts',(-2.91113297348212,1.,-3.02156522742431));
#55590=CARTESIAN_POINT('Ctrl Pts',(-2.91409518070399,-1.,-3.02261975104593));
#55591=CARTESIAN_POINT('Ctrl Pts',(-2.91409518070399,1.,-3.02261975104593));
#55592=CARTESIAN_POINT('Ctrl Pts',(-2.91557726271063,-1.,-3.02314558451372));
#55593=CARTESIAN_POINT('Ctrl Pts',(-2.91557726271063,1.,-3.02314558451372));
#55594=CARTESIAN_POINT('',(-2.50410331873176,1.,-2.79140942341258));
#55595=CARTESIAN_POINT('Ctrl Pts',(-2.50410331873176,-1.,-2.79140942341258));
#55596=CARTESIAN_POINT('Ctrl Pts',(-2.50410331873176,-0.666666666666667,
-2.79140942341258));
#55597=CARTESIAN_POINT('Ctrl Pts',(-2.50410331873176,-0.333333333333333,
-2.79140942341258));
#55598=CARTESIAN_POINT('Ctrl Pts',(-2.50410331873176,0.333333333333333,
-2.79140942341258));
#55599=CARTESIAN_POINT('Ctrl Pts',(-2.50410331873176,0.666666666666667,
-2.79140942341258));
#55600=CARTESIAN_POINT('Ctrl Pts',(-2.50410331873176,1.,-2.79140942341258));
#55601=CARTESIAN_POINT('',(-2.91557726271063,1.,-3.02314558451372));
#55602=CARTESIAN_POINT('',(-2.91557726271063,0.,-3.02314558451372));
#55603=CARTESIAN_POINT('Ctrl Pts',(-2.50410331873176,1.,-2.79140942341258));
#55604=CARTESIAN_POINT('Ctrl Pts',(-2.50410700351493,1.,-2.79145823440781));
#55605=CARTESIAN_POINT('Ctrl Pts',(-2.50417932839313,1.,-2.79164172518905));
#55606=CARTESIAN_POINT('Ctrl Pts',(-2.50455968395146,1.,-2.79217568804755));
#55607=CARTESIAN_POINT('Ctrl Pts',(-2.50567182569081,1.,-2.79344192164147));
#55608=CARTESIAN_POINT('Ctrl Pts',(-2.50810555977671,1.,-2.79596878057287));
#55609=CARTESIAN_POINT('Ctrl Pts',(-2.51186983687818,1.,-2.79970585014168));
#55610=CARTESIAN_POINT('Ctrl Pts',(-2.51660190465805,1.,-2.80427363984653));
#55611=CARTESIAN_POINT('Ctrl Pts',(-2.52205778589653,1.,-2.80941521966941));
#55612=CARTESIAN_POINT('Ctrl Pts',(-2.52796388055278,1.,-2.81484379048475));
#55613=CARTESIAN_POINT('Ctrl Pts',(-2.53405679667412,1.,-2.82028550483689));
#55614=CARTESIAN_POINT('Ctrl Pts',(-2.54012272520199,1.,-2.8255216764922));
#55615=CARTESIAN_POINT('Ctrl Pts',(-2.54604736792655,1.,-2.83044254225917));
#55616=CARTESIAN_POINT('Ctrl Pts',(-2.55182152807077,1.,-2.83505269592536));
#55617=CARTESIAN_POINT('Ctrl Pts',(-2.55749952145241,1.,-2.83942515220782));
#55618=CARTESIAN_POINT('Ctrl Pts',(-2.56316920798513,1.,-2.84366802680237));
#55619=CARTESIAN_POINT('Ctrl Pts',(-2.56891984251721,1.,-2.84788893329067));
#55620=CARTESIAN_POINT('Ctrl Pts',(-2.57480482727081,1.,-2.85215360144431));
#55621=CARTESIAN_POINT('Ctrl Pts',(-2.58082875254357,1.,-2.85647171715092));
#55622=CARTESIAN_POINT('Ctrl Pts',(-2.58696770643524,1.,-2.86081999003629));
#55623=CARTESIAN_POINT('Ctrl Pts',(-2.59318160184908,1.,-2.86515629953513));
#55624=CARTESIAN_POINT('Ctrl Pts',(-2.5994287522321,1.,-2.86943633170722));
#55625=CARTESIAN_POINT('Ctrl Pts',(-2.60568177881303,1.,-2.87363176656501));
#55626=CARTESIAN_POINT('Ctrl Pts',(-2.61193507170955,1.,-2.87773881947915));
#55627=CARTESIAN_POINT('Ctrl Pts',(-2.61819596473108,1.,-2.88176821427525));
#55628=CARTESIAN_POINT('Ctrl Pts',(-2.62447947640262,1.,-2.88573922195059));
#55629=CARTESIAN_POINT('Ctrl Pts',(-2.63080195420767,1.,-2.88967244854239));
#55630=CARTESIAN_POINT('Ctrl Pts',(-2.63717442263932,1.,-2.89358228854544));
#55631=CARTESIAN_POINT('Ctrl Pts',(-2.64359851684131,1.,-2.89747231723345));
#55632=CARTESIAN_POINT('Ctrl Pts',(-2.65007017365564,1.,-2.90133950224867));
#55633=CARTESIAN_POINT('Ctrl Pts',(-2.65658188464282,1.,-2.90517678087461));
#55634=CARTESIAN_POINT('Ctrl Pts',(-2.6631254261681,1.,-2.90897617968923));
#55635=CARTESIAN_POINT('Ctrl Pts',(-2.66969458792631,1.,-2.91273193382882));
#55636=CARTESIAN_POINT('Ctrl Pts',(-2.67628728855312,1.,-2.91644290704285));
#55637=CARTESIAN_POINT('Ctrl Pts',(-2.68290409279688,1.,-2.92011090722152));
#55638=CARTESIAN_POINT('Ctrl Pts',(-2.68954721165339,1.,-2.92373955325875));
#55639=CARTESIAN_POINT('Ctrl Pts',(-2.69621932864301,1.,-2.92733294395267));
#55640=CARTESIAN_POINT('Ctrl Pts',(-2.70292247416885,1.,-2.93089438233749));
#55641=CARTESIAN_POINT('Ctrl Pts',(-2.70965695523787,1.,-2.93442516311179));
#55642=CARTESIAN_POINT('Ctrl Pts',(-2.71642190053592,1.,-2.93792519474972));
#55643=CARTESIAN_POINT('Ctrl Pts',(-2.72321571511337,1.,-2.94139351933897));
#55644=CARTESIAN_POINT('Ctrl Pts',(-2.73003657371617,1.,-2.94482887675143));
#55645=CARTESIAN_POINT('Ctrl Pts',(-2.73688288329808,1.,-2.94823023414364));
#55646=CARTESIAN_POINT('Ctrl Pts',(-2.74375379492172,1.,-2.95159737214266));
#55647=CARTESIAN_POINT('Ctrl Pts',(-2.75064903318947,1.,-2.95493069316161));
#55648=CARTESIAN_POINT('Ctrl Pts',(-2.7575686788835,1.,-2.95823097665896));
#55649=CARTESIAN_POINT('Ctrl Pts',(-2.76451296269557,1.,-2.96149914764818));
#55650=CARTESIAN_POINT('Ctrl Pts',(-2.77148206836498,1.,-2.96473605585583));
#55651=CARTESIAN_POINT('Ctrl Pts',(-2.7784758954285,1.,-2.96794221043036));
#55652=CARTESIAN_POINT('Ctrl Pts',(-2.78549409123769,1.,-2.97111781461465));
#55653=CARTESIAN_POINT('Ctrl Pts',(-2.79253615718248,1.,-2.9742628834758));
#55654=CARTESIAN_POINT('Ctrl Pts',(-2.7996015327823,1.,-2.97737733718287));
#55655=CARTESIAN_POINT('Ctrl Pts',(-2.80668968101106,1.,-2.98046109647241));
#55656=CARTESIAN_POINT('Ctrl Pts',(-2.81380019196286,1.,-2.98351419779767));
#55657=CARTESIAN_POINT('Ctrl Pts',(-2.82093279065457,1.,-2.9865368066918));
#55658=CARTESIAN_POINT('Ctrl Pts',(-2.82808728190157,1.,-2.98952916401446));
#55659=CARTESIAN_POINT('Ctrl Pts',(-2.83526351254248,1.,-2.99249155170339));
#55660=CARTESIAN_POINT('Ctrl Pts',(-2.84246132984415,1.,-2.99542425341685));
#55661=CARTESIAN_POINT('Ctrl Pts',(-2.84968053289451,1.,-2.99832751144925));
#55662=CARTESIAN_POINT('Ctrl Pts',(-2.85692085715686,1.,-3.00120150796095));
#55663=CARTESIAN_POINT('Ctrl Pts',(-2.86418200833667,1.,-3.00404638316867));
#55664=CARTESIAN_POINT('Ctrl Pts',(-2.87146368430502,1.,-3.00686224485784));
#55665=CARTESIAN_POINT('Ctrl Pts',(-2.87876560072727,1.,-3.00964918108476));
#55666=CARTESIAN_POINT('Ctrl Pts',(-2.8860875170608,1.,-3.01240727308829));
#55667=CARTESIAN_POINT('Ctrl Pts',(-2.89342925566321,1.,-3.01513660431928));
#55668=CARTESIAN_POINT('Ctrl Pts',(-2.9007906910105,1.,-3.01783725121981));
#55669=CARTESIAN_POINT('Ctrl Pts',(-2.90669553302526,1.,-3.01997487193503));
#55670=CARTESIAN_POINT('Ctrl Pts',(-2.91113297348212,1.,-3.02156522742431));
#55671=CARTESIAN_POINT('Ctrl Pts',(-2.91409518070399,1.,-3.02261975104593));
#55672=CARTESIAN_POINT('Ctrl Pts',(-2.91557726271063,1.,-3.02314558451372));
#55673=CARTESIAN_POINT('Origin',(-2.91557726271063,0.,-3.02314558451372));
#55674=CARTESIAN_POINT('',(-3.02314558451372,1.,-2.91557726271063));
#55675=CARTESIAN_POINT('Origin',(0.,0.,0.));
#55676=CARTESIAN_POINT('',(-2.36531447826213,1.,-2.90994629141562));
#55677=CARTESIAN_POINT('Origin',(0.,1.,0.));
#55678=CARTESIAN_POINT('Ctrl Pts',(-2.36531447826213,1.,-2.90994629141562));
#55679=CARTESIAN_POINT('Ctrl Pts',(-2.36531447826213,0.666666666666667,
-2.90994629141562));
#55680=CARTESIAN_POINT('Ctrl Pts',(-2.36531447826213,0.333333333333333,
-2.90994629141562));
#55681=CARTESIAN_POINT('Ctrl Pts',(-2.36531447826213,-0.333333333333333,
-2.90994629141562));
#55682=CARTESIAN_POINT('Ctrl Pts',(-2.36531447826213,-0.666666666666667,
-2.90994629141562));
#55683=CARTESIAN_POINT('Ctrl Pts',(-2.36531447826213,-1.,-2.90994629141562));
#55684=CARTESIAN_POINT('Ctrl Pts',(-2.52982887637028,-1.,-3.35260583073571));
#55685=CARTESIAN_POINT('Ctrl Pts',(-2.52982887637028,1.,-3.35260583073571));
#55686=CARTESIAN_POINT('Ctrl Pts',(-2.52954136549357,-1.,-3.35105973714426));
#55687=CARTESIAN_POINT('Ctrl Pts',(-2.52954136549357,1.,-3.35105973714426));
#55688=CARTESIAN_POINT('Ctrl Pts',(-2.5289632161143,-1.,-3.34796903577628));
#55689=CARTESIAN_POINT('Ctrl Pts',(-2.5289632161143,1.,-3.34796903577628));
#55690=CARTESIAN_POINT('Ctrl Pts',(-2.52808660916879,-1.,-3.34333744117093));
#55691=CARTESIAN_POINT('Ctrl Pts',(-2.52808660916879,1.,-3.34333744117093));
#55692=CARTESIAN_POINT('Ctrl Pts',(-2.52689902691551,-1.,-3.33717090000955));
#55693=CARTESIAN_POINT('Ctrl Pts',(-2.52689902691551,1.,-3.33717090000955));
#55694=CARTESIAN_POINT('Ctrl Pts',(-2.52538321165774,-1.,-3.32947762189049));
#55695=CARTESIAN_POINT('Ctrl Pts',(-2.52538321165774,1.,-3.32947762189049));
#55696=CARTESIAN_POINT('Ctrl Pts',(-2.52383598396878,-1.,-3.32179931079521));
#55697=CARTESIAN_POINT('Ctrl Pts',(-2.52383598396878,1.,-3.32179931079521));
#55698=CARTESIAN_POINT('Ctrl Pts',(-2.52225724871375,-1.,-3.31413607874727));
#55699=CARTESIAN_POINT('Ctrl Pts',(-2.52225724871375,1.,-3.31413607874727));
#55700=CARTESIAN_POINT('Ctrl Pts',(-2.52064689568167,-1.,-3.30648808814986));
#55701=CARTESIAN_POINT('Ctrl Pts',(-2.52064689568167,1.,-3.30648808814986));
#55702=CARTESIAN_POINT('Ctrl Pts',(-2.51900480700548,-1.,-3.29885556387661));
#55703=CARTESIAN_POINT('Ctrl Pts',(-2.51900480700548,1.,-3.29885556387661));
#55704=CARTESIAN_POINT('Ctrl Pts',(-2.51733085123316,-1.,-3.2912387729863));
#55705=CARTESIAN_POINT('Ctrl Pts',(-2.51733085123316,1.,-3.2912387729863));
#55706=CARTESIAN_POINT('Ctrl Pts',(-2.51562487464215,-1.,-3.28363799702583));
#55707=CARTESIAN_POINT('Ctrl Pts',(-2.51562487464215,1.,-3.28363799702583));
#55708=CARTESIAN_POINT('Ctrl Pts',(-2.51388669270329,-1.,-3.27605350473048));
#55709=CARTESIAN_POINT('Ctrl Pts',(-2.51388669270329,1.,-3.27605350473048));
#55710=CARTESIAN_POINT('Ctrl Pts',(-2.51211608411539,-1.,-3.26848552888271));
#55711=CARTESIAN_POINT('Ctrl Pts',(-2.51211608411539,1.,-3.26848552888271));
#55712=CARTESIAN_POINT('Ctrl Pts',(-2.51031277813697,-1.,-3.26093423001716));
#55713=CARTESIAN_POINT('Ctrl Pts',(-2.51031277813697,1.,-3.26093423001716));
#55714=CARTESIAN_POINT('Ctrl Pts',(-2.50847647070936,-1.,-3.25339971461265));
#55715=CARTESIAN_POINT('Ctrl Pts',(-2.50847647070936,1.,-3.25339971461265));
#55716=CARTESIAN_POINT('Ctrl Pts',(-2.50660685940645,-1.,-3.24588208984042));
#55717=CARTESIAN_POINT('Ctrl Pts',(-2.50660685940645,1.,-3.24588208984042));
#55718=CARTESIAN_POINT('Ctrl Pts',(-2.50470367580078,-1.,-3.23838151080383));
#55719=CARTESIAN_POINT('Ctrl Pts',(-2.50470367580078,1.,-3.23838151080383));
#55720=CARTESIAN_POINT('Ctrl Pts',(-2.50276671338074,-1.,-3.23089822320596));
#55721=CARTESIAN_POINT('Ctrl Pts',(-2.50276671338074,1.,-3.23089822320596));
#55722=CARTESIAN_POINT('Ctrl Pts',(-2.5007958720187,-1.,-3.22343262620387));
#55723=CARTESIAN_POINT('Ctrl Pts',(-2.5007958720187,1.,-3.22343262620387));
#55724=CARTESIAN_POINT('Ctrl Pts',(-2.49879114599293,-1.,-3.21598526261157));
#55725=CARTESIAN_POINT('Ctrl Pts',(-2.49879114599293,1.,-3.21598526261157));
#55726=CARTESIAN_POINT('Ctrl Pts',(-2.49675252647298,-1.,-3.2085566984974));
#55727=CARTESIAN_POINT('Ctrl Pts',(-2.49675252647298,1.,-3.2085566984974));
#55728=CARTESIAN_POINT('Ctrl Pts',(-2.49467992057726,-1.,-3.20114742397549));
#55729=CARTESIAN_POINT('Ctrl Pts',(-2.49467992057726,1.,-3.20114742397549));
#55730=CARTESIAN_POINT('Ctrl Pts',(-2.4925730723986,-1.,-3.19375775555814));
#55731=CARTESIAN_POINT('Ctrl Pts',(-2.4925730723986,1.,-3.19375775555814));
#55732=CARTESIAN_POINT('Ctrl Pts',(-2.49043146334095,-1.,-3.18638771282315));
#55733=CARTESIAN_POINT('Ctrl Pts',(-2.49043146334095,1.,-3.18638771282315));
#55734=CARTESIAN_POINT('Ctrl Pts',(-2.48825428288243,-1.,-3.17903698136679));
#55735=CARTESIAN_POINT('Ctrl Pts',(-2.48825428288243,1.,-3.17903698136679));
#55736=CARTESIAN_POINT('Ctrl Pts',(-2.48604065348619,-1.,-3.17170518863357));
#55737=CARTESIAN_POINT('Ctrl Pts',(-2.48604065348619,1.,-3.17170518863357));
#55738=CARTESIAN_POINT('Ctrl Pts',(-2.48378981792739,-1.,-3.16439213290181));
#55739=CARTESIAN_POINT('Ctrl Pts',(-2.48378981792739,1.,-3.16439213290181));
#55740=CARTESIAN_POINT('Ctrl Pts',(-2.48150133566568,-1.,-3.15709802322735));
#55741=CARTESIAN_POINT('Ctrl Pts',(-2.48150133566568,1.,-3.15709802322735));
#55742=CARTESIAN_POINT('Ctrl Pts',(-2.47917529057016,-1.,-3.14982373241335));
#55743=CARTESIAN_POINT('Ctrl Pts',(-2.47917529057016,1.,-3.14982373241335));
#55744=CARTESIAN_POINT('Ctrl Pts',(-2.47681245356095,-1.,-3.14257099546531));
#55745=CARTESIAN_POINT('Ctrl Pts',(-2.47681245356095,1.,-3.14257099546531));
#55746=CARTESIAN_POINT('Ctrl Pts',(-2.47441378371923,-1.,-3.13534181229282));
#55747=CARTESIAN_POINT('Ctrl Pts',(-2.47441378371923,1.,-3.13534181229282));
#55748=CARTESIAN_POINT('Ctrl Pts',(-2.47197997765868,-1.,-3.12813790805948));
#55749=CARTESIAN_POINT('Ctrl Pts',(-2.47197997765868,1.,-3.12813790805948));
#55750=CARTESIAN_POINT('Ctrl Pts',(-2.4695109894747,-1.,-3.12096015766984));
#55751=CARTESIAN_POINT('Ctrl Pts',(-2.4695109894747,1.,-3.12096015766984));
#55752=CARTESIAN_POINT('Ctrl Pts',(-2.46700558843507,-1.,-3.11380805536124));
#55753=CARTESIAN_POINT('Ctrl Pts',(-2.46700558843507,1.,-3.11380805536124));
#55754=CARTESIAN_POINT('Ctrl Pts',(-2.46446082979645,-1.,-3.10667907901981));
#55755=CARTESIAN_POINT('Ctrl Pts',(-2.46446082979645,1.,-3.10667907901981));
#55756=CARTESIAN_POINT('Ctrl Pts',(-2.4618730850188,-1.,-3.09956993697048));
#55757=CARTESIAN_POINT('Ctrl Pts',(-2.4618730850188,1.,-3.09956993697048));
#55758=CARTESIAN_POINT('Ctrl Pts',(-2.45923912563875,-1.,-3.09247787931881));
#55759=CARTESIAN_POINT('Ctrl Pts',(-2.45923912563875,1.,-3.09247787931881));
#55760=CARTESIAN_POINT('Ctrl Pts',(-2.45655725437037,-1.,-3.08540206545313));
#55761=CARTESIAN_POINT('Ctrl Pts',(-2.45655725437037,1.,-3.08540206545313));
#55762=CARTESIAN_POINT('Ctrl Pts',(-2.45382826787795,-1.,-3.07834472886145));
#55763=CARTESIAN_POINT('Ctrl Pts',(-2.45382826787795,1.,-3.07834472886145));
#55764=CARTESIAN_POINT('Ctrl Pts',(-2.45105688854432,-1.,-3.0713129052131));
#55765=CARTESIAN_POINT('Ctrl Pts',(-2.45105688854432,1.,-3.0713129052131));
#55766=CARTESIAN_POINT('Ctrl Pts',(-2.44824970516558,-1.,-3.06431596421422));
#55767=CARTESIAN_POINT('Ctrl Pts',(-2.44824970516558,1.,-3.06431596421422));
#55768=CARTESIAN_POINT('Ctrl Pts',(-2.44541251892568,-1.,-3.05736242671521));
#55769=CARTESIAN_POINT('Ctrl Pts',(-2.44541251892568,1.,-3.05736242671521));
#55770=CARTESIAN_POINT('Ctrl Pts',(-2.44254768923109,-1.,-3.05045678021509));
#55771=CARTESIAN_POINT('Ctrl Pts',(-2.44254768923109,1.,-3.05045678021509));
#55772=CARTESIAN_POINT('Ctrl Pts',(-2.43965194061849,-1.,-3.04359685040545));
#55773=CARTESIAN_POINT('Ctrl Pts',(-2.43965194061849,1.,-3.04359685040545));
#55774=CARTESIAN_POINT('Ctrl Pts',(-2.43671278042394,-1.,-3.03676949672797));
#55775=CARTESIAN_POINT('Ctrl Pts',(-2.43671278042394,1.,-3.03676949672797));
#55776=CARTESIAN_POINT('Ctrl Pts',(-2.43371241361462,-1.,-3.02995534946946));
#55777=CARTESIAN_POINT('Ctrl Pts',(-2.43371241361462,1.,-3.02995534946946));
#55778=CARTESIAN_POINT('Ctrl Pts',(-2.43063415586615,-1.,-3.02313656035977));
#55779=CARTESIAN_POINT('Ctrl Pts',(-2.43063415586615,1.,-3.02313656035977));
#55780=CARTESIAN_POINT('Ctrl Pts',(-2.4274685626416,-1.,-3.01630420830494));
#55781=CARTESIAN_POINT('Ctrl Pts',(-2.4274685626416,1.,-3.01630420830494));
#55782=CARTESIAN_POINT('Ctrl Pts',(-2.42421849439625,-1.,-3.00946442616674));
#55783=CARTESIAN_POINT('Ctrl Pts',(-2.42421849439625,1.,-3.00946442616674));
#55784=CARTESIAN_POINT('Ctrl Pts',(-2.42090763946812,-1.,-3.00264868586038));
#55785=CARTESIAN_POINT('Ctrl Pts',(-2.42090763946812,1.,-3.00264868586038));
#55786=CARTESIAN_POINT('Ctrl Pts',(-2.4175732450056,-1.,-2.99590509293561));
#55787=CARTESIAN_POINT('Ctrl Pts',(-2.4175732450056,1.,-2.99590509293561));
#55788=CARTESIAN_POINT('Ctrl Pts',(-2.4142506419963,-1.,-2.98927983005851));
#55789=CARTESIAN_POINT('Ctrl Pts',(-2.4142506419963,1.,-2.98927983005851));
#55790=CARTESIAN_POINT('Ctrl Pts',(-2.41095909342591,-1.,-2.98280015815132));
#55791=CARTESIAN_POINT('Ctrl Pts',(-2.41095909342591,1.,-2.98280015815132));
#55792=CARTESIAN_POINT('Ctrl Pts',(-2.40768975073691,-1.,-2.97646002822395));
#55793=CARTESIAN_POINT('Ctrl Pts',(-2.40768975073691,1.,-2.97646002822395));
#55794=CARTESIAN_POINT('Ctrl Pts',(-2.40438604734848,-1.,-2.97019641312272));
#55795=CARTESIAN_POINT('Ctrl Pts',(-2.40438604734848,1.,-2.97019641312272));
#55796=CARTESIAN_POINT('Ctrl Pts',(-2.40095565711535,-1.,-2.96390432240181));
#55797=CARTESIAN_POINT('Ctrl Pts',(-2.40095565711535,1.,-2.96390432240181));
#55798=CARTESIAN_POINT('Ctrl Pts',(-2.39730553974412,-1.,-2.95748006482811));
#55799=CARTESIAN_POINT('Ctrl Pts',(-2.39730553974412,1.,-2.95748006482811));
#55800=CARTESIAN_POINT('Ctrl Pts',(-2.39337207631613,-1.,-2.95085857128372));
#55801=CARTESIAN_POINT('Ctrl Pts',(-2.39337207631613,1.,-2.95085857128372));
#55802=CARTESIAN_POINT('Ctrl Pts',(-2.38914929090806,-1.,-2.94404820669135));
#55803=CARTESIAN_POINT('Ctrl Pts',(-2.38914929090806,1.,-2.94404820669135));
#55804=CARTESIAN_POINT('Ctrl Pts',(-2.38472771516476,-1.,-2.93717903280599));
#55805=CARTESIAN_POINT('Ctrl Pts',(-2.38472771516476,1.,-2.93717903280599));
#55806=CARTESIAN_POINT('Ctrl Pts',(-2.3802898958232,-1.,-2.93049643640517));
#55807=CARTESIAN_POINT('Ctrl Pts',(-2.3802898958232,1.,-2.93049643640517));
#55808=CARTESIAN_POINT('Ctrl Pts',(-2.37606510524271,-1.,-2.92430340582912));
#55809=CARTESIAN_POINT('Ctrl Pts',(-2.37606510524271,1.,-2.92430340582912));
#55810=CARTESIAN_POINT('Ctrl Pts',(-2.37229381109939,-1.,-2.9189150379156));
#55811=CARTESIAN_POINT('Ctrl Pts',(-2.37229381109939,1.,-2.9189150379156));
#55812=CARTESIAN_POINT('Ctrl Pts',(-2.36919161373074,-1.,-2.91461249883016));
#55813=CARTESIAN_POINT('Ctrl Pts',(-2.36919161373074,1.,-2.91461249883016));
#55814=CARTESIAN_POINT('Ctrl Pts',(-2.36690501170317,-1.,-2.9115863784165));
#55815=CARTESIAN_POINT('Ctrl Pts',(-2.36690501170317,1.,-2.9115863784165));
#55816=CARTESIAN_POINT('Ctrl Pts',(-2.36578327194396,-1.,-2.91025813829606));
#55817=CARTESIAN_POINT('Ctrl Pts',(-2.36578327194396,1.,-2.91025813829606));
#55818=CARTESIAN_POINT('Ctrl Pts',(-2.36535052956704,-1.,-2.90989022547738));
#55819=CARTESIAN_POINT('Ctrl Pts',(-2.36535052956704,1.,-2.90989022547738));
#55820=CARTESIAN_POINT('Ctrl Pts',(-2.36524348105023,-1.,-2.90992398626098));
#55821=CARTESIAN_POINT('Ctrl Pts',(-2.36524348105023,1.,-2.90992398626098));
#55822=CARTESIAN_POINT('Ctrl Pts',(-2.36523532225181,-1.,-2.91001063062876));
#55823=CARTESIAN_POINT('Ctrl Pts',(-2.36523532225181,1.,-2.91001063062876));
#55824=CARTESIAN_POINT('',(-2.52982887637028,1.,-3.35260583073571));
#55825=CARTESIAN_POINT('Ctrl Pts',(-2.52982887637028,1.,-3.35260583073571));
#55826=CARTESIAN_POINT('Ctrl Pts',(-2.52954136549357,1.,-3.35105973714426));
#55827=CARTESIAN_POINT('Ctrl Pts',(-2.5289632161143,1.,-3.34796903577628));
#55828=CARTESIAN_POINT('Ctrl Pts',(-2.52808660916879,1.,-3.34333744117093));
#55829=CARTESIAN_POINT('Ctrl Pts',(-2.52689902691551,1.,-3.33717090000955));
#55830=CARTESIAN_POINT('Ctrl Pts',(-2.52538321165774,1.,-3.32947762189049));
#55831=CARTESIAN_POINT('Ctrl Pts',(-2.52383598396878,1.,-3.32179931079521));
#55832=CARTESIAN_POINT('Ctrl Pts',(-2.52225724871375,1.,-3.31413607874727));
#55833=CARTESIAN_POINT('Ctrl Pts',(-2.52064689568167,1.,-3.30648808814986));
#55834=CARTESIAN_POINT('Ctrl Pts',(-2.51900480700548,1.,-3.29885556387661));
#55835=CARTESIAN_POINT('Ctrl Pts',(-2.51733085123316,1.,-3.2912387729863));
#55836=CARTESIAN_POINT('Ctrl Pts',(-2.51562487464215,1.,-3.28363799702583));
#55837=CARTESIAN_POINT('Ctrl Pts',(-2.51388669270329,1.,-3.27605350473048));
#55838=CARTESIAN_POINT('Ctrl Pts',(-2.51211608411539,1.,-3.26848552888271));
#55839=CARTESIAN_POINT('Ctrl Pts',(-2.51031277813697,1.,-3.26093423001716));
#55840=CARTESIAN_POINT('Ctrl Pts',(-2.50847647070936,1.,-3.25339971461265));
#55841=CARTESIAN_POINT('Ctrl Pts',(-2.50660685940645,1.,-3.24588208984042));
#55842=CARTESIAN_POINT('Ctrl Pts',(-2.50470367580078,1.,-3.23838151080383));
#55843=CARTESIAN_POINT('Ctrl Pts',(-2.50276671338074,1.,-3.23089822320596));
#55844=CARTESIAN_POINT('Ctrl Pts',(-2.5007958720187,1.,-3.22343262620387));
#55845=CARTESIAN_POINT('Ctrl Pts',(-2.49879114599293,1.,-3.21598526261157));
#55846=CARTESIAN_POINT('Ctrl Pts',(-2.49675252647298,1.,-3.2085566984974));
#55847=CARTESIAN_POINT('Ctrl Pts',(-2.49467992057726,1.,-3.20114742397549));
#55848=CARTESIAN_POINT('Ctrl Pts',(-2.4925730723986,1.,-3.19375775555814));
#55849=CARTESIAN_POINT('Ctrl Pts',(-2.49043146334095,1.,-3.18638771282315));
#55850=CARTESIAN_POINT('Ctrl Pts',(-2.48825428288243,1.,-3.17903698136679));
#55851=CARTESIAN_POINT('Ctrl Pts',(-2.48604065348619,1.,-3.17170518863357));
#55852=CARTESIAN_POINT('Ctrl Pts',(-2.48378981792739,1.,-3.16439213290181));
#55853=CARTESIAN_POINT('Ctrl Pts',(-2.48150133566568,1.,-3.15709802322735));
#55854=CARTESIAN_POINT('Ctrl Pts',(-2.47917529057016,1.,-3.14982373241335));
#55855=CARTESIAN_POINT('Ctrl Pts',(-2.47681245356095,1.,-3.14257099546531));
#55856=CARTESIAN_POINT('Ctrl Pts',(-2.47441378371923,1.,-3.13534181229282));
#55857=CARTESIAN_POINT('Ctrl Pts',(-2.47197997765868,1.,-3.12813790805948));
#55858=CARTESIAN_POINT('Ctrl Pts',(-2.4695109894747,1.,-3.12096015766984));
#55859=CARTESIAN_POINT('Ctrl Pts',(-2.46700558843507,1.,-3.11380805536124));
#55860=CARTESIAN_POINT('Ctrl Pts',(-2.46446082979645,1.,-3.10667907901981));
#55861=CARTESIAN_POINT('Ctrl Pts',(-2.4618730850188,1.,-3.09956993697048));
#55862=CARTESIAN_POINT('Ctrl Pts',(-2.45923912563875,1.,-3.09247787931881));
#55863=CARTESIAN_POINT('Ctrl Pts',(-2.45655725437037,1.,-3.08540206545313));
#55864=CARTESIAN_POINT('Ctrl Pts',(-2.45382826787795,1.,-3.07834472886145));
#55865=CARTESIAN_POINT('Ctrl Pts',(-2.45105688854432,1.,-3.0713129052131));
#55866=CARTESIAN_POINT('Ctrl Pts',(-2.44824970516558,1.,-3.06431596421422));
#55867=CARTESIAN_POINT('Ctrl Pts',(-2.44541251892568,1.,-3.05736242671521));
#55868=CARTESIAN_POINT('Ctrl Pts',(-2.44254768923109,1.,-3.05045678021509));
#55869=CARTESIAN_POINT('Ctrl Pts',(-2.43965194061849,1.,-3.04359685040545));
#55870=CARTESIAN_POINT('Ctrl Pts',(-2.43671278042394,1.,-3.03676949672797));
#55871=CARTESIAN_POINT('Ctrl Pts',(-2.43371241361462,1.,-3.02995534946946));
#55872=CARTESIAN_POINT('Ctrl Pts',(-2.43063415586615,1.,-3.02313656035977));
#55873=CARTESIAN_POINT('Ctrl Pts',(-2.4274685626416,1.,-3.01630420830494));
#55874=CARTESIAN_POINT('Ctrl Pts',(-2.42421849439625,1.,-3.00946442616674));
#55875=CARTESIAN_POINT('Ctrl Pts',(-2.42090763946812,1.,-3.00264868586038));
#55876=CARTESIAN_POINT('Ctrl Pts',(-2.4175732450056,1.,-2.99590509293561));
#55877=CARTESIAN_POINT('Ctrl Pts',(-2.4142506419963,1.,-2.98927983005851));
#55878=CARTESIAN_POINT('Ctrl Pts',(-2.41095909342591,1.,-2.98280015815132));
#55879=CARTESIAN_POINT('Ctrl Pts',(-2.40768975073691,1.,-2.97646002822395));
#55880=CARTESIAN_POINT('Ctrl Pts',(-2.40438604734848,1.,-2.97019641312272));
#55881=CARTESIAN_POINT('Ctrl Pts',(-2.40095565711535,1.,-2.96390432240181));
#55882=CARTESIAN_POINT('Ctrl Pts',(-2.39730553974412,1.,-2.95748006482811));
#55883=CARTESIAN_POINT('Ctrl Pts',(-2.39337207631613,1.,-2.95085857128372));
#55884=CARTESIAN_POINT('Ctrl Pts',(-2.38914929090806,1.,-2.94404820669135));
#55885=CARTESIAN_POINT('Ctrl Pts',(-2.38472771516476,1.,-2.93717903280599));
#55886=CARTESIAN_POINT('Ctrl Pts',(-2.3802898958232,1.,-2.93049643640517));
#55887=CARTESIAN_POINT('Ctrl Pts',(-2.37606510524271,1.,-2.92430340582912));
#55888=CARTESIAN_POINT('Ctrl Pts',(-2.37229381109939,1.,-2.9189150379156));
#55889=CARTESIAN_POINT('Ctrl Pts',(-2.36919161373074,1.,-2.91461249883016));
#55890=CARTESIAN_POINT('Ctrl Pts',(-2.36707658451709,1.,-2.91181344022628));
#55891=CARTESIAN_POINT('Ctrl Pts',(-2.36599991765853,1.,-2.91051690822262));
#55892=CARTESIAN_POINT('Ctrl Pts',(-2.36553202948741,1.,-2.9100577052777));
#55893=CARTESIAN_POINT('Ctrl Pts',(-2.3653621118858,1.,-2.90995756655559));
#55894=CARTESIAN_POINT('Ctrl Pts',(-2.36531447826213,1.,-2.90994629141563));
#55895=CARTESIAN_POINT('',(-2.52982887637028,0.,-3.35260583073571));
#55896=CARTESIAN_POINT('Ctrl Pts',(-2.03668666247593,-1.,-3.1487152044751));
#55897=CARTESIAN_POINT('Ctrl Pts',(-2.03668666247593,1.,-3.1487152044751));
#55898=CARTESIAN_POINT('Ctrl Pts',(-2.03660173757879,-1.,-3.14869618937258));
#55899=CARTESIAN_POINT('Ctrl Pts',(-2.03660173757879,1.,-3.14869618937258));
#55900=CARTESIAN_POINT('Ctrl Pts',(-2.03653654935592,-1.,-3.14878756590812));
#55901=CARTESIAN_POINT('Ctrl Pts',(-2.03653654935592,1.,-3.14878756590812));
#55902=CARTESIAN_POINT('Ctrl Pts',(-2.03675273049189,-1.,-3.14931281968048));
#55903=CARTESIAN_POINT('Ctrl Pts',(-2.03675273049189,1.,-3.14931281968048));
#55904=CARTESIAN_POINT('Ctrl Pts',(-2.03766932526445,-1.,-3.15079010635742));
#55905=CARTESIAN_POINT('Ctrl Pts',(-2.03766932526445,1.,-3.15079010635742));
#55906=CARTESIAN_POINT('Ctrl Pts',(-2.03984073791519,-1.,-3.15389991674792));
#55907=CARTESIAN_POINT('Ctrl Pts',(-2.03984073791519,1.,-3.15389991674792));
#55908=CARTESIAN_POINT('Ctrl Pts',(-2.04297406404027,-1.,-3.15817983946367));
#55909=CARTESIAN_POINT('Ctrl Pts',(-2.04297406404027,1.,-3.15817983946367));
#55910=CARTESIAN_POINT('Ctrl Pts',(-2.04693331247446,-1.,-3.16343165058912));
#55911=CARTESIAN_POINT('Ctrl Pts',(-2.04693331247446,1.,-3.16343165058912));
#55912=CARTESIAN_POINT('Ctrl Pts',(-2.05151770247233,-1.,-3.16936341689527));
#55913=CARTESIAN_POINT('Ctrl Pts',(-2.05151770247233,1.,-3.16936341689527));
#55914=CARTESIAN_POINT('Ctrl Pts',(-2.05650186773132,-1.,-3.17564906975371));
#55915=CARTESIAN_POINT('Ctrl Pts',(-2.05650186773132,1.,-3.17564906975371));
#55916=CARTESIAN_POINT('Ctrl Pts',(-2.06166849827101,-1.,-3.18197692964614));
#55917=CARTESIAN_POINT('Ctrl Pts',(-2.06166849827101,1.,-3.18197692964614));
#55918=CARTESIAN_POINT('Ctrl Pts',(-2.06684062744112,-1.,-3.18809755562368));
#55919=CARTESIAN_POINT('Ctrl Pts',(-2.06684062744112,1.,-3.18809755562368));
#55920=CARTESIAN_POINT('Ctrl Pts',(-2.07192253497857,-1.,-3.19388465568252));
#55921=CARTESIAN_POINT('Ctrl Pts',(-2.07192253497857,1.,-3.19388465568252));
#55922=CARTESIAN_POINT('Ctrl Pts',(-2.07690441870722,-1.,-3.19934132836019));
#55923=CARTESIAN_POINT('Ctrl Pts',(-2.07690441870722,1.,-3.19934132836019));
#55924=CARTESIAN_POINT('Ctrl Pts',(-2.08182850370878,-1.,-3.2045481863073));
#55925=CARTESIAN_POINT('Ctrl Pts',(-2.08182850370878,1.,-3.2045481863073));
#55926=CARTESIAN_POINT('Ctrl Pts',(-2.08676465517455,-1.,-3.20962575845463));
#55927=CARTESIAN_POINT('Ctrl Pts',(-2.08676465517455,1.,-3.20962575845463));
#55928=CARTESIAN_POINT('Ctrl Pts',(-2.09178419460443,-1.,-3.21469429601654));
#55929=CARTESIAN_POINT('Ctrl Pts',(-2.09178419460443,1.,-3.21469429601654));
#55930=CARTESIAN_POINT('Ctrl Pts',(-2.09692958434895,-1.,-3.21982707347009));
#55931=CARTESIAN_POINT('Ctrl Pts',(-2.09692958434895,1.,-3.21982707347009));
#55932=CARTESIAN_POINT('Ctrl Pts',(-2.10220384298492,-1.,-3.22503437553434));
#55933=CARTESIAN_POINT('Ctrl Pts',(-2.10220384298492,1.,-3.22503437553434));
#55934=CARTESIAN_POINT('Ctrl Pts',(-2.10758699642451,-1.,-3.23028945793289));
#55935=CARTESIAN_POINT('Ctrl Pts',(-2.10758699642451,1.,-3.23028945793289));
#55936=CARTESIAN_POINT('Ctrl Pts',(-2.11304604021773,-1.,-3.23554444767099));
#55937=CARTESIAN_POINT('Ctrl Pts',(-2.11304604021773,1.,-3.23554444767099));
#55938=CARTESIAN_POINT('Ctrl Pts',(-2.11854673326979,-1.,-3.24074905517293));
#55939=CARTESIAN_POINT('Ctrl Pts',(-2.11854673326979,1.,-3.24074905517293));
#55940=CARTESIAN_POINT('Ctrl Pts',(-2.12406646410962,-1.,-3.24587102613376));
#55941=CARTESIAN_POINT('Ctrl Pts',(-2.12406646410962,1.,-3.24587102613376));
#55942=CARTESIAN_POINT('Ctrl Pts',(-2.12960028396832,-1.,-3.25090574494028));
#55943=CARTESIAN_POINT('Ctrl Pts',(-2.12960028396832,1.,-3.25090574494028));
#55944=CARTESIAN_POINT('Ctrl Pts',(-2.13515375878803,-1.,-3.25586495065054));
#55945=CARTESIAN_POINT('Ctrl Pts',(-2.13515375878803,1.,-3.25586495065054));
#55946=CARTESIAN_POINT('Ctrl Pts',(-2.14073870754264,-1.,-3.26077002641879));
#55947=CARTESIAN_POINT('Ctrl Pts',(-2.14073870754264,1.,-3.26077002641879));
#55948=CARTESIAN_POINT('Ctrl Pts',(-2.1463680529566,-1.,-3.26564388189759));
#55949=CARTESIAN_POINT('Ctrl Pts',(-2.1463680529566,1.,-3.26564388189759));
#55950=CARTESIAN_POINT('Ctrl Pts',(-2.15205043199808,-1.,-3.27050245897228));
#55951=CARTESIAN_POINT('Ctrl Pts',(-2.15205043199808,1.,-3.27050245897228));
#55952=CARTESIAN_POINT('Ctrl Pts',(-2.15778690038347,-1.,-3.27534954469187));
#55953=CARTESIAN_POINT('Ctrl Pts',(-2.15778690038347,1.,-3.27534954469187));
#55954=CARTESIAN_POINT('Ctrl Pts',(-2.16357391934425,-1.,-3.280181508414));
#55955=CARTESIAN_POINT('Ctrl Pts',(-2.16357391934425,1.,-3.280181508414));
#55956=CARTESIAN_POINT('Ctrl Pts',(-2.16940517773455,-1.,-3.28499019979724));
#55957=CARTESIAN_POINT('Ctrl Pts',(-2.16940517773455,1.,-3.28499019979724));
#55958=CARTESIAN_POINT('Ctrl Pts',(-2.17527380048423,-1.,-3.28976645712568));
#55959=CARTESIAN_POINT('Ctrl Pts',(-2.17527380048423,1.,-3.28976645712568));
#55960=CARTESIAN_POINT('Ctrl Pts',(-2.18117455557065,-1.,-3.2945036150049));
#55961=CARTESIAN_POINT('Ctrl Pts',(-2.18117455557065,1.,-3.2945036150049));
#55962=CARTESIAN_POINT('Ctrl Pts',(-2.18710556500327,-1.,-3.29920022557639));
#55963=CARTESIAN_POINT('Ctrl Pts',(-2.18710556500327,1.,-3.29920022557639));
#55964=CARTESIAN_POINT('Ctrl Pts',(-2.19306710376111,-1.,-3.30385816281831));
#55965=CARTESIAN_POINT('Ctrl Pts',(-2.19306710376111,1.,-3.30385816281831));
#55966=CARTESIAN_POINT('Ctrl Pts',(-2.19906078949923,-1.,-3.30848134694595));
#55967=CARTESIAN_POINT('Ctrl Pts',(-2.19906078949923,1.,-3.30848134694595));
#55968=CARTESIAN_POINT('Ctrl Pts',(-2.20508863150607,-1.,-3.31307424608949));
#55969=CARTESIAN_POINT('Ctrl Pts',(-2.20508863150607,1.,-3.31307424608949));
#55970=CARTESIAN_POINT('Ctrl Pts',(-2.21115211847875,-1.,-3.31764044024235));
#55971=CARTESIAN_POINT('Ctrl Pts',(-2.21115211847875,1.,-3.31764044024235));
#55972=CARTESIAN_POINT('Ctrl Pts',(-2.21725135110898,-1.,-3.32218125618968));
#55973=CARTESIAN_POINT('Ctrl Pts',(-2.21725135110898,1.,-3.32218125618968));
#55974=CARTESIAN_POINT('Ctrl Pts',(-2.22338548312772,-1.,-3.3266964672289));
#55975=CARTESIAN_POINT('Ctrl Pts',(-2.22338548312772,1.,-3.3266964672289));
#55976=CARTESIAN_POINT('Ctrl Pts',(-2.22955308907233,-1.,-3.33118487773611));
#55977=CARTESIAN_POINT('Ctrl Pts',(-2.22955308907233,1.,-3.33118487773611));
#55978=CARTESIAN_POINT('Ctrl Pts',(-2.23575256328812,-1.,-3.33564495756482));
#55979=CARTESIAN_POINT('Ctrl Pts',(-2.23575256328812,1.,-3.33564495756482));
#55980=CARTESIAN_POINT('Ctrl Pts',(-2.24198249391422,-1.,-3.34007543738025));
#55981=CARTESIAN_POINT('Ctrl Pts',(-2.24198249391422,1.,-3.34007543738025));
#55982=CARTESIAN_POINT('Ctrl Pts',(-2.24824207678256,-1.,-3.34447596770723));
#55983=CARTESIAN_POINT('Ctrl Pts',(-2.24824207678256,1.,-3.34447596770723));
#55984=CARTESIAN_POINT('Ctrl Pts',(-2.25453097693483,-1.,-3.34884690292285));
#55985=CARTESIAN_POINT('Ctrl Pts',(-2.25453097693483,1.,-3.34884690292285));
#55986=CARTESIAN_POINT('Ctrl Pts',(-2.26084915222449,-1.,-3.35318902552626));
#55987=CARTESIAN_POINT('Ctrl Pts',(-2.26084915222449,1.,-3.35318902552626));
#55988=CARTESIAN_POINT('Ctrl Pts',(-2.2671966857991,-1.,-3.35750328523061));
#55989=CARTESIAN_POINT('Ctrl Pts',(-2.2671966857991,1.,-3.35750328523061));
#55990=CARTESIAN_POINT('Ctrl Pts',(-2.2735736262093,-1.,-3.36179055004409));
#55991=CARTESIAN_POINT('Ctrl Pts',(-2.2735736262093,1.,-3.36179055004409));
#55992=CARTESIAN_POINT('Ctrl Pts',(-2.27997979458037,-1.,-3.36605130713076));
#55993=CARTESIAN_POINT('Ctrl Pts',(-2.27997979458037,1.,-3.36605130713076));
#55994=CARTESIAN_POINT('Ctrl Pts',(-2.28641481081137,-1.,-3.37028570206488));
#55995=CARTESIAN_POINT('Ctrl Pts',(-2.28641481081137,1.,-3.37028570206488));
#55996=CARTESIAN_POINT('Ctrl Pts',(-2.29287818007393,-1.,-3.37449367172826));
#55997=CARTESIAN_POINT('Ctrl Pts',(-2.29287818007393,1.,-3.37449367172826));
#55998=CARTESIAN_POINT('Ctrl Pts',(-2.29936936127624,-1.,-3.37867504959433));
#55999=CARTESIAN_POINT('Ctrl Pts',(-2.29936936127624,1.,-3.37867504959433));
#56000=CARTESIAN_POINT('Ctrl Pts',(-2.30588783640343,-1.,-3.3828296733661));
#56001=CARTESIAN_POINT('Ctrl Pts',(-2.30588783640343,1.,-3.3828296733661));
#56002=CARTESIAN_POINT('Ctrl Pts',(-2.31243319489367,-1.,-3.38695751492462));
#56003=CARTESIAN_POINT('Ctrl Pts',(-2.31243319489367,1.,-3.38695751492462));
#56004=CARTESIAN_POINT('Ctrl Pts',(-2.31900513925424,-1.,-3.39105869474822));
#56005=CARTESIAN_POINT('Ctrl Pts',(-2.31900513925424,1.,-3.39105869474822));
#56006=CARTESIAN_POINT('Ctrl Pts',(-2.3256034390248,-1.,-3.39513342019756));
#56007=CARTESIAN_POINT('Ctrl Pts',(-2.3256034390248,1.,-3.39513342019756));
#56008=CARTESIAN_POINT('Ctrl Pts',(-2.33222789882489,-1.,-3.39918194577956));
#56009=CARTESIAN_POINT('Ctrl Pts',(-2.33222789882489,1.,-3.39918194577956));
#56010=CARTESIAN_POINT('Ctrl Pts',(-2.33887832342782,-1.,-3.40320452776743));
#56011=CARTESIAN_POINT('Ctrl Pts',(-2.33887832342782,1.,-3.40320452776743));
#56012=CARTESIAN_POINT('Ctrl Pts',(-2.34555447649188,-1.,-3.40720137404297));
#56013=CARTESIAN_POINT('Ctrl Pts',(-2.34555447649188,1.,-3.40720137404297));
#56014=CARTESIAN_POINT('Ctrl Pts',(-2.35225606824109,-1.,-3.41117262314119));
#56015=CARTESIAN_POINT('Ctrl Pts',(-2.35225606824109,1.,-3.41117262314119));
#56016=CARTESIAN_POINT('Ctrl Pts',(-2.35898278606946,-1.,-3.41511836751469));
#56017=CARTESIAN_POINT('Ctrl Pts',(-2.35898278606946,1.,-3.41511836751469));
#56018=CARTESIAN_POINT('Ctrl Pts',(-2.36573431470642,-1.,-3.41903866635852));
#56019=CARTESIAN_POINT('Ctrl Pts',(-2.36573431470642,1.,-3.41903866635852));
#56020=CARTESIAN_POINT('Ctrl Pts',(-2.37251035954292,-1.,-3.42293356216511));
#56021=CARTESIAN_POINT('Ctrl Pts',(-2.37251035954292,1.,-3.42293356216511));
#56022=CARTESIAN_POINT('Ctrl Pts',(-2.37931067028926,-1.,-3.42680309754399));
#56023=CARTESIAN_POINT('Ctrl Pts',(-2.37931067028926,1.,-3.42680309754399));
#56024=CARTESIAN_POINT('Ctrl Pts',(-2.38613505843552,-1.,-3.4306473271292));
#56025=CARTESIAN_POINT('Ctrl Pts',(-2.38613505843552,1.,-3.4306473271292));
#56026=CARTESIAN_POINT('Ctrl Pts',(-2.39298338804493,-1.,-3.4344663067854));
#56027=CARTESIAN_POINT('Ctrl Pts',(-2.39298338804493,1.,-3.4344663067854));
#56028=CARTESIAN_POINT('Ctrl Pts',(-2.39848113410292,-1.,-3.43750133064416));
#56029=CARTESIAN_POINT('Ctrl Pts',(-2.39848113410292,1.,-3.43750133064416));
#56030=CARTESIAN_POINT('Ctrl Pts',(-2.40261515589405,-1.,-3.43976627484234));
#56031=CARTESIAN_POINT('Ctrl Pts',(-2.40261515589405,1.,-3.43976627484234));
#56032=CARTESIAN_POINT('Ctrl Pts',(-2.4053759295909,-1.,-3.44127120683039));
#56033=CARTESIAN_POINT('Ctrl Pts',(-2.4053759295909,1.,-3.44127120683039));
#56034=CARTESIAN_POINT('Ctrl Pts',(-2.40675750623143,-1.,-3.44202241512147));
#56035=CARTESIAN_POINT('Ctrl Pts',(-2.40675750623143,1.,-3.44202241512147));
#56036=CARTESIAN_POINT('',(-2.03660101169714,1.,-3.14877060440328));
#56037=CARTESIAN_POINT('Ctrl Pts',(-2.03660101169715,-1.,-3.14877060440327));
#56038=CARTESIAN_POINT('Ctrl Pts',(-2.03660101169715,-0.666666666666667,
-3.14877060440327));
#56039=CARTESIAN_POINT('Ctrl Pts',(-2.03660101169715,-0.333333333333333,
-3.14877060440327));
#56040=CARTESIAN_POINT('Ctrl Pts',(-2.03660101169715,0.333333333333333,
-3.14877060440327));
#56041=CARTESIAN_POINT('Ctrl Pts',(-2.03660101169715,0.666666666666667,
-3.14877060440327));
#56042=CARTESIAN_POINT('Ctrl Pts',(-2.03660101169715,1.,-3.14877060440327));
#56043=CARTESIAN_POINT('',(-2.40675750623143,1.,-3.44202241512147));
#56044=CARTESIAN_POINT('',(-2.40675750623143,0.,-3.44202241512147));
#56045=CARTESIAN_POINT('Ctrl Pts',(-2.03660101169715,1.,-3.14877060440328));
#56046=CARTESIAN_POINT('Ctrl Pts',(-2.03659701539259,1.,-3.14881939088124));
#56047=CARTESIAN_POINT('Ctrl Pts',(-2.03663974554932,1.,-3.1490119366901));
#56048=CARTESIAN_POINT('Ctrl Pts',(-2.03693188810545,1.,-3.14959882629805));
#56049=CARTESIAN_POINT('Ctrl Pts',(-2.03783225495961,1.,-3.15102344775328));
#56050=CARTESIAN_POINT('Ctrl Pts',(-2.03984073791519,1.,-3.15389991674792));
#56051=CARTESIAN_POINT('Ctrl Pts',(-2.04297406404027,1.,-3.15817983946367));
#56052=CARTESIAN_POINT('Ctrl Pts',(-2.04693331247446,1.,-3.16343165058912));
#56053=CARTESIAN_POINT('Ctrl Pts',(-2.05151770247233,1.,-3.16936341689527));
#56054=CARTESIAN_POINT('Ctrl Pts',(-2.05650186773132,1.,-3.17564906975371));
#56055=CARTESIAN_POINT('Ctrl Pts',(-2.06166849827101,1.,-3.18197692964614));
#56056=CARTESIAN_POINT('Ctrl Pts',(-2.06684062744112,1.,-3.18809755562368));
#56057=CARTESIAN_POINT('Ctrl Pts',(-2.07192253497857,1.,-3.19388465568252));
#56058=CARTESIAN_POINT('Ctrl Pts',(-2.07690441870722,1.,-3.19934132836019));
#56059=CARTESIAN_POINT('Ctrl Pts',(-2.08182850370878,1.,-3.2045481863073));
#56060=CARTESIAN_POINT('Ctrl Pts',(-2.08676465517455,1.,-3.20962575845463));
#56061=CARTESIAN_POINT('Ctrl Pts',(-2.09178419460443,1.,-3.21469429601654));
#56062=CARTESIAN_POINT('Ctrl Pts',(-2.09692958434895,1.,-3.21982707347009));
#56063=CARTESIAN_POINT('Ctrl Pts',(-2.10220384298492,1.,-3.22503437553434));
#56064=CARTESIAN_POINT('Ctrl Pts',(-2.10758699642451,1.,-3.23028945793289));
#56065=CARTESIAN_POINT('Ctrl Pts',(-2.11304604021773,1.,-3.23554444767099));
#56066=CARTESIAN_POINT('Ctrl Pts',(-2.11854673326979,1.,-3.24074905517293));
#56067=CARTESIAN_POINT('Ctrl Pts',(-2.12406646410962,1.,-3.24587102613376));
#56068=CARTESIAN_POINT('Ctrl Pts',(-2.12960028396832,1.,-3.25090574494028));
#56069=CARTESIAN_POINT('Ctrl Pts',(-2.13515375878803,1.,-3.25586495065054));
#56070=CARTESIAN_POINT('Ctrl Pts',(-2.14073870754264,1.,-3.26077002641879));
#56071=CARTESIAN_POINT('Ctrl Pts',(-2.1463680529566,1.,-3.26564388189759));
#56072=CARTESIAN_POINT('Ctrl Pts',(-2.15205043199808,1.,-3.27050245897228));
#56073=CARTESIAN_POINT('Ctrl Pts',(-2.15778690038347,1.,-3.27534954469187));
#56074=CARTESIAN_POINT('Ctrl Pts',(-2.16357391934425,1.,-3.280181508414));
#56075=CARTESIAN_POINT('Ctrl Pts',(-2.16940517773455,1.,-3.28499019979724));
#56076=CARTESIAN_POINT('Ctrl Pts',(-2.17527380048423,1.,-3.28976645712568));
#56077=CARTESIAN_POINT('Ctrl Pts',(-2.18117455557065,1.,-3.2945036150049));
#56078=CARTESIAN_POINT('Ctrl Pts',(-2.18710556500327,1.,-3.29920022557639));
#56079=CARTESIAN_POINT('Ctrl Pts',(-2.19306710376111,1.,-3.30385816281831));
#56080=CARTESIAN_POINT('Ctrl Pts',(-2.19906078949923,1.,-3.30848134694595));
#56081=CARTESIAN_POINT('Ctrl Pts',(-2.20508863150607,1.,-3.31307424608949));
#56082=CARTESIAN_POINT('Ctrl Pts',(-2.21115211847875,1.,-3.31764044024235));
#56083=CARTESIAN_POINT('Ctrl Pts',(-2.21725135110898,1.,-3.32218125618968));
#56084=CARTESIAN_POINT('Ctrl Pts',(-2.22338548312772,1.,-3.3266964672289));
#56085=CARTESIAN_POINT('Ctrl Pts',(-2.22955308907233,1.,-3.33118487773611));
#56086=CARTESIAN_POINT('Ctrl Pts',(-2.23575256328812,1.,-3.33564495756482));
#56087=CARTESIAN_POINT('Ctrl Pts',(-2.24198249391422,1.,-3.34007543738025));
#56088=CARTESIAN_POINT('Ctrl Pts',(-2.24824207678256,1.,-3.34447596770723));
#56089=CARTESIAN_POINT('Ctrl Pts',(-2.25453097693483,1.,-3.34884690292285));
#56090=CARTESIAN_POINT('Ctrl Pts',(-2.26084915222449,1.,-3.35318902552626));
#56091=CARTESIAN_POINT('Ctrl Pts',(-2.2671966857991,1.,-3.35750328523061));
#56092=CARTESIAN_POINT('Ctrl Pts',(-2.2735736262093,1.,-3.36179055004409));
#56093=CARTESIAN_POINT('Ctrl Pts',(-2.27997979458037,1.,-3.36605130713076));
#56094=CARTESIAN_POINT('Ctrl Pts',(-2.28641481081137,1.,-3.37028570206488));
#56095=CARTESIAN_POINT('Ctrl Pts',(-2.29287818007393,1.,-3.37449367172826));
#56096=CARTESIAN_POINT('Ctrl Pts',(-2.29936936127624,1.,-3.37867504959433));
#56097=CARTESIAN_POINT('Ctrl Pts',(-2.30588783640343,1.,-3.3828296733661));
#56098=CARTESIAN_POINT('Ctrl Pts',(-2.31243319489367,1.,-3.38695751492462));
#56099=CARTESIAN_POINT('Ctrl Pts',(-2.31900513925424,1.,-3.39105869474822));
#56100=CARTESIAN_POINT('Ctrl Pts',(-2.3256034390248,1.,-3.39513342019756));
#56101=CARTESIAN_POINT('Ctrl Pts',(-2.33222789882489,1.,-3.39918194577956));
#56102=CARTESIAN_POINT('Ctrl Pts',(-2.33887832342782,1.,-3.40320452776743));
#56103=CARTESIAN_POINT('Ctrl Pts',(-2.34555447649188,1.,-3.40720137404297));
#56104=CARTESIAN_POINT('Ctrl Pts',(-2.35225606824109,1.,-3.41117262314119));
#56105=CARTESIAN_POINT('Ctrl Pts',(-2.35898278606946,1.,-3.41511836751469));
#56106=CARTESIAN_POINT('Ctrl Pts',(-2.36573431470642,1.,-3.41903866635852));
#56107=CARTESIAN_POINT('Ctrl Pts',(-2.37251035954292,1.,-3.42293356216511));
#56108=CARTESIAN_POINT('Ctrl Pts',(-2.37931067028926,1.,-3.42680309754399));
#56109=CARTESIAN_POINT('Ctrl Pts',(-2.38613505843552,1.,-3.4306473271292));
#56110=CARTESIAN_POINT('Ctrl Pts',(-2.39298338804493,1.,-3.4344663067854));
#56111=CARTESIAN_POINT('Ctrl Pts',(-2.39848113410292,1.,-3.43750133064416));
#56112=CARTESIAN_POINT('Ctrl Pts',(-2.40261515589405,1.,-3.43976627484234));
#56113=CARTESIAN_POINT('Ctrl Pts',(-2.4053759295909,1.,-3.44127120683039));
#56114=CARTESIAN_POINT('Ctrl Pts',(-2.40675750623143,1.,-3.44202241512147));
#56115=CARTESIAN_POINT('Origin',(-2.40675750623143,0.,-3.44202241512147));
#56116=CARTESIAN_POINT('',(-2.52982887637028,1.,-3.35260583073571));
#56117=CARTESIAN_POINT('Origin',(0.,0.,0.));
#56118=CARTESIAN_POINT('',(-1.88097764062697,1.,-3.24413672884812));
#56119=CARTESIAN_POINT('Origin',(0.,1.,0.));
#56120=CARTESIAN_POINT('Ctrl Pts',(-1.88097764062697,1.,-3.24413672884812));
#56121=CARTESIAN_POINT('Ctrl Pts',(-1.88097764062697,0.666666666666667,
-3.24413672884812));
#56122=CARTESIAN_POINT('Ctrl Pts',(-1.88097764062697,0.333333333333333,
-3.24413672884812));
#56123=CARTESIAN_POINT('Ctrl Pts',(-1.88097764062697,-0.333333333333333,
-3.24413672884812));
#56124=CARTESIAN_POINT('Ctrl Pts',(-1.88097764062697,-0.666666666666667,
-3.24413672884812));
#56125=CARTESIAN_POINT('Ctrl Pts',(-1.88097764062697,-1.,-3.24413672884812));
#56126=CARTESIAN_POINT('Ctrl Pts',(-1.97421938526992,-1.,-3.70708211654725));
#56127=CARTESIAN_POINT('Ctrl Pts',(-1.97421938526992,1.,-3.70708211654725));
#56128=CARTESIAN_POINT('Ctrl Pts',(-1.97417727645308,-1.,-3.70551008132332));
#56129=CARTESIAN_POINT('Ctrl Pts',(-1.97417727645308,1.,-3.70551008132332));
#56130=CARTESIAN_POINT('Ctrl Pts',(-1.97408973726715,-1.,-3.70236698912904));
#56131=CARTESIAN_POINT('Ctrl Pts',(-1.97408973726715,1.,-3.70236698912904));
#56132=CARTESIAN_POINT('Ctrl Pts',(-1.97394846383216,-1.,-3.6976552856004));
#56133=CARTESIAN_POINT('Ctrl Pts',(-1.97394846383216,1.,-3.6976552856004));
#56134=CARTESIAN_POINT('Ctrl Pts',(-1.97374016225483,-1.,-3.69137888599902));
#56135=CARTESIAN_POINT('Ctrl Pts',(-1.97374016225483,1.,-3.69137888599902));
#56136=CARTESIAN_POINT('Ctrl Pts',(-1.97344650304519,-1.,-3.68354319915092));
#56137=CARTESIAN_POINT('Ctrl Pts',(-1.97344650304519,1.,-3.68354319915092));
#56138=CARTESIAN_POINT('Ctrl Pts',(-1.97311947678517,-1.,-3.67571738107084));
#56139=CARTESIAN_POINT('Ctrl Pts',(-1.97311947678517,1.,-3.67571738107084));
#56140=CARTESIAN_POINT('Ctrl Pts',(-1.97275897198678,-1.,-3.66790152752075));
#56141=CARTESIAN_POINT('Ctrl Pts',(-1.97275897198678,1.,-3.66790152752075));
#56142=CARTESIAN_POINT('Ctrl Pts',(-1.9723648543905,-1.,-3.6600957816636));
#56143=CARTESIAN_POINT('Ctrl Pts',(-1.9723648543905,1.,-3.6600957816636));
#56144=CARTESIAN_POINT('Ctrl Pts',(-1.9719369724024,-1.,-3.652300347166));
#56145=CARTESIAN_POINT('Ctrl Pts',(-1.9719369724024,1.,-3.652300347166));
#56146=CARTESIAN_POINT('Ctrl Pts',(-1.97147515441164,-1.,-3.64451546723514));
#56147=CARTESIAN_POINT('Ctrl Pts',(-1.97147515441164,1.,-3.64451546723514));
#56148=CARTESIAN_POINT('Ctrl Pts',(-1.97097920454464,-1.,-3.63674139590412));
#56149=CARTESIAN_POINT('Ctrl Pts',(-1.97097920454464,1.,-3.63674139590412));
#56150=CARTESIAN_POINT('Ctrl Pts',(-1.97044889850463,-1.,-3.62897836973293));
#56151=CARTESIAN_POINT('Ctrl Pts',(-1.97044889850463,1.,-3.62897836973293));
#56152=CARTESIAN_POINT('Ctrl Pts',(-1.96988398129978,-1.,-3.62122658401893));
#56153=CARTESIAN_POINT('Ctrl Pts',(-1.96988398129978,1.,-3.62122658401893));
#56154=CARTESIAN_POINT('Ctrl Pts',(-1.96928416040877,-1.,-3.61348615496704));
#56155=CARTESIAN_POINT('Ctrl Pts',(-1.96928416040877,1.,-3.61348615496704));
#56156=CARTESIAN_POINT('Ctrl Pts',(-1.9686491188594,-1.,-3.60575714017989));
#56157=CARTESIAN_POINT('Ctrl Pts',(-1.9686491188594,1.,-3.60575714017989));
#56158=CARTESIAN_POINT('Ctrl Pts',(-1.96797854118369,-1.,-3.59803959819938));
#56159=CARTESIAN_POINT('Ctrl Pts',(-1.96797854118369,1.,-3.59803959819938));
#56160=CARTESIAN_POINT('Ctrl Pts',(-1.96727213799544,-1.,-3.59033364022801));
#56161=CARTESIAN_POINT('Ctrl Pts',(-1.96727213799544,1.,-3.59033364022801));
#56162=CARTESIAN_POINT('Ctrl Pts',(-1.96652966688911,-1.,-3.58263947663829));
#56163=CARTESIAN_POINT('Ctrl Pts',(-1.96652966688911,1.,-3.58263947663829));
#56164=CARTESIAN_POINT('Ctrl Pts',(-1.96575096652789,-1.,-3.57495748600959));
#56165=CARTESIAN_POINT('Ctrl Pts',(-1.96575096652789,1.,-3.57495748600959));
#56166=CARTESIAN_POINT('Ctrl Pts',(-1.96493594634567,-1.,-3.56728820357791));
#56167=CARTESIAN_POINT('Ctrl Pts',(-1.96493594634567,1.,-3.56728820357791));
#56168=CARTESIAN_POINT('Ctrl Pts',(-1.96408450906812,-1.,-3.55963218706096));
#56169=CARTESIAN_POINT('Ctrl Pts',(-1.96408450906812,1.,-3.55963218706096));
#56170=CARTESIAN_POINT('Ctrl Pts',(-1.96319648628644,-1.,-3.55198990600886));
#56171=CARTESIAN_POINT('Ctrl Pts',(-1.96319648628644,1.,-3.55198990600886));
#56172=CARTESIAN_POINT('Ctrl Pts',(-1.96227157573067,-1.,-3.54436163300443));
#56173=CARTESIAN_POINT('Ctrl Pts',(-1.96227157573067,1.,-3.54436163300443));
#56174=CARTESIAN_POINT('Ctrl Pts',(-1.96130926212689,-1.,-3.53674730625813));
#56175=CARTESIAN_POINT('Ctrl Pts',(-1.96130926212689,1.,-3.53674730625813));
#56176=CARTESIAN_POINT('Ctrl Pts',(-1.96030879411566,-1.,-3.52914648844351));
#56177=CARTESIAN_POINT('Ctrl Pts',(-1.96030879411566,1.,-3.52914648844351));
#56178=CARTESIAN_POINT('Ctrl Pts',(-1.95926936324461,-1.,-3.52155867431486));
#56179=CARTESIAN_POINT('Ctrl Pts',(-1.95926936324461,1.,-3.52155867431486));
#56180=CARTESIAN_POINT('Ctrl Pts',(-1.95819025316779,-1.,-3.51398354617794));
#56181=CARTESIAN_POINT('Ctrl Pts',(-1.95819025316779,1.,-3.51398354617794));
#56182=CARTESIAN_POINT('Ctrl Pts',(-1.95707099606511,-1.,-3.50642124159909));
#56183=CARTESIAN_POINT('Ctrl Pts',(-1.95707099606511,1.,-3.50642124159909));
#56184=CARTESIAN_POINT('Ctrl Pts',(-1.95591153823661,-1.,-3.49887263575583));
#56185=CARTESIAN_POINT('Ctrl Pts',(-1.95591153823661,1.,-3.49887263575583));
#56186=CARTESIAN_POINT('Ctrl Pts',(-1.95471236969643,-1.,-3.49133956289133));
#56187=CARTESIAN_POINT('Ctrl Pts',(-1.95471236969643,1.,-3.49133956289133));
#56188=CARTESIAN_POINT('Ctrl Pts',(-1.95347412486309,-1.,-3.48382414832634));
#56189=CARTESIAN_POINT('Ctrl Pts',(-1.95347412486309,1.,-3.48382414832634));
#56190=CARTESIAN_POINT('Ctrl Pts',(-1.95219722189876,-1.,-3.47632820495921));
#56191=CARTESIAN_POINT('Ctrl Pts',(-1.95219722189876,1.,-3.47632820495921));
#56192=CARTESIAN_POINT('Ctrl Pts',(-1.95088147859877,-1.,-3.46885258974191));
#56193=CARTESIAN_POINT('Ctrl Pts',(-1.95088147859877,1.,-3.46885258974191));
#56194=CARTESIAN_POINT('Ctrl Pts',(-1.94952575850197,-1.,-3.46139661060962));
#56195=CARTESIAN_POINT('Ctrl Pts',(-1.94952575850197,1.,-3.46139661060962));
#56196=CARTESIAN_POINT('Ctrl Pts',(-1.94812754766524,-1.,-3.45395731584051));
#56197=CARTESIAN_POINT('Ctrl Pts',(-1.94812754766524,1.,-3.45395731584051));
#56198=CARTESIAN_POINT('Ctrl Pts',(-1.94668377715329,-1.,-3.44653088665681));
#56199=CARTESIAN_POINT('Ctrl Pts',(-1.94668377715329,1.,-3.44653088665681));
#56200=CARTESIAN_POINT('Ctrl Pts',(-1.94519168842879,-1.,-3.43911410197687));
#56201=CARTESIAN_POINT('Ctrl Pts',(-1.94519168842879,1.,-3.43911410197687));
#56202=CARTESIAN_POINT('Ctrl Pts',(-1.94364973660284,-1.,-3.43170586602434));
#56203=CARTESIAN_POINT('Ctrl Pts',(-1.94364973660284,1.,-3.43170586602434));
#56204=CARTESIAN_POINT('Ctrl Pts',(-1.94205835913696,-1.,-3.42430850941503));
#56205=CARTESIAN_POINT('Ctrl Pts',(-1.94205835913696,1.,-3.42430850941503));
#56206=CARTESIAN_POINT('Ctrl Pts',(-1.94042111965246,-1.,-3.41692971994096));
#56207=CARTESIAN_POINT('Ctrl Pts',(-1.94042111965246,1.,-3.41692971994096));
#56208=CARTESIAN_POINT('Ctrl Pts',(-1.93874306008143,-1.,-3.40957978266642));
#56209=CARTESIAN_POINT('Ctrl Pts',(-1.93874306008143,1.,-3.40957978266642));
#56210=CARTESIAN_POINT('Ctrl Pts',(-1.93702857723098,-1.,-3.40226802104109));
#56211=CARTESIAN_POINT('Ctrl Pts',(-1.93702857723098,1.,-3.40226802104109));
#56212=CARTESIAN_POINT('Ctrl Pts',(-1.93527929945985,-1.,-3.39499923640795));
#56213=CARTESIAN_POINT('Ctrl Pts',(-1.93527929945985,1.,-3.39499923640795));
#56214=CARTESIAN_POINT('Ctrl Pts',(-1.93349233176788,-1.,-3.38777076883256));
#56215=CARTESIAN_POINT('Ctrl Pts',(-1.93349233176788,1.,-3.38777076883256));
#56216=CARTESIAN_POINT('Ctrl Pts',(-1.93165739093276,-1.,-3.3805676852555));
#56217=CARTESIAN_POINT('Ctrl Pts',(-1.93165739093276,1.,-3.3805676852555));
#56218=CARTESIAN_POINT('Ctrl Pts',(-1.92975993109877,-1.,-3.37336807068043));
#56219=CARTESIAN_POINT('Ctrl Pts',(-1.92975993109877,1.,-3.37336807068043));
#56220=CARTESIAN_POINT('Ctrl Pts',(-1.92778626543786,-1.,-3.36615168657567));
#56221=CARTESIAN_POINT('Ctrl Pts',(-1.92778626543786,1.,-3.36615168657567));
#56222=CARTESIAN_POINT('Ctrl Pts',(-1.92572846125756,-1.,-3.35890824422965));
#56223=CARTESIAN_POINT('Ctrl Pts',(-1.92572846125756,1.,-3.35890824422965));
#56224=CARTESIAN_POINT('Ctrl Pts',(-1.92358838440528,-1.,-3.35164424847223));
#56225=CARTESIAN_POINT('Ctrl Pts',(-1.92358838440528,1.,-3.35164424847223));
#56226=CARTESIAN_POINT('Ctrl Pts',(-1.92138450828404,-1.,-3.34439448941961));
#56227=CARTESIAN_POINT('Ctrl Pts',(-1.92138450828404,1.,-3.34439448941961));
#56228=CARTESIAN_POINT('Ctrl Pts',(-1.9191460961021,-1.,-3.33721230710012));
#56229=CARTESIAN_POINT('Ctrl Pts',(-1.9191460961021,1.,-3.33721230710012));
#56230=CARTESIAN_POINT('Ctrl Pts',(-1.91690081930331,-1.,-3.33014884257873));
#56231=CARTESIAN_POINT('Ctrl Pts',(-1.91690081930331,1.,-3.33014884257873));
#56232=CARTESIAN_POINT('Ctrl Pts',(-1.91466343916628,-1.,-3.32323403454535));
#56233=CARTESIAN_POINT('Ctrl Pts',(-1.91466343916628,1.,-3.32323403454535));
#56234=CARTESIAN_POINT('Ctrl Pts',(-1.91242616234442,-1.,-3.31646052426364));
#56235=CARTESIAN_POINT('Ctrl Pts',(-1.91242616234442,1.,-3.31646052426364));
#56236=CARTESIAN_POINT('Ctrl Pts',(-1.91014297830446,-1.,-3.30975721158596));
#56237=CARTESIAN_POINT('Ctrl Pts',(-1.91014297830446,1.,-3.30975721158596));
#56238=CARTESIAN_POINT('Ctrl Pts',(-1.90773912171341,-1.,-3.30300595568195));
#56239=CARTESIAN_POINT('Ctrl Pts',(-1.90773912171341,1.,-3.30300595568195));
#56240=CARTESIAN_POINT('Ctrl Pts',(-1.90513891864087,-1.,-3.29608978722113));
#56241=CARTESIAN_POINT('Ctrl Pts',(-1.90513891864087,1.,-3.29608978722113));
#56242=CARTESIAN_POINT('Ctrl Pts',(-1.90228971247527,-1.,-3.2889344860029));
#56243=CARTESIAN_POINT('Ctrl Pts',(-1.90228971247527,1.,-3.2889344860029));
#56244=CARTESIAN_POINT('Ctrl Pts',(-1.89918429230462,-1.,-3.28154737912352));
#56245=CARTESIAN_POINT('Ctrl Pts',(-1.89918429230462,1.,-3.28154737912352));
#56246=CARTESIAN_POINT('Ctrl Pts',(-1.89589172903793,-1.,-3.27407108933139));
#56247=CARTESIAN_POINT('Ctrl Pts',(-1.89589172903793,1.,-3.27407108933139));
#56248=CARTESIAN_POINT('Ctrl Pts',(-1.89255393500965,-1.,-3.26677653888676));
#56249=CARTESIAN_POINT('Ctrl Pts',(-1.89255393500965,1.,-3.26677653888676));
#56250=CARTESIAN_POINT('Ctrl Pts',(-1.88934996203698,-1.,-3.25999885193947));
#56251=CARTESIAN_POINT('Ctrl Pts',(-1.88934996203698,1.,-3.25999885193947));
#56252=CARTESIAN_POINT('Ctrl Pts',(-1.88646802523466,-1.,-3.25408686339463));
#56253=CARTESIAN_POINT('Ctrl Pts',(-1.88646802523466,1.,-3.25408686339463));
#56254=CARTESIAN_POINT('Ctrl Pts',(-1.88407708646357,-1.,-3.24935200511918));
#56255=CARTESIAN_POINT('Ctrl Pts',(-1.88407708646357,1.,-3.24935200511918));
#56256=CARTESIAN_POINT('Ctrl Pts',(-1.88229202582941,-1.,-3.24600543790443));
#56257=CARTESIAN_POINT('Ctrl Pts',(-1.88229202582941,1.,-3.24600543790443));
#56258=CARTESIAN_POINT('Ctrl Pts',(-1.88139187908074,-1.,-3.24451807186481));
#56259=CARTESIAN_POINT('Ctrl Pts',(-1.88139187908074,1.,-3.24451807186481));
#56260=CARTESIAN_POINT('Ctrl Pts',(-1.88102201872555,-1.,-3.24408699284121));
#56261=CARTESIAN_POINT('Ctrl Pts',(-1.88102201872555,1.,-3.24408699284121));
#56262=CARTESIAN_POINT('Ctrl Pts',(-1.88091100680349,-1.,-3.24410359189609));
#56263=CARTESIAN_POINT('Ctrl Pts',(-1.88091100680349,1.,-3.24410359189609));
#56264=CARTESIAN_POINT('Ctrl Pts',(-1.8808893942881,-1.,-3.24418789321065));
#56265=CARTESIAN_POINT('Ctrl Pts',(-1.8808893942881,1.,-3.24418789321065));
#56266=CARTESIAN_POINT('',(-1.97421938526992,1.,-3.70708211654725));
#56267=CARTESIAN_POINT('Ctrl Pts',(-1.97421938526992,1.,-3.70708211654725));
#56268=CARTESIAN_POINT('Ctrl Pts',(-1.97417727645308,1.,-3.70551008132332));
#56269=CARTESIAN_POINT('Ctrl Pts',(-1.97408973726715,1.,-3.70236698912904));
#56270=CARTESIAN_POINT('Ctrl Pts',(-1.97394846383216,1.,-3.6976552856004));
#56271=CARTESIAN_POINT('Ctrl Pts',(-1.97374016225483,1.,-3.69137888599902));
#56272=CARTESIAN_POINT('Ctrl Pts',(-1.97344650304519,1.,-3.68354319915092));
#56273=CARTESIAN_POINT('Ctrl Pts',(-1.97311947678517,1.,-3.67571738107084));
#56274=CARTESIAN_POINT('Ctrl Pts',(-1.97275897198678,1.,-3.66790152752075));
#56275=CARTESIAN_POINT('Ctrl Pts',(-1.9723648543905,1.,-3.6600957816636));
#56276=CARTESIAN_POINT('Ctrl Pts',(-1.9719369724024,1.,-3.652300347166));
#56277=CARTESIAN_POINT('Ctrl Pts',(-1.97147515441164,1.,-3.64451546723514));
#56278=CARTESIAN_POINT('Ctrl Pts',(-1.97097920454464,1.,-3.63674139590412));
#56279=CARTESIAN_POINT('Ctrl Pts',(-1.97044889850463,1.,-3.62897836973293));
#56280=CARTESIAN_POINT('Ctrl Pts',(-1.96988398129978,1.,-3.62122658401893));
#56281=CARTESIAN_POINT('Ctrl Pts',(-1.96928416040877,1.,-3.61348615496704));
#56282=CARTESIAN_POINT('Ctrl Pts',(-1.9686491188594,1.,-3.60575714017989));
#56283=CARTESIAN_POINT('Ctrl Pts',(-1.96797854118369,1.,-3.59803959819938));
#56284=CARTESIAN_POINT('Ctrl Pts',(-1.96727213799544,1.,-3.59033364022801));
#56285=CARTESIAN_POINT('Ctrl Pts',(-1.96652966688911,1.,-3.58263947663829));
#56286=CARTESIAN_POINT('Ctrl Pts',(-1.96575096652789,1.,-3.57495748600959));
#56287=CARTESIAN_POINT('Ctrl Pts',(-1.96493594634567,1.,-3.56728820357791));
#56288=CARTESIAN_POINT('Ctrl Pts',(-1.96408450906812,1.,-3.55963218706096));
#56289=CARTESIAN_POINT('Ctrl Pts',(-1.96319648628644,1.,-3.55198990600886));
#56290=CARTESIAN_POINT('Ctrl Pts',(-1.96227157573067,1.,-3.54436163300443));
#56291=CARTESIAN_POINT('Ctrl Pts',(-1.96130926212689,1.,-3.53674730625813));
#56292=CARTESIAN_POINT('Ctrl Pts',(-1.96030879411566,1.,-3.52914648844351));
#56293=CARTESIAN_POINT('Ctrl Pts',(-1.95926936324461,1.,-3.52155867431486));
#56294=CARTESIAN_POINT('Ctrl Pts',(-1.95819025316779,1.,-3.51398354617794));
#56295=CARTESIAN_POINT('Ctrl Pts',(-1.95707099606511,1.,-3.50642124159909));
#56296=CARTESIAN_POINT('Ctrl Pts',(-1.95591153823661,1.,-3.49887263575583));
#56297=CARTESIAN_POINT('Ctrl Pts',(-1.95471236969643,1.,-3.49133956289133));
#56298=CARTESIAN_POINT('Ctrl Pts',(-1.95347412486309,1.,-3.48382414832634));
#56299=CARTESIAN_POINT('Ctrl Pts',(-1.95219722189876,1.,-3.47632820495921));
#56300=CARTESIAN_POINT('Ctrl Pts',(-1.95088147859877,1.,-3.46885258974191));
#56301=CARTESIAN_POINT('Ctrl Pts',(-1.94952575850197,1.,-3.46139661060962));
#56302=CARTESIAN_POINT('Ctrl Pts',(-1.94812754766524,1.,-3.45395731584051));
#56303=CARTESIAN_POINT('Ctrl Pts',(-1.94668377715329,1.,-3.44653088665681));
#56304=CARTESIAN_POINT('Ctrl Pts',(-1.94519168842879,1.,-3.43911410197687));
#56305=CARTESIAN_POINT('Ctrl Pts',(-1.94364973660284,1.,-3.43170586602434));
#56306=CARTESIAN_POINT('Ctrl Pts',(-1.94205835913696,1.,-3.42430850941503));
#56307=CARTESIAN_POINT('Ctrl Pts',(-1.94042111965246,1.,-3.41692971994096));
#56308=CARTESIAN_POINT('Ctrl Pts',(-1.93874306008143,1.,-3.40957978266642));
#56309=CARTESIAN_POINT('Ctrl Pts',(-1.93702857723098,1.,-3.40226802104109));
#56310=CARTESIAN_POINT('Ctrl Pts',(-1.93527929945985,1.,-3.39499923640795));
#56311=CARTESIAN_POINT('Ctrl Pts',(-1.93349233176788,1.,-3.38777076883256));
#56312=CARTESIAN_POINT('Ctrl Pts',(-1.93165739093276,1.,-3.3805676852555));
#56313=CARTESIAN_POINT('Ctrl Pts',(-1.92975993109877,1.,-3.37336807068043));
#56314=CARTESIAN_POINT('Ctrl Pts',(-1.92778626543786,1.,-3.36615168657567));
#56315=CARTESIAN_POINT('Ctrl Pts',(-1.92572846125756,1.,-3.35890824422965));
#56316=CARTESIAN_POINT('Ctrl Pts',(-1.92358838440528,1.,-3.35164424847223));
#56317=CARTESIAN_POINT('Ctrl Pts',(-1.92138450828404,1.,-3.34439448941961));
#56318=CARTESIAN_POINT('Ctrl Pts',(-1.9191460961021,1.,-3.33721230710012));
#56319=CARTESIAN_POINT('Ctrl Pts',(-1.91690081930331,1.,-3.33014884257873));
#56320=CARTESIAN_POINT('Ctrl Pts',(-1.91466343916628,1.,-3.32323403454535));
#56321=CARTESIAN_POINT('Ctrl Pts',(-1.91242616234442,1.,-3.31646052426364));
#56322=CARTESIAN_POINT('Ctrl Pts',(-1.91014297830446,1.,-3.30975721158596));
#56323=CARTESIAN_POINT('Ctrl Pts',(-1.90773912171341,1.,-3.30300595568195));
#56324=CARTESIAN_POINT('Ctrl Pts',(-1.90513891864087,1.,-3.29608978722113));
#56325=CARTESIAN_POINT('Ctrl Pts',(-1.90228971247527,1.,-3.2889344860029));
#56326=CARTESIAN_POINT('Ctrl Pts',(-1.89918429230462,1.,-3.28154737912352));
#56327=CARTESIAN_POINT('Ctrl Pts',(-1.89589172903793,1.,-3.27407108933139));
#56328=CARTESIAN_POINT('Ctrl Pts',(-1.89255393500965,1.,-3.26677653888676));
#56329=CARTESIAN_POINT('Ctrl Pts',(-1.88934996203698,1.,-3.25999885193947));
#56330=CARTESIAN_POINT('Ctrl Pts',(-1.88646802523466,1.,-3.25408686339463));
#56331=CARTESIAN_POINT('Ctrl Pts',(-1.88407708646357,1.,-3.24935200511918));
#56332=CARTESIAN_POINT('Ctrl Pts',(-1.88242596600454,1.,-3.2462565441079));
#56333=CARTESIAN_POINT('Ctrl Pts',(-1.88156537699203,1.,-3.24480754676064));
#56334=CARTESIAN_POINT('Ctrl Pts',(-1.88117508446775,1.,-3.24428080353022));
#56335=CARTESIAN_POINT('Ctrl Pts',(-1.8810229239812,1.,-3.24415531671284));
#56336=CARTESIAN_POINT('Ctrl Pts',(-1.88097764062697,1.,-3.24413672884812));
#56337=CARTESIAN_POINT('',(-1.97421938526992,0.,-3.70708211654725));
#56338=CARTESIAN_POINT('Ctrl Pts',(-1.519044091397,-1.,-3.42855728381368));
#56339=CARTESIAN_POINT('Ctrl Pts',(-1.519044091397,1.,-3.42855728381368));
#56340=CARTESIAN_POINT('Ctrl Pts',(-1.51896318668366,-1.,-3.42852521763778));
#56341=CARTESIAN_POINT('Ctrl Pts',(-1.51896318668366,1.,-3.42852521763778));
#56342=CARTESIAN_POINT('Ctrl Pts',(-1.51888450659652,-1.,-3.42860527149177));
#56343=CARTESIAN_POINT('Ctrl Pts',(-1.51888450659652,1.,-3.42860527149177));
#56344=CARTESIAN_POINT('Ctrl Pts',(-1.51901585839109,-1.,-3.42915787669893));
#56345=CARTESIAN_POINT('Ctrl Pts',(-1.51901585839109,1.,-3.42915787669893));
#56346=CARTESIAN_POINT('Ctrl Pts',(-1.51969006980999,-1.,-3.43076036253837));
#56347=CARTESIAN_POINT('Ctrl Pts',(-1.51969006980999,1.,-3.43076036253837));
#56348=CARTESIAN_POINT('Ctrl Pts',(-1.52134826724293,-1.,-3.43417156977893));
#56349=CARTESIAN_POINT('Ctrl Pts',(-1.52134826724293,1.,-3.43417156977893));
#56350=CARTESIAN_POINT('Ctrl Pts',(-1.5237734895035,-1.,-3.4388889597401));
#56351=CARTESIAN_POINT('Ctrl Pts',(-1.5237734895035,1.,-3.4388889597401));
#56352=CARTESIAN_POINT('Ctrl Pts',(-1.52686242875556,-1.,-3.44469547526647));
#56353=CARTESIAN_POINT('Ctrl Pts',(-1.52686242875556,1.,-3.44469547526647));
#56354=CARTESIAN_POINT('Ctrl Pts',(-1.53046244461635,-1.,-3.45127136828305));
#56355=CARTESIAN_POINT('Ctrl Pts',(-1.53046244461635,1.,-3.45127136828305));
#56356=CARTESIAN_POINT('Ctrl Pts',(-1.53440195378792,-1.,-3.45825932955032));
#56357=CARTESIAN_POINT('Ctrl Pts',(-1.53440195378792,1.,-3.45825932955032));
#56358=CARTESIAN_POINT('Ctrl Pts',(-1.53851507915502,-1.,-3.46531752207153));
#56359=CARTESIAN_POINT('Ctrl Pts',(-1.53851507915502,1.,-3.46531752207153));
#56360=CARTESIAN_POINT('Ctrl Pts',(-1.54266605398187,-1.,-3.47217189224653));
#56361=CARTESIAN_POINT('Ctrl Pts',(-1.54266605398187,1.,-3.47217189224653));
#56362=CARTESIAN_POINT('Ctrl Pts',(-1.54678009290276,-1.,-3.47868272898751));
#56363=CARTESIAN_POINT('Ctrl Pts',(-1.54678009290276,1.,-3.47868272898751));
#56364=CARTESIAN_POINT('Ctrl Pts',(-1.55084702970452,-1.,-3.48485155928567));
#56365=CARTESIAN_POINT('Ctrl Pts',(-1.55084702970452,1.,-3.48485155928567));
#56366=CARTESIAN_POINT('Ctrl Pts',(-1.55489595901116,-1.,-3.4907646087742));
#56367=CARTESIAN_POINT('Ctrl Pts',(-1.55489595901116,1.,-3.4907646087742));
#56368=CARTESIAN_POINT('Ctrl Pts',(-1.55897703097874,-1.,-3.49655185179655));
#56369=CARTESIAN_POINT('Ctrl Pts',(-1.55897703097874,1.,-3.49655185179655));
#56370=CARTESIAN_POINT('Ctrl Pts',(-1.56314187758675,-1.,-3.50234321621578));
#56371=CARTESIAN_POINT('Ctrl Pts',(-1.56314187758675,1.,-3.50234321621578));
#56372=CARTESIAN_POINT('Ctrl Pts',(-1.56742097575012,-1.,-3.50821771695363));
#56373=CARTESIAN_POINT('Ctrl Pts',(-1.56742097575012,1.,-3.50821771695363));
#56374=CARTESIAN_POINT('Ctrl Pts',(-1.57181569799743,-1.,-3.51418598431665));
#56375=CARTESIAN_POINT('Ctrl Pts',(-1.57181569799743,1.,-3.51418598431665));
#56376=CARTESIAN_POINT('Ctrl Pts',(-1.57631049988158,-1.,-3.52021847865912));
#56377=CARTESIAN_POINT('Ctrl Pts',(-1.57631049988158,1.,-3.52021847865912));
#56378=CARTESIAN_POINT('Ctrl Pts',(-1.58088027227848,-1.,-3.52626275334881));
#56379=CARTESIAN_POINT('Ctrl Pts',(-1.58088027227848,1.,-3.52626275334881));
#56380=CARTESIAN_POINT('Ctrl Pts',(-1.58549906268088,-1.,-3.5322637814708));
#56381=CARTESIAN_POINT('Ctrl Pts',(-1.58549906268088,1.,-3.5322637814708));
#56382=CARTESIAN_POINT('Ctrl Pts',(-1.59014958368739,-1.,-3.53818616861077));
#56383=CARTESIAN_POINT('Ctrl Pts',(-1.59014958368739,1.,-3.53818616861077));
#56384=CARTESIAN_POINT('Ctrl Pts',(-1.59482766949766,-1.,-3.54402458182337));
#56385=CARTESIAN_POINT('Ctrl Pts',(-1.59482766949766,1.,-3.54402458182337));
#56386=CARTESIAN_POINT('Ctrl Pts',(-1.59953698113457,-1.,-3.54979148634454));
#56387=CARTESIAN_POINT('Ctrl Pts',(-1.59953698113457,1.,-3.54979148634454));
#56388=CARTESIAN_POINT('Ctrl Pts',(-1.60428584699853,-1.,-3.55550985096129));
#56389=CARTESIAN_POINT('Ctrl Pts',(-1.60428584699853,1.,-3.55550985096129));
#56390=CARTESIAN_POINT('Ctrl Pts',(-1.60908344685457,-1.,-3.5612043248298));
#56391=CARTESIAN_POINT('Ctrl Pts',(-1.60908344685457,1.,-3.5612043248298));
#56392=CARTESIAN_POINT('Ctrl Pts',(-1.61393581747514,-1.,-3.56689200468387));
#56393=CARTESIAN_POINT('Ctrl Pts',(-1.61393581747514,1.,-3.56689200468387));
#56394=CARTESIAN_POINT('Ctrl Pts',(-1.61884340915404,-1.,-3.57257679609806));
#56395=CARTESIAN_POINT('Ctrl Pts',(-1.61884340915404,1.,-3.57257679609806));
#56396=CARTESIAN_POINT('Ctrl Pts',(-1.62380329464844,-1.,-3.5782545595439));
#56397=CARTESIAN_POINT('Ctrl Pts',(-1.62380329464844,1.,-3.5782545595439));
#56398=CARTESIAN_POINT('Ctrl Pts',(-1.62881051550745,-1.,-3.58391625774343));
#56399=CARTESIAN_POINT('Ctrl Pts',(-1.62881051550745,1.,-3.58391625774343));
#56400=CARTESIAN_POINT('Ctrl Pts',(-1.6338597145126,-1.,-3.58955176627879));
#56401=CARTESIAN_POINT('Ctrl Pts',(-1.6338597145126,1.,-3.58955176627879));
#56402=CARTESIAN_POINT('Ctrl Pts',(-1.63894676675352,-1.,-3.59515368334893));
#56403=CARTESIAN_POINT('Ctrl Pts',(-1.63894676675352,1.,-3.59515368334893));
#56404=CARTESIAN_POINT('Ctrl Pts',(-1.64407004385582,-1.,-3.60072028513845));
#56405=CARTESIAN_POINT('Ctrl Pts',(-1.64407004385582,1.,-3.60072028513845));
#56406=CARTESIAN_POINT('Ctrl Pts',(-1.64922952425832,-1.,-3.60625346556992));
#56407=CARTESIAN_POINT('Ctrl Pts',(-1.64922952425832,1.,-3.60625346556992));
#56408=CARTESIAN_POINT('Ctrl Pts',(-1.65442619244325,-1.,-3.61175734965127));
#56409=CARTESIAN_POINT('Ctrl Pts',(-1.65442619244325,1.,-3.61175734965127));
#56410=CARTESIAN_POINT('Ctrl Pts',(-1.65966133399186,-1.,-3.61723666482456));
#56411=CARTESIAN_POINT('Ctrl Pts',(-1.65966133399186,1.,-3.61723666482456));
#56412=CARTESIAN_POINT('Ctrl Pts',(-1.66493585923855,-1.,-3.62269517989109));
#56413=CARTESIAN_POINT('Ctrl Pts',(-1.66493585923855,1.,-3.62269517989109));
#56414=CARTESIAN_POINT('Ctrl Pts',(-1.67024966008045,-1.,-3.62813422105271));
#56415=CARTESIAN_POINT('Ctrl Pts',(-1.67024966008045,1.,-3.62813422105271));
#56416=CARTESIAN_POINT('Ctrl Pts',(-1.67560193613156,-1.,-3.63355343201232));
#56417=CARTESIAN_POINT('Ctrl Pts',(-1.67560193613156,1.,-3.63355343201232));
#56418=CARTESIAN_POINT('Ctrl Pts',(-1.68099146651586,-1.,-3.63895140887462));
#56419=CARTESIAN_POINT('Ctrl Pts',(-1.68099146651586,1.,-3.63895140887462));
#56420=CARTESIAN_POINT('Ctrl Pts',(-1.68641690471457,-1.,-3.64432638915203));
#56421=CARTESIAN_POINT('Ctrl Pts',(-1.68641690471457,1.,-3.64432638915203));
#56422=CARTESIAN_POINT('Ctrl Pts',(-1.69187705481689,-1.,-3.64967689827371));
#56423=CARTESIAN_POINT('Ctrl Pts',(-1.69187705481689,1.,-3.64967689827371));
#56424=CARTESIAN_POINT('Ctrl Pts',(-1.69737117722534,-1.,-3.65500246526749));
#56425=CARTESIAN_POINT('Ctrl Pts',(-1.69737117722534,1.,-3.65500246526749));
#56426=CARTESIAN_POINT('Ctrl Pts',(-1.70289888566873,-1.,-3.66030338774847));
#56427=CARTESIAN_POINT('Ctrl Pts',(-1.70289888566873,1.,-3.66030338774847));
#56428=CARTESIAN_POINT('Ctrl Pts',(-1.70846001610956,-1.,-3.66558043198876));
#56429=CARTESIAN_POINT('Ctrl Pts',(-1.70846001610956,1.,-3.66558043198876));
#56430=CARTESIAN_POINT('Ctrl Pts',(-1.71405450210384,-1.,-3.67083454901611));
#56431=CARTESIAN_POINT('Ctrl Pts',(-1.71405450210384,1.,-3.67083454901611));
#56432=CARTESIAN_POINT('Ctrl Pts',(-1.71968225581808,-1.,-3.67606660374709));
#56433=CARTESIAN_POINT('Ctrl Pts',(-1.71968225581808,1.,-3.67606660374709));
#56434=CARTESIAN_POINT('Ctrl Pts',(-1.72534302437056,-1.,-3.68127704936579));
#56435=CARTESIAN_POINT('Ctrl Pts',(-1.72534302437056,1.,-3.68127704936579));
#56436=CARTESIAN_POINT('Ctrl Pts',(-1.73103640956717,-1.,-3.68646597019332));
#56437=CARTESIAN_POINT('Ctrl Pts',(-1.73103640956717,1.,-3.68646597019332));
#56438=CARTESIAN_POINT('Ctrl Pts',(-1.73676193254557,-1.,-3.69163322648036));
#56439=CARTESIAN_POINT('Ctrl Pts',(-1.73676193254557,1.,-3.69163322648036));
#56440=CARTESIAN_POINT('Ctrl Pts',(-1.74251908492617,-1.,-3.69677856910517));
#56441=CARTESIAN_POINT('Ctrl Pts',(-1.74251908492617,1.,-3.69677856910517));
#56442=CARTESIAN_POINT('Ctrl Pts',(-1.74830738046057,-1.,-3.7019017567335));
#56443=CARTESIAN_POINT('Ctrl Pts',(-1.74830738046057,1.,-3.7019017567335));
#56444=CARTESIAN_POINT('Ctrl Pts',(-1.75412641804042,-1.,-3.70700269736659));
#56445=CARTESIAN_POINT('Ctrl Pts',(-1.75412641804042,1.,-3.70700269736659));
#56446=CARTESIAN_POINT('Ctrl Pts',(-1.75997588498865,-1.,-3.71208146346136));
#56447=CARTESIAN_POINT('Ctrl Pts',(-1.75997588498865,1.,-3.71208146346136));
#56448=CARTESIAN_POINT('Ctrl Pts',(-1.76585552124394,-1.,-3.71713822377359));
#56449=CARTESIAN_POINT('Ctrl Pts',(-1.76585552124394,1.,-3.71713822377359));
#56450=CARTESIAN_POINT('Ctrl Pts',(-1.77176509401761,-1.,-3.72217319911254));
#56451=CARTESIAN_POINT('Ctrl Pts',(-1.77176509401761,1.,-3.72217319911254));
#56452=CARTESIAN_POINT('Ctrl Pts',(-1.77770437039658,-1.,-3.72718661205609));
#56453=CARTESIAN_POINT('Ctrl Pts',(-1.77770437039658,1.,-3.72718661205609));
#56454=CARTESIAN_POINT('Ctrl Pts',(-1.78367308442901,-1.,-3.7321786309547));
#56455=CARTESIAN_POINT('Ctrl Pts',(-1.78367308442901,1.,-3.7321786309547));
#56456=CARTESIAN_POINT('Ctrl Pts',(-1.78967092823491,-1.,-3.73714934730681));
#56457=CARTESIAN_POINT('Ctrl Pts',(-1.78967092823491,1.,-3.73714934730681));
#56458=CARTESIAN_POINT('Ctrl Pts',(-1.79569757859422,-1.,-3.74209880352445));
#56459=CARTESIAN_POINT('Ctrl Pts',(-1.79569757859422,1.,-3.74209880352445));
#56460=CARTESIAN_POINT('Ctrl Pts',(-1.8017527148577,-1.,-3.74702700875467));
#56461=CARTESIAN_POINT('Ctrl Pts',(-1.8017527148577,1.,-3.74702700875467));
#56462=CARTESIAN_POINT('Ctrl Pts',(-1.80783603939617,-1.,-3.75193395887977));
#56463=CARTESIAN_POINT('Ctrl Pts',(-1.80783603939617,1.,-3.75193395887977));
#56464=CARTESIAN_POINT('Ctrl Pts',(-1.8139472983358,-1.,-3.75681965683071));
#56465=CARTESIAN_POINT('Ctrl Pts',(-1.8139472983358,1.,-3.75681965683071));
#56466=CARTESIAN_POINT('Ctrl Pts',(-1.82008629694091,-1.,-3.76168412707948));
#56467=CARTESIAN_POINT('Ctrl Pts',(-1.82008629694091,1.,-3.76168412707948));
#56468=CARTESIAN_POINT('Ctrl Pts',(-1.82625289220915,-1.,-3.76652740353775));
#56469=CARTESIAN_POINT('Ctrl Pts',(-1.82625289220915,1.,-3.76652740353775));
#56470=CARTESIAN_POINT('Ctrl Pts',(-1.83120816955645,-1.,-3.77038509817999));
#56471=CARTESIAN_POINT('Ctrl Pts',(-1.83120816955645,1.,-3.77038509817999));
#56472=CARTESIAN_POINT('Ctrl Pts',(-1.83493697934534,-1.,-3.77326886064398));
#56473=CARTESIAN_POINT('Ctrl Pts',(-1.83493697934534,1.,-3.77326886064398));
#56474=CARTESIAN_POINT('Ctrl Pts',(-1.83742834010626,-1.,-3.77518714457833));
#56475=CARTESIAN_POINT('Ctrl Pts',(-1.83742834010626,1.,-3.77518714457833));
#56476=CARTESIAN_POINT('Ctrl Pts',(-1.83867539237861,-1.,-3.77614523045147));
#56477=CARTESIAN_POINT('Ctrl Pts',(-1.83867539237861,1.,-3.77614523045147));
#56478=CARTESIAN_POINT('',(-1.5189508286633,1.,-3.42859860294306));
#56479=CARTESIAN_POINT('Ctrl Pts',(-1.5189508286633,-1.,-3.42859860294306));
#56480=CARTESIAN_POINT('Ctrl Pts',(-1.5189508286633,-0.666666666666667,
-3.42859860294306));
#56481=CARTESIAN_POINT('Ctrl Pts',(-1.5189508286633,-0.333333333333333,
-3.42859860294306));
#56482=CARTESIAN_POINT('Ctrl Pts',(-1.5189508286633,0.333333333333333,-3.42859860294306));
#56483=CARTESIAN_POINT('Ctrl Pts',(-1.5189508286633,0.666666666666667,-3.42859860294305));
#56484=CARTESIAN_POINT('Ctrl Pts',(-1.5189508286633,1.,-3.42859860294305));
#56485=CARTESIAN_POINT('',(-1.83867539237861,1.,-3.77614523045147));
#56486=CARTESIAN_POINT('',(-1.83867539237861,0.,-3.77614523045147));
#56487=CARTESIAN_POINT('Ctrl Pts',(-1.5189508286633,1.,-3.42859860294306));
#56488=CARTESIAN_POINT('Ctrl Pts',(-1.51893924967331,1.,-3.42864616361875));
#56489=CARTESIAN_POINT('Ctrl Pts',(-1.5189513329503,1.,-3.42884302333841));
#56490=CARTESIAN_POINT('Ctrl Pts',(-1.51914806898491,1.,-3.42946838852588));
#56491=CARTESIAN_POINT('Ctrl Pts',(-1.5198144909338,1.,-3.43101631893414));
#56492=CARTESIAN_POINT('Ctrl Pts',(-1.52134826724293,1.,-3.43417156977893));
#56493=CARTESIAN_POINT('Ctrl Pts',(-1.5237734895035,1.,-3.4388889597401));
#56494=CARTESIAN_POINT('Ctrl Pts',(-1.52686242875556,1.,-3.44469547526647));
#56495=CARTESIAN_POINT('Ctrl Pts',(-1.53046244461635,1.,-3.45127136828305));
#56496=CARTESIAN_POINT('Ctrl Pts',(-1.53440195378792,1.,-3.45825932955032));
#56497=CARTESIAN_POINT('Ctrl Pts',(-1.53851507915502,1.,-3.46531752207153));
#56498=CARTESIAN_POINT('Ctrl Pts',(-1.54266605398187,1.,-3.47217189224653));
#56499=CARTESIAN_POINT('Ctrl Pts',(-1.54678009290276,1.,-3.47868272898751));
#56500=CARTESIAN_POINT('Ctrl Pts',(-1.55084702970452,1.,-3.48485155928567));
#56501=CARTESIAN_POINT('Ctrl Pts',(-1.55489595901116,1.,-3.4907646087742));
#56502=CARTESIAN_POINT('Ctrl Pts',(-1.55897703097874,1.,-3.49655185179655));
#56503=CARTESIAN_POINT('Ctrl Pts',(-1.56314187758675,1.,-3.50234321621578));
#56504=CARTESIAN_POINT('Ctrl Pts',(-1.56742097575012,1.,-3.50821771695363));
#56505=CARTESIAN_POINT('Ctrl Pts',(-1.57181569799743,1.,-3.51418598431665));
#56506=CARTESIAN_POINT('Ctrl Pts',(-1.57631049988158,1.,-3.52021847865912));
#56507=CARTESIAN_POINT('Ctrl Pts',(-1.58088027227848,1.,-3.52626275334881));
#56508=CARTESIAN_POINT('Ctrl Pts',(-1.58549906268088,1.,-3.5322637814708));
#56509=CARTESIAN_POINT('Ctrl Pts',(-1.59014958368739,1.,-3.53818616861077));
#56510=CARTESIAN_POINT('Ctrl Pts',(-1.59482766949766,1.,-3.54402458182337));
#56511=CARTESIAN_POINT('Ctrl Pts',(-1.59953698113457,1.,-3.54979148634454));
#56512=CARTESIAN_POINT('Ctrl Pts',(-1.60428584699853,1.,-3.55550985096129));
#56513=CARTESIAN_POINT('Ctrl Pts',(-1.60908344685457,1.,-3.5612043248298));
#56514=CARTESIAN_POINT('Ctrl Pts',(-1.61393581747514,1.,-3.56689200468387));
#56515=CARTESIAN_POINT('Ctrl Pts',(-1.61884340915404,1.,-3.57257679609806));
#56516=CARTESIAN_POINT('Ctrl Pts',(-1.62380329464844,1.,-3.5782545595439));
#56517=CARTESIAN_POINT('Ctrl Pts',(-1.62881051550745,1.,-3.58391625774343));
#56518=CARTESIAN_POINT('Ctrl Pts',(-1.6338597145126,1.,-3.58955176627879));
#56519=CARTESIAN_POINT('Ctrl Pts',(-1.63894676675352,1.,-3.59515368334893));
#56520=CARTESIAN_POINT('Ctrl Pts',(-1.64407004385582,1.,-3.60072028513845));
#56521=CARTESIAN_POINT('Ctrl Pts',(-1.64922952425832,1.,-3.60625346556992));
#56522=CARTESIAN_POINT('Ctrl Pts',(-1.65442619244325,1.,-3.61175734965127));
#56523=CARTESIAN_POINT('Ctrl Pts',(-1.65966133399186,1.,-3.61723666482456));
#56524=CARTESIAN_POINT('Ctrl Pts',(-1.66493585923855,1.,-3.62269517989109));
#56525=CARTESIAN_POINT('Ctrl Pts',(-1.67024966008045,1.,-3.62813422105271));
#56526=CARTESIAN_POINT('Ctrl Pts',(-1.67560193613156,1.,-3.63355343201232));
#56527=CARTESIAN_POINT('Ctrl Pts',(-1.68099146651586,1.,-3.63895140887462));
#56528=CARTESIAN_POINT('Ctrl Pts',(-1.68641690471457,1.,-3.64432638915203));
#56529=CARTESIAN_POINT('Ctrl Pts',(-1.69187705481689,1.,-3.64967689827371));
#56530=CARTESIAN_POINT('Ctrl Pts',(-1.69737117722534,1.,-3.65500246526749));
#56531=CARTESIAN_POINT('Ctrl Pts',(-1.70289888566873,1.,-3.66030338774847));
#56532=CARTESIAN_POINT('Ctrl Pts',(-1.70846001610956,1.,-3.66558043198876));
#56533=CARTESIAN_POINT('Ctrl Pts',(-1.71405450210384,1.,-3.67083454901611));
#56534=CARTESIAN_POINT('Ctrl Pts',(-1.71968225581808,1.,-3.67606660374709));
#56535=CARTESIAN_POINT('Ctrl Pts',(-1.72534302437056,1.,-3.68127704936579));
#56536=CARTESIAN_POINT('Ctrl Pts',(-1.73103640956717,1.,-3.68646597019332));
#56537=CARTESIAN_POINT('Ctrl Pts',(-1.73676193254557,1.,-3.69163322648036));
#56538=CARTESIAN_POINT('Ctrl Pts',(-1.74251908492617,1.,-3.69677856910517));
#56539=CARTESIAN_POINT('Ctrl Pts',(-1.74830738046057,1.,-3.7019017567335));
#56540=CARTESIAN_POINT('Ctrl Pts',(-1.75412641804042,1.,-3.70700269736659));
#56541=CARTESIAN_POINT('Ctrl Pts',(-1.75997588498865,1.,-3.71208146346136));
#56542=CARTESIAN_POINT('Ctrl Pts',(-1.76585552124394,1.,-3.71713822377359));
#56543=CARTESIAN_POINT('Ctrl Pts',(-1.77176509401761,1.,-3.72217319911254));
#56544=CARTESIAN_POINT('Ctrl Pts',(-1.77770437039658,1.,-3.72718661205609));
#56545=CARTESIAN_POINT('Ctrl Pts',(-1.78367308442901,1.,-3.7321786309547));
#56546=CARTESIAN_POINT('Ctrl Pts',(-1.78967092823491,1.,-3.73714934730681));
#56547=CARTESIAN_POINT('Ctrl Pts',(-1.79569757859422,1.,-3.74209880352445));
#56548=CARTESIAN_POINT('Ctrl Pts',(-1.8017527148577,1.,-3.74702700875467));
#56549=CARTESIAN_POINT('Ctrl Pts',(-1.80783603939617,1.,-3.75193395887977));
#56550=CARTESIAN_POINT('Ctrl Pts',(-1.8139472983358,1.,-3.75681965683071));
#56551=CARTESIAN_POINT('Ctrl Pts',(-1.82008629694091,1.,-3.76168412707948));
#56552=CARTESIAN_POINT('Ctrl Pts',(-1.82625289220915,1.,-3.76652740353775));
#56553=CARTESIAN_POINT('Ctrl Pts',(-1.83120816955645,1.,-3.77038509817999));
#56554=CARTESIAN_POINT('Ctrl Pts',(-1.83493697934534,1.,-3.77326886064398));
#56555=CARTESIAN_POINT('Ctrl Pts',(-1.83742834010626,1.,-3.77518714457833));
#56556=CARTESIAN_POINT('Ctrl Pts',(-1.83867539237861,1.,-3.77614523045147));
#56557=CARTESIAN_POINT('Origin',(-1.83867539237861,0.,-3.77614523045147));
#56558=CARTESIAN_POINT('',(-1.97421938526992,1.,-3.70708211654725));
#56559=CARTESIAN_POINT('Origin',(0.,0.,0.));
#56560=CARTESIAN_POINT('',(-1.35032489087269,1.,-3.49844575334386));
#56561=CARTESIAN_POINT('Origin',(0.,1.,0.));
#56562=CARTESIAN_POINT('Ctrl Pts',(-1.35032489087269,1.,-3.49844575334386));
#56563=CARTESIAN_POINT('Ctrl Pts',(-1.35032489087269,0.666666666666667,
-3.49844575334386));
#56564=CARTESIAN_POINT('Ctrl Pts',(-1.35032489087269,0.333333333333333,
-3.49844575334386));
#56565=CARTESIAN_POINT('Ctrl Pts',(-1.35032489087269,-0.333333333333333,
-3.49844575334386));
#56566=CARTESIAN_POINT('Ctrl Pts',(-1.35032489087269,-0.666666666666667,
-3.49844575334386));
#56567=CARTESIAN_POINT('Ctrl Pts',(-1.35032489087269,-1.,-3.49844575334386));
#56568=CARTESIAN_POINT('Ctrl Pts',(-1.36999806084572,-1.,-3.97027773754922));
#56569=CARTESIAN_POINT('Ctrl Pts',(-1.36999806084572,1.,-3.97027773754922));
#56570=CARTESIAN_POINT('Ctrl Pts',(-1.37020239094758,-1.,-3.9687184694173));
#56571=CARTESIAN_POINT('Ctrl Pts',(-1.37020239094758,1.,-3.9687184694173));
#56572=CARTESIAN_POINT('Ctrl Pts',(-1.37060761746027,-1.,-3.96560037975788));
#56573=CARTESIAN_POINT('Ctrl Pts',(-1.37060761746027,1.,-3.96560037975788));
#56574=CARTESIAN_POINT('Ctrl Pts',(-1.37120515615663,-1.,-3.96092458508407));
#56575=CARTESIAN_POINT('Ctrl Pts',(-1.37120515615663,1.,-3.96092458508407));
#56576=CARTESIAN_POINT('Ctrl Pts',(-1.37198126433139,-1.,-3.95469287283105));
#56577=CARTESIAN_POINT('Ctrl Pts',(-1.37198126433139,1.,-3.95469287283105));
#56578=CARTESIAN_POINT('Ctrl Pts',(-1.37291699203423,-1.,-3.94690771786926));
#56579=CARTESIAN_POINT('Ctrl Pts',(-1.37291699203423,1.,-3.94690771786926));
#56580=CARTESIAN_POINT('Ctrl Pts',(-1.37381821967499,-1.,-3.93912709041791));
#56581=CARTESIAN_POINT('Ctrl Pts',(-1.37381821967499,1.,-3.93912709041791));
#56582=CARTESIAN_POINT('Ctrl Pts',(-1.37468482215784,-1.,-3.93135106761941));
#56583=CARTESIAN_POINT('Ctrl Pts',(-1.37468482215784,1.,-3.93135106761941));
#56584=CARTESIAN_POINT('Ctrl Pts',(-1.37551664448057,-1.,-3.92357976987132));
#56585=CARTESIAN_POINT('Ctrl Pts',(-1.37551664448057,1.,-3.92357976987132));
#56586=CARTESIAN_POINT('Ctrl Pts',(-1.37631350505516,-1.,-3.91581337461825));
#56587=CARTESIAN_POINT('Ctrl Pts',(-1.37631350505516,1.,-3.91581337461825));
#56588=CARTESIAN_POINT('Ctrl Pts',(-1.3770751963376,-1.,-3.90805209522729));
#56589=CARTESIAN_POINT('Ctrl Pts',(-1.3770751963376,1.,-3.90805209522729));
#56590=CARTESIAN_POINT('Ctrl Pts',(-1.3778014851263,-1.,-3.90029615196255));
#56591=CARTESIAN_POINT('Ctrl Pts',(-1.3778014851263,1.,-3.90029615196255));
#56592=CARTESIAN_POINT('Ctrl Pts',(-1.37849211287981,-1.,-3.89254574338385));
#56593=CARTESIAN_POINT('Ctrl Pts',(-1.37849211287981,1.,-3.89254574338385));
#56594=CARTESIAN_POINT('Ctrl Pts',(-1.37914679719446,-1.,-3.88480102249461));
#56595=CARTESIAN_POINT('Ctrl Pts',(-1.37914679719446,1.,-3.88480102249461));
#56596=CARTESIAN_POINT('Ctrl Pts',(-1.37976523097187,-1.,-3.87706205830865));
#56597=CARTESIAN_POINT('Ctrl Pts',(-1.37976523097187,1.,-3.87706205830865));
#56598=CARTESIAN_POINT('Ctrl Pts',(-1.38034709213129,-1.,-3.86932885813403));
#56599=CARTESIAN_POINT('Ctrl Pts',(-1.38034709213129,1.,-3.86932885813403));
#56600=CARTESIAN_POINT('Ctrl Pts',(-1.38089205993067,-1.,-3.86160143044187));
#56601=CARTESIAN_POINT('Ctrl Pts',(-1.38089205993067,1.,-3.86160143044187));
#56602=CARTESIAN_POINT('Ctrl Pts',(-1.38139983115075,-1.,-3.85387983979557));
#56603=CARTESIAN_POINT('Ctrl Pts',(-1.38139983115075,1.,-3.85387983979557));
#56604=CARTESIAN_POINT('Ctrl Pts',(-1.38187013346089,-1.,-3.84616425605705));
#56605=CARTESIAN_POINT('Ctrl Pts',(-1.38187013346089,1.,-3.84616425605705));
#56606=CARTESIAN_POINT('Ctrl Pts',(-1.38230274828774,-1.,-3.83845502790609));
#56607=CARTESIAN_POINT('Ctrl Pts',(-1.38230274828774,1.,-3.83845502790609));
#56608=CARTESIAN_POINT('Ctrl Pts',(-1.38269750245086,-1.,-3.83075266982138));
#56609=CARTESIAN_POINT('Ctrl Pts',(-1.38269750245086,1.,-3.83075266982138));
#56610=CARTESIAN_POINT('Ctrl Pts',(-1.38305421262724,-1.,-3.82305771743715));
#56611=CARTESIAN_POINT('Ctrl Pts',(-1.38305421262724,1.,-3.82305771743715));
#56612=CARTESIAN_POINT('Ctrl Pts',(-1.38337263902766,-1.,-3.81537060817765));
#56613=CARTESIAN_POINT('Ctrl Pts',(-1.38337263902766,1.,-3.81537060817765));
#56614=CARTESIAN_POINT('Ctrl Pts',(-1.38365244046226,-1.,-3.80769156398429));
#56615=CARTESIAN_POINT('Ctrl Pts',(-1.38365244046226,1.,-3.80769156398429));
#56616=CARTESIAN_POINT('Ctrl Pts',(-1.38389311766701,-1.,-3.80002044322169));
#56617=CARTESIAN_POINT('Ctrl Pts',(-1.38389311766701,1.,-3.80002044322169));
#56618=CARTESIAN_POINT('Ctrl Pts',(-1.38409399694589,-1.,-3.79235669640907));
#56619=CARTESIAN_POINT('Ctrl Pts',(-1.38409399694589,1.,-3.79235669640907));
#56620=CARTESIAN_POINT('Ctrl Pts',(-1.38425435883773,-1.,-3.78469969805134));
#56621=CARTESIAN_POINT('Ctrl Pts',(-1.38425435883773,1.,-3.78469969805134));
#56622=CARTESIAN_POINT('Ctrl Pts',(-1.38437354551435,-1.,-3.77704902230441));
#56623=CARTESIAN_POINT('Ctrl Pts',(-1.38437354551435,1.,-3.77704902230441));
#56624=CARTESIAN_POINT('Ctrl Pts',(-1.38445107339517,-1.,-3.76940473185775));
#56625=CARTESIAN_POINT('Ctrl Pts',(-1.38445107339517,1.,-3.76940473185775));
#56626=CARTESIAN_POINT('Ctrl Pts',(-1.38448675253343,-1.,-3.76176768271347));
#56627=CARTESIAN_POINT('Ctrl Pts',(-1.38448675253343,1.,-3.76176768271347));
#56628=CARTESIAN_POINT('Ctrl Pts',(-1.38448077997155,-1.,-3.75413976318727));
#56629=CARTESIAN_POINT('Ctrl Pts',(-1.38448077997155,1.,-3.75413976318727));
#56630=CARTESIAN_POINT('Ctrl Pts',(-1.38443344984389,-1.,-3.7465231716786));
#56631=CARTESIAN_POINT('Ctrl Pts',(-1.38443344984389,1.,-3.7465231716786));
#56632=CARTESIAN_POINT('Ctrl Pts',(-1.38434489156456,-1.,-3.73891976418099));
#56633=CARTESIAN_POINT('Ctrl Pts',(-1.38434489156456,1.,-3.73891976418099));
#56634=CARTESIAN_POINT('Ctrl Pts',(-1.38421479111531,-1.,-3.73133035859283));
#56635=CARTESIAN_POINT('Ctrl Pts',(-1.38421479111531,1.,-3.73133035859283));
#56636=CARTESIAN_POINT('Ctrl Pts',(-1.3840421342895,-1.,-3.72375409358805));
#56637=CARTESIAN_POINT('Ctrl Pts',(-1.3840421342895,1.,-3.72375409358805));
#56638=CARTESIAN_POINT('Ctrl Pts',(-1.38382489984585,-1.,-3.7161876605181));
#56639=CARTESIAN_POINT('Ctrl Pts',(-1.38382489984585,1.,-3.7161876605181));
#56640=CARTESIAN_POINT('Ctrl Pts',(-1.38356065402122,-1.,-3.70862680753343));
#56641=CARTESIAN_POINT('Ctrl Pts',(-1.38356065402122,1.,-3.70862680753343));
#56642=CARTESIAN_POINT('Ctrl Pts',(-1.38324717612862,-1.,-3.70106792167894));
#56643=CARTESIAN_POINT('Ctrl Pts',(-1.38324717612862,1.,-3.70106792167894));
#56644=CARTESIAN_POINT('Ctrl Pts',(-1.38288311171649,-1.,-3.69350967899523));
#56645=CARTESIAN_POINT('Ctrl Pts',(-1.38288311171649,1.,-3.69350967899523));
#56646=CARTESIAN_POINT('Ctrl Pts',(-1.38246852827185,-1.,-3.68595444983844));
#56647=CARTESIAN_POINT('Ctrl Pts',(-1.38246852827185,1.,-3.68595444983844));
#56648=CARTESIAN_POINT('Ctrl Pts',(-1.38200574290626,-1.,-3.6784103848243));
#56649=CARTESIAN_POINT('Ctrl Pts',(-1.38200574290626,1.,-3.6784103848243));
#56650=CARTESIAN_POINT('Ctrl Pts',(-1.38149812653876,-1.,-3.67088843112282));
#56651=CARTESIAN_POINT('Ctrl Pts',(-1.38149812653876,1.,-3.67088843112282));
#56652=CARTESIAN_POINT('Ctrl Pts',(-1.38094856333558,-1.,-3.66339848520874));
#56653=CARTESIAN_POINT('Ctrl Pts',(-1.38094856333558,1.,-3.66339848520874));
#56654=CARTESIAN_POINT('Ctrl Pts',(-1.38035791051215,-1.,-3.65594554404396));
#56655=CARTESIAN_POINT('Ctrl Pts',(-1.38035791051215,1.,-3.65594554404396));
#56656=CARTESIAN_POINT('Ctrl Pts',(-1.37972372481598,-1.,-3.64852652756444));
#56657=CARTESIAN_POINT('Ctrl Pts',(-1.37972372481598,1.,-3.64852652756444));
#56658=CARTESIAN_POINT('Ctrl Pts',(-1.37903818567347,-1.,-3.64112507791112));
#56659=CARTESIAN_POINT('Ctrl Pts',(-1.37903818567347,1.,-3.64112507791112));
#56660=CARTESIAN_POINT('Ctrl Pts',(-1.37829035457324,-1.,-3.63371727442448));
#56661=CARTESIAN_POINT('Ctrl Pts',(-1.37829035457324,1.,-3.63371727442448));
#56662=CARTESIAN_POINT('Ctrl Pts',(-1.37746987919868,-1.,-3.62628098665112));
#56663=CARTESIAN_POINT('Ctrl Pts',(-1.37746987919868,1.,-3.62628098665112));
#56664=CARTESIAN_POINT('Ctrl Pts',(-1.37657053403102,-1.,-3.61880481160408));
#56665=CARTESIAN_POINT('Ctrl Pts',(-1.37657053403102,1.,-3.61880481160408));
#56666=CARTESIAN_POINT('Ctrl Pts',(-1.37559314436641,-1.,-3.61129546591082));
#56667=CARTESIAN_POINT('Ctrl Pts',(-1.37559314436641,1.,-3.61129546591082));
#56668=CARTESIAN_POINT('Ctrl Pts',(-1.37455051379642,-1.,-3.60379020124038));
#56669=CARTESIAN_POINT('Ctrl Pts',(-1.37455051379642,1.,-3.60379020124038));
#56670=CARTESIAN_POINT('Ctrl Pts',(-1.37346320103184,-1.,-3.59634627869117));
#56671=CARTESIAN_POINT('Ctrl Pts',(-1.37346320103184,1.,-3.59634627869117));
#56672=CARTESIAN_POINT('Ctrl Pts',(-1.37235053661,-1.,-3.5890185384643));
#56673=CARTESIAN_POINT('Ctrl Pts',(-1.37235053661,1.,-3.5890185384643));
#56674=CARTESIAN_POINT('Ctrl Pts',(-1.37122241663073,-1.,-3.58183885982745));
#56675=CARTESIAN_POINT('Ctrl Pts',(-1.37122241663073,1.,-3.58183885982745));
#56676=CARTESIAN_POINT('Ctrl Pts',(-1.37007229485646,-1.,-3.57479875549453));
#56677=CARTESIAN_POINT('Ctrl Pts',(-1.37007229485646,1.,-3.57479875549453));
#56678=CARTESIAN_POINT('Ctrl Pts',(-1.36886584973349,-1.,-3.56782080304554));
#56679=CARTESIAN_POINT('Ctrl Pts',(-1.36886584973349,1.,-3.56782080304554));
#56680=CARTESIAN_POINT('Ctrl Pts',(-1.36754771771174,-1.,-3.56077662028492));
#56681=CARTESIAN_POINT('Ctrl Pts',(-1.36754771771174,1.,-3.56077662028492));
#56682=CARTESIAN_POINT('Ctrl Pts',(-1.36606145456711,-1.,-3.55353883995793));
#56683=CARTESIAN_POINT('Ctrl Pts',(-1.36606145456711,1.,-3.55353883995793));
#56684=CARTESIAN_POINT('Ctrl Pts',(-1.36436666257567,-1.,-3.54602591832893));
#56685=CARTESIAN_POINT('Ctrl Pts',(-1.36436666257567,1.,-3.54602591832893));
#56686=CARTESIAN_POINT('Ctrl Pts',(-1.36245507339334,-1.,-3.53824396425032));
#56687=CARTESIAN_POINT('Ctrl Pts',(-1.36245507339334,1.,-3.53824396425032));
#56688=CARTESIAN_POINT('Ctrl Pts',(-1.36037259643827,-1.,-3.53034464961849));
#56689=CARTESIAN_POINT('Ctrl Pts',(-1.36037259643827,1.,-3.53034464961849));
#56690=CARTESIAN_POINT('Ctrl Pts',(-1.35821701528975,-1.,-3.52261776117121));
#56691=CARTESIAN_POINT('Ctrl Pts',(-1.35821701528975,1.,-3.52261776117121));
#56692=CARTESIAN_POINT('Ctrl Pts',(-1.35611275237288,-1.,-3.51542230699919));
#56693=CARTESIAN_POINT('Ctrl Pts',(-1.35611275237288,1.,-3.51542230699919));
#56694=CARTESIAN_POINT('Ctrl Pts',(-1.35419113576022,-1.,-3.50913227060177));
#56695=CARTESIAN_POINT('Ctrl Pts',(-1.35419113576022,1.,-3.50913227060177));
#56696=CARTESIAN_POINT('Ctrl Pts',(-1.3525703284343,-1.,-3.50408168106113));
#56697=CARTESIAN_POINT('Ctrl Pts',(-1.3525703284343,1.,-3.50408168106113));
#56698=CARTESIAN_POINT('Ctrl Pts',(-1.35133076331065,-1.,-3.50049707063673));
#56699=CARTESIAN_POINT('Ctrl Pts',(-1.35133076331065,1.,-3.50049707063673));
#56700=CARTESIAN_POINT('Ctrl Pts',(-1.35067437417289,-1.,-3.49888720256612));
#56701=CARTESIAN_POINT('Ctrl Pts',(-1.35067437417289,1.,-3.49888720256612));
#56702=CARTESIAN_POINT('Ctrl Pts',(-1.35037650302887,-1.,-3.49840357193384));
#56703=CARTESIAN_POINT('Ctrl Pts',(-1.35037650302887,1.,-3.49840357193384));
#56704=CARTESIAN_POINT('Ctrl Pts',(-1.35026426118351,-1.,-3.49840260053616));
#56705=CARTESIAN_POINT('Ctrl Pts',(-1.35026426118351,1.,-3.49840260053616));
#56706=CARTESIAN_POINT('Ctrl Pts',(-1.35022972712301,-1.,-3.49848248301936));
#56707=CARTESIAN_POINT('Ctrl Pts',(-1.35022972712301,1.,-3.49848248301936));
#56708=CARTESIAN_POINT('',(-1.36999806084572,1.,-3.97027773754922));
#56709=CARTESIAN_POINT('Ctrl Pts',(-1.36999806084572,1.,-3.97027773754922));
#56710=CARTESIAN_POINT('Ctrl Pts',(-1.37020239094758,1.,-3.9687184694173));
#56711=CARTESIAN_POINT('Ctrl Pts',(-1.37060761746027,1.,-3.96560037975788));
#56712=CARTESIAN_POINT('Ctrl Pts',(-1.37120515615663,1.,-3.96092458508407));
#56713=CARTESIAN_POINT('Ctrl Pts',(-1.37198126433139,1.,-3.95469287283105));
#56714=CARTESIAN_POINT('Ctrl Pts',(-1.37291699203423,1.,-3.94690771786926));
#56715=CARTESIAN_POINT('Ctrl Pts',(-1.37381821967499,1.,-3.93912709041791));
#56716=CARTESIAN_POINT('Ctrl Pts',(-1.37468482215784,1.,-3.93135106761941));
#56717=CARTESIAN_POINT('Ctrl Pts',(-1.37551664448057,1.,-3.92357976987132));
#56718=CARTESIAN_POINT('Ctrl Pts',(-1.37631350505516,1.,-3.91581337461825));
#56719=CARTESIAN_POINT('Ctrl Pts',(-1.3770751963376,1.,-3.90805209522729));
#56720=CARTESIAN_POINT('Ctrl Pts',(-1.3778014851263,1.,-3.90029615196255));
#56721=CARTESIAN_POINT('Ctrl Pts',(-1.37849211287981,1.,-3.89254574338385));
#56722=CARTESIAN_POINT('Ctrl Pts',(-1.37914679719446,1.,-3.88480102249461));
#56723=CARTESIAN_POINT('Ctrl Pts',(-1.37976523097187,1.,-3.87706205830865));
#56724=CARTESIAN_POINT('Ctrl Pts',(-1.38034709213129,1.,-3.86932885813403));
#56725=CARTESIAN_POINT('Ctrl Pts',(-1.38089205993067,1.,-3.86160143044187));
#56726=CARTESIAN_POINT('Ctrl Pts',(-1.38139983115075,1.,-3.85387983979557));
#56727=CARTESIAN_POINT('Ctrl Pts',(-1.38187013346089,1.,-3.84616425605705));
#56728=CARTESIAN_POINT('Ctrl Pts',(-1.38230274828774,1.,-3.83845502790609));
#56729=CARTESIAN_POINT('Ctrl Pts',(-1.38269750245086,1.,-3.83075266982138));
#56730=CARTESIAN_POINT('Ctrl Pts',(-1.38305421262724,1.,-3.82305771743715));
#56731=CARTESIAN_POINT('Ctrl Pts',(-1.38337263902766,1.,-3.81537060817765));
#56732=CARTESIAN_POINT('Ctrl Pts',(-1.38365244046226,1.,-3.80769156398429));
#56733=CARTESIAN_POINT('Ctrl Pts',(-1.38389311766701,1.,-3.80002044322169));
#56734=CARTESIAN_POINT('Ctrl Pts',(-1.38409399694589,1.,-3.79235669640907));
#56735=CARTESIAN_POINT('Ctrl Pts',(-1.38425435883773,1.,-3.78469969805134));
#56736=CARTESIAN_POINT('Ctrl Pts',(-1.38437354551435,1.,-3.77704902230441));
#56737=CARTESIAN_POINT('Ctrl Pts',(-1.38445107339517,1.,-3.76940473185775));
#56738=CARTESIAN_POINT('Ctrl Pts',(-1.38448675253343,1.,-3.76176768271347));
#56739=CARTESIAN_POINT('Ctrl Pts',(-1.38448077997155,1.,-3.75413976318727));
#56740=CARTESIAN_POINT('Ctrl Pts',(-1.38443344984389,1.,-3.7465231716786));
#56741=CARTESIAN_POINT('Ctrl Pts',(-1.38434489156456,1.,-3.73891976418099));
#56742=CARTESIAN_POINT('Ctrl Pts',(-1.38421479111531,1.,-3.73133035859283));
#56743=CARTESIAN_POINT('Ctrl Pts',(-1.3840421342895,1.,-3.72375409358805));
#56744=CARTESIAN_POINT('Ctrl Pts',(-1.38382489984585,1.,-3.7161876605181));
#56745=CARTESIAN_POINT('Ctrl Pts',(-1.38356065402122,1.,-3.70862680753343));
#56746=CARTESIAN_POINT('Ctrl Pts',(-1.38324717612862,1.,-3.70106792167894));
#56747=CARTESIAN_POINT('Ctrl Pts',(-1.38288311171649,1.,-3.69350967899523));
#56748=CARTESIAN_POINT('Ctrl Pts',(-1.38246852827185,1.,-3.68595444983844));
#56749=CARTESIAN_POINT('Ctrl Pts',(-1.38200574290626,1.,-3.6784103848243));
#56750=CARTESIAN_POINT('Ctrl Pts',(-1.38149812653876,1.,-3.67088843112282));
#56751=CARTESIAN_POINT('Ctrl Pts',(-1.38094856333558,1.,-3.66339848520874));
#56752=CARTESIAN_POINT('Ctrl Pts',(-1.38035791051215,1.,-3.65594554404396));
#56753=CARTESIAN_POINT('Ctrl Pts',(-1.37972372481598,1.,-3.64852652756444));
#56754=CARTESIAN_POINT('Ctrl Pts',(-1.37903818567347,1.,-3.64112507791112));
#56755=CARTESIAN_POINT('Ctrl Pts',(-1.37829035457324,1.,-3.63371727442448));
#56756=CARTESIAN_POINT('Ctrl Pts',(-1.37746987919868,1.,-3.62628098665112));
#56757=CARTESIAN_POINT('Ctrl Pts',(-1.37657053403102,1.,-3.61880481160408));
#56758=CARTESIAN_POINT('Ctrl Pts',(-1.37559314436641,1.,-3.61129546591082));
#56759=CARTESIAN_POINT('Ctrl Pts',(-1.37455051379642,1.,-3.60379020124038));
#56760=CARTESIAN_POINT('Ctrl Pts',(-1.37346320103184,1.,-3.59634627869117));
#56761=CARTESIAN_POINT('Ctrl Pts',(-1.37235053661,1.,-3.5890185384643));
#56762=CARTESIAN_POINT('Ctrl Pts',(-1.37122241663073,1.,-3.58183885982745));
#56763=CARTESIAN_POINT('Ctrl Pts',(-1.37007229485646,1.,-3.57479875549453));
#56764=CARTESIAN_POINT('Ctrl Pts',(-1.36886584973349,1.,-3.56782080304554));
#56765=CARTESIAN_POINT('Ctrl Pts',(-1.36754771771174,1.,-3.56077662028492));
#56766=CARTESIAN_POINT('Ctrl Pts',(-1.36606145456711,1.,-3.55353883995793));
#56767=CARTESIAN_POINT('Ctrl Pts',(-1.36436666257567,1.,-3.54602591832893));
#56768=CARTESIAN_POINT('Ctrl Pts',(-1.36245507339334,1.,-3.53824396425032));
#56769=CARTESIAN_POINT('Ctrl Pts',(-1.36037259643827,1.,-3.53034464961849));
#56770=CARTESIAN_POINT('Ctrl Pts',(-1.35821701528975,1.,-3.52261776117121));
#56771=CARTESIAN_POINT('Ctrl Pts',(-1.35611275237288,1.,-3.51542230699919));
#56772=CARTESIAN_POINT('Ctrl Pts',(-1.35419113576022,1.,-3.50913227060177));
#56773=CARTESIAN_POINT('Ctrl Pts',(-1.3525703284343,1.,-3.50408168106113));
#56774=CARTESIAN_POINT('Ctrl Pts',(-1.35142377279535,1.,-3.5007660381658));
#56775=CARTESIAN_POINT('Ctrl Pts',(-1.35080045218652,1.,-3.49920025459856));
#56776=CARTESIAN_POINT('Ctrl Pts',(-1.35049736560633,1.,-3.49861894124915));
#56777=CARTESIAN_POINT('Ctrl Pts',(-1.35036670893102,1.,-3.49847119623841));
#56778=CARTESIAN_POINT('Ctrl Pts',(-1.35032489087269,1.,-3.49844575334386));
#56779=CARTESIAN_POINT('',(-1.36999806084572,0.,-3.97027773754922));
#56780=CARTESIAN_POINT('Ctrl Pts',(-0.96399761336957,-1.,-3.62397690409552));
#56781=CARTESIAN_POINT('Ctrl Pts',(-0.96399761336957,1.,-3.62397690409552));
#56782=CARTESIAN_POINT('Ctrl Pts',(-0.963922720982576,-1.,-3.62393257642191));
#56783=CARTESIAN_POINT('Ctrl Pts',(-0.963922720982576,1.,-3.62393257642191));
#56784=CARTESIAN_POINT('Ctrl Pts',(-0.963832486396055,-1.,-3.62399933640277));
#56785=CARTESIAN_POINT('Ctrl Pts',(-0.963832486396055,1.,-3.62399933640277));
#56786=CARTESIAN_POINT('Ctrl Pts',(-0.963875774532103,-1.,-3.62456568607055));
#56787=CARTESIAN_POINT('Ctrl Pts',(-0.963875774532103,1.,-3.62456568607055));
#56788=CARTESIAN_POINT('Ctrl Pts',(-0.964291001274618,-1.,-3.62625391255277));
#56789=CARTESIAN_POINT('Ctrl Pts',(-0.964291001274618,1.,-3.62625391255277));
#56790=CARTESIAN_POINT('Ctrl Pts',(-0.965395153165716,-1.,-3.62988252139998));
#56791=CARTESIAN_POINT('Ctrl Pts',(-0.965395153165716,1.,-3.62988252139998));
#56792=CARTESIAN_POINT('Ctrl Pts',(-0.967052554540877,-1.,-3.6349212208096));
#56793=CARTESIAN_POINT('Ctrl Pts',(-0.967052554540877,1.,-3.6349212208096));
#56794=CARTESIAN_POINT('Ctrl Pts',(-0.969195124674829,-1.,-3.64113946505393));
#56795=CARTESIAN_POINT('Ctrl Pts',(-0.969195124674829,1.,-3.64113946505393));
#56796=CARTESIAN_POINT('Ctrl Pts',(-0.971722122060277,-1.,-3.64819756447072));
#56797=CARTESIAN_POINT('Ctrl Pts',(-0.971722122060277,1.,-3.64819756447072));
#56798=CARTESIAN_POINT('Ctrl Pts',(-0.974519971354139,-1.,-3.6557157673487));
#56799=CARTESIAN_POINT('Ctrl Pts',(-0.974519971354139,1.,-3.6557157673487));
#56800=CARTESIAN_POINT('Ctrl Pts',(-0.977478312751416,-1.,-3.66333049637403));
#56801=CARTESIAN_POINT('Ctrl Pts',(-0.977478312751416,1.,-3.66333049637403));
#56802=CARTESIAN_POINT('Ctrl Pts',(-0.980505922458494,-1.,-3.67074983340444));
#56803=CARTESIAN_POINT('Ctrl Pts',(-0.980505922458494,1.,-3.67074983340444));
#56804=CARTESIAN_POINT('Ctrl Pts',(-0.983550791470864,-1.,-3.67782408841876));
#56805=CARTESIAN_POINT('Ctrl Pts',(-0.983550791470864,1.,-3.67782408841876));
#56806=CARTESIAN_POINT('Ctrl Pts',(-0.986602639864286,-1.,-3.6845531792623));
#56807=CARTESIAN_POINT('Ctrl Pts',(-0.986602639864286,1.,-3.6845531792623));
#56808=CARTESIAN_POINT('Ctrl Pts',(-0.989676715398858,-1.,-3.69102682138955));
#56809=CARTESIAN_POINT('Ctrl Pts',(-0.989676715398858,1.,-3.69102682138955));
#56810=CARTESIAN_POINT('Ctrl Pts',(-0.992802218332104,-1.,-3.69738123415696));
#56811=CARTESIAN_POINT('Ctrl Pts',(-0.992802218332104,1.,-3.69738123415696));
#56812=CARTESIAN_POINT('Ctrl Pts',(-0.996009819772432,-1.,-3.70375282282107));
#56813=CARTESIAN_POINT('Ctrl Pts',(-0.996009819772432,1.,-3.70375282282107));
#56814=CARTESIAN_POINT('Ctrl Pts',(-0.999317260756344,-1.,-3.7102243971387));
#56815=CARTESIAN_POINT('Ctrl Pts',(-0.999317260756344,1.,-3.7102243971387));
#56816=CARTESIAN_POINT('Ctrl Pts',(-1.00272423396802,-1.,-3.71680667125047));
#56817=CARTESIAN_POINT('Ctrl Pts',(-1.00272423396802,1.,-3.71680667125047));
#56818=CARTESIAN_POINT('Ctrl Pts',(-1.00622000735696,-1.,-3.72346803750544));
#56819=CARTESIAN_POINT('Ctrl Pts',(-1.00622000735696,1.,-3.72346803750544));
#56820=CARTESIAN_POINT('Ctrl Pts',(-1.00978798539491,-1.,-3.73015276704407));
#56821=CARTESIAN_POINT('Ctrl Pts',(-1.00978798539491,1.,-3.73015276704407));
#56822=CARTESIAN_POINT('Ctrl Pts',(-1.01341114319906,-1.,-3.73680245055747));
#56823=CARTESIAN_POINT('Ctrl Pts',(-1.01341114319906,1.,-3.73680245055747));
#56824=CARTESIAN_POINT('Ctrl Pts',(-1.01707794311088,-1.,-3.74337942504993));
#56825=CARTESIAN_POINT('Ctrl Pts',(-1.01707794311088,1.,-3.74337942504993));
#56826=CARTESIAN_POINT('Ctrl Pts',(-1.02078510487439,-1.,-3.74987777155873));
#56827=CARTESIAN_POINT('Ctrl Pts',(-1.02078510487439,1.,-3.74987777155873));
#56828=CARTESIAN_POINT('Ctrl Pts',(-1.02453429444668,-1.,-3.75631037456224));
#56829=CARTESIAN_POINT('Ctrl Pts',(-1.02453429444668,1.,-3.75631037456224));
#56830=CARTESIAN_POINT('Ctrl Pts',(-1.02833014458184,-1.,-3.76270122291245));
#56831=CARTESIAN_POINT('Ctrl Pts',(-1.02833014458184,1.,-3.76270122291245));
#56832=CARTESIAN_POINT('Ctrl Pts',(-1.03217786604919,-1.,-3.76907609832516));
#56833=CARTESIAN_POINT('Ctrl Pts',(-1.03217786604919,1.,-3.76907609832516));
#56834=CARTESIAN_POINT('Ctrl Pts',(-1.03608074678008,-1.,-3.77545283140427));
#56835=CARTESIAN_POINT('Ctrl Pts',(-1.03608074678008,1.,-3.77545283140427));
#56836=CARTESIAN_POINT('Ctrl Pts',(-1.04003862055798,-1.,-3.7818353500817));
#56837=CARTESIAN_POINT('Ctrl Pts',(-1.04003862055798,1.,-3.7818353500817));
#56838=CARTESIAN_POINT('Ctrl Pts',(-1.04404924374422,-1.,-3.78821910787179));
#56839=CARTESIAN_POINT('Ctrl Pts',(-1.04404924374422,1.,-3.78821910787179));
#56840=CARTESIAN_POINT('Ctrl Pts',(-1.04810913267639,-1.,-3.79459440308786));
#56841=CARTESIAN_POINT('Ctrl Pts',(-1.04810913267639,1.,-3.79459440308786));
#56842=CARTESIAN_POINT('Ctrl Pts',(-1.05221457990016,-1.,-3.80095039790681));
#56843=CARTESIAN_POINT('Ctrl Pts',(-1.05221457990016,1.,-3.80095039790681));
#56844=CARTESIAN_POINT('Ctrl Pts',(-1.05636266918644,-1.,-3.80727913637791));
#56845=CARTESIAN_POINT('Ctrl Pts',(-1.05636266918644,1.,-3.80727913637791));
#56846=CARTESIAN_POINT('Ctrl Pts',(-1.06055206187299,-1.,-3.8135786611749));
#56847=CARTESIAN_POINT('Ctrl Pts',(-1.06055206187299,1.,-3.8135786611749));
#56848=CARTESIAN_POINT('Ctrl Pts',(-1.0647824403893,-1.,-3.81985083953012));
#56849=CARTESIAN_POINT('Ctrl Pts',(-1.0647824403893,1.,-3.81985083953012));
#56850=CARTESIAN_POINT('Ctrl Pts',(-1.06905413180359,-1.,-3.82609989967276));
#56851=CARTESIAN_POINT('Ctrl Pts',(-1.06905413180359,1.,-3.82609989967276));
#56852=CARTESIAN_POINT('Ctrl Pts',(-1.07336766633459,-1.,-3.83233071195144));
#56853=CARTESIAN_POINT('Ctrl Pts',(-1.07336766633459,1.,-3.83233071195144));
#56854=CARTESIAN_POINT('Ctrl Pts',(-1.07772335353858,-1.,-3.83854714117491));
#56855=CARTESIAN_POINT('Ctrl Pts',(-1.07772335353858,1.,-3.83854714117491));
#56856=CARTESIAN_POINT('Ctrl Pts',(-1.08212087917991,-1.,-3.8447504803063));
#56857=CARTESIAN_POINT('Ctrl Pts',(-1.08212087917991,1.,-3.8447504803063));
#56858=CARTESIAN_POINT('Ctrl Pts',(-1.08655950846384,-1.,-3.85094025222713));
#56859=CARTESIAN_POINT('Ctrl Pts',(-1.08655950846384,1.,-3.85094025222713));
#56860=CARTESIAN_POINT('Ctrl Pts',(-1.09103825516294,-1.,-3.85711487933931));
#56861=CARTESIAN_POINT('Ctrl Pts',(-1.09103825516294,1.,-3.85711487933931));
#56862=CARTESIAN_POINT('Ctrl Pts',(-1.09555606505013,-1.,-3.86327241021247));
#56863=CARTESIAN_POINT('Ctrl Pts',(-1.09555606505013,1.,-3.86327241021247));
#56864=CARTESIAN_POINT('Ctrl Pts',(-1.10011198761195,-1.,-3.86941120134849));
#56865=CARTESIAN_POINT('Ctrl Pts',(-1.10011198761195,1.,-3.86941120134849));
#56866=CARTESIAN_POINT('Ctrl Pts',(-1.10470536603287,-1.,-3.87553067187514));
#56867=CARTESIAN_POINT('Ctrl Pts',(-1.10470536603287,1.,-3.87553067187514));
#56868=CARTESIAN_POINT('Ctrl Pts',(-1.10933577224008,-1.,-3.88163105531724));
#56869=CARTESIAN_POINT('Ctrl Pts',(-1.10933577224008,1.,-3.88163105531724));
#56870=CARTESIAN_POINT('Ctrl Pts',(-1.11400292434429,-1.,-3.88771308285171));
#56871=CARTESIAN_POINT('Ctrl Pts',(-1.11400292434429,1.,-3.88771308285171));
#56872=CARTESIAN_POINT('Ctrl Pts',(-1.11870660794603,-1.,-3.89377768340344));
#56873=CARTESIAN_POINT('Ctrl Pts',(-1.11870660794603,1.,-3.89377768340344));
#56874=CARTESIAN_POINT('Ctrl Pts',(-1.12344660099043,-1.,-3.89982569750025));
#56875=CARTESIAN_POINT('Ctrl Pts',(-1.12344660099043,1.,-3.89982569750025));
#56876=CARTESIAN_POINT('Ctrl Pts',(-1.12822258281553,-1.,-3.90585753318737));
#56877=CARTESIAN_POINT('Ctrl Pts',(-1.12822258281553,1.,-3.90585753318737));
#56878=CARTESIAN_POINT('Ctrl Pts',(-1.13303414693896,-1.,-3.91187321145649));
#56879=CARTESIAN_POINT('Ctrl Pts',(-1.13303414693896,1.,-3.91187321145649));
#56880=CARTESIAN_POINT('Ctrl Pts',(-1.13788084225554,-1.,-3.91787251936827));
#56881=CARTESIAN_POINT('Ctrl Pts',(-1.13788084225554,1.,-3.91787251936827));
#56882=CARTESIAN_POINT('Ctrl Pts',(-1.14276220561593,-1.,-3.92385513133997));
#56883=CARTESIAN_POINT('Ctrl Pts',(-1.14276220561593,1.,-3.92385513133997));
#56884=CARTESIAN_POINT('Ctrl Pts',(-1.14767779451123,-1.,-3.92982073294257));
#56885=CARTESIAN_POINT('Ctrl Pts',(-1.14767779451123,1.,-3.92982073294257));
#56886=CARTESIAN_POINT('Ctrl Pts',(-1.1526272271632,-1.,-3.9357691705628));
#56887=CARTESIAN_POINT('Ctrl Pts',(-1.1526272271632,1.,-3.9357691705628));
#56888=CARTESIAN_POINT('Ctrl Pts',(-1.15761018340956,-1.,-3.94170046685203));
#56889=CARTESIAN_POINT('Ctrl Pts',(-1.15761018340956,1.,-3.94170046685203));
#56890=CARTESIAN_POINT('Ctrl Pts',(-1.16262637999157,-1.,-3.94761474780583));
#56891=CARTESIAN_POINT('Ctrl Pts',(-1.16262637999157,1.,-3.94761474780583));
#56892=CARTESIAN_POINT('Ctrl Pts',(-1.16767555244438,-1.,-3.95351219509876));
#56893=CARTESIAN_POINT('Ctrl Pts',(-1.16767555244438,1.,-3.95351219509876));
#56894=CARTESIAN_POINT('Ctrl Pts',(-1.17275743590361,-1.,-3.95939299213276));
#56895=CARTESIAN_POINT('Ctrl Pts',(-1.17275743590361,1.,-3.95939299213276));
#56896=CARTESIAN_POINT('Ctrl Pts',(-1.17787174135592,-1.,-3.96525726358159));
#56897=CARTESIAN_POINT('Ctrl Pts',(-1.17787174135592,1.,-3.96525726358159));
#56898=CARTESIAN_POINT('Ctrl Pts',(-1.18301815039831,-1.,-3.97110505165415));
#56899=CARTESIAN_POINT('Ctrl Pts',(-1.18301815039831,1.,-3.97110505165415));
#56900=CARTESIAN_POINT('Ctrl Pts',(-1.18819633715539,-1.,-3.97693634767754));
#56901=CARTESIAN_POINT('Ctrl Pts',(-1.18819633715539,1.,-3.97693634767754));
#56902=CARTESIAN_POINT('Ctrl Pts',(-1.19340598349475,-1.,-3.98275111052561));
#56903=CARTESIAN_POINT('Ctrl Pts',(-1.19340598349475,1.,-3.98275111052561));
#56904=CARTESIAN_POINT('Ctrl Pts',(-1.19864679609566,-1.,-3.98854928957189));
#56905=CARTESIAN_POINT('Ctrl Pts',(-1.19864679609566,1.,-3.98854928957189));
#56906=CARTESIAN_POINT('Ctrl Pts',(-1.20391852375139,-1.,-3.99433084799666));
#56907=CARTESIAN_POINT('Ctrl Pts',(-1.20391852375139,1.,-3.99433084799666));
#56908=CARTESIAN_POINT('Ctrl Pts',(-1.20922097029551,-1.,-4.00009577950721));
#56909=CARTESIAN_POINT('Ctrl Pts',(-1.20922097029551,1.,-4.00009577950721));
#56910=CARTESIAN_POINT('Ctrl Pts',(-1.21455398918133,-1.,-4.00584409522722));
#56911=CARTESIAN_POINT('Ctrl Pts',(-1.21455398918133,1.,-4.00584409522722));
#56912=CARTESIAN_POINT('Ctrl Pts',(-1.21884478244403,-1.,-4.01042947140789));
#56913=CARTESIAN_POINT('Ctrl Pts',(-1.21884478244403,1.,-4.01042947140789));
#56914=CARTESIAN_POINT('Ctrl Pts',(-1.22207656455845,-1.,-4.01386104433519));
#56915=CARTESIAN_POINT('Ctrl Pts',(-1.22207656455845,1.,-4.01386104433519));
#56916=CARTESIAN_POINT('Ctrl Pts',(-1.22423716681317,-1.,-4.01614544569895));
#56917=CARTESIAN_POINT('Ctrl Pts',(-1.22423716681317,1.,-4.01614544569895));
#56918=CARTESIAN_POINT('Ctrl Pts',(-1.22531898815164,-1.,-4.01728681790024));
#56919=CARTESIAN_POINT('Ctrl Pts',(-1.22531898815164,1.,-4.01728681790024));
#56920=CARTESIAN_POINT('',(-0.963899035118984,1.,-3.62400312501199));
#56921=CARTESIAN_POINT('Ctrl Pts',(-0.963899035118985,-1.,-3.62400312501199));
#56922=CARTESIAN_POINT('Ctrl Pts',(-0.963899035118985,-0.666666666666667,
-3.62400312501199));
#56923=CARTESIAN_POINT('Ctrl Pts',(-0.963899035118985,-0.333333333333333,
-3.62400312501199));
#56924=CARTESIAN_POINT('Ctrl Pts',(-0.963899035118985,0.333333333333333,
-3.62400312501199));
#56925=CARTESIAN_POINT('Ctrl Pts',(-0.963899035118986,0.666666666666667,
-3.62400312501199));
#56926=CARTESIAN_POINT('Ctrl Pts',(-0.963899035118986,1.,-3.62400312501199));
#56927=CARTESIAN_POINT('',(-1.22531898815164,1.,-4.01728681790024));
#56928=CARTESIAN_POINT('',(-1.22531898815164,0.,-4.01728681790024));
#56929=CARTESIAN_POINT('Ctrl Pts',(-0.963899035118985,1.,-3.62400312501199));
#56930=CARTESIAN_POINT('Ctrl Pts',(-0.963880158556713,1.,-3.62404828878375));
#56931=CARTESIAN_POINT('Ctrl Pts',(-0.963861297423579,1.,-3.62424461507455));
#56932=CARTESIAN_POINT('Ctrl Pts',(-0.963957782642589,1.,-3.62489305727516));
#56933=CARTESIAN_POINT('Ctrl Pts',(-0.964373850166081,1.,-3.62652618145252));
#56934=CARTESIAN_POINT('Ctrl Pts',(-0.965395153165716,1.,-3.62988252139998));
#56935=CARTESIAN_POINT('Ctrl Pts',(-0.967052554540877,1.,-3.6349212208096));
#56936=CARTESIAN_POINT('Ctrl Pts',(-0.969195124674829,1.,-3.64113946505393));
#56937=CARTESIAN_POINT('Ctrl Pts',(-0.971722122060277,1.,-3.64819756447072));
#56938=CARTESIAN_POINT('Ctrl Pts',(-0.974519971354139,1.,-3.6557157673487));
#56939=CARTESIAN_POINT('Ctrl Pts',(-0.977478312751416,1.,-3.66333049637403));
#56940=CARTESIAN_POINT('Ctrl Pts',(-0.980505922458494,1.,-3.67074983340444));
#56941=CARTESIAN_POINT('Ctrl Pts',(-0.983550791470864,1.,-3.67782408841876));
#56942=CARTESIAN_POINT('Ctrl Pts',(-0.986602639864286,1.,-3.6845531792623));
#56943=CARTESIAN_POINT('Ctrl Pts',(-0.989676715398858,1.,-3.69102682138955));
#56944=CARTESIAN_POINT('Ctrl Pts',(-0.992802218332104,1.,-3.69738123415696));
#56945=CARTESIAN_POINT('Ctrl Pts',(-0.996009819772432,1.,-3.70375282282107));
#56946=CARTESIAN_POINT('Ctrl Pts',(-0.999317260756344,1.,-3.7102243971387));
#56947=CARTESIAN_POINT('Ctrl Pts',(-1.00272423396802,1.,-3.71680667125047));
#56948=CARTESIAN_POINT('Ctrl Pts',(-1.00622000735696,1.,-3.72346803750544));
#56949=CARTESIAN_POINT('Ctrl Pts',(-1.00978798539491,1.,-3.73015276704407));
#56950=CARTESIAN_POINT('Ctrl Pts',(-1.01341114319906,1.,-3.73680245055747));
#56951=CARTESIAN_POINT('Ctrl Pts',(-1.01707794311088,1.,-3.74337942504993));
#56952=CARTESIAN_POINT('Ctrl Pts',(-1.02078510487439,1.,-3.74987777155873));
#56953=CARTESIAN_POINT('Ctrl Pts',(-1.02453429444668,1.,-3.75631037456224));
#56954=CARTESIAN_POINT('Ctrl Pts',(-1.02833014458184,1.,-3.76270122291245));
#56955=CARTESIAN_POINT('Ctrl Pts',(-1.03217786604919,1.,-3.76907609832516));
#56956=CARTESIAN_POINT('Ctrl Pts',(-1.03608074678008,1.,-3.77545283140427));
#56957=CARTESIAN_POINT('Ctrl Pts',(-1.04003862055798,1.,-3.7818353500817));
#56958=CARTESIAN_POINT('Ctrl Pts',(-1.04404924374422,1.,-3.78821910787179));
#56959=CARTESIAN_POINT('Ctrl Pts',(-1.04810913267639,1.,-3.79459440308786));
#56960=CARTESIAN_POINT('Ctrl Pts',(-1.05221457990016,1.,-3.80095039790681));
#56961=CARTESIAN_POINT('Ctrl Pts',(-1.05636266918644,1.,-3.80727913637791));
#56962=CARTESIAN_POINT('Ctrl Pts',(-1.06055206187299,1.,-3.8135786611749));
#56963=CARTESIAN_POINT('Ctrl Pts',(-1.0647824403893,1.,-3.81985083953012));
#56964=CARTESIAN_POINT('Ctrl Pts',(-1.06905413180359,1.,-3.82609989967276));
#56965=CARTESIAN_POINT('Ctrl Pts',(-1.07336766633459,1.,-3.83233071195144));
#56966=CARTESIAN_POINT('Ctrl Pts',(-1.07772335353858,1.,-3.83854714117491));
#56967=CARTESIAN_POINT('Ctrl Pts',(-1.08212087917991,1.,-3.8447504803063));
#56968=CARTESIAN_POINT('Ctrl Pts',(-1.08655950846384,1.,-3.85094025222713));
#56969=CARTESIAN_POINT('Ctrl Pts',(-1.09103825516294,1.,-3.85711487933931));
#56970=CARTESIAN_POINT('Ctrl Pts',(-1.09555606505013,1.,-3.86327241021247));
#56971=CARTESIAN_POINT('Ctrl Pts',(-1.10011198761195,1.,-3.86941120134849));
#56972=CARTESIAN_POINT('Ctrl Pts',(-1.10470536603287,1.,-3.87553067187514));
#56973=CARTESIAN_POINT('Ctrl Pts',(-1.10933577224008,1.,-3.88163105531724));
#56974=CARTESIAN_POINT('Ctrl Pts',(-1.11400292434429,1.,-3.88771308285171));
#56975=CARTESIAN_POINT('Ctrl Pts',(-1.11870660794603,1.,-3.89377768340344));
#56976=CARTESIAN_POINT('Ctrl Pts',(-1.12344660099043,1.,-3.89982569750025));
#56977=CARTESIAN_POINT('Ctrl Pts',(-1.12822258281553,1.,-3.90585753318737));
#56978=CARTESIAN_POINT('Ctrl Pts',(-1.13303414693896,1.,-3.91187321145649));
#56979=CARTESIAN_POINT('Ctrl Pts',(-1.13788084225554,1.,-3.91787251936827));
#56980=CARTESIAN_POINT('Ctrl Pts',(-1.14276220561593,1.,-3.92385513133997));
#56981=CARTESIAN_POINT('Ctrl Pts',(-1.14767779451123,1.,-3.92982073294257));
#56982=CARTESIAN_POINT('Ctrl Pts',(-1.1526272271632,1.,-3.9357691705628));
#56983=CARTESIAN_POINT('Ctrl Pts',(-1.15761018340956,1.,-3.94170046685203));
#56984=CARTESIAN_POINT('Ctrl Pts',(-1.16262637999157,1.,-3.94761474780583));
#56985=CARTESIAN_POINT('Ctrl Pts',(-1.16767555244438,1.,-3.95351219509876));
#56986=CARTESIAN_POINT('Ctrl Pts',(-1.17275743590361,1.,-3.95939299213276));
#56987=CARTESIAN_POINT('Ctrl Pts',(-1.17787174135592,1.,-3.96525726358159));
#56988=CARTESIAN_POINT('Ctrl Pts',(-1.18301815039831,1.,-3.97110505165415));
#56989=CARTESIAN_POINT('Ctrl Pts',(-1.18819633715539,1.,-3.97693634767754));
#56990=CARTESIAN_POINT('Ctrl Pts',(-1.19340598349475,1.,-3.98275111052561));
#56991=CARTESIAN_POINT('Ctrl Pts',(-1.19864679609566,1.,-3.98854928957189));
#56992=CARTESIAN_POINT('Ctrl Pts',(-1.20391852375139,1.,-3.99433084799666));
#56993=CARTESIAN_POINT('Ctrl Pts',(-1.20922097029551,1.,-4.00009577950721));
#56994=CARTESIAN_POINT('Ctrl Pts',(-1.21455398918133,1.,-4.00584409522722));
#56995=CARTESIAN_POINT('Ctrl Pts',(-1.21884478244403,1.,-4.01042947140789));
#56996=CARTESIAN_POINT('Ctrl Pts',(-1.22207656455845,1.,-4.01386104433519));
#56997=CARTESIAN_POINT('Ctrl Pts',(-1.22423716681317,1.,-4.01614544569895));
#56998=CARTESIAN_POINT('Ctrl Pts',(-1.22531898815164,1.,-4.01728681790024));
#56999=CARTESIAN_POINT('Origin',(-1.22531898815164,0.,-4.01728681790024));
#57000=CARTESIAN_POINT('',(-1.36999806084572,1.,-3.97027773754922));
#57001=CARTESIAN_POINT('Origin',(0.,0.,0.));
#57002=CARTESIAN_POINT('',(-0.786422660833743,1.,-3.66661143271648));
#57003=CARTESIAN_POINT('Origin',(0.,1.,0.));
#57004=CARTESIAN_POINT('Ctrl Pts',(-0.786422660833742,1.,-3.66661143271648));
#57005=CARTESIAN_POINT('Ctrl Pts',(-0.786422660833742,0.666666666666667,
-3.66661143271648));
#57006=CARTESIAN_POINT('Ctrl Pts',(-0.786422660833742,0.333333333333333,
-3.66661143271648));
#57007=CARTESIAN_POINT('Ctrl Pts',(-0.786422660833742,-0.333333333333333,
-3.66661143271648));
#57008=CARTESIAN_POINT('Ctrl Pts',(-0.786422660833742,-0.666666666666667,
-3.66661143271648));
#57009=CARTESIAN_POINT('Ctrl Pts',(-0.786422660833742,-1.,-3.66661143271648));
#57010=CARTESIAN_POINT('Ctrl Pts',(-0.732042837400619,-1.,-4.13571194405636));
#57011=CARTESIAN_POINT('Ctrl Pts',(-0.732042837400619,1.,-4.13571194405636));
#57012=CARTESIAN_POINT('Ctrl Pts',(-0.732488575135926,-1.,-4.13420383737278));
#57013=CARTESIAN_POINT('Ctrl Pts',(-0.732488575135926,1.,-4.13420383737278));
#57014=CARTESIAN_POINT('Ctrl Pts',(-0.733376589325634,-1.,-4.13118752796397));
#57015=CARTESIAN_POINT('Ctrl Pts',(-0.733376589325634,1.,-4.13118752796397));
#57016=CARTESIAN_POINT('Ctrl Pts',(-0.734698226767512,-1.,-4.12666277572794));
#57017=CARTESIAN_POINT('Ctrl Pts',(-0.734698226767512,1.,-4.12666277572794));
#57018=CARTESIAN_POINT('Ctrl Pts',(-0.736439634335347,-1.,-4.12062919626082));
#57019=CARTESIAN_POINT('Ctrl Pts',(-0.736439634335347,1.,-4.12062919626082));
#57020=CARTESIAN_POINT('Ctrl Pts',(-0.738581708229119,-1.,-4.11308626953795));
#57021=CARTESIAN_POINT('Ctrl Pts',(-0.738581708229119,1.,-4.11308626953795));
#57022=CARTESIAN_POINT('Ctrl Pts',(-0.740688998555152,-1.,-4.1055424175856));
#57023=CARTESIAN_POINT('Ctrl Pts',(-0.740688998555152,1.,-4.1055424175856));
#57024=CARTESIAN_POINT('Ctrl Pts',(-0.742761369690018,-1.,-4.09799769702712));
#57025=CARTESIAN_POINT('Ctrl Pts',(-0.742761369690018,1.,-4.09799769702712));
#57026=CARTESIAN_POINT('Ctrl Pts',(-0.744798649705514,-1.,-4.09045220253011));
#57027=CARTESIAN_POINT('Ctrl Pts',(-0.744798649705514,1.,-4.09045220253011));
#57028=CARTESIAN_POINT('Ctrl Pts',(-0.746800631490822,-1.,-4.08290608094789));
#57029=CARTESIAN_POINT('Ctrl Pts',(-0.746800631490822,1.,-4.08290608094789));
#57030=CARTESIAN_POINT('Ctrl Pts',(-0.748767076679177,-1.,-4.07535951055363));
#57031=CARTESIAN_POINT('Ctrl Pts',(-0.748767076679177,1.,-4.07535951055363));
#57032=CARTESIAN_POINT('Ctrl Pts',(-0.750697720483176,-1.,-4.06781267241886));
#57033=CARTESIAN_POINT('Ctrl Pts',(-0.750697720483176,1.,-4.06781267241886));
#57034=CARTESIAN_POINT('Ctrl Pts',(-0.752592276482869,-1.,-4.06026572221399));
#57035=CARTESIAN_POINT('Ctrl Pts',(-0.752592276482869,1.,-4.06026572221399));
#57036=CARTESIAN_POINT('Ctrl Pts',(-0.754450441816412,-1.,-4.05271876688106));
#57037=CARTESIAN_POINT('Ctrl Pts',(-0.754450441816412,1.,-4.05271876688106));
#57038=CARTESIAN_POINT('Ctrl Pts',(-0.756271902370187,-1.,-4.04517182654344));
#57039=CARTESIAN_POINT('Ctrl Pts',(-0.756271902370187,1.,-4.04517182654344));
#57040=CARTESIAN_POINT('Ctrl Pts',(-0.758056338885554,-1.,-4.03762485803468));
#57041=CARTESIAN_POINT('Ctrl Pts',(-0.758056338885554,1.,-4.03762485803468));
#57042=CARTESIAN_POINT('Ctrl Pts',(-0.759803433244166,-1.,-4.0300778195465));
#57043=CARTESIAN_POINT('Ctrl Pts',(-0.759803433244166,1.,-4.0300778195465));
#57044=CARTESIAN_POINT('Ctrl Pts',(-0.761512875859942,-1.,-4.02253072741347));
#57045=CARTESIAN_POINT('Ctrl Pts',(-0.761512875859942,1.,-4.02253072741347));
#57046=CARTESIAN_POINT('Ctrl Pts',(-0.763184371182827,-1.,-4.01498370680434));
#57047=CARTESIAN_POINT('Ctrl Pts',(-0.763184371182827,1.,-4.01498370680434));
#57048=CARTESIAN_POINT('Ctrl Pts',(-0.764817648784946,-1.,-4.00743706791366));
#57049=CARTESIAN_POINT('Ctrl Pts',(-0.764817648784946,1.,-4.00743706791366));
#57050=CARTESIAN_POINT('Ctrl Pts',(-0.766412457135786,-1.,-3.99989129179464));
#57051=CARTESIAN_POINT('Ctrl Pts',(-0.766412457135786,1.,-3.99989129179464));
#57052=CARTESIAN_POINT('Ctrl Pts',(-0.767968531377708,-1.,-3.99234687880892));
#57053=CARTESIAN_POINT('Ctrl Pts',(-0.767968531377708,1.,-3.99234687880892));
#57054=CARTESIAN_POINT('Ctrl Pts',(-0.769485566245459,-1.,-3.98480422348403));
#57055=CARTESIAN_POINT('Ctrl Pts',(-0.769485566245459,1.,-3.98480422348403));
#57056=CARTESIAN_POINT('Ctrl Pts',(-0.770963190030504,-1.,-3.97726349165507));
#57057=CARTESIAN_POINT('Ctrl Pts',(-0.770963190030504,1.,-3.97726349165507));
#57058=CARTESIAN_POINT('Ctrl Pts',(-0.772400931772239,-1.,-3.96972446532832));
#57059=CARTESIAN_POINT('Ctrl Pts',(-0.772400931772239,1.,-3.96972446532832));
#57060=CARTESIAN_POINT('Ctrl Pts',(-0.773798212026683,-1.,-3.96218649639876));
#57061=CARTESIAN_POINT('Ctrl Pts',(-0.773798212026683,1.,-3.96218649639876));
#57062=CARTESIAN_POINT('Ctrl Pts',(-0.775154418039441,-1.,-3.95464885452364));
#57063=CARTESIAN_POINT('Ctrl Pts',(-0.775154418039441,1.,-3.95464885452364));
#57064=CARTESIAN_POINT('Ctrl Pts',(-0.77646896669796,-1.,-3.94711101619471));
#57065=CARTESIAN_POINT('Ctrl Pts',(-0.77646896669796,1.,-3.94711101619471));
#57066=CARTESIAN_POINT('Ctrl Pts',(-0.77774137056855,-1.,-3.93957296768098));
#57067=CARTESIAN_POINT('Ctrl Pts',(-0.77774137056855,1.,-3.93957296768098));
#57068=CARTESIAN_POINT('Ctrl Pts',(-0.778971308134786,-1.,-3.93203552473153));
#57069=CARTESIAN_POINT('Ctrl Pts',(-0.778971308134786,1.,-3.93203552473153));
#57070=CARTESIAN_POINT('Ctrl Pts',(-0.780158678615507,-1.,-3.92450058323799));
#57071=CARTESIAN_POINT('Ctrl Pts',(-0.780158678615507,1.,-3.92450058323799));
#57072=CARTESIAN_POINT('Ctrl Pts',(-0.781303428618344,-1.,-3.9169703605466));
#57073=CARTESIAN_POINT('Ctrl Pts',(-0.781303428618344,1.,-3.9169703605466));
#57074=CARTESIAN_POINT('Ctrl Pts',(-0.782405395622759,-1.,-3.90944671004536));
#57075=CARTESIAN_POINT('Ctrl Pts',(-0.782405395622759,1.,-3.90944671004536));
#57076=CARTESIAN_POINT('Ctrl Pts',(-0.783464141529082,-1.,-3.90193039043971));
#57077=CARTESIAN_POINT('Ctrl Pts',(-0.783464141529082,1.,-3.90193039043971));
#57078=CARTESIAN_POINT('Ctrl Pts',(-0.784478799358336,-1.,-3.89442039235105));
#57079=CARTESIAN_POINT('Ctrl Pts',(-0.784478799358336,1.,-3.89442039235105));
#57080=CARTESIAN_POINT('Ctrl Pts',(-0.785447890340723,-1.,-3.88691313167399));
#57081=CARTESIAN_POINT('Ctrl Pts',(-0.785447890340723,1.,-3.88691313167399));
#57082=CARTESIAN_POINT('Ctrl Pts',(-0.786369675812592,-1.,-3.87940402818186));
#57083=CARTESIAN_POINT('Ctrl Pts',(-0.786369675812592,1.,-3.87940402818186));
#57084=CARTESIAN_POINT('Ctrl Pts',(-0.78724252761798,-1.,-3.87188916600905));
#57085=CARTESIAN_POINT('Ctrl Pts',(-0.78724252761798,1.,-3.87188916600905));
#57086=CARTESIAN_POINT('Ctrl Pts',(-0.788065315093771,-1.,-3.86436702561342));
#57087=CARTESIAN_POINT('Ctrl Pts',(-0.788065315093771,1.,-3.86436702561342));
#57088=CARTESIAN_POINT('Ctrl Pts',(-0.788837734090688,-1.,-3.85683995872536));
#57089=CARTESIAN_POINT('Ctrl Pts',(-0.788837734090688,1.,-3.85683995872536));
#57090=CARTESIAN_POINT('Ctrl Pts',(-0.789560798155619,-1.,-3.8493163780891));
#57091=CARTESIAN_POINT('Ctrl Pts',(-0.789560798155619,1.,-3.8493163780891));
#57092=CARTESIAN_POINT('Ctrl Pts',(-0.790236124191289,-1.,-3.84180762342476));
#57093=CARTESIAN_POINT('Ctrl Pts',(-0.790236124191289,1.,-3.84180762342476));
#57094=CARTESIAN_POINT('Ctrl Pts',(-0.79086501270534,-1.,-3.83432392054804));
#57095=CARTESIAN_POINT('Ctrl Pts',(-0.79086501270534,1.,-3.83432392054804));
#57096=CARTESIAN_POINT('Ctrl Pts',(-0.791447528662381,-1.,-3.82687033899799));
#57097=CARTESIAN_POINT('Ctrl Pts',(-0.791447528662381,1.,-3.82687033899799));
#57098=CARTESIAN_POINT('Ctrl Pts',(-0.791981740718606,-1.,-3.81944345442237));
#57099=CARTESIAN_POINT('Ctrl Pts',(-0.791981740718606,1.,-3.81944345442237));
#57100=CARTESIAN_POINT('Ctrl Pts',(-0.792462483517568,-1.,-3.81202588694726));
#57101=CARTESIAN_POINT('Ctrl Pts',(-0.792462483517568,1.,-3.81202588694726));
#57102=CARTESIAN_POINT('Ctrl Pts',(-0.792882695234693,-1.,-3.80459229925598));
#57103=CARTESIAN_POINT('Ctrl Pts',(-0.792882695234693,1.,-3.80459229925598));
#57104=CARTESIAN_POINT('Ctrl Pts',(-0.7932356129732,-1.,-3.79711921389862));
#57105=CARTESIAN_POINT('Ctrl Pts',(-0.7932356129732,1.,-3.79711921389862));
#57106=CARTESIAN_POINT('Ctrl Pts',(-0.793516871680966,-1.,-3.78959439439222));
#57107=CARTESIAN_POINT('Ctrl Pts',(-0.793516871680966,1.,-3.78959439439222));
#57108=CARTESIAN_POINT('Ctrl Pts',(-0.793726235781339,-1.,-3.78202460377617));
#57109=CARTESIAN_POINT('Ctrl Pts',(-0.793726235781339,1.,-3.78202460377617));
#57110=CARTESIAN_POINT('Ctrl Pts',(-0.793870523787515,-1.,-3.77444863801264));
#57111=CARTESIAN_POINT('Ctrl Pts',(-0.793870523787515,1.,-3.77444863801264));
#57112=CARTESIAN_POINT('Ctrl Pts',(-0.793961083689141,-1.,-3.76692626931184));
#57113=CARTESIAN_POINT('Ctrl Pts',(-0.793961083689141,1.,-3.76692626931184));
#57114=CARTESIAN_POINT('Ctrl Pts',(-0.794008429135047,-1.,-3.75951468666325));
#57115=CARTESIAN_POINT('Ctrl Pts',(-0.794008429135047,1.,-3.75951468666325));
#57116=CARTESIAN_POINT('Ctrl Pts',(-0.794017347371441,-1.,-3.75224692493895));
#57117=CARTESIAN_POINT('Ctrl Pts',(-0.794017347371441,1.,-3.75224692493895));
#57118=CARTESIAN_POINT('Ctrl Pts',(-0.79398270045988,-1.,-3.74511357728827));
#57119=CARTESIAN_POINT('Ctrl Pts',(-0.79398270045988,1.,-3.74511357728827));
#57120=CARTESIAN_POINT('Ctrl Pts',(-0.79388270093679,-1.,-3.73803280541576));
#57121=CARTESIAN_POINT('Ctrl Pts',(-0.79388270093679,1.,-3.73803280541576));
#57122=CARTESIAN_POINT('Ctrl Pts',(-0.793682750269347,-1.,-3.7308691469564));
#57123=CARTESIAN_POINT('Ctrl Pts',(-0.793682750269347,1.,-3.7308691469564));
#57124=CARTESIAN_POINT('Ctrl Pts',(-0.79334702378387,-1.,-3.7234879729357));
#57125=CARTESIAN_POINT('Ctrl Pts',(-0.79334702378387,1.,-3.7234879729357));
#57126=CARTESIAN_POINT('Ctrl Pts',(-0.792848377370115,-1.,-3.7158024239604));
#57127=CARTESIAN_POINT('Ctrl Pts',(-0.792848377370115,1.,-3.7158024239604));
#57128=CARTESIAN_POINT('Ctrl Pts',(-0.792177688845968,-1.,-3.70781724021879));
#57129=CARTESIAN_POINT('Ctrl Pts',(-0.792177688845968,1.,-3.70781724021879));
#57130=CARTESIAN_POINT('Ctrl Pts',(-0.791356575696509,-1.,-3.69968940808982));
#57131=CARTESIAN_POINT('Ctrl Pts',(-0.791356575696509,1.,-3.69968940808982));
#57132=CARTESIAN_POINT('Ctrl Pts',(-0.79043628498958,-1.,-3.69172044327754));
#57133=CARTESIAN_POINT('Ctrl Pts',(-0.79043628498958,1.,-3.69172044327754));
#57134=CARTESIAN_POINT('Ctrl Pts',(-0.789483546065158,-1.,-3.68428439784285));
#57135=CARTESIAN_POINT('Ctrl Pts',(-0.789483546065158,1.,-3.68428439784285));
#57136=CARTESIAN_POINT('Ctrl Pts',(-0.788569566220662,-1.,-3.67777119516438));
#57137=CARTESIAN_POINT('Ctrl Pts',(-0.788569566220662,1.,-3.67777119516438));
#57138=CARTESIAN_POINT('Ctrl Pts',(-0.787758799995426,-1.,-3.672529236635));
#57139=CARTESIAN_POINT('Ctrl Pts',(-0.787758799995426,1.,-3.672529236635));
#57140=CARTESIAN_POINT('Ctrl Pts',(-0.787095252589508,-1.,-3.66879484800625));
#57141=CARTESIAN_POINT('Ctrl Pts',(-0.787095252589508,1.,-3.66879484800625));
#57142=CARTESIAN_POINT('Ctrl Pts',(-0.786698783541658,-1.,-3.66710211819938));
#57143=CARTESIAN_POINT('Ctrl Pts',(-0.786698783541658,1.,-3.66710211819938));
#57144=CARTESIAN_POINT('Ctrl Pts',(-0.786480236184947,-1.,-3.66657784454965));
#57145=CARTESIAN_POINT('Ctrl Pts',(-0.786480236184947,1.,-3.66657784454965));
#57146=CARTESIAN_POINT('Ctrl Pts',(-0.786369528183039,-1.,-3.66655932661846));
#57147=CARTESIAN_POINT('Ctrl Pts',(-0.786369528183039,1.,-3.66655932661846));
#57148=CARTESIAN_POINT('Ctrl Pts',(-0.786322922920599,-1.,-3.66663282329846));
#57149=CARTESIAN_POINT('Ctrl Pts',(-0.786322922920599,1.,-3.66663282329846));
#57150=CARTESIAN_POINT('',(-0.732042837400619,1.,-4.13571194405636));
#57151=CARTESIAN_POINT('Ctrl Pts',(-0.732042837400619,1.,-4.13571194405636));
#57152=CARTESIAN_POINT('Ctrl Pts',(-0.732488575135926,1.,-4.13420383737278));
#57153=CARTESIAN_POINT('Ctrl Pts',(-0.733376589325634,1.,-4.13118752796397));
#57154=CARTESIAN_POINT('Ctrl Pts',(-0.734698226767512,1.,-4.12666277572794));
#57155=CARTESIAN_POINT('Ctrl Pts',(-0.736439634335347,1.,-4.12062919626082));
#57156=CARTESIAN_POINT('Ctrl Pts',(-0.738581708229119,1.,-4.11308626953795));
#57157=CARTESIAN_POINT('Ctrl Pts',(-0.740688998555152,1.,-4.1055424175856));
#57158=CARTESIAN_POINT('Ctrl Pts',(-0.742761369690018,1.,-4.09799769702712));
#57159=CARTESIAN_POINT('Ctrl Pts',(-0.744798649705514,1.,-4.09045220253011));
#57160=CARTESIAN_POINT('Ctrl Pts',(-0.746800631490822,1.,-4.08290608094789));
#57161=CARTESIAN_POINT('Ctrl Pts',(-0.748767076679177,1.,-4.07535951055363));
#57162=CARTESIAN_POINT('Ctrl Pts',(-0.750697720483176,1.,-4.06781267241886));
#57163=CARTESIAN_POINT('Ctrl Pts',(-0.752592276482869,1.,-4.06026572221399));
#57164=CARTESIAN_POINT('Ctrl Pts',(-0.754450441816412,1.,-4.05271876688106));
#57165=CARTESIAN_POINT('Ctrl Pts',(-0.756271902370187,1.,-4.04517182654344));
#57166=CARTESIAN_POINT('Ctrl Pts',(-0.758056338885554,1.,-4.03762485803468));
#57167=CARTESIAN_POINT('Ctrl Pts',(-0.759803433244166,1.,-4.0300778195465));
#57168=CARTESIAN_POINT('Ctrl Pts',(-0.761512875859942,1.,-4.02253072741347));
#57169=CARTESIAN_POINT('Ctrl Pts',(-0.763184371182827,1.,-4.01498370680434));
#57170=CARTESIAN_POINT('Ctrl Pts',(-0.764817648784946,1.,-4.00743706791366));
#57171=CARTESIAN_POINT('Ctrl Pts',(-0.766412457135786,1.,-3.99989129179464));
#57172=CARTESIAN_POINT('Ctrl Pts',(-0.767968531377708,1.,-3.99234687880892));
#57173=CARTESIAN_POINT('Ctrl Pts',(-0.769485566245459,1.,-3.98480422348403));
#57174=CARTESIAN_POINT('Ctrl Pts',(-0.770963190030504,1.,-3.97726349165507));
#57175=CARTESIAN_POINT('Ctrl Pts',(-0.772400931772239,1.,-3.96972446532832));
#57176=CARTESIAN_POINT('Ctrl Pts',(-0.773798212026683,1.,-3.96218649639876));
#57177=CARTESIAN_POINT('Ctrl Pts',(-0.775154418039441,1.,-3.95464885452364));
#57178=CARTESIAN_POINT('Ctrl Pts',(-0.77646896669796,1.,-3.94711101619471));
#57179=CARTESIAN_POINT('Ctrl Pts',(-0.77774137056855,1.,-3.93957296768098));
#57180=CARTESIAN_POINT('Ctrl Pts',(-0.778971308134786,1.,-3.93203552473153));
#57181=CARTESIAN_POINT('Ctrl Pts',(-0.780158678615507,1.,-3.92450058323799));
#57182=CARTESIAN_POINT('Ctrl Pts',(-0.781303428618344,1.,-3.9169703605466));
#57183=CARTESIAN_POINT('Ctrl Pts',(-0.782405395622759,1.,-3.90944671004536));
#57184=CARTESIAN_POINT('Ctrl Pts',(-0.783464141529082,1.,-3.90193039043971));
#57185=CARTESIAN_POINT('Ctrl Pts',(-0.784478799358336,1.,-3.89442039235105));
#57186=CARTESIAN_POINT('Ctrl Pts',(-0.785447890340723,1.,-3.88691313167399));
#57187=CARTESIAN_POINT('Ctrl Pts',(-0.786369675812592,1.,-3.87940402818186));
#57188=CARTESIAN_POINT('Ctrl Pts',(-0.78724252761798,1.,-3.87188916600905));
#57189=CARTESIAN_POINT('Ctrl Pts',(-0.788065315093771,1.,-3.86436702561342));
#57190=CARTESIAN_POINT('Ctrl Pts',(-0.788837734090688,1.,-3.85683995872536));
#57191=CARTESIAN_POINT('Ctrl Pts',(-0.789560798155619,1.,-3.8493163780891));
#57192=CARTESIAN_POINT('Ctrl Pts',(-0.790236124191289,1.,-3.84180762342476));
#57193=CARTESIAN_POINT('Ctrl Pts',(-0.79086501270534,1.,-3.83432392054804));
#57194=CARTESIAN_POINT('Ctrl Pts',(-0.791447528662381,1.,-3.82687033899799));
#57195=CARTESIAN_POINT('Ctrl Pts',(-0.791981740718606,1.,-3.81944345442237));
#57196=CARTESIAN_POINT('Ctrl Pts',(-0.792462483517568,1.,-3.81202588694726));
#57197=CARTESIAN_POINT('Ctrl Pts',(-0.792882695234693,1.,-3.80459229925598));
#57198=CARTESIAN_POINT('Ctrl Pts',(-0.7932356129732,1.,-3.79711921389862));
#57199=CARTESIAN_POINT('Ctrl Pts',(-0.793516871680966,1.,-3.78959439439222));
#57200=CARTESIAN_POINT('Ctrl Pts',(-0.793726235781339,1.,-3.78202460377617));
#57201=CARTESIAN_POINT('Ctrl Pts',(-0.793870523787515,1.,-3.77444863801264));
#57202=CARTESIAN_POINT('Ctrl Pts',(-0.793961083689141,1.,-3.76692626931184));
#57203=CARTESIAN_POINT('Ctrl Pts',(-0.794008429135047,1.,-3.75951468666325));
#57204=CARTESIAN_POINT('Ctrl Pts',(-0.794017347371441,1.,-3.75224692493895));
#57205=CARTESIAN_POINT('Ctrl Pts',(-0.79398270045988,1.,-3.74511357728827));
#57206=CARTESIAN_POINT('Ctrl Pts',(-0.79388270093679,1.,-3.73803280541576));
#57207=CARTESIAN_POINT('Ctrl Pts',(-0.793682750269347,1.,-3.7308691469564));
#57208=CARTESIAN_POINT('Ctrl Pts',(-0.79334702378387,1.,-3.7234879729357));
#57209=CARTESIAN_POINT('Ctrl Pts',(-0.792848377370115,1.,-3.7158024239604));
#57210=CARTESIAN_POINT('Ctrl Pts',(-0.792177688845968,1.,-3.70781724021879));
#57211=CARTESIAN_POINT('Ctrl Pts',(-0.791356575696509,1.,-3.69968940808982));
#57212=CARTESIAN_POINT('Ctrl Pts',(-0.79043628498958,1.,-3.69172044327754));
#57213=CARTESIAN_POINT('Ctrl Pts',(-0.789483546065158,1.,-3.68428439784285));
#57214=CARTESIAN_POINT('Ctrl Pts',(-0.788569566220662,1.,-3.67777119516438));
#57215=CARTESIAN_POINT('Ctrl Pts',(-0.787758799995426,1.,-3.672529236635));
#57216=CARTESIAN_POINT('Ctrl Pts',(-0.787145041181589,1.,-3.66907505398769));
#57217=CARTESIAN_POINT('Ctrl Pts',(-0.7867743371985,1.,-3.66743103898844));
#57218=CARTESIAN_POINT('Ctrl Pts',(-0.78656591955989,1.,-3.66680946938396));
#57219=CARTESIAN_POINT('Ctrl Pts',(-0.786459983896781,1.,-3.66664310415236));
#57220=CARTESIAN_POINT('Ctrl Pts',(-0.786422660833743,1.,-3.66661143271648));
#57221=CARTESIAN_POINT('',(-0.732042837400619,0.,-4.13571194405636));
#57222=CARTESIAN_POINT('Ctrl Pts',(-0.385214314776329,-1.,-3.73016218570874));
#57223=CARTESIAN_POINT('Ctrl Pts',(-0.385214314776329,1.,-3.73016218570874));
#57224=CARTESIAN_POINT('Ctrl Pts',(-0.385147278814804,-1.,-3.73010668803185));
#57225=CARTESIAN_POINT('Ctrl Pts',(-0.385147278814804,1.,-3.73010668803185));
#57226=CARTESIAN_POINT('Ctrl Pts',(-0.385047711603887,-1.,-3.73015851028729));
#57227=CARTESIAN_POINT('Ctrl Pts',(-0.385047711603887,1.,-3.73015851028729));
#57228=CARTESIAN_POINT('Ctrl Pts',(-0.385001870183841,-1.,-3.73072465900727));
#57229=CARTESIAN_POINT('Ctrl Pts',(-0.385001870183841,1.,-3.73072465900727));
#57230=CARTESIAN_POINT('Ctrl Pts',(-0.385147887989515,-1.,-3.73245705639337));
#57231=CARTESIAN_POINT('Ctrl Pts',(-0.385147887989515,1.,-3.73245705639337));
#57232=CARTESIAN_POINT('Ctrl Pts',(-0.385670806454744,-1.,-3.73621371845475));
#57233=CARTESIAN_POINT('Ctrl Pts',(-0.385670806454744,1.,-3.73621371845475));
#57234=CARTESIAN_POINT('Ctrl Pts',(-0.386519576222035,-1.,-3.74144965781088));
#57235=CARTESIAN_POINT('Ctrl Pts',(-0.386519576222035,1.,-3.74144965781088));
#57236=CARTESIAN_POINT('Ctrl Pts',(-0.387663020050396,-1.,-3.74792651696269));
#57237=CARTESIAN_POINT('Ctrl Pts',(-0.387663020050396,1.,-3.74792651696269));
#57238=CARTESIAN_POINT('Ctrl Pts',(-0.389054775898251,-1.,-3.75529302894757));
#57239=CARTESIAN_POINT('Ctrl Pts',(-0.389054775898251,1.,-3.75529302894757));
#57240=CARTESIAN_POINT('Ctrl Pts',(-0.390642072979259,-1.,-3.76315635032993));
#57241=CARTESIAN_POINT('Ctrl Pts',(-0.390642072979259,1.,-3.76315635032993));
#57242=CARTESIAN_POINT('Ctrl Pts',(-0.392372786223347,-1.,-3.77114011595892));
#57243=CARTESIAN_POINT('Ctrl Pts',(-0.392372786223347,1.,-3.77114011595892));
#57244=CARTESIAN_POINT('Ctrl Pts',(-0.394202481011595,-1.,-3.77894173114368));
#57245=CARTESIAN_POINT('Ctrl Pts',(-0.394202481011595,1.,-3.77894173114368));
#57246=CARTESIAN_POINT('Ctrl Pts',(-0.396103205335029,-1.,-3.78640521279479));
#57247=CARTESIAN_POINT('Ctrl Pts',(-0.396103205335029,1.,-3.78640521279479));
#57248=CARTESIAN_POINT('Ctrl Pts',(-0.398064818684158,-1.,-3.79352887163457));
#57249=CARTESIAN_POINT('Ctrl Pts',(-0.398064818684158,1.,-3.79352887163457));
#57250=CARTESIAN_POINT('Ctrl Pts',(-0.400088346504727,-1.,-3.80040370384659));
#57251=CARTESIAN_POINT('Ctrl Pts',(-0.400088346504727,1.,-3.80040370384659));
#57252=CARTESIAN_POINT('Ctrl Pts',(-0.402181320148475,-1.,-3.80716881962763));
#57253=CARTESIAN_POINT('Ctrl Pts',(-0.402181320148475,1.,-3.80716881962763));
#57254=CARTESIAN_POINT('Ctrl Pts',(-0.404352694628236,-1.,-3.81396374287762));
#57255=CARTESIAN_POINT('Ctrl Pts',(-0.404352694628236,1.,-3.81396374287762));
#57256=CARTESIAN_POINT('Ctrl Pts',(-0.406607038258906,-1.,-3.82087303913741));
#57257=CARTESIAN_POINT('Ctrl Pts',(-0.406607038258906,1.,-3.82087303913741));
#57258=CARTESIAN_POINT('Ctrl Pts',(-0.408942371447377,-1.,-3.82790724256397));
#57259=CARTESIAN_POINT('Ctrl Pts',(-0.408942371447377,1.,-3.82790724256397));
#57260=CARTESIAN_POINT('Ctrl Pts',(-0.41135303879846,-1.,-3.83503345578645));
#57261=CARTESIAN_POINT('Ctrl Pts',(-0.41135303879846,1.,-3.83503345578645));
#57262=CARTESIAN_POINT('Ctrl Pts',(-0.413831367016727,-1.,-3.84219403994742));
#57263=CARTESIAN_POINT('Ctrl Pts',(-0.413831367016727,1.,-3.84219403994742));
#57264=CARTESIAN_POINT('Ctrl Pts',(-0.41636967805292,-1.,-3.8493286415751));
#57265=CARTESIAN_POINT('Ctrl Pts',(-0.41636967805292,1.,-3.8493286415751));
#57266=CARTESIAN_POINT('Ctrl Pts',(-0.41896246808681,-1.,-3.85639825648031));
#57267=CARTESIAN_POINT('Ctrl Pts',(-0.41896246808681,1.,-3.85639825648031));
#57268=CARTESIAN_POINT('Ctrl Pts',(-0.421607423177576,-1.,-3.86339652542749));
#57269=CARTESIAN_POINT('Ctrl Pts',(-0.421607423177576,1.,-3.86339652542749));
#57270=CARTESIAN_POINT('Ctrl Pts',(-0.424304173195142,-1.,-3.87033643487882));
#57271=CARTESIAN_POINT('Ctrl Pts',(-0.424304173195142,1.,-3.87033643487882));
#57272=CARTESIAN_POINT('Ctrl Pts',(-0.427053541173469,-1.,-3.87724240306609));
#57273=CARTESIAN_POINT('Ctrl Pts',(-0.427053541173469,1.,-3.87724240306609));
#57274=CARTESIAN_POINT('Ctrl Pts',(-0.429856640579734,-1.,-3.88414070943334));
#57275=CARTESIAN_POINT('Ctrl Pts',(-0.429856640579734,1.,-3.88414070943334));
#57276=CARTESIAN_POINT('Ctrl Pts',(-0.432713929544439,-1.,-3.89104947940592));
#57277=CARTESIAN_POINT('Ctrl Pts',(-0.432713929544439,1.,-3.89104947940592));
#57278=CARTESIAN_POINT('Ctrl Pts',(-0.435624629433506,-1.,-3.8979725665544));
#57279=CARTESIAN_POINT('Ctrl Pts',(-0.435624629433506,1.,-3.8979725665544));
#57280=CARTESIAN_POINT('Ctrl Pts',(-0.438587235458233,-1.,-3.90490512938546));
#57281=CARTESIAN_POINT('Ctrl Pts',(-0.438587235458233,1.,-3.90490512938546));
#57282=CARTESIAN_POINT('Ctrl Pts',(-0.441599824524047,-1.,-3.91183704069146));
#57283=CARTESIAN_POINT('Ctrl Pts',(-0.441599824524047,1.,-3.91183704069146));
#57284=CARTESIAN_POINT('Ctrl Pts',(-0.444660430230593,-1.,-3.91875701610721));
#57285=CARTESIAN_POINT('Ctrl Pts',(-0.444660430230593,1.,-3.91875701610721));
#57286=CARTESIAN_POINT('Ctrl Pts',(-0.447767416837297,-1.,-3.92565674143424));
#57287=CARTESIAN_POINT('Ctrl Pts',(-0.447767416837297,1.,-3.92565674143424));
#57288=CARTESIAN_POINT('Ctrl Pts',(-0.450919768356347,-1.,-3.93253407403128));
#57289=CARTESIAN_POINT('Ctrl Pts',(-0.450919768356347,1.,-3.93253407403128));
#57290=CARTESIAN_POINT('Ctrl Pts',(-0.454116879027576,-1.,-3.93939080846298));
#57291=CARTESIAN_POINT('Ctrl Pts',(-0.454116879027576,1.,-3.93939080846298));
#57292=CARTESIAN_POINT('Ctrl Pts',(-0.457358410451674,-1.,-3.94623117206675));
#57293=CARTESIAN_POINT('Ctrl Pts',(-0.457358410451674,1.,-3.94623117206675));
#57294=CARTESIAN_POINT('Ctrl Pts',(-0.460644124429119,-1.,-3.95306005817363));
#57295=CARTESIAN_POINT('Ctrl Pts',(-0.460644124429119,1.,-3.95306005817363));
#57296=CARTESIAN_POINT('Ctrl Pts',(-0.463973722115744,-1.,-3.95988133243543));
#57297=CARTESIAN_POINT('Ctrl Pts',(-0.463973722115744,1.,-3.95988133243543));
#57298=CARTESIAN_POINT('Ctrl Pts',(-0.467346690880672,-1.,-3.96669622273946));
#57299=CARTESIAN_POINT('Ctrl Pts',(-0.467346690880672,1.,-3.96669622273946));
#57300=CARTESIAN_POINT('Ctrl Pts',(-0.470762379613477,-1.,-3.97350414289415));
#57301=CARTESIAN_POINT('Ctrl Pts',(-0.470762379613477,1.,-3.97350414289415));
#57302=CARTESIAN_POINT('Ctrl Pts',(-0.474220061019542,-1.,-3.9803033804443));
#57303=CARTESIAN_POINT('Ctrl Pts',(-0.474220061019542,1.,-3.9803033804443));
#57304=CARTESIAN_POINT('Ctrl Pts',(-0.477718999122033,-1.,-3.98709184306743));
#57305=CARTESIAN_POINT('Ctrl Pts',(-0.477718999122033,1.,-3.98709184306743));
#57306=CARTESIAN_POINT('Ctrl Pts',(-0.481258512209638,-1.,-3.99386775880655));
#57307=CARTESIAN_POINT('Ctrl Pts',(-0.481258512209638,1.,-3.99386775880655));
#57308=CARTESIAN_POINT('Ctrl Pts',(-0.484838042421754,-1.,-4.00063045119234));
#57309=CARTESIAN_POINT('Ctrl Pts',(-0.484838042421754,1.,-4.00063045119234));
#57310=CARTESIAN_POINT('Ctrl Pts',(-0.488457130424531,-1.,-4.0073800839092));
#57311=CARTESIAN_POINT('Ctrl Pts',(-0.488457130424531,1.,-4.0073800839092));
#57312=CARTESIAN_POINT('Ctrl Pts',(-0.492115383417931,-1.,-4.01411733503486));
#57313=CARTESIAN_POINT('Ctrl Pts',(-0.492115383417931,1.,-4.01411733503486));
#57314=CARTESIAN_POINT('Ctrl Pts',(-0.495812444326223,-1.,-4.02084308851813));
#57315=CARTESIAN_POINT('Ctrl Pts',(-0.495812444326223,1.,-4.02084308851813));
#57316=CARTESIAN_POINT('Ctrl Pts',(-0.49954796234089,-1.,-4.0275581398015));
#57317=CARTESIAN_POINT('Ctrl Pts',(-0.49954796234089,1.,-4.0275581398015));
#57318=CARTESIAN_POINT('Ctrl Pts',(-0.503321556915514,-1.,-4.0342628417439));
#57319=CARTESIAN_POINT('Ctrl Pts',(-0.503321556915514,1.,-4.0342628417439));
#57320=CARTESIAN_POINT('Ctrl Pts',(-0.507132823288362,-1.,-4.04095715149074));
#57321=CARTESIAN_POINT('Ctrl Pts',(-0.507132823288362,1.,-4.04095715149074));
#57322=CARTESIAN_POINT('Ctrl Pts',(-0.510981349219174,-1.,-4.04764078815591));
#57323=CARTESIAN_POINT('Ctrl Pts',(-0.510981349219174,1.,-4.04764078815591));
#57324=CARTESIAN_POINT('Ctrl Pts',(-0.514866728193104,-1.,-4.05431335771261));
#57325=CARTESIAN_POINT('Ctrl Pts',(-0.514866728193104,1.,-4.05431335771261));
#57326=CARTESIAN_POINT('Ctrl Pts',(-0.51878857233681,-1.,-4.06097448037934));
#57327=CARTESIAN_POINT('Ctrl Pts',(-0.51878857233681,1.,-4.06097448037934));
#57328=CARTESIAN_POINT('Ctrl Pts',(-0.522746528602768,-1.,-4.06762394471075));
#57329=CARTESIAN_POINT('Ctrl Pts',(-0.522746528602768,1.,-4.06762394471075));
#57330=CARTESIAN_POINT('Ctrl Pts',(-0.526740277227,-1.,-4.07426172299496));
#57331=CARTESIAN_POINT('Ctrl Pts',(-0.526740277227,1.,-4.07426172299496));
#57332=CARTESIAN_POINT('Ctrl Pts',(-0.530769518728075,-1.,-4.08088789536488));
#57333=CARTESIAN_POINT('Ctrl Pts',(-0.530769518728075,1.,-4.08088789536488));
#57334=CARTESIAN_POINT('Ctrl Pts',(-0.534833963476999,-1.,-4.08750259988693));
#57335=CARTESIAN_POINT('Ctrl Pts',(-0.534833963476999,1.,-4.08750259988693));
#57336=CARTESIAN_POINT('Ctrl Pts',(-0.538933321179921,-1.,-4.09410597627116));
#57337=CARTESIAN_POINT('Ctrl Pts',(-0.538933321179921,1.,-4.09410597627116));
#57338=CARTESIAN_POINT('Ctrl Pts',(-0.543067286878457,-1.,-4.10069810244473));
#57339=CARTESIAN_POINT('Ctrl Pts',(-0.543067286878457,1.,-4.10069810244473));
#57340=CARTESIAN_POINT('Ctrl Pts',(-0.54723553948676,-1.,-4.1072789702877));
#57341=CARTESIAN_POINT('Ctrl Pts',(-0.54723553948676,1.,-4.1072789702877));
#57342=CARTESIAN_POINT('Ctrl Pts',(-0.551437758498247,-1.,-4.11384852025578));
#57343=CARTESIAN_POINT('Ctrl Pts',(-0.551437758498247,1.,-4.11384852025578));
#57344=CARTESIAN_POINT('Ctrl Pts',(-0.555673636130778,-1.,-4.1204066619623));
#57345=CARTESIAN_POINT('Ctrl Pts',(-0.555673636130778,1.,-4.1204066619623));
#57346=CARTESIAN_POINT('Ctrl Pts',(-0.559942890594628,-1.,-4.12695329951859));
#57347=CARTESIAN_POINT('Ctrl Pts',(-0.559942890594628,1.,-4.12695329951859));
#57348=CARTESIAN_POINT('Ctrl Pts',(-0.564245279535705,-1.,-4.13348835726086));
#57349=CARTESIAN_POINT('Ctrl Pts',(-0.564245279535705,1.,-4.13348835726086));
#57350=CARTESIAN_POINT('Ctrl Pts',(-0.568580610187116,-1.,-4.14001179828669));
#57351=CARTESIAN_POINT('Ctrl Pts',(-0.568580610187116,1.,-4.14001179828669));
#57352=CARTESIAN_POINT('Ctrl Pts',(-0.572948736066277,-1.,-4.14652361065787));
#57353=CARTESIAN_POINT('Ctrl Pts',(-0.572948736066277,1.,-4.14652361065787));
#57354=CARTESIAN_POINT('Ctrl Pts',(-0.576469391673917,-1.,-4.1517237611974));
#57355=CARTESIAN_POINT('Ctrl Pts',(-0.576469391673917,1.,-4.1517237611974));
#57356=CARTESIAN_POINT('Ctrl Pts',(-0.579124568912543,-1.,-4.15561864787379));
#57357=CARTESIAN_POINT('Ctrl Pts',(-0.579124568912543,1.,-4.15561864787379));
#57358=CARTESIAN_POINT('Ctrl Pts',(-0.580901211462913,-1.,-4.15821291712391));
#57359=CARTESIAN_POINT('Ctrl Pts',(-0.580901211462913,1.,-4.15821291712391));
#57360=CARTESIAN_POINT('Ctrl Pts',(-0.581791163835814,-1.,-4.15950947128175));
#57361=CARTESIAN_POINT('Ctrl Pts',(-0.581791163835814,1.,-4.15950947128175));
#57362=CARTESIAN_POINT('',(-0.385112848332548,1.,-3.73017266276632));
#57363=CARTESIAN_POINT('Ctrl Pts',(-0.385112848332549,-1.,-3.73017266276632));
#57364=CARTESIAN_POINT('Ctrl Pts',(-0.385112848332549,-0.666666666666667,
-3.73017266276632));
#57365=CARTESIAN_POINT('Ctrl Pts',(-0.385112848332549,-0.333333333333333,
-3.73017266276632));
#57366=CARTESIAN_POINT('Ctrl Pts',(-0.385112848332549,0.333333333333333,
-3.73017266276632));
#57367=CARTESIAN_POINT('Ctrl Pts',(-0.385112848332549,0.666666666666667,
-3.73017266276632));
#57368=CARTESIAN_POINT('Ctrl Pts',(-0.385112848332549,1.,-3.73017266276632));
#57369=CARTESIAN_POINT('',(-0.581791163835814,1.,-4.15950947128175));
#57370=CARTESIAN_POINT('',(-0.581791163835814,0.,-4.15950947128175));
#57371=CARTESIAN_POINT('Ctrl Pts',(-0.385112848332549,1.,-3.73017266276632));
#57372=CARTESIAN_POINT('Ctrl Pts',(-0.385087139001609,1.,-3.73021431755218));
#57373=CARTESIAN_POINT('Ctrl Pts',(-0.385037797882046,1.,-3.73040527620929));
#57374=CARTESIAN_POINT('Ctrl Pts',(-0.385031656499142,1.,-3.731060828624));
#57375=CARTESIAN_POINT('Ctrl Pts',(-0.385187124633965,1.,-3.73273893363318));
#57376=CARTESIAN_POINT('Ctrl Pts',(-0.385670806454744,1.,-3.73621371845475));
#57377=CARTESIAN_POINT('Ctrl Pts',(-0.386519576222035,1.,-3.74144965781088));
#57378=CARTESIAN_POINT('Ctrl Pts',(-0.387663020050396,1.,-3.74792651696269));
#57379=CARTESIAN_POINT('Ctrl Pts',(-0.389054775898251,1.,-3.75529302894757));
#57380=CARTESIAN_POINT('Ctrl Pts',(-0.390642072979259,1.,-3.76315635032993));
#57381=CARTESIAN_POINT('Ctrl Pts',(-0.392372786223347,1.,-3.77114011595892));
#57382=CARTESIAN_POINT('Ctrl Pts',(-0.394202481011595,1.,-3.77894173114368));
#57383=CARTESIAN_POINT('Ctrl Pts',(-0.396103205335029,1.,-3.78640521279479));
#57384=CARTESIAN_POINT('Ctrl Pts',(-0.398064818684158,1.,-3.79352887163457));
#57385=CARTESIAN_POINT('Ctrl Pts',(-0.400088346504727,1.,-3.80040370384659));
#57386=CARTESIAN_POINT('Ctrl Pts',(-0.402181320148475,1.,-3.80716881962763));
#57387=CARTESIAN_POINT('Ctrl Pts',(-0.404352694628236,1.,-3.81396374287762));
#57388=CARTESIAN_POINT('Ctrl Pts',(-0.406607038258906,1.,-3.82087303913741));
#57389=CARTESIAN_POINT('Ctrl Pts',(-0.408942371447377,1.,-3.82790724256397));
#57390=CARTESIAN_POINT('Ctrl Pts',(-0.41135303879846,1.,-3.83503345578645));
#57391=CARTESIAN_POINT('Ctrl Pts',(-0.413831367016727,1.,-3.84219403994742));
#57392=CARTESIAN_POINT('Ctrl Pts',(-0.41636967805292,1.,-3.8493286415751));
#57393=CARTESIAN_POINT('Ctrl Pts',(-0.41896246808681,1.,-3.85639825648031));
#57394=CARTESIAN_POINT('Ctrl Pts',(-0.421607423177576,1.,-3.86339652542749));
#57395=CARTESIAN_POINT('Ctrl Pts',(-0.424304173195142,1.,-3.87033643487882));
#57396=CARTESIAN_POINT('Ctrl Pts',(-0.427053541173469,1.,-3.87724240306609));
#57397=CARTESIAN_POINT('Ctrl Pts',(-0.429856640579734,1.,-3.88414070943334));
#57398=CARTESIAN_POINT('Ctrl Pts',(-0.432713929544439,1.,-3.89104947940592));
#57399=CARTESIAN_POINT('Ctrl Pts',(-0.435624629433506,1.,-3.8979725665544));
#57400=CARTESIAN_POINT('Ctrl Pts',(-0.438587235458233,1.,-3.90490512938546));
#57401=CARTESIAN_POINT('Ctrl Pts',(-0.441599824524047,1.,-3.91183704069146));
#57402=CARTESIAN_POINT('Ctrl Pts',(-0.444660430230593,1.,-3.91875701610721));
#57403=CARTESIAN_POINT('Ctrl Pts',(-0.447767416837297,1.,-3.92565674143424));
#57404=CARTESIAN_POINT('Ctrl Pts',(-0.450919768356347,1.,-3.93253407403128));
#57405=CARTESIAN_POINT('Ctrl Pts',(-0.454116879027576,1.,-3.93939080846298));
#57406=CARTESIAN_POINT('Ctrl Pts',(-0.457358410451674,1.,-3.94623117206675));
#57407=CARTESIAN_POINT('Ctrl Pts',(-0.460644124429119,1.,-3.95306005817363));
#57408=CARTESIAN_POINT('Ctrl Pts',(-0.463973722115744,1.,-3.95988133243543));
#57409=CARTESIAN_POINT('Ctrl Pts',(-0.467346690880672,1.,-3.96669622273946));
#57410=CARTESIAN_POINT('Ctrl Pts',(-0.470762379613477,1.,-3.97350414289415));
#57411=CARTESIAN_POINT('Ctrl Pts',(-0.474220061019542,1.,-3.9803033804443));
#57412=CARTESIAN_POINT('Ctrl Pts',(-0.477718999122033,1.,-3.98709184306743));
#57413=CARTESIAN_POINT('Ctrl Pts',(-0.481258512209638,1.,-3.99386775880655));
#57414=CARTESIAN_POINT('Ctrl Pts',(-0.484838042421754,1.,-4.00063045119234));
#57415=CARTESIAN_POINT('Ctrl Pts',(-0.488457130424531,1.,-4.0073800839092));
#57416=CARTESIAN_POINT('Ctrl Pts',(-0.492115383417931,1.,-4.01411733503486));
#57417=CARTESIAN_POINT('Ctrl Pts',(-0.495812444326223,1.,-4.02084308851813));
#57418=CARTESIAN_POINT('Ctrl Pts',(-0.49954796234089,1.,-4.0275581398015));
#57419=CARTESIAN_POINT('Ctrl Pts',(-0.503321556915514,1.,-4.0342628417439));
#57420=CARTESIAN_POINT('Ctrl Pts',(-0.507132823288362,1.,-4.04095715149074));
#57421=CARTESIAN_POINT('Ctrl Pts',(-0.510981349219174,1.,-4.04764078815591));
#57422=CARTESIAN_POINT('Ctrl Pts',(-0.514866728193104,1.,-4.05431335771261));
#57423=CARTESIAN_POINT('Ctrl Pts',(-0.51878857233681,1.,-4.06097448037934));
#57424=CARTESIAN_POINT('Ctrl Pts',(-0.522746528602768,1.,-4.06762394471075));
#57425=CARTESIAN_POINT('Ctrl Pts',(-0.526740277227,1.,-4.07426172299496));
#57426=CARTESIAN_POINT('Ctrl Pts',(-0.530769518728075,1.,-4.08088789536488));
#57427=CARTESIAN_POINT('Ctrl Pts',(-0.534833963476999,1.,-4.08750259988693));
#57428=CARTESIAN_POINT('Ctrl Pts',(-0.538933321179921,1.,-4.09410597627116));
#57429=CARTESIAN_POINT('Ctrl Pts',(-0.543067286878457,1.,-4.10069810244473));
#57430=CARTESIAN_POINT('Ctrl Pts',(-0.54723553948676,1.,-4.1072789702877));
#57431=CARTESIAN_POINT('Ctrl Pts',(-0.551437758498247,1.,-4.11384852025578));
#57432=CARTESIAN_POINT('Ctrl Pts',(-0.555673636130778,1.,-4.1204066619623));
#57433=CARTESIAN_POINT('Ctrl Pts',(-0.559942890594628,1.,-4.12695329951859));
#57434=CARTESIAN_POINT('Ctrl Pts',(-0.564245279535705,1.,-4.13348835726086));
#57435=CARTESIAN_POINT('Ctrl Pts',(-0.568580610187116,1.,-4.14001179828669));
#57436=CARTESIAN_POINT('Ctrl Pts',(-0.572948736066277,1.,-4.14652361065787));
#57437=CARTESIAN_POINT('Ctrl Pts',(-0.576469391673917,1.,-4.1517237611974));
#57438=CARTESIAN_POINT('Ctrl Pts',(-0.579124568912543,1.,-4.15561864787379));
#57439=CARTESIAN_POINT('Ctrl Pts',(-0.580901211462913,1.,-4.15821291712391));
#57440=CARTESIAN_POINT('Ctrl Pts',(-0.581791163835814,1.,-4.15950947128175));
#57441=CARTESIAN_POINT('Origin',(-0.581791163835814,0.,-4.15950947128175));
#57442=CARTESIAN_POINT('',(-0.732042837400619,1.,-4.13571194405636));
#57443=CARTESIAN_POINT('Origin',(0.,0.,0.));
#57444=CARTESIAN_POINT('',(-0.203156094897896,1.,-3.74449296982994));
#57445=CARTESIAN_POINT('Origin',(0.,1.,0.));
#57446=CARTESIAN_POINT('Ctrl Pts',(-0.203156094897896,1.,-3.74449296982994));
#57447=CARTESIAN_POINT('Ctrl Pts',(-0.203156094897896,0.666666666666667,
-3.74449296982994));
#57448=CARTESIAN_POINT('Ctrl Pts',(-0.203156094897896,0.333333333333333,
-3.74449296982994));
#57449=CARTESIAN_POINT('Ctrl Pts',(-0.203156094897896,-0.333333333333333,
-3.74449296982994));
#57450=CARTESIAN_POINT('Ctrl Pts',(-0.203156094897896,-0.666666666666667,
-3.74449296982994));
#57451=CARTESIAN_POINT('Ctrl Pts',(-0.203156094897896,-1.,-3.74449296982994));
#57452=CARTESIAN_POINT('Ctrl Pts',(-0.0760622897878238,-1.,-4.19931119685982));
#57453=CARTESIAN_POINT('Ctrl Pts',(-0.0760622897878238,1.,-4.19931119685982));
#57454=CARTESIAN_POINT('Ctrl Pts',(-0.0767384596142197,-1.,-4.19789138621624));
#57455=CARTESIAN_POINT('Ctrl Pts',(-0.0767384596142197,1.,-4.19789138621624));
#57456=CARTESIAN_POINT('Ctrl Pts',(-0.0780873956244405,-1.,-4.19505112860624));
#57457=CARTESIAN_POINT('Ctrl Pts',(-0.0780873956244405,1.,-4.19505112860624));
#57458=CARTESIAN_POINT('Ctrl Pts',(-0.0801005887117605,-1.,-4.19078883322483));
#57459=CARTESIAN_POINT('Ctrl Pts',(-0.0801005887117605,1.,-4.19078883322483));
#57460=CARTESIAN_POINT('Ctrl Pts',(-0.0827644164389512,-1.,-4.1851019532944));
#57461=CARTESIAN_POINT('Ctrl Pts',(-0.0827644164389512,1.,-4.1851019532944));
#57462=CARTESIAN_POINT('Ctrl Pts',(-0.0860600915552517,-1.,-4.17798698669991));
#57463=CARTESIAN_POINT('Ctrl Pts',(-0.0860600915552517,1.,-4.17798698669991));
#57464=CARTESIAN_POINT('Ctrl Pts',(-0.089321556085033,-1.,-4.17086566491823));
#57465=CARTESIAN_POINT('Ctrl Pts',(-0.089321556085033,1.,-4.17086566491823));
#57466=CARTESIAN_POINT('Ctrl Pts',(-0.0925486672167692,-1.,-4.16373802265942));
#57467=CARTESIAN_POINT('Ctrl Pts',(-0.0925486672167692,1.,-4.16373802265942));
#57468=CARTESIAN_POINT('Ctrl Pts',(-0.095741240329707,-1.,-4.15660412653006));
#57469=CARTESIAN_POINT('Ctrl Pts',(-0.095741240329707,1.,-4.15660412653006));
#57470=CARTESIAN_POINT('Ctrl Pts',(-0.0988990478899814,-1.,-4.1494640891762));
#57471=CARTESIAN_POINT('Ctrl Pts',(-0.0988990478899814,1.,-4.1494640891762));
#57472=CARTESIAN_POINT('Ctrl Pts',(-0.102021826577454,-1.,-4.14231804938737));
#57473=CARTESIAN_POINT('Ctrl Pts',(-0.102021826577454,1.,-4.14231804938737));
#57474=CARTESIAN_POINT('Ctrl Pts',(-0.105109286538864,-1.,-4.13516614458396));
#57475=CARTESIAN_POINT('Ctrl Pts',(-0.105109286538864,1.,-4.13516614458396));
#57476=CARTESIAN_POINT('Ctrl Pts',(-0.10816112052835,-1.,-4.12800848371386));
#57477=CARTESIAN_POINT('Ctrl Pts',(-0.10816112052835,1.,-4.12800848371386));
#57478=CARTESIAN_POINT('Ctrl Pts',(-0.111177012683377,-1.,-4.12084512502444));
#57479=CARTESIAN_POINT('Ctrl Pts',(-0.111177012683377,1.,-4.12084512502444));
#57480=CARTESIAN_POINT('Ctrl Pts',(-0.114156649609602,-1.,-4.11367603925313));
#57481=CARTESIAN_POINT('Ctrl Pts',(-0.114156649609602,1.,-4.11367603925313));
#57482=CARTESIAN_POINT('Ctrl Pts',(-0.117099722731705,-1.,-4.10650113382187));
#57483=CARTESIAN_POINT('Ctrl Pts',(-0.117099722731705,1.,-4.10650113382187));
#57484=CARTESIAN_POINT('Ctrl Pts',(-0.120005924388162,-1.,-4.09932031767243));
#57485=CARTESIAN_POINT('Ctrl Pts',(-0.120005924388162,1.,-4.09932031767243));
#57486=CARTESIAN_POINT('Ctrl Pts',(-0.122874946249119,-1.,-4.09213355850836));
#57487=CARTESIAN_POINT('Ctrl Pts',(-0.122874946249119,1.,-4.09213355850836));
#57488=CARTESIAN_POINT('Ctrl Pts',(-0.125706476822529,-1.,-4.08494093372315));
#57489=CARTESIAN_POINT('Ctrl Pts',(-0.125706476822529,1.,-4.08494093372315));
#57490=CARTESIAN_POINT('Ctrl Pts',(-0.128500200484814,-1.,-4.07774270738809));
#57491=CARTESIAN_POINT('Ctrl Pts',(-0.128500200484814,1.,-4.07774270738809));
#57492=CARTESIAN_POINT('Ctrl Pts',(-0.131255793548914,-1.,-4.07053931528579));
#57493=CARTESIAN_POINT('Ctrl Pts',(-0.131255793548914,1.,-4.07053931528579));
#57494=CARTESIAN_POINT('Ctrl Pts',(-0.133972916144225,-1.,-4.06333121018476));
#57495=CARTESIAN_POINT('Ctrl Pts',(-0.133972916144225,1.,-4.06333121018476));
#57496=CARTESIAN_POINT('Ctrl Pts',(-0.136651205046111,-1.,-4.05611873400122));
#57497=CARTESIAN_POINT('Ctrl Pts',(-0.136651205046111,1.,-4.05611873400122));
#57498=CARTESIAN_POINT('Ctrl Pts',(-0.13929026718006,-1.,-4.04890199238056));
#57499=CARTESIAN_POINT('Ctrl Pts',(-0.13929026718006,1.,-4.04890199238056));
#57500=CARTESIAN_POINT('Ctrl Pts',(-0.141889671485508,-1.,-4.04168069633842));
#57501=CARTESIAN_POINT('Ctrl Pts',(-0.141889671485508,1.,-4.04168069633842));
#57502=CARTESIAN_POINT('Ctrl Pts',(-0.144448947038352,-1.,-4.03445411510403));
#57503=CARTESIAN_POINT('Ctrl Pts',(-0.144448947038352,1.,-4.03445411510403));
#57504=CARTESIAN_POINT('Ctrl Pts',(-0.146967602878999,-1.,-4.02722143147048));
#57505=CARTESIAN_POINT('Ctrl Pts',(-0.146967602878999,1.,-4.02722143147048));
#57506=CARTESIAN_POINT('Ctrl Pts',(-0.149445144968708,-1.,-4.01998203715588));
#57507=CARTESIAN_POINT('Ctrl Pts',(-0.149445144968708,1.,-4.01998203715588));
#57508=CARTESIAN_POINT('Ctrl Pts',(-0.151881094022909,-1.,-4.01273584234684));
#57509=CARTESIAN_POINT('Ctrl Pts',(-0.151881094022909,1.,-4.01273584234684));
#57510=CARTESIAN_POINT('Ctrl Pts',(-0.15427500487231,-1.,-4.00548360245297));
#57511=CARTESIAN_POINT('Ctrl Pts',(-0.15427500487231,1.,-4.00548360245297));
#57512=CARTESIAN_POINT('Ctrl Pts',(-0.156626481393736,-1.,-3.99822717425869));
#57513=CARTESIAN_POINT('Ctrl Pts',(-0.156626481393736,1.,-3.99822717425869));
#57514=CARTESIAN_POINT('Ctrl Pts',(-0.158935123982796,-1.,-3.99096873945862));
#57515=CARTESIAN_POINT('Ctrl Pts',(-0.158935123982796,1.,-3.99096873945862));
#57516=CARTESIAN_POINT('Ctrl Pts',(-0.161200482186088,-1.,-3.98371010319866));
#57517=CARTESIAN_POINT('Ctrl Pts',(-0.161200482186088,1.,-3.98371010319866));
#57518=CARTESIAN_POINT('Ctrl Pts',(-0.163422004609999,-1.,-3.97645194630944));
#57519=CARTESIAN_POINT('Ctrl Pts',(-0.163422004609999,1.,-3.97645194630944));
#57520=CARTESIAN_POINT('Ctrl Pts',(-0.165598992851098,-1.,-3.9691931362141));
#57521=CARTESIAN_POINT('Ctrl Pts',(-0.165598992851098,1.,-3.9691931362141));
#57522=CARTESIAN_POINT('Ctrl Pts',(-0.167730547023312,-1.,-3.96192990160296));
#57523=CARTESIAN_POINT('Ctrl Pts',(-0.167730547023312,1.,-3.96192990160296));
#57524=CARTESIAN_POINT('Ctrl Pts',(-0.16981566637413,-1.,-3.95465744665263));
#57525=CARTESIAN_POINT('Ctrl Pts',(-0.16981566637413,1.,-3.95465744665263));
#57526=CARTESIAN_POINT('Ctrl Pts',(-0.171853355369233,-1.,-3.94737164900861));
#57527=CARTESIAN_POINT('Ctrl Pts',(-0.171853355369233,1.,-3.94737164900861));
#57528=CARTESIAN_POINT('Ctrl Pts',(-0.173842734974607,-1.,-3.94007083096214));
#57529=CARTESIAN_POINT('Ctrl Pts',(-0.173842734974607,1.,-3.94007083096214));
#57530=CARTESIAN_POINT('Ctrl Pts',(-0.175783136893873,-1.,-3.93275726771049));
#57531=CARTESIAN_POINT('Ctrl Pts',(-0.175783136893873,1.,-3.93275726771049));
#57532=CARTESIAN_POINT('Ctrl Pts',(-0.177674246152328,-1.,-3.92543942697672));
#57533=CARTESIAN_POINT('Ctrl Pts',(-0.177674246152328,1.,-3.92543942697672));
#57534=CARTESIAN_POINT('Ctrl Pts',(-0.179515885822895,-1.,-3.91812876180948));
#57535=CARTESIAN_POINT('Ctrl Pts',(-0.179515885822895,1.,-3.91812876180948));
#57536=CARTESIAN_POINT('Ctrl Pts',(-0.181307740731796,-1.,-3.91083557557193));
#57537=CARTESIAN_POINT('Ctrl Pts',(-0.181307740731796,1.,-3.91083557557193));
#57538=CARTESIAN_POINT('Ctrl Pts',(-0.183049081993193,-1.,-3.90356488555138));
#57539=CARTESIAN_POINT('Ctrl Pts',(-0.183049081993193,1.,-3.90356488555138));
#57540=CARTESIAN_POINT('Ctrl Pts',(-0.184738537728035,-1.,-3.89631300742633));
#57541=CARTESIAN_POINT('Ctrl Pts',(-0.184738537728035,1.,-3.89631300742633));
#57542=CARTESIAN_POINT('Ctrl Pts',(-0.186373724985263,-1.,-3.88906196725817));
#57543=CARTESIAN_POINT('Ctrl Pts',(-0.186373724985263,1.,-3.88906196725817));
#57544=CARTESIAN_POINT('Ctrl Pts',(-0.187951632512663,-1.,-3.88178563496187));
#57545=CARTESIAN_POINT('Ctrl Pts',(-0.187951632512663,1.,-3.88178563496187));
#57546=CARTESIAN_POINT('Ctrl Pts',(-0.189469253358254,-1.,-3.87445976418377));
#57547=CARTESIAN_POINT('Ctrl Pts',(-0.189469253358254,1.,-3.87445976418377));
#57548=CARTESIAN_POINT('Ctrl Pts',(-0.190924190418613,-1.,-3.8670715862477));
#57549=CARTESIAN_POINT('Ctrl Pts',(-0.190924190418613,1.,-3.8670715862477));
#57550=CARTESIAN_POINT('Ctrl Pts',(-0.19231515304498,-1.,-3.85962774407652));
#57551=CARTESIAN_POINT('Ctrl Pts',(-0.19231515304498,1.,-3.85962774407652));
#57552=CARTESIAN_POINT('Ctrl Pts',(-0.193642806777748,-1.,-3.85216762264019));
#57553=CARTESIAN_POINT('Ctrl Pts',(-0.193642806777748,1.,-3.85216762264019));
#57554=CARTESIAN_POINT('Ctrl Pts',(-0.194909009460255,-1.,-3.84475203347052));
#57555=CARTESIAN_POINT('Ctrl Pts',(-0.194909009460255,1.,-3.84475203347052));
#57556=CARTESIAN_POINT('Ctrl Pts',(-0.19611519897189,-1.,-3.83743910616265));
#57557=CARTESIAN_POINT('Ctrl Pts',(-0.19611519897189,1.,-3.83743910616265));
#57558=CARTESIAN_POINT('Ctrl Pts',(-0.197260935827375,-1.,-3.83026221776488));
#57559=CARTESIAN_POINT('Ctrl Pts',(-0.197260935827375,1.,-3.83026221776488));
#57560=CARTESIAN_POINT('Ctrl Pts',(-0.19834261690047,-1.,-3.82321127348981));
#57561=CARTESIAN_POINT('Ctrl Pts',(-0.19834261690047,1.,-3.82321127348981));
#57562=CARTESIAN_POINT('Ctrl Pts',(-0.199351525297396,-1.,-3.81620203429702));
#57563=CARTESIAN_POINT('Ctrl Pts',(-0.199351525297396,1.,-3.81620203429702));
#57564=CARTESIAN_POINT('Ctrl Pts',(-0.20027467943329,-1.,-3.80909529318501));
#57565=CARTESIAN_POINT('Ctrl Pts',(-0.20027467943329,1.,-3.80909529318501));
#57566=CARTESIAN_POINT('Ctrl Pts',(-0.201097756307252,-1.,-3.80175247447171));
#57567=CARTESIAN_POINT('Ctrl Pts',(-0.201097756307252,1.,-3.80175247447171));
#57568=CARTESIAN_POINT('Ctrl Pts',(-0.201807533800799,-1.,-3.79408354187274));
#57569=CARTESIAN_POINT('Ctrl Pts',(-0.201807533800799,1.,-3.79408354187274));
#57570=CARTESIAN_POINT('Ctrl Pts',(-0.202394260512193,-1.,-3.78609175019317));
#57571=CARTESIAN_POINT('Ctrl Pts',(-0.202394260512193,1.,-3.78609175019317));
#57572=CARTESIAN_POINT('Ctrl Pts',(-0.202854729699197,-1.,-3.77793553476879));
#57573=CARTESIAN_POINT('Ctrl Pts',(-0.202854729699197,1.,-3.77793553476879));
#57574=CARTESIAN_POINT('Ctrl Pts',(-0.203192390045337,-1.,-3.76992071595267));
#57575=CARTESIAN_POINT('Ctrl Pts',(-0.203192390045337,1.,-3.76992071595267));
#57576=CARTESIAN_POINT('Ctrl Pts',(-0.203414634707646,-1.,-3.76242717937273));
#57577=CARTESIAN_POINT('Ctrl Pts',(-0.203414634707646,1.,-3.76242717937273));
#57578=CARTESIAN_POINT('Ctrl Pts',(-0.203530796848404,-1.,-3.75585118707924));
#57579=CARTESIAN_POINT('Ctrl Pts',(-0.203530796848404,1.,-3.75585118707924));
#57580=CARTESIAN_POINT('Ctrl Pts',(-0.203550035479097,-1.,-3.75054693397716));
#57581=CARTESIAN_POINT('Ctrl Pts',(-0.203550035479097,1.,-3.75054693397716));
#57582=CARTESIAN_POINT('Ctrl Pts',(-0.20347884453023,-1.,-3.74675472018582));
#57583=CARTESIAN_POINT('Ctrl Pts',(-0.20347884453023,1.,-3.74675472018582));
#57584=CARTESIAN_POINT('Ctrl Pts',(-0.203352057956055,-1.,-3.7450208092684));
#57585=CARTESIAN_POINT('Ctrl Pts',(-0.203352057956055,1.,-3.7450208092684));
#57586=CARTESIAN_POINT('Ctrl Pts',(-0.203218215747895,-1.,-3.74446880195845));
#57587=CARTESIAN_POINT('Ctrl Pts',(-0.203218215747895,1.,-3.74446880195845));
#57588=CARTESIAN_POINT('Ctrl Pts',(-0.20311176758786,-1.,-3.74443319346666));
#57589=CARTESIAN_POINT('Ctrl Pts',(-0.20311176758786,1.,-3.74443319346666));
#57590=CARTESIAN_POINT('Ctrl Pts',(-0.203054238699719,-1.,-3.74449849461127));
#57591=CARTESIAN_POINT('Ctrl Pts',(-0.203054238699719,1.,-3.74449849461127));
#57592=CARTESIAN_POINT('',(-0.0760622897878238,1.,-4.19931119685982));
#57593=CARTESIAN_POINT('Ctrl Pts',(-0.0760622897878238,1.,-4.19931119685982));
#57594=CARTESIAN_POINT('Ctrl Pts',(-0.0767384596142197,1.,-4.19789138621624));
#57595=CARTESIAN_POINT('Ctrl Pts',(-0.0780873956244405,1.,-4.19505112860624));
#57596=CARTESIAN_POINT('Ctrl Pts',(-0.0801005887117605,1.,-4.19078883322483));
#57597=CARTESIAN_POINT('Ctrl Pts',(-0.0827644164389512,1.,-4.1851019532944));
#57598=CARTESIAN_POINT('Ctrl Pts',(-0.0860600915552517,1.,-4.17798698669991));
#57599=CARTESIAN_POINT('Ctrl Pts',(-0.089321556085033,1.,-4.17086566491823));
#57600=CARTESIAN_POINT('Ctrl Pts',(-0.0925486672167692,1.,-4.16373802265942));
#57601=CARTESIAN_POINT('Ctrl Pts',(-0.095741240329707,1.,-4.15660412653006));
#57602=CARTESIAN_POINT('Ctrl Pts',(-0.0988990478899814,1.,-4.1494640891762));
#57603=CARTESIAN_POINT('Ctrl Pts',(-0.102021826577454,1.,-4.14231804938737));
#57604=CARTESIAN_POINT('Ctrl Pts',(-0.105109286538864,1.,-4.13516614458396));
#57605=CARTESIAN_POINT('Ctrl Pts',(-0.10816112052835,1.,-4.12800848371386));
#57606=CARTESIAN_POINT('Ctrl Pts',(-0.111177012683377,1.,-4.12084512502444));
#57607=CARTESIAN_POINT('Ctrl Pts',(-0.114156649609602,1.,-4.11367603925313));
#57608=CARTESIAN_POINT('Ctrl Pts',(-0.117099722731705,1.,-4.10650113382187));
#57609=CARTESIAN_POINT('Ctrl Pts',(-0.120005924388162,1.,-4.09932031767243));
#57610=CARTESIAN_POINT('Ctrl Pts',(-0.122874946249119,1.,-4.09213355850836));
#57611=CARTESIAN_POINT('Ctrl Pts',(-0.125706476822529,1.,-4.08494093372315));
#57612=CARTESIAN_POINT('Ctrl Pts',(-0.128500200484814,1.,-4.07774270738809));
#57613=CARTESIAN_POINT('Ctrl Pts',(-0.131255793548914,1.,-4.07053931528579));
#57614=CARTESIAN_POINT('Ctrl Pts',(-0.133972916144225,1.,-4.06333121018476));
#57615=CARTESIAN_POINT('Ctrl Pts',(-0.136651205046111,1.,-4.05611873400122));
#57616=CARTESIAN_POINT('Ctrl Pts',(-0.13929026718006,1.,-4.04890199238056));
#57617=CARTESIAN_POINT('Ctrl Pts',(-0.141889671485508,1.,-4.04168069633842));
#57618=CARTESIAN_POINT('Ctrl Pts',(-0.144448947038352,1.,-4.03445411510403));
#57619=CARTESIAN_POINT('Ctrl Pts',(-0.146967602878999,1.,-4.02722143147048));
#57620=CARTESIAN_POINT('Ctrl Pts',(-0.149445144968708,1.,-4.01998203715588));
#57621=CARTESIAN_POINT('Ctrl Pts',(-0.151881094022909,1.,-4.01273584234684));
#57622=CARTESIAN_POINT('Ctrl Pts',(-0.15427500487231,1.,-4.00548360245297));
#57623=CARTESIAN_POINT('Ctrl Pts',(-0.156626481393736,1.,-3.99822717425869));
#57624=CARTESIAN_POINT('Ctrl Pts',(-0.158935123982796,1.,-3.99096873945862));
#57625=CARTESIAN_POINT('Ctrl Pts',(-0.161200482186088,1.,-3.98371010319866));
#57626=CARTESIAN_POINT('Ctrl Pts',(-0.163422004609999,1.,-3.97645194630944));
#57627=CARTESIAN_POINT('Ctrl Pts',(-0.165598992851098,1.,-3.9691931362141));
#57628=CARTESIAN_POINT('Ctrl Pts',(-0.167730547023312,1.,-3.96192990160296));
#57629=CARTESIAN_POINT('Ctrl Pts',(-0.16981566637413,1.,-3.95465744665263));
#57630=CARTESIAN_POINT('Ctrl Pts',(-0.171853355369233,1.,-3.94737164900861));
#57631=CARTESIAN_POINT('Ctrl Pts',(-0.173842734974607,1.,-3.94007083096214));
#57632=CARTESIAN_POINT('Ctrl Pts',(-0.175783136893873,1.,-3.93275726771049));
#57633=CARTESIAN_POINT('Ctrl Pts',(-0.177674246152328,1.,-3.92543942697672));
#57634=CARTESIAN_POINT('Ctrl Pts',(-0.179515885822895,1.,-3.91812876180948));
#57635=CARTESIAN_POINT('Ctrl Pts',(-0.181307740731796,1.,-3.91083557557193));
#57636=CARTESIAN_POINT('Ctrl Pts',(-0.183049081993193,1.,-3.90356488555138));
#57637=CARTESIAN_POINT('Ctrl Pts',(-0.184738537728035,1.,-3.89631300742633));
#57638=CARTESIAN_POINT('Ctrl Pts',(-0.186373724985263,1.,-3.88906196725817));
#57639=CARTESIAN_POINT('Ctrl Pts',(-0.187951632512663,1.,-3.88178563496187));
#57640=CARTESIAN_POINT('Ctrl Pts',(-0.189469253358254,1.,-3.87445976418377));
#57641=CARTESIAN_POINT('Ctrl Pts',(-0.190924190418613,1.,-3.8670715862477));
#57642=CARTESIAN_POINT('Ctrl Pts',(-0.19231515304498,1.,-3.85962774407652));
#57643=CARTESIAN_POINT('Ctrl Pts',(-0.193642806777748,1.,-3.85216762264019));
#57644=CARTESIAN_POINT('Ctrl Pts',(-0.194909009460255,1.,-3.84475203347052));
#57645=CARTESIAN_POINT('Ctrl Pts',(-0.19611519897189,1.,-3.83743910616265));
#57646=CARTESIAN_POINT('Ctrl Pts',(-0.197260935827375,1.,-3.83026221776488));
#57647=CARTESIAN_POINT('Ctrl Pts',(-0.19834261690047,1.,-3.82321127348981));
#57648=CARTESIAN_POINT('Ctrl Pts',(-0.199351525297396,1.,-3.81620203429702));
#57649=CARTESIAN_POINT('Ctrl Pts',(-0.20027467943329,1.,-3.80909529318501));
#57650=CARTESIAN_POINT('Ctrl Pts',(-0.201097756307252,1.,-3.80175247447171));
#57651=CARTESIAN_POINT('Ctrl Pts',(-0.201807533800799,1.,-3.79408354187274));
#57652=CARTESIAN_POINT('Ctrl Pts',(-0.202394260512193,1.,-3.78609175019317));
#57653=CARTESIAN_POINT('Ctrl Pts',(-0.202854729699197,1.,-3.77793553476879));
#57654=CARTESIAN_POINT('Ctrl Pts',(-0.203192390045337,1.,-3.76992071595267));
#57655=CARTESIAN_POINT('Ctrl Pts',(-0.203414634707646,1.,-3.76242717937273));
#57656=CARTESIAN_POINT('Ctrl Pts',(-0.203530796848404,1.,-3.75585118707924));
#57657=CARTESIAN_POINT('Ctrl Pts',(-0.203550035479097,1.,-3.75054693397716));
#57658=CARTESIAN_POINT('Ctrl Pts',(-0.203484186269315,1.,-3.74703926501843));
#57659=CARTESIAN_POINT('Ctrl Pts',(-0.203375226874331,1.,-3.74535749969262));
#57660=CARTESIAN_POINT('Ctrl Pts',(-0.203266610111264,1.,-3.74471097893961));
#57661=CARTESIAN_POINT('Ctrl Pts',(-0.203188003947965,1.,-3.74453008995129));
#57662=CARTESIAN_POINT('Ctrl Pts',(-0.203156094897896,1.,-3.74449296982994));
#57663=CARTESIAN_POINT('',(-0.0760622897878238,0.,-4.19931119685982));
#57664=CARTESIAN_POINT('Ctrl Pts',(0.20305423869972,-1.,-3.74449849461127));
#57665=CARTESIAN_POINT('Ctrl Pts',(0.20305423869972,1.,-3.74449849461127));
#57666=CARTESIAN_POINT('Ctrl Pts',(0.203111767587923,-1.,-3.7444331934681));
#57667=CARTESIAN_POINT('Ctrl Pts',(0.203111767587923,1.,-3.7444331934681));
#57668=CARTESIAN_POINT('Ctrl Pts',(0.203218215748058,-1.,-3.7444688019622));
#57669=CARTESIAN_POINT('Ctrl Pts',(0.203218215748058,1.,-3.7444688019622));
#57670=CARTESIAN_POINT('Ctrl Pts',(0.203352057956297,-1.,-3.74502080927395));
#57671=CARTESIAN_POINT('Ctrl Pts',(0.203352057956297,1.,-3.74502080927395));
#57672=CARTESIAN_POINT('Ctrl Pts',(0.203478844530447,-1.,-3.7467547201908));
#57673=CARTESIAN_POINT('Ctrl Pts',(0.203478844530447,1.,-3.7467547201908));
#57674=CARTESIAN_POINT('Ctrl Pts',(0.203550035479166,-1.,-3.75054693397875));
#57675=CARTESIAN_POINT('Ctrl Pts',(0.203550035479166,1.,-3.75054693397875));
#57676=CARTESIAN_POINT('Ctrl Pts',(0.203530796848321,-1.,-3.75585118707734));
#57677=CARTESIAN_POINT('Ctrl Pts',(0.203530796848321,1.,-3.75585118707734));
#57678=CARTESIAN_POINT('Ctrl Pts',(0.203414634707478,-1.,-3.76242717936885));
#57679=CARTESIAN_POINT('Ctrl Pts',(0.203414634707478,1.,-3.76242717936885));
#57680=CARTESIAN_POINT('Ctrl Pts',(0.203192390045164,-1.,-3.7699207159487));
#57681=CARTESIAN_POINT('Ctrl Pts',(0.203192390045164,1.,-3.7699207159487));
#57682=CARTESIAN_POINT('Ctrl Pts',(0.202854729699081,-1.,-3.77793553476614));
#57683=CARTESIAN_POINT('Ctrl Pts',(0.202854729699081,1.,-3.77793553476614));
#57684=CARTESIAN_POINT('Ctrl Pts',(0.20239426051216,-1.,-3.78609175019242));
#57685=CARTESIAN_POINT('Ctrl Pts',(0.20239426051216,1.,-3.78609175019242));
#57686=CARTESIAN_POINT('Ctrl Pts',(0.201807533800837,-1.,-3.7940835418736));
#57687=CARTESIAN_POINT('Ctrl Pts',(0.201807533800837,1.,-3.7940835418736));
#57688=CARTESIAN_POINT('Ctrl Pts',(0.201097756307326,-1.,-3.80175247447337));
#57689=CARTESIAN_POINT('Ctrl Pts',(0.201097756307326,1.,-3.80175247447337));
#57690=CARTESIAN_POINT('Ctrl Pts',(0.200274679433364,-1.,-3.80909529318669));
#57691=CARTESIAN_POINT('Ctrl Pts',(0.200274679433364,1.,-3.80909529318669));
#57692=CARTESIAN_POINT('Ctrl Pts',(0.199351525297447,-1.,-3.81620203429815));
#57693=CARTESIAN_POINT('Ctrl Pts',(0.199351525297447,1.,-3.81620203429815));
#57694=CARTESIAN_POINT('Ctrl Pts',(0.198342616900486,-1.,-3.82321127349016));
#57695=CARTESIAN_POINT('Ctrl Pts',(0.198342616900486,1.,-3.82321127349016));
#57696=CARTESIAN_POINT('Ctrl Pts',(0.197260935827361,-1.,-3.83026221776456));
#57697=CARTESIAN_POINT('Ctrl Pts',(0.197260935827361,1.,-3.83026221776456));
#57698=CARTESIAN_POINT('Ctrl Pts',(0.196115198971859,-1.,-3.83743910616195));
#57699=CARTESIAN_POINT('Ctrl Pts',(0.196115198971859,1.,-3.83743910616195));
#57700=CARTESIAN_POINT('Ctrl Pts',(0.19490900946022,-1.,-3.84475203346977));
#57701=CARTESIAN_POINT('Ctrl Pts',(0.19490900946022,1.,-3.84475203346977));
#57702=CARTESIAN_POINT('Ctrl Pts',(0.193642806777723,-1.,-3.85216762263966));
#57703=CARTESIAN_POINT('Ctrl Pts',(0.193642806777723,1.,-3.85216762263966));
#57704=CARTESIAN_POINT('Ctrl Pts',(0.19231515304497,-1.,-3.85962774407633));
#57705=CARTESIAN_POINT('Ctrl Pts',(0.19231515304497,1.,-3.85962774407633));
#57706=CARTESIAN_POINT('Ctrl Pts',(0.19092419041862,-1.,-3.86707158624783));
#57707=CARTESIAN_POINT('Ctrl Pts',(0.19092419041862,1.,-3.86707158624783));
#57708=CARTESIAN_POINT('Ctrl Pts',(0.189469253358272,-1.,-3.87445976418412));
#57709=CARTESIAN_POINT('Ctrl Pts',(0.189469253358272,1.,-3.87445976418412));
#57710=CARTESIAN_POINT('Ctrl Pts',(0.187951632512685,-1.,-3.88178563496228));
#57711=CARTESIAN_POINT('Ctrl Pts',(0.187951632512685,1.,-3.88178563496228));
#57712=CARTESIAN_POINT('Ctrl Pts',(0.18637372498528,-1.,-3.88906196725848));
#57713=CARTESIAN_POINT('Ctrl Pts',(0.18637372498528,1.,-3.88906196725848));
#57714=CARTESIAN_POINT('Ctrl Pts',(0.184738537728043,-1.,-3.89631300742646));
#57715=CARTESIAN_POINT('Ctrl Pts',(0.184738537728043,1.,-3.89631300742646));
#57716=CARTESIAN_POINT('Ctrl Pts',(0.18304908199319,-1.,-3.90356488555132));
#57717=CARTESIAN_POINT('Ctrl Pts',(0.18304908199319,1.,-3.90356488555132));
#57718=CARTESIAN_POINT('Ctrl Pts',(0.181307740731785,-1.,-3.91083557557175));
#57719=CARTESIAN_POINT('Ctrl Pts',(0.181307740731785,1.,-3.91083557557175));
#57720=CARTESIAN_POINT('Ctrl Pts',(0.179515885822881,-1.,-3.91812876180926));
#57721=CARTESIAN_POINT('Ctrl Pts',(0.179515885822881,1.,-3.91812876180926));
#57722=CARTESIAN_POINT('Ctrl Pts',(0.177674246152317,-1.,-3.92543942697655));
#57723=CARTESIAN_POINT('Ctrl Pts',(0.177674246152317,1.,-3.92543942697655));
#57724=CARTESIAN_POINT('Ctrl Pts',(0.175783136893868,-1.,-3.93275726771042));
#57725=CARTESIAN_POINT('Ctrl Pts',(0.175783136893868,1.,-3.93275726771042));
#57726=CARTESIAN_POINT('Ctrl Pts',(0.173842734974609,-1.,-3.94007083096217));
#57727=CARTESIAN_POINT('Ctrl Pts',(0.173842734974609,1.,-3.94007083096217));
#57728=CARTESIAN_POINT('Ctrl Pts',(0.17185335536924,-1.,-3.94737164900868));
#57729=CARTESIAN_POINT('Ctrl Pts',(0.17185335536924,1.,-3.94737164900868));
#57730=CARTESIAN_POINT('Ctrl Pts',(0.169815666374139,-1.,-3.95465744665268));
#57731=CARTESIAN_POINT('Ctrl Pts',(0.169815666374139,1.,-3.95465744665268));
#57732=CARTESIAN_POINT('Ctrl Pts',(0.167730547023319,-1.,-3.96192990160296));
#57733=CARTESIAN_POINT('Ctrl Pts',(0.167730547023319,1.,-3.96192990160296));
#57734=CARTESIAN_POINT('Ctrl Pts',(0.165598992851102,-1.,-3.96919313621407));
#57735=CARTESIAN_POINT('Ctrl Pts',(0.165598992851102,1.,-3.96919313621407));
#57736=CARTESIAN_POINT('Ctrl Pts',(0.163422004609999,-1.,-3.97645194630943));
#57737=CARTESIAN_POINT('Ctrl Pts',(0.163422004609999,1.,-3.97645194630943));
#57738=CARTESIAN_POINT('Ctrl Pts',(0.161200482186084,-1.,-3.98371010319872));
#57739=CARTESIAN_POINT('Ctrl Pts',(0.161200482186084,1.,-3.98371010319872));
#57740=CARTESIAN_POINT('Ctrl Pts',(0.158935123982793,-1.,-3.99096873945878));
#57741=CARTESIAN_POINT('Ctrl Pts',(0.158935123982793,1.,-3.99096873945878));
#57742=CARTESIAN_POINT('Ctrl Pts',(0.156626481393734,-1.,-3.99822717425893));
#57743=CARTESIAN_POINT('Ctrl Pts',(0.156626481393734,1.,-3.99822717425893));
#57744=CARTESIAN_POINT('Ctrl Pts',(0.15427500487231,-1.,-4.00548360245319));
#57745=CARTESIAN_POINT('Ctrl Pts',(0.15427500487231,1.,-4.00548360245319));
#57746=CARTESIAN_POINT('Ctrl Pts',(0.15188109402291,-1.,-4.01273584234689));
#57747=CARTESIAN_POINT('Ctrl Pts',(0.15188109402291,1.,-4.01273584234689));
#57748=CARTESIAN_POINT('Ctrl Pts',(0.149445144968707,-1.,-4.01998203715564));
#57749=CARTESIAN_POINT('Ctrl Pts',(0.149445144968707,1.,-4.01998203715564));
#57750=CARTESIAN_POINT('Ctrl Pts',(0.146967602878994,-1.,-4.02722143146994));
#57751=CARTESIAN_POINT('Ctrl Pts',(0.146967602878994,1.,-4.02722143146994));
#57752=CARTESIAN_POINT('Ctrl Pts',(0.144448947038344,-1.,-4.03445411510333));
#57753=CARTESIAN_POINT('Ctrl Pts',(0.144448947038344,1.,-4.03445411510333));
#57754=CARTESIAN_POINT('Ctrl Pts',(0.1418896714855,-1.,-4.04168069633781));
#57755=CARTESIAN_POINT('Ctrl Pts',(0.1418896714855,1.,-4.04168069633781));
#57756=CARTESIAN_POINT('Ctrl Pts',(0.139290267180057,-1.,-4.04890199238036));
#57757=CARTESIAN_POINT('Ctrl Pts',(0.139290267180057,1.,-4.04890199238036));
#57758=CARTESIAN_POINT('Ctrl Pts',(0.136651205046119,-1.,-4.05611873400172));
#57759=CARTESIAN_POINT('Ctrl Pts',(0.136651205046119,1.,-4.05611873400172));
#57760=CARTESIAN_POINT('Ctrl Pts',(0.133972916144245,-1.,-4.06333121018596));
#57761=CARTESIAN_POINT('Ctrl Pts',(0.133972916144245,1.,-4.06333121018596));
#57762=CARTESIAN_POINT('Ctrl Pts',(0.13125579354894,-1.,-4.0705393152874));
#57763=CARTESIAN_POINT('Ctrl Pts',(0.13125579354894,1.,-4.0705393152874));
#57764=CARTESIAN_POINT('Ctrl Pts',(0.128500200484837,-1.,-4.07774270738954));
#57765=CARTESIAN_POINT('Ctrl Pts',(0.128500200484837,1.,-4.07774270738954));
#57766=CARTESIAN_POINT('Ctrl Pts',(0.12570647682254,-1.,-4.08494093372377));
#57767=CARTESIAN_POINT('Ctrl Pts',(0.12570647682254,1.,-4.08494093372377));
#57768=CARTESIAN_POINT('Ctrl Pts',(0.122874946249107,-1.,-4.09213355850756));
#57769=CARTESIAN_POINT('Ctrl Pts',(0.122874946249107,1.,-4.09213355850756));
#57770=CARTESIAN_POINT('Ctrl Pts',(0.120005924388124,-1.,-4.09932031767002));
#57771=CARTESIAN_POINT('Ctrl Pts',(0.120005924388124,1.,-4.09932031767002));
#57772=CARTESIAN_POINT('Ctrl Pts',(0.117099722731648,-1.,-4.10650113381833));
#57773=CARTESIAN_POINT('Ctrl Pts',(0.117099722731648,1.,-4.10650113381833));
#57774=CARTESIAN_POINT('Ctrl Pts',(0.114156649609545,-1.,-4.11367603924961));
#57775=CARTESIAN_POINT('Ctrl Pts',(0.114156649609545,1.,-4.11367603924961));
#57776=CARTESIAN_POINT('Ctrl Pts',(0.111177012683346,-1.,-4.1208451250225));
#57777=CARTESIAN_POINT('Ctrl Pts',(0.111177012683346,1.,-4.1208451250225));
#57778=CARTESIAN_POINT('Ctrl Pts',(0.108161120528369,-1.,-4.12800848371504));
#57779=CARTESIAN_POINT('Ctrl Pts',(0.108161120528369,1.,-4.12800848371504));
#57780=CARTESIAN_POINT('Ctrl Pts',(0.105109286538945,-1.,-4.13516614458895));
#57781=CARTESIAN_POINT('Ctrl Pts',(0.105109286538945,1.,-4.13516614458895));
#57782=CARTESIAN_POINT('Ctrl Pts',(0.102021826577584,-1.,-4.14231804939538));
#57783=CARTESIAN_POINT('Ctrl Pts',(0.102021826577584,1.,-4.14231804939538));
#57784=CARTESIAN_POINT('Ctrl Pts',(0.0988990478901223,-1.,-4.14946408918485));
#57785=CARTESIAN_POINT('Ctrl Pts',(0.0988990478901223,1.,-4.14946408918485));
#57786=CARTESIAN_POINT('Ctrl Pts',(0.0957412403298004,-1.,-4.15660412653577));
#57787=CARTESIAN_POINT('Ctrl Pts',(0.0957412403298004,1.,-4.15660412653577));
#57788=CARTESIAN_POINT('Ctrl Pts',(0.0925486672167528,-1.,-4.16373802265839));
#57789=CARTESIAN_POINT('Ctrl Pts',(0.0925486672167528,1.,-4.16373802265839));
#57790=CARTESIAN_POINT('Ctrl Pts',(0.0893215560848647,-1.,-4.17086566490794));
#57791=CARTESIAN_POINT('Ctrl Pts',(0.0893215560848647,1.,-4.17086566490794));
#57792=CARTESIAN_POINT('Ctrl Pts',(0.0860600915549394,-1.,-4.17798698668094));
#57793=CARTESIAN_POINT('Ctrl Pts',(0.0860600915549394,1.,-4.17798698668094));
#57794=CARTESIAN_POINT('Ctrl Pts',(0.0827644164385676,-1.,-4.18510195327123));
#57795=CARTESIAN_POINT('Ctrl Pts',(0.0827644164385676,1.,-4.18510195327123));
#57796=CARTESIAN_POINT('Ctrl Pts',(0.0801005887114317,-1.,-4.19078883320504));
#57797=CARTESIAN_POINT('Ctrl Pts',(0.0801005887114317,1.,-4.19078883320504));
#57798=CARTESIAN_POINT('Ctrl Pts',(0.0780873956242395,-1.,-4.19505112859416));
#57799=CARTESIAN_POINT('Ctrl Pts',(0.0780873956242395,1.,-4.19505112859416));
#57800=CARTESIAN_POINT('Ctrl Pts',(0.0767384596141462,-1.,-4.1978913862118));
#57801=CARTESIAN_POINT('Ctrl Pts',(0.0767384596141462,1.,-4.1978913862118));
#57802=CARTESIAN_POINT('Ctrl Pts',(0.0760622897878244,-1.,-4.19931119685982));
#57803=CARTESIAN_POINT('Ctrl Pts',(0.0760622897878244,1.,-4.19931119685982));
#57804=CARTESIAN_POINT('',(0.203156094896102,1.,-3.74449296983004));
#57805=CARTESIAN_POINT('Ctrl Pts',(0.2031560948961,-1.,-3.74449296983004));
#57806=CARTESIAN_POINT('Ctrl Pts',(0.2031560948961,-0.666666666666667,-3.74449296983004));
#57807=CARTESIAN_POINT('Ctrl Pts',(0.2031560948961,-0.333333333333333,-3.74449296983004));
#57808=CARTESIAN_POINT('Ctrl Pts',(0.2031560948961,0.333333333333333,-3.74449296983004));
#57809=CARTESIAN_POINT('Ctrl Pts',(0.203156094896101,0.666666666666667,
-3.74449296983004));
#57810=CARTESIAN_POINT('Ctrl Pts',(0.203156094896101,1.,-3.74449296983004));
#57811=CARTESIAN_POINT('',(0.0760622897878244,1.,-4.19931119685982));
#57812=CARTESIAN_POINT('',(0.0760622897878244,0.,-4.19931119685982));
#57813=CARTESIAN_POINT('Ctrl Pts',(0.203156094896101,1.,-3.74449296983004));
#57814=CARTESIAN_POINT('Ctrl Pts',(0.203188003946657,1.,-3.74453008995093));
#57815=CARTESIAN_POINT('Ctrl Pts',(0.203266610110531,1.,-3.74471097893845));
#57816=CARTESIAN_POINT('Ctrl Pts',(0.203375226874121,1.,-3.74535749969115));
#57817=CARTESIAN_POINT('Ctrl Pts',(0.203484186269415,1.,-3.74703926501752));
#57818=CARTESIAN_POINT('Ctrl Pts',(0.203550035479166,1.,-3.75054693397875));
#57819=CARTESIAN_POINT('Ctrl Pts',(0.203530796848321,1.,-3.75585118707734));
#57820=CARTESIAN_POINT('Ctrl Pts',(0.203414634707478,1.,-3.76242717936885));
#57821=CARTESIAN_POINT('Ctrl Pts',(0.203192390045164,1.,-3.7699207159487));
#57822=CARTESIAN_POINT('Ctrl Pts',(0.202854729699081,1.,-3.77793553476614));
#57823=CARTESIAN_POINT('Ctrl Pts',(0.20239426051216,1.,-3.78609175019242));
#57824=CARTESIAN_POINT('Ctrl Pts',(0.201807533800837,1.,-3.7940835418736));
#57825=CARTESIAN_POINT('Ctrl Pts',(0.201097756307326,1.,-3.80175247447337));
#57826=CARTESIAN_POINT('Ctrl Pts',(0.200274679433364,1.,-3.80909529318669));
#57827=CARTESIAN_POINT('Ctrl Pts',(0.199351525297447,1.,-3.81620203429815));
#57828=CARTESIAN_POINT('Ctrl Pts',(0.198342616900486,1.,-3.82321127349016));
#57829=CARTESIAN_POINT('Ctrl Pts',(0.197260935827361,1.,-3.83026221776456));
#57830=CARTESIAN_POINT('Ctrl Pts',(0.196115198971859,1.,-3.83743910616195));
#57831=CARTESIAN_POINT('Ctrl Pts',(0.19490900946022,1.,-3.84475203346977));
#57832=CARTESIAN_POINT('Ctrl Pts',(0.193642806777723,1.,-3.85216762263966));
#57833=CARTESIAN_POINT('Ctrl Pts',(0.19231515304497,1.,-3.85962774407633));
#57834=CARTESIAN_POINT('Ctrl Pts',(0.19092419041862,1.,-3.86707158624783));
#57835=CARTESIAN_POINT('Ctrl Pts',(0.189469253358272,1.,-3.87445976418412));
#57836=CARTESIAN_POINT('Ctrl Pts',(0.187951632512685,1.,-3.88178563496228));
#57837=CARTESIAN_POINT('Ctrl Pts',(0.18637372498528,1.,-3.88906196725848));
#57838=CARTESIAN_POINT('Ctrl Pts',(0.184738537728043,1.,-3.89631300742646));
#57839=CARTESIAN_POINT('Ctrl Pts',(0.18304908199319,1.,-3.90356488555132));
#57840=CARTESIAN_POINT('Ctrl Pts',(0.181307740731785,1.,-3.91083557557175));
#57841=CARTESIAN_POINT('Ctrl Pts',(0.179515885822881,1.,-3.91812876180926));
#57842=CARTESIAN_POINT('Ctrl Pts',(0.177674246152317,1.,-3.92543942697655));
#57843=CARTESIAN_POINT('Ctrl Pts',(0.175783136893868,1.,-3.93275726771042));
#57844=CARTESIAN_POINT('Ctrl Pts',(0.173842734974609,1.,-3.94007083096217));
#57845=CARTESIAN_POINT('Ctrl Pts',(0.17185335536924,1.,-3.94737164900868));
#57846=CARTESIAN_POINT('Ctrl Pts',(0.169815666374139,1.,-3.95465744665268));
#57847=CARTESIAN_POINT('Ctrl Pts',(0.167730547023319,1.,-3.96192990160296));
#57848=CARTESIAN_POINT('Ctrl Pts',(0.165598992851102,1.,-3.96919313621407));
#57849=CARTESIAN_POINT('Ctrl Pts',(0.163422004609999,1.,-3.97645194630943));
#57850=CARTESIAN_POINT('Ctrl Pts',(0.161200482186084,1.,-3.98371010319872));
#57851=CARTESIAN_POINT('Ctrl Pts',(0.158935123982793,1.,-3.99096873945878));
#57852=CARTESIAN_POINT('Ctrl Pts',(0.156626481393734,1.,-3.99822717425893));
#57853=CARTESIAN_POINT('Ctrl Pts',(0.15427500487231,1.,-4.00548360245319));
#57854=CARTESIAN_POINT('Ctrl Pts',(0.15188109402291,1.,-4.01273584234689));
#57855=CARTESIAN_POINT('Ctrl Pts',(0.149445144968707,1.,-4.01998203715564));
#57856=CARTESIAN_POINT('Ctrl Pts',(0.146967602878994,1.,-4.02722143146994));
#57857=CARTESIAN_POINT('Ctrl Pts',(0.144448947038344,1.,-4.03445411510333));
#57858=CARTESIAN_POINT('Ctrl Pts',(0.1418896714855,1.,-4.04168069633781));
#57859=CARTESIAN_POINT('Ctrl Pts',(0.139290267180057,1.,-4.04890199238036));
#57860=CARTESIAN_POINT('Ctrl Pts',(0.136651205046119,1.,-4.05611873400172));
#57861=CARTESIAN_POINT('Ctrl Pts',(0.133972916144245,1.,-4.06333121018596));
#57862=CARTESIAN_POINT('Ctrl Pts',(0.13125579354894,1.,-4.0705393152874));
#57863=CARTESIAN_POINT('Ctrl Pts',(0.128500200484837,1.,-4.07774270738954));
#57864=CARTESIAN_POINT('Ctrl Pts',(0.12570647682254,1.,-4.08494093372377));
#57865=CARTESIAN_POINT('Ctrl Pts',(0.122874946249107,1.,-4.09213355850756));
#57866=CARTESIAN_POINT('Ctrl Pts',(0.120005924388124,1.,-4.09932031767002));
#57867=CARTESIAN_POINT('Ctrl Pts',(0.117099722731648,1.,-4.10650113381833));
#57868=CARTESIAN_POINT('Ctrl Pts',(0.114156649609545,1.,-4.11367603924961));
#57869=CARTESIAN_POINT('Ctrl Pts',(0.111177012683346,1.,-4.1208451250225));
#57870=CARTESIAN_POINT('Ctrl Pts',(0.108161120528369,1.,-4.12800848371504));
#57871=CARTESIAN_POINT('Ctrl Pts',(0.105109286538945,1.,-4.13516614458895));
#57872=CARTESIAN_POINT('Ctrl Pts',(0.102021826577584,1.,-4.14231804939538));
#57873=CARTESIAN_POINT('Ctrl Pts',(0.0988990478901223,1.,-4.14946408918485));
#57874=CARTESIAN_POINT('Ctrl Pts',(0.0957412403298004,1.,-4.15660412653577));
#57875=CARTESIAN_POINT('Ctrl Pts',(0.0925486672167528,1.,-4.16373802265839));
#57876=CARTESIAN_POINT('Ctrl Pts',(0.0893215560848647,1.,-4.17086566490794));
#57877=CARTESIAN_POINT('Ctrl Pts',(0.0860600915549394,1.,-4.17798698668094));
#57878=CARTESIAN_POINT('Ctrl Pts',(0.0827644164385676,1.,-4.18510195327123));
#57879=CARTESIAN_POINT('Ctrl Pts',(0.0801005887114317,1.,-4.19078883320504));
#57880=CARTESIAN_POINT('Ctrl Pts',(0.0780873956242395,1.,-4.19505112859416));
#57881=CARTESIAN_POINT('Ctrl Pts',(0.0767384596141462,1.,-4.1978913862118));
#57882=CARTESIAN_POINT('Ctrl Pts',(0.0760622897878244,1.,-4.19931119685982));
#57883=CARTESIAN_POINT('Origin',(0.0760622897878244,0.,-4.19931119685982));
#57884=CARTESIAN_POINT('',(-0.0760622897878238,1.,-4.19931119685982));
#57885=CARTESIAN_POINT('Origin',(0.,0.,0.));
#57886=CARTESIAN_POINT('',(0.385112848330761,1.,-3.73017266276651));
#57887=CARTESIAN_POINT('Origin',(0.,1.,0.));
#57888=CARTESIAN_POINT('Ctrl Pts',(0.385112848330762,1.,-3.73017266276651));
#57889=CARTESIAN_POINT('Ctrl Pts',(0.385112848330762,0.666666666666667,
-3.73017266276651));
#57890=CARTESIAN_POINT('Ctrl Pts',(0.385112848330762,0.333333333333333,
-3.73017266276651));
#57891=CARTESIAN_POINT('Ctrl Pts',(0.385112848330762,-0.333333333333333,
-3.73017266276651));
#57892=CARTESIAN_POINT('Ctrl Pts',(0.385112848330762,-0.666666666666667,
-3.73017266276651));
#57893=CARTESIAN_POINT('Ctrl Pts',(0.385112848330762,-1.,-3.73017266276651));
#57894=CARTESIAN_POINT('Ctrl Pts',(0.581791163835815,-1.,-4.15950947128175));
#57895=CARTESIAN_POINT('Ctrl Pts',(0.581791163835815,1.,-4.15950947128175));
#57896=CARTESIAN_POINT('Ctrl Pts',(0.580901211463535,-1.,-4.1582129171283));
#57897=CARTESIAN_POINT('Ctrl Pts',(0.580901211463535,1.,-4.1582129171283));
#57898=CARTESIAN_POINT('Ctrl Pts',(0.579124568914235,-1.,-4.15561864788576));
#57899=CARTESIAN_POINT('Ctrl Pts',(0.579124568914235,1.,-4.15561864788576));
#57900=CARTESIAN_POINT('Ctrl Pts',(0.576469391676688,-1.,-4.151723761217));
#57901=CARTESIAN_POINT('Ctrl Pts',(0.576469391676688,1.,-4.151723761217));
#57902=CARTESIAN_POINT('Ctrl Pts',(0.572948736069522,-1.,-4.14652361068081));
#57903=CARTESIAN_POINT('Ctrl Pts',(0.572948736069522,1.,-4.14652361068081));
#57904=CARTESIAN_POINT('Ctrl Pts',(0.568580610189774,-1.,-4.14001179830547));
#57905=CARTESIAN_POINT('Ctrl Pts',(0.568580610189774,1.,-4.14001179830547));
#57906=CARTESIAN_POINT('Ctrl Pts',(0.564245279537148,-1.,-4.13348835727104));
#57907=CARTESIAN_POINT('Ctrl Pts',(0.564245279537148,1.,-4.13348835727104));
#57908=CARTESIAN_POINT('Ctrl Pts',(0.559942890594773,-1.,-4.12695329951961));
#57909=CARTESIAN_POINT('Ctrl Pts',(0.559942890594773,1.,-4.12695329951961));
#57910=CARTESIAN_POINT('Ctrl Pts',(0.555673636129977,-1.,-4.12040666195664));
#57911=CARTESIAN_POINT('Ctrl Pts',(0.555673636129977,1.,-4.12040666195664));
#57912=CARTESIAN_POINT('Ctrl Pts',(0.551437758497032,-1.,-4.11384852024721));
#57913=CARTESIAN_POINT('Ctrl Pts',(0.551437758497032,1.,-4.11384852024721));
#57914=CARTESIAN_POINT('Ctrl Pts',(0.547235539485636,-1.,-4.10727897027977));
#57915=CARTESIAN_POINT('Ctrl Pts',(0.547235539485636,1.,-4.10727897027977));
#57916=CARTESIAN_POINT('Ctrl Pts',(0.543067286877757,-1.,-4.10069810243979));
#57917=CARTESIAN_POINT('Ctrl Pts',(0.543067286877757,1.,-4.10069810243979));
#57918=CARTESIAN_POINT('Ctrl Pts',(0.538933321179755,-1.,-4.09410597627));
#57919=CARTESIAN_POINT('Ctrl Pts',(0.538933321179755,1.,-4.09410597627));
#57920=CARTESIAN_POINT('Ctrl Pts',(0.534833963477273,-1.,-4.08750259988885));
#57921=CARTESIAN_POINT('Ctrl Pts',(0.534833963477273,1.,-4.08750259988885));
#57922=CARTESIAN_POINT('Ctrl Pts',(0.53076951872857,-1.,-4.08088789536836));
#57923=CARTESIAN_POINT('Ctrl Pts',(0.53076951872857,1.,-4.08088789536836));
#57924=CARTESIAN_POINT('Ctrl Pts',(0.526740277227498,-1.,-4.07426172299847));
#57925=CARTESIAN_POINT('Ctrl Pts',(0.526740277227498,1.,-4.07426172299847));
#57926=CARTESIAN_POINT('Ctrl Pts',(0.522746528603107,-1.,-4.06762394471314));
#57927=CARTESIAN_POINT('Ctrl Pts',(0.522746528603107,1.,-4.06762394471314));
#57928=CARTESIAN_POINT('Ctrl Pts',(0.518788572336923,-1.,-4.06097448038013));
#57929=CARTESIAN_POINT('Ctrl Pts',(0.518788572336923,1.,-4.06097448038013));
#57930=CARTESIAN_POINT('Ctrl Pts',(0.514866728193016,-1.,-4.05431335771199));
#57931=CARTESIAN_POINT('Ctrl Pts',(0.514866728193016,1.,-4.05431335771199));
#57932=CARTESIAN_POINT('Ctrl Pts',(0.51098134921897,-1.,-4.04764078815447));
#57933=CARTESIAN_POINT('Ctrl Pts',(0.51098134921897,1.,-4.04764078815447));
#57934=CARTESIAN_POINT('Ctrl Pts',(0.507132823288136,-1.,-4.04095715148915));
#57935=CARTESIAN_POINT('Ctrl Pts',(0.507132823288136,1.,-4.04095715148915));
#57936=CARTESIAN_POINT('Ctrl Pts',(0.503321556915346,-1.,-4.03426284174272));
#57937=CARTESIAN_POINT('Ctrl Pts',(0.503321556915346,1.,-4.03426284174272));
#57938=CARTESIAN_POINT('Ctrl Pts',(0.499547962340821,-1.,-4.02755813980101));
#57939=CARTESIAN_POINT('Ctrl Pts',(0.499547962340821,1.,-4.02755813980101));
#57940=CARTESIAN_POINT('Ctrl Pts',(0.495812444326251,-1.,-4.02084308851832));
#57941=CARTESIAN_POINT('Ctrl Pts',(0.495812444326251,1.,-4.02084308851832));
#57942=CARTESIAN_POINT('Ctrl Pts',(0.492115383418018,-1.,-4.01411733503546));
#57943=CARTESIAN_POINT('Ctrl Pts',(0.492115383418018,1.,-4.01411733503546));
#57944=CARTESIAN_POINT('Ctrl Pts',(0.488457130424633,-1.,-4.0073800839099));
#57945=CARTESIAN_POINT('Ctrl Pts',(0.488457130424633,1.,-4.0073800839099));
#57946=CARTESIAN_POINT('Ctrl Pts',(0.484838042421834,-1.,-4.00063045119288));
#57947=CARTESIAN_POINT('Ctrl Pts',(0.484838042421834,1.,-4.00063045119288));
#57948=CARTESIAN_POINT('Ctrl Pts',(0.481258512209675,-1.,-3.99386775880679));
#57949=CARTESIAN_POINT('Ctrl Pts',(0.481258512209675,1.,-3.99386775880679));
#57950=CARTESIAN_POINT('Ctrl Pts',(0.477718999122027,-1.,-3.98709184306738));
#57951=CARTESIAN_POINT('Ctrl Pts',(0.477718999122027,1.,-3.98709184306738));
#57952=CARTESIAN_POINT('Ctrl Pts',(0.474220061019509,-1.,-3.98030338044409));
#57953=CARTESIAN_POINT('Ctrl Pts',(0.474220061019509,1.,-3.98030338044409));
#57954=CARTESIAN_POINT('Ctrl Pts',(0.470762379613439,-1.,-3.97350414289392));
#57955=CARTESIAN_POINT('Ctrl Pts',(0.470762379613439,1.,-3.97350414289392));
#57956=CARTESIAN_POINT('Ctrl Pts',(0.467346690880643,-1.,-3.9666962227393));
#57957=CARTESIAN_POINT('Ctrl Pts',(0.467346690880643,1.,-3.9666962227393));
#57958=CARTESIAN_POINT('Ctrl Pts',(0.463973722115733,-1.,-3.95988133243538));
#57959=CARTESIAN_POINT('Ctrl Pts',(0.463973722115733,1.,-3.95988133243538));
#57960=CARTESIAN_POINT('Ctrl Pts',(0.460644124429121,-1.,-3.95306005817364));
#57961=CARTESIAN_POINT('Ctrl Pts',(0.460644124429121,1.,-3.95306005817364));
#57962=CARTESIAN_POINT('Ctrl Pts',(0.457358410451682,-1.,-3.94623117206678));
#57963=CARTESIAN_POINT('Ctrl Pts',(0.457358410451682,1.,-3.94623117206678));
#57964=CARTESIAN_POINT('Ctrl Pts',(0.454116879027584,-1.,-3.93939080846298));
#57965=CARTESIAN_POINT('Ctrl Pts',(0.454116879027584,1.,-3.93939080846298));
#57966=CARTESIAN_POINT('Ctrl Pts',(0.450919768356348,-1.,-3.93253407403123));
#57967=CARTESIAN_POINT('Ctrl Pts',(0.450919768356348,1.,-3.93253407403123));
#57968=CARTESIAN_POINT('Ctrl Pts',(0.447767416837292,-1.,-3.92565674143416));
#57969=CARTESIAN_POINT('Ctrl Pts',(0.447767416837292,1.,-3.92565674143416));
#57970=CARTESIAN_POINT('Ctrl Pts',(0.44466043023059,-1.,-3.91875701610719));
#57971=CARTESIAN_POINT('Ctrl Pts',(0.44466043023059,1.,-3.91875701610719));
#57972=CARTESIAN_POINT('Ctrl Pts',(0.441599824524054,-1.,-3.91183704069153));
#57973=CARTESIAN_POINT('Ctrl Pts',(0.441599824524054,1.,-3.91183704069153));
#57974=CARTESIAN_POINT('Ctrl Pts',(0.438587235458249,-1.,-3.90490512938563));
#57975=CARTESIAN_POINT('Ctrl Pts',(0.438587235458249,1.,-3.90490512938563));
#57976=CARTESIAN_POINT('Ctrl Pts',(0.435624629433527,-1.,-3.89797256655462));
#57977=CARTESIAN_POINT('Ctrl Pts',(0.435624629433527,1.,-3.89797256655462));
#57978=CARTESIAN_POINT('Ctrl Pts',(0.432713929544458,-1.,-3.89104947940611));
#57979=CARTESIAN_POINT('Ctrl Pts',(0.432713929544458,1.,-3.89104947940611));
#57980=CARTESIAN_POINT('Ctrl Pts',(0.429856640579741,-1.,-3.88414070943341));
#57981=CARTESIAN_POINT('Ctrl Pts',(0.429856640579741,1.,-3.88414070943341));
#57982=CARTESIAN_POINT('Ctrl Pts',(0.427053541173457,-1.,-3.87724240306597));
#57983=CARTESIAN_POINT('Ctrl Pts',(0.427053541173457,1.,-3.87724240306597));
#57984=CARTESIAN_POINT('Ctrl Pts',(0.42430417319511,-1.,-3.87033643487851));
#57985=CARTESIAN_POINT('Ctrl Pts',(0.42430417319511,1.,-3.87033643487851));
#57986=CARTESIAN_POINT('Ctrl Pts',(0.421607423177534,-1.,-3.86339652542709));
#57987=CARTESIAN_POINT('Ctrl Pts',(0.421607423177534,1.,-3.86339652542709));
#57988=CARTESIAN_POINT('Ctrl Pts',(0.418962468086773,-1.,-3.85639825647996));
#57989=CARTESIAN_POINT('Ctrl Pts',(0.418962468086773,1.,-3.85639825647996));
#57990=CARTESIAN_POINT('Ctrl Pts',(0.416369678052906,-1.,-3.84932864157497));
#57991=CARTESIAN_POINT('Ctrl Pts',(0.416369678052906,1.,-3.84932864157497));
#57992=CARTESIAN_POINT('Ctrl Pts',(0.413831367016748,-1.,-3.84219403994762));
#57993=CARTESIAN_POINT('Ctrl Pts',(0.413831367016748,1.,-3.84219403994762));
#57994=CARTESIAN_POINT('Ctrl Pts',(0.411353038798518,-1.,-3.83503345578698));
#57995=CARTESIAN_POINT('Ctrl Pts',(0.411353038798518,1.,-3.83503345578698));
#57996=CARTESIAN_POINT('Ctrl Pts',(0.408942371447459,-1.,-3.82790724256471));
#57997=CARTESIAN_POINT('Ctrl Pts',(0.408942371447459,1.,-3.82790724256471));
#57998=CARTESIAN_POINT('Ctrl Pts',(0.406607038258985,-1.,-3.8208730391381));
#57999=CARTESIAN_POINT('Ctrl Pts',(0.406607038258985,1.,-3.8208730391381));
#58000=CARTESIAN_POINT('Ctrl Pts',(0.404352694628273,-1.,-3.81396374287793));
#58001=CARTESIAN_POINT('Ctrl Pts',(0.404352694628273,1.,-3.81396374287793));
#58002=CARTESIAN_POINT('Ctrl Pts',(0.402181320148435,-1.,-3.80716881962728));
#58003=CARTESIAN_POINT('Ctrl Pts',(0.402181320148435,1.,-3.80716881962728));
#58004=CARTESIAN_POINT('Ctrl Pts',(0.4000883465046,-1.,-3.80040370384546));
#58005=CARTESIAN_POINT('Ctrl Pts',(0.4000883465046,1.,-3.80040370384546));
#58006=CARTESIAN_POINT('Ctrl Pts',(0.398064818683969,-1.,-3.7935288716329));
#58007=CARTESIAN_POINT('Ctrl Pts',(0.398064818683969,1.,-3.7935288716329));
#58008=CARTESIAN_POINT('Ctrl Pts',(0.39610320533484,-1.,-3.78640521279313));
#58009=CARTESIAN_POINT('Ctrl Pts',(0.39610320533484,1.,-3.78640521279313));
#58010=CARTESIAN_POINT('Ctrl Pts',(0.394202481011499,-1.,-3.77894173114283));
#58011=CARTESIAN_POINT('Ctrl Pts',(0.394202481011499,1.,-3.77894173114283));
#58012=CARTESIAN_POINT('Ctrl Pts',(0.392372786223432,-1.,-3.77114011595967));
#58013=CARTESIAN_POINT('Ctrl Pts',(0.392372786223432,1.,-3.77114011595967));
#58014=CARTESIAN_POINT('Ctrl Pts',(0.390642072979559,-1.,-3.76315635033257));
#58015=CARTESIAN_POINT('Ctrl Pts',(0.390642072979559,1.,-3.76315635033257));
#58016=CARTESIAN_POINT('Ctrl Pts',(0.389054775898701,-1.,-3.75529302895152));
#58017=CARTESIAN_POINT('Ctrl Pts',(0.389054775898701,1.,-3.75529302895152));
#58018=CARTESIAN_POINT('Ctrl Pts',(0.387663020050836,-1.,-3.74792651696654));
#58019=CARTESIAN_POINT('Ctrl Pts',(0.387663020050836,1.,-3.74792651696654));
#58020=CARTESIAN_POINT('Ctrl Pts',(0.386519576222251,-1.,-3.74144965781276));
#58021=CARTESIAN_POINT('Ctrl Pts',(0.386519576222251,1.,-3.74144965781276));
#58022=CARTESIAN_POINT('Ctrl Pts',(0.385670806454565,-1.,-3.73621371845318));
#58023=CARTESIAN_POINT('Ctrl Pts',(0.385670806454565,1.,-3.73621371845318));
#58024=CARTESIAN_POINT('Ctrl Pts',(0.385147887988951,-1.,-3.73245705638843));
#58025=CARTESIAN_POINT('Ctrl Pts',(0.385147887988951,1.,-3.73245705638843));
#58026=CARTESIAN_POINT('Ctrl Pts',(0.385001870183213,-1.,-3.73072465900175));
#58027=CARTESIAN_POINT('Ctrl Pts',(0.385001870183213,1.,-3.73072465900175));
#58028=CARTESIAN_POINT('Ctrl Pts',(0.385047711603462,-1.,-3.73015851028356));
#58029=CARTESIAN_POINT('Ctrl Pts',(0.385047711603462,1.,-3.73015851028356));
#58030=CARTESIAN_POINT('Ctrl Pts',(0.385147278814642,-1.,-3.73010668803042));
#58031=CARTESIAN_POINT('Ctrl Pts',(0.385147278814642,1.,-3.73010668803042));
#58032=CARTESIAN_POINT('Ctrl Pts',(0.385214314776329,-1.,-3.73016218570874));
#58033=CARTESIAN_POINT('Ctrl Pts',(0.385214314776329,1.,-3.73016218570874));
#58034=CARTESIAN_POINT('',(0.581791163835815,1.,-4.15950947128175));
#58035=CARTESIAN_POINT('Ctrl Pts',(0.581791163835815,1.,-4.15950947128175));
#58036=CARTESIAN_POINT('Ctrl Pts',(0.580901211463535,1.,-4.1582129171283));
#58037=CARTESIAN_POINT('Ctrl Pts',(0.579124568914235,1.,-4.15561864788576));
#58038=CARTESIAN_POINT('Ctrl Pts',(0.576469391676688,1.,-4.151723761217));
#58039=CARTESIAN_POINT('Ctrl Pts',(0.572948736069522,1.,-4.14652361068081));
#58040=CARTESIAN_POINT('Ctrl Pts',(0.568580610189774,1.,-4.14001179830547));
#58041=CARTESIAN_POINT('Ctrl Pts',(0.564245279537148,1.,-4.13348835727104));
#58042=CARTESIAN_POINT('Ctrl Pts',(0.559942890594773,1.,-4.12695329951961));
#58043=CARTESIAN_POINT('Ctrl Pts',(0.555673636129977,1.,-4.12040666195664));
#58044=CARTESIAN_POINT('Ctrl Pts',(0.551437758497032,1.,-4.11384852024721));
#58045=CARTESIAN_POINT('Ctrl Pts',(0.547235539485636,1.,-4.10727897027977));
#58046=CARTESIAN_POINT('Ctrl Pts',(0.543067286877757,1.,-4.10069810243979));
#58047=CARTESIAN_POINT('Ctrl Pts',(0.538933321179755,1.,-4.09410597627));
#58048=CARTESIAN_POINT('Ctrl Pts',(0.534833963477273,1.,-4.08750259988885));
#58049=CARTESIAN_POINT('Ctrl Pts',(0.53076951872857,1.,-4.08088789536836));
#58050=CARTESIAN_POINT('Ctrl Pts',(0.526740277227498,1.,-4.07426172299847));
#58051=CARTESIAN_POINT('Ctrl Pts',(0.522746528603107,1.,-4.06762394471314));
#58052=CARTESIAN_POINT('Ctrl Pts',(0.518788572336923,1.,-4.06097448038013));
#58053=CARTESIAN_POINT('Ctrl Pts',(0.514866728193016,1.,-4.05431335771199));
#58054=CARTESIAN_POINT('Ctrl Pts',(0.51098134921897,1.,-4.04764078815447));
#58055=CARTESIAN_POINT('Ctrl Pts',(0.507132823288136,1.,-4.04095715148915));
#58056=CARTESIAN_POINT('Ctrl Pts',(0.503321556915346,1.,-4.03426284174272));
#58057=CARTESIAN_POINT('Ctrl Pts',(0.499547962340821,1.,-4.02755813980101));
#58058=CARTESIAN_POINT('Ctrl Pts',(0.495812444326251,1.,-4.02084308851832));
#58059=CARTESIAN_POINT('Ctrl Pts',(0.492115383418018,1.,-4.01411733503546));
#58060=CARTESIAN_POINT('Ctrl Pts',(0.488457130424633,1.,-4.0073800839099));
#58061=CARTESIAN_POINT('Ctrl Pts',(0.484838042421834,1.,-4.00063045119288));
#58062=CARTESIAN_POINT('Ctrl Pts',(0.481258512209675,1.,-3.99386775880679));
#58063=CARTESIAN_POINT('Ctrl Pts',(0.477718999122027,1.,-3.98709184306738));
#58064=CARTESIAN_POINT('Ctrl Pts',(0.474220061019509,1.,-3.98030338044409));
#58065=CARTESIAN_POINT('Ctrl Pts',(0.470762379613439,1.,-3.97350414289392));
#58066=CARTESIAN_POINT('Ctrl Pts',(0.467346690880643,1.,-3.9666962227393));
#58067=CARTESIAN_POINT('Ctrl Pts',(0.463973722115733,1.,-3.95988133243538));
#58068=CARTESIAN_POINT('Ctrl Pts',(0.460644124429121,1.,-3.95306005817364));
#58069=CARTESIAN_POINT('Ctrl Pts',(0.457358410451682,1.,-3.94623117206678));
#58070=CARTESIAN_POINT('Ctrl Pts',(0.454116879027584,1.,-3.93939080846298));
#58071=CARTESIAN_POINT('Ctrl Pts',(0.450919768356348,1.,-3.93253407403123));
#58072=CARTESIAN_POINT('Ctrl Pts',(0.447767416837292,1.,-3.92565674143416));
#58073=CARTESIAN_POINT('Ctrl Pts',(0.44466043023059,1.,-3.91875701610719));
#58074=CARTESIAN_POINT('Ctrl Pts',(0.441599824524054,1.,-3.91183704069153));
#58075=CARTESIAN_POINT('Ctrl Pts',(0.438587235458249,1.,-3.90490512938563));
#58076=CARTESIAN_POINT('Ctrl Pts',(0.435624629433527,1.,-3.89797256655462));
#58077=CARTESIAN_POINT('Ctrl Pts',(0.432713929544458,1.,-3.89104947940611));
#58078=CARTESIAN_POINT('Ctrl Pts',(0.429856640579741,1.,-3.88414070943341));
#58079=CARTESIAN_POINT('Ctrl Pts',(0.427053541173457,1.,-3.87724240306597));
#58080=CARTESIAN_POINT('Ctrl Pts',(0.42430417319511,1.,-3.87033643487851));
#58081=CARTESIAN_POINT('Ctrl Pts',(0.421607423177534,1.,-3.86339652542709));
#58082=CARTESIAN_POINT('Ctrl Pts',(0.418962468086773,1.,-3.85639825647996));
#58083=CARTESIAN_POINT('Ctrl Pts',(0.416369678052906,1.,-3.84932864157497));
#58084=CARTESIAN_POINT('Ctrl Pts',(0.413831367016748,1.,-3.84219403994762));
#58085=CARTESIAN_POINT('Ctrl Pts',(0.411353038798518,1.,-3.83503345578698));
#58086=CARTESIAN_POINT('Ctrl Pts',(0.408942371447459,1.,-3.82790724256471));
#58087=CARTESIAN_POINT('Ctrl Pts',(0.406607038258985,1.,-3.8208730391381));
#58088=CARTESIAN_POINT('Ctrl Pts',(0.404352694628273,1.,-3.81396374287793));
#58089=CARTESIAN_POINT('Ctrl Pts',(0.402181320148435,1.,-3.80716881962728));
#58090=CARTESIAN_POINT('Ctrl Pts',(0.4000883465046,1.,-3.80040370384546));
#58091=CARTESIAN_POINT('Ctrl Pts',(0.398064818683969,1.,-3.7935288716329));
#58092=CARTESIAN_POINT('Ctrl Pts',(0.39610320533484,1.,-3.78640521279313));
#58093=CARTESIAN_POINT('Ctrl Pts',(0.394202481011499,1.,-3.77894173114283));
#58094=CARTESIAN_POINT('Ctrl Pts',(0.392372786223432,1.,-3.77114011595967));
#58095=CARTESIAN_POINT('Ctrl Pts',(0.390642072979559,1.,-3.76315635033257));
#58096=CARTESIAN_POINT('Ctrl Pts',(0.389054775898701,1.,-3.75529302895152));
#58097=CARTESIAN_POINT('Ctrl Pts',(0.387663020050836,1.,-3.74792651696654));
#58098=CARTESIAN_POINT('Ctrl Pts',(0.386519576222251,1.,-3.74144965781276));
#58099=CARTESIAN_POINT('Ctrl Pts',(0.385670806454565,1.,-3.73621371845318));
#58100=CARTESIAN_POINT('Ctrl Pts',(0.385187124634206,1.,-3.73273893363406));
#58101=CARTESIAN_POINT('Ctrl Pts',(0.385031656499163,1.,-3.73106082862548));
#58102=CARTESIAN_POINT('Ctrl Pts',(0.385037797881504,1.,-3.73040527621055));
#58103=CARTESIAN_POINT('Ctrl Pts',(0.385087139000374,1.,-3.73021431755274));
#58104=CARTESIAN_POINT('Ctrl Pts',(0.385112848330761,1.,-3.73017266276651));
#58105=CARTESIAN_POINT('',(0.581791163835815,0.,-4.15950947128175));
#58106=CARTESIAN_POINT('Ctrl Pts',(0.786322922920599,-1.,-3.66663282329846));
#58107=CARTESIAN_POINT('Ctrl Pts',(0.786322922920599,1.,-3.66663282329846));
#58108=CARTESIAN_POINT('Ctrl Pts',(0.786369528183326,-1.,-3.66655932661986));
#58109=CARTESIAN_POINT('Ctrl Pts',(0.786369528183326,1.,-3.66655932661986));
#58110=CARTESIAN_POINT('Ctrl Pts',(0.786480236185696,-1.,-3.66657784455334));
#58111=CARTESIAN_POINT('Ctrl Pts',(0.786480236185696,1.,-3.66657784455334));
#58112=CARTESIAN_POINT('Ctrl Pts',(0.786698783542764,-1.,-3.66710211820482));
#58113=CARTESIAN_POINT('Ctrl Pts',(0.786698783542764,1.,-3.66710211820482));
#58114=CARTESIAN_POINT('Ctrl Pts',(0.787095252590501,-1.,-3.66879484801113));
#58115=CARTESIAN_POINT('Ctrl Pts',(0.787095252590501,1.,-3.66879484801113));
#58116=CARTESIAN_POINT('Ctrl Pts',(0.787758799995742,-1.,-3.67252923663655));
#58117=CARTESIAN_POINT('Ctrl Pts',(0.787758799995742,1.,-3.67252923663655));
#58118=CARTESIAN_POINT('Ctrl Pts',(0.788569566220285,-1.,-3.67777119516252));
#58119=CARTESIAN_POINT('Ctrl Pts',(0.788569566220285,1.,-3.67777119516252));
#58120=CARTESIAN_POINT('Ctrl Pts',(0.789483546064386,-1.,-3.68428439783905));
#58121=CARTESIAN_POINT('Ctrl Pts',(0.789483546064386,1.,-3.68428439783905));
#58122=CARTESIAN_POINT('Ctrl Pts',(0.790436284988787,-1.,-3.69172044327364));
#58123=CARTESIAN_POINT('Ctrl Pts',(0.790436284988787,1.,-3.69172044327364));
#58124=CARTESIAN_POINT('Ctrl Pts',(0.79135657569598,-1.,-3.69968940808721));
#58125=CARTESIAN_POINT('Ctrl Pts',(0.79135657569598,1.,-3.69968940808721));
#58126=CARTESIAN_POINT('Ctrl Pts',(0.792177688845817,-1.,-3.70781724021806));
#58127=CARTESIAN_POINT('Ctrl Pts',(0.792177688845817,1.,-3.70781724021806));
#58128=CARTESIAN_POINT('Ctrl Pts',(0.792848377370287,-1.,-3.71580242396124));
#58129=CARTESIAN_POINT('Ctrl Pts',(0.792848377370287,1.,-3.71580242396124));
#58130=CARTESIAN_POINT('Ctrl Pts',(0.793347023784204,-1.,-3.72348797293734));
#58131=CARTESIAN_POINT('Ctrl Pts',(0.793347023784204,1.,-3.72348797293734));
#58132=CARTESIAN_POINT('Ctrl Pts',(0.793682750269684,-1.,-3.73086914695805));
#58133=CARTESIAN_POINT('Ctrl Pts',(0.793682750269684,1.,-3.73086914695805));
#58134=CARTESIAN_POINT('Ctrl Pts',(0.793882700937016,-1.,-3.73803280541687));
#58135=CARTESIAN_POINT('Ctrl Pts',(0.793882700937016,1.,-3.73803280541687));
#58136=CARTESIAN_POINT('Ctrl Pts',(0.793982700459951,-1.,-3.74511357728861));
#58137=CARTESIAN_POINT('Ctrl Pts',(0.793982700459951,1.,-3.74511357728861));
#58138=CARTESIAN_POINT('Ctrl Pts',(0.794017347371377,-1.,-3.75224692493864));
#58139=CARTESIAN_POINT('Ctrl Pts',(0.794017347371377,1.,-3.75224692493864));
#58140=CARTESIAN_POINT('Ctrl Pts',(0.794008429134907,-1.,-3.75951468666257));
#58141=CARTESIAN_POINT('Ctrl Pts',(0.794008429134907,1.,-3.75951468666257));
#58142=CARTESIAN_POINT('Ctrl Pts',(0.793961083688991,-1.,-3.76692626931111));
#58143=CARTESIAN_POINT('Ctrl Pts',(0.793961083688991,1.,-3.76692626931111));
#58144=CARTESIAN_POINT('Ctrl Pts',(0.793870523787407,-1.,-3.77444863801212));
#58145=CARTESIAN_POINT('Ctrl Pts',(0.793870523787407,1.,-3.77444863801212));
#58146=CARTESIAN_POINT('Ctrl Pts',(0.7937262357813,-1.,-3.78202460377598));
#58147=CARTESIAN_POINT('Ctrl Pts',(0.7937262357813,1.,-3.78202460377598));
#58148=CARTESIAN_POINT('Ctrl Pts',(0.793516871680993,-1.,-3.78959439439235));
#58149=CARTESIAN_POINT('Ctrl Pts',(0.793516871680993,1.,-3.78959439439235));
#58150=CARTESIAN_POINT('Ctrl Pts',(0.793235612973273,-1.,-3.79711921389897));
#58151=CARTESIAN_POINT('Ctrl Pts',(0.793235612973273,1.,-3.79711921389897));
#58152=CARTESIAN_POINT('Ctrl Pts',(0.792882695234777,-1.,-3.80459229925637));
#58153=CARTESIAN_POINT('Ctrl Pts',(0.792882695234777,1.,-3.80459229925637));
#58154=CARTESIAN_POINT('Ctrl Pts',(0.792462483517634,-1.,-3.81202588694756));
#58155=CARTESIAN_POINT('Ctrl Pts',(0.792462483517634,1.,-3.81202588694756));
#58156=CARTESIAN_POINT('Ctrl Pts',(0.791981740718634,-1.,-3.81944345442249));
#58157=CARTESIAN_POINT('Ctrl Pts',(0.791981740718634,1.,-3.81944345442249));
#58158=CARTESIAN_POINT('Ctrl Pts',(0.791447528662369,-1.,-3.82687033899792));
#58159=CARTESIAN_POINT('Ctrl Pts',(0.791447528662369,1.,-3.82687033899792));
#58160=CARTESIAN_POINT('Ctrl Pts',(0.7908650127053,-1.,-3.83432392054786));
#58161=CARTESIAN_POINT('Ctrl Pts',(0.7908650127053,1.,-3.83432392054786));
#58162=CARTESIAN_POINT('Ctrl Pts',(0.790236124191242,-1.,-3.84180762342454));
#58163=CARTESIAN_POINT('Ctrl Pts',(0.790236124191242,1.,-3.84180762342454));
#58164=CARTESIAN_POINT('Ctrl Pts',(0.789560798155582,-1.,-3.84931637808894));
#58165=CARTESIAN_POINT('Ctrl Pts',(0.789560798155582,1.,-3.84931637808894));
#58166=CARTESIAN_POINT('Ctrl Pts',(0.788837734090671,-1.,-3.85683995872529));
#58167=CARTESIAN_POINT('Ctrl Pts',(0.788837734090671,1.,-3.85683995872529));
#58168=CARTESIAN_POINT('Ctrl Pts',(0.788065315093777,-1.,-3.86436702561345));
#58169=CARTESIAN_POINT('Ctrl Pts',(0.788065315093777,1.,-3.86436702561345));
#58170=CARTESIAN_POINT('Ctrl Pts',(0.787242527617999,-1.,-3.87188916600912));
#58171=CARTESIAN_POINT('Ctrl Pts',(0.787242527617999,1.,-3.87188916600912));
#58172=CARTESIAN_POINT('Ctrl Pts',(0.786369675812608,-1.,-3.8794040281819));
#58173=CARTESIAN_POINT('Ctrl Pts',(0.786369675812608,1.,-3.8794040281819));
#58174=CARTESIAN_POINT('Ctrl Pts',(0.78544789034073,-1.,-3.88691313167398));
#58175=CARTESIAN_POINT('Ctrl Pts',(0.78544789034073,1.,-3.88691313167398));
#58176=CARTESIAN_POINT('Ctrl Pts',(0.784478799358336,-1.,-3.89442039235103));
#58177=CARTESIAN_POINT('Ctrl Pts',(0.784478799358336,1.,-3.89442039235103));
#58178=CARTESIAN_POINT('Ctrl Pts',(0.783464141529081,-1.,-3.9019303904397));
#58179=CARTESIAN_POINT('Ctrl Pts',(0.783464141529081,1.,-3.9019303904397));
#58180=CARTESIAN_POINT('Ctrl Pts',(0.782405395622764,-1.,-3.90944671004542));
#58181=CARTESIAN_POINT('Ctrl Pts',(0.782405395622764,1.,-3.90944671004542));
#58182=CARTESIAN_POINT('Ctrl Pts',(0.781303428618366,-1.,-3.91697036054676));
#58183=CARTESIAN_POINT('Ctrl Pts',(0.781303428618366,1.,-3.91697036054676));
#58184=CARTESIAN_POINT('Ctrl Pts',(0.780158678615542,-1.,-3.92450058323823));
#58185=CARTESIAN_POINT('Ctrl Pts',(0.780158678615542,1.,-3.92450058323823));
#58186=CARTESIAN_POINT('Ctrl Pts',(0.77897130813482,-1.,-3.93203552473174));
#58187=CARTESIAN_POINT('Ctrl Pts',(0.77897130813482,1.,-3.93203552473174));
#58188=CARTESIAN_POINT('Ctrl Pts',(0.777741370568558,-1.,-3.93957296768103));
#58189=CARTESIAN_POINT('Ctrl Pts',(0.777741370568558,1.,-3.93957296768103));
#58190=CARTESIAN_POINT('Ctrl Pts',(0.776468966697921,-1.,-3.94711101619447));
#58191=CARTESIAN_POINT('Ctrl Pts',(0.776468966697921,1.,-3.94711101619447));
#58192=CARTESIAN_POINT('Ctrl Pts',(0.775154418039351,-1.,-3.9546488545231));
#58193=CARTESIAN_POINT('Ctrl Pts',(0.775154418039351,1.,-3.9546488545231));
#58194=CARTESIAN_POINT('Ctrl Pts',(0.773798212026565,-1.,-3.96218649639807));
#58195=CARTESIAN_POINT('Ctrl Pts',(0.773798212026565,1.,-3.96218649639807));
#58196=CARTESIAN_POINT('Ctrl Pts',(0.772400931772136,-1.,-3.96972446532772));
#58197=CARTESIAN_POINT('Ctrl Pts',(0.772400931772136,1.,-3.96972446532772));
#58198=CARTESIAN_POINT('Ctrl Pts',(0.77096319003047,-1.,-3.97726349165488));
#58199=CARTESIAN_POINT('Ctrl Pts',(0.77096319003047,1.,-3.97726349165488));
#58200=CARTESIAN_POINT('Ctrl Pts',(0.769485566245544,-1.,-3.98480422348451));
#58201=CARTESIAN_POINT('Ctrl Pts',(0.769485566245544,1.,-3.98480422348451));
#58202=CARTESIAN_POINT('Ctrl Pts',(0.767968531377914,-1.,-3.9923468788101));
#58203=CARTESIAN_POINT('Ctrl Pts',(0.767968531377914,1.,-3.9923468788101));
#58204=CARTESIAN_POINT('Ctrl Pts',(0.766412457136063,-1.,-3.99989129179622));
#58205=CARTESIAN_POINT('Ctrl Pts',(0.766412457136063,1.,-3.99989129179622));
#58206=CARTESIAN_POINT('Ctrl Pts',(0.764817648785197,-1.,-4.00743706791509));
#58207=CARTESIAN_POINT('Ctrl Pts',(0.764817648785197,1.,-4.00743706791509));
#58208=CARTESIAN_POINT('Ctrl Pts',(0.763184371182935,-1.,-4.01498370680496));
#58209=CARTESIAN_POINT('Ctrl Pts',(0.763184371182935,1.,-4.01498370680496));
#58210=CARTESIAN_POINT('Ctrl Pts',(0.761512875859804,-1.,-4.02253072741268));
#58211=CARTESIAN_POINT('Ctrl Pts',(0.761512875859804,1.,-4.02253072741268));
#58212=CARTESIAN_POINT('Ctrl Pts',(0.759803433243751,-1.,-4.03007781954412));
#58213=CARTESIAN_POINT('Ctrl Pts',(0.759803433243751,1.,-4.03007781954412));
#58214=CARTESIAN_POINT('Ctrl Pts',(0.758056338884944,-1.,-4.03762485803119));
#58215=CARTESIAN_POINT('Ctrl Pts',(0.758056338884944,1.,-4.03762485803119));
#58216=CARTESIAN_POINT('Ctrl Pts',(0.75627190236958,-1.,-4.04517182653997));
#58217=CARTESIAN_POINT('Ctrl Pts',(0.75627190236958,1.,-4.04517182653997));
#58218=CARTESIAN_POINT('Ctrl Pts',(0.754450441816078,-1.,-4.05271876687915));
#58219=CARTESIAN_POINT('Ctrl Pts',(0.754450441816078,1.,-4.05271876687915));
#58220=CARTESIAN_POINT('Ctrl Pts',(0.752592276483072,-1.,-4.06026572221515));
#58221=CARTESIAN_POINT('Ctrl Pts',(0.752592276483072,1.,-4.06026572221515));
#58222=CARTESIAN_POINT('Ctrl Pts',(0.750697720484036,-1.,-4.06781267242378));
#58223=CARTESIAN_POINT('Ctrl Pts',(0.750697720484036,1.,-4.06781267242378));
#58224=CARTESIAN_POINT('Ctrl Pts',(0.748767076680557,-1.,-4.07535951056152));
#58225=CARTESIAN_POINT('Ctrl Pts',(0.748767076680557,1.,-4.07535951056152));
#58226=CARTESIAN_POINT('Ctrl Pts',(0.746800631492315,-1.,-4.08290608095642));
#58227=CARTESIAN_POINT('Ctrl Pts',(0.746800631492315,1.,-4.08290608095642));
#58228=CARTESIAN_POINT('Ctrl Pts',(0.7447986497065,-1.,-4.09045220253573));
#58229=CARTESIAN_POINT('Ctrl Pts',(0.7447986497065,1.,-4.09045220253573));
#58230=CARTESIAN_POINT('Ctrl Pts',(0.742761369689841,-1.,-4.09799769702611));
#58231=CARTESIAN_POINT('Ctrl Pts',(0.742761369689841,1.,-4.09799769702611));
#58232=CARTESIAN_POINT('Ctrl Pts',(0.740688998553376,-1.,-4.10554241757547));
#58233=CARTESIAN_POINT('Ctrl Pts',(0.740688998553376,1.,-4.10554241757547));
#58234=CARTESIAN_POINT('Ctrl Pts',(0.738581708225843,-1.,-4.11308626951927));
#58235=CARTESIAN_POINT('Ctrl Pts',(0.738581708225843,1.,-4.11308626951927));
#58236=CARTESIAN_POINT('Ctrl Pts',(0.736439634331344,-1.,-4.120629196238));
#58237=CARTESIAN_POINT('Ctrl Pts',(0.736439634331344,1.,-4.120629196238));
#58238=CARTESIAN_POINT('Ctrl Pts',(0.734698226764092,-1.,-4.12666277570844));
#58239=CARTESIAN_POINT('Ctrl Pts',(0.734698226764092,1.,-4.12666277570844));
#58240=CARTESIAN_POINT('Ctrl Pts',(0.733376589323546,-1.,-4.13118752795207));
#58241=CARTESIAN_POINT('Ctrl Pts',(0.733376589323546,1.,-4.13118752795207));
#58242=CARTESIAN_POINT('Ctrl Pts',(0.732488575135159,-1.,-4.1342038373684));
#58243=CARTESIAN_POINT('Ctrl Pts',(0.732488575135159,1.,-4.1342038373684));
#58244=CARTESIAN_POINT('Ctrl Pts',(0.73204283740062,-1.,-4.13571194405636));
#58245=CARTESIAN_POINT('Ctrl Pts',(0.73204283740062,1.,-4.13571194405636));
#58246=CARTESIAN_POINT('',(0.786422660831986,1.,-3.66661143271685));
#58247=CARTESIAN_POINT('Ctrl Pts',(0.786422660831985,-1.,-3.66661143271685));
#58248=CARTESIAN_POINT('Ctrl Pts',(0.786422660831985,-0.666666666666667,
-3.66661143271685));
#58249=CARTESIAN_POINT('Ctrl Pts',(0.786422660831985,-0.333333333333333,
-3.66661143271685));
#58250=CARTESIAN_POINT('Ctrl Pts',(0.786422660831985,0.333333333333333,
-3.66661143271685));
#58251=CARTESIAN_POINT('Ctrl Pts',(0.786422660831985,0.666666666666667,
-3.66661143271685));
#58252=CARTESIAN_POINT('Ctrl Pts',(0.786422660831985,1.,-3.66661143271685));
#58253=CARTESIAN_POINT('',(0.73204283740062,1.,-4.13571194405636));
#58254=CARTESIAN_POINT('',(0.73204283740062,0.,-4.13571194405636));
#58255=CARTESIAN_POINT('Ctrl Pts',(0.786422660831986,1.,-3.66661143271685));
#58256=CARTESIAN_POINT('Ctrl Pts',(0.786459983895432,1.,-3.6666431041522));
#58257=CARTESIAN_POINT('Ctrl Pts',(0.786565919558984,1.,-3.66680946938293));
#58258=CARTESIAN_POINT('Ctrl Pts',(0.786774337198062,1.,-3.66743103898702));
#58259=CARTESIAN_POINT('Ctrl Pts',(0.787145041181546,1.,-3.66907505398677));
#58260=CARTESIAN_POINT('Ctrl Pts',(0.787758799995742,1.,-3.67252923663655));
#58261=CARTESIAN_POINT('Ctrl Pts',(0.788569566220285,1.,-3.67777119516252));
#58262=CARTESIAN_POINT('Ctrl Pts',(0.789483546064386,1.,-3.68428439783905));
#58263=CARTESIAN_POINT('Ctrl Pts',(0.790436284988787,1.,-3.69172044327364));
#58264=CARTESIAN_POINT('Ctrl Pts',(0.79135657569598,1.,-3.69968940808721));
#58265=CARTESIAN_POINT('Ctrl Pts',(0.792177688845817,1.,-3.70781724021806));
#58266=CARTESIAN_POINT('Ctrl Pts',(0.792848377370287,1.,-3.71580242396124));
#58267=CARTESIAN_POINT('Ctrl Pts',(0.793347023784204,1.,-3.72348797293734));
#58268=CARTESIAN_POINT('Ctrl Pts',(0.793682750269684,1.,-3.73086914695805));
#58269=CARTESIAN_POINT('Ctrl Pts',(0.793882700937016,1.,-3.73803280541687));
#58270=CARTESIAN_POINT('Ctrl Pts',(0.793982700459951,1.,-3.74511357728861));
#58271=CARTESIAN_POINT('Ctrl Pts',(0.794017347371377,1.,-3.75224692493864));
#58272=CARTESIAN_POINT('Ctrl Pts',(0.794008429134907,1.,-3.75951468666257));
#58273=CARTESIAN_POINT('Ctrl Pts',(0.793961083688991,1.,-3.76692626931111));
#58274=CARTESIAN_POINT('Ctrl Pts',(0.793870523787407,1.,-3.77444863801212));
#58275=CARTESIAN_POINT('Ctrl Pts',(0.7937262357813,1.,-3.78202460377598));
#58276=CARTESIAN_POINT('Ctrl Pts',(0.793516871680993,1.,-3.78959439439235));
#58277=CARTESIAN_POINT('Ctrl Pts',(0.793235612973273,1.,-3.79711921389897));
#58278=CARTESIAN_POINT('Ctrl Pts',(0.792882695234777,1.,-3.80459229925637));
#58279=CARTESIAN_POINT('Ctrl Pts',(0.792462483517634,1.,-3.81202588694756));
#58280=CARTESIAN_POINT('Ctrl Pts',(0.791981740718634,1.,-3.81944345442249));
#58281=CARTESIAN_POINT('Ctrl Pts',(0.791447528662369,1.,-3.82687033899792));
#58282=CARTESIAN_POINT('Ctrl Pts',(0.7908650127053,1.,-3.83432392054786));
#58283=CARTESIAN_POINT('Ctrl Pts',(0.790236124191242,1.,-3.84180762342454));
#58284=CARTESIAN_POINT('Ctrl Pts',(0.789560798155582,1.,-3.84931637808894));
#58285=CARTESIAN_POINT('Ctrl Pts',(0.788837734090671,1.,-3.85683995872529));
#58286=CARTESIAN_POINT('Ctrl Pts',(0.788065315093777,1.,-3.86436702561345));
#58287=CARTESIAN_POINT('Ctrl Pts',(0.787242527617999,1.,-3.87188916600912));
#58288=CARTESIAN_POINT('Ctrl Pts',(0.786369675812608,1.,-3.8794040281819));
#58289=CARTESIAN_POINT('Ctrl Pts',(0.78544789034073,1.,-3.88691313167398));
#58290=CARTESIAN_POINT('Ctrl Pts',(0.784478799358336,1.,-3.89442039235103));
#58291=CARTESIAN_POINT('Ctrl Pts',(0.783464141529081,1.,-3.9019303904397));
#58292=CARTESIAN_POINT('Ctrl Pts',(0.782405395622764,1.,-3.90944671004542));
#58293=CARTESIAN_POINT('Ctrl Pts',(0.781303428618366,1.,-3.91697036054676));
#58294=CARTESIAN_POINT('Ctrl Pts',(0.780158678615542,1.,-3.92450058323823));
#58295=CARTESIAN_POINT('Ctrl Pts',(0.77897130813482,1.,-3.93203552473174));
#58296=CARTESIAN_POINT('Ctrl Pts',(0.777741370568558,1.,-3.93957296768103));
#58297=CARTESIAN_POINT('Ctrl Pts',(0.776468966697921,1.,-3.94711101619447));
#58298=CARTESIAN_POINT('Ctrl Pts',(0.775154418039351,1.,-3.9546488545231));
#58299=CARTESIAN_POINT('Ctrl Pts',(0.773798212026565,1.,-3.96218649639807));
#58300=CARTESIAN_POINT('Ctrl Pts',(0.772400931772136,1.,-3.96972446532772));
#58301=CARTESIAN_POINT('Ctrl Pts',(0.77096319003047,1.,-3.97726349165488));
#58302=CARTESIAN_POINT('Ctrl Pts',(0.769485566245544,1.,-3.98480422348451));
#58303=CARTESIAN_POINT('Ctrl Pts',(0.767968531377914,1.,-3.9923468788101));
#58304=CARTESIAN_POINT('Ctrl Pts',(0.766412457136063,1.,-3.99989129179622));
#58305=CARTESIAN_POINT('Ctrl Pts',(0.764817648785197,1.,-4.00743706791509));
#58306=CARTESIAN_POINT('Ctrl Pts',(0.763184371182935,1.,-4.01498370680496));
#58307=CARTESIAN_POINT('Ctrl Pts',(0.761512875859804,1.,-4.02253072741268));
#58308=CARTESIAN_POINT('Ctrl Pts',(0.759803433243751,1.,-4.03007781954412));
#58309=CARTESIAN_POINT('Ctrl Pts',(0.758056338884944,1.,-4.03762485803119));
#58310=CARTESIAN_POINT('Ctrl Pts',(0.75627190236958,1.,-4.04517182653997));
#58311=CARTESIAN_POINT('Ctrl Pts',(0.754450441816078,1.,-4.05271876687915));
#58312=CARTESIAN_POINT('Ctrl Pts',(0.752592276483072,1.,-4.06026572221515));
#58313=CARTESIAN_POINT('Ctrl Pts',(0.750697720484036,1.,-4.06781267242378));
#58314=CARTESIAN_POINT('Ctrl Pts',(0.748767076680557,1.,-4.07535951056152));
#58315=CARTESIAN_POINT('Ctrl Pts',(0.746800631492315,1.,-4.08290608095642));
#58316=CARTESIAN_POINT('Ctrl Pts',(0.7447986497065,1.,-4.09045220253573));
#58317=CARTESIAN_POINT('Ctrl Pts',(0.742761369689841,1.,-4.09799769702611));
#58318=CARTESIAN_POINT('Ctrl Pts',(0.740688998553376,1.,-4.10554241757547));
#58319=CARTESIAN_POINT('Ctrl Pts',(0.738581708225843,1.,-4.11308626951927));
#58320=CARTESIAN_POINT('Ctrl Pts',(0.736439634331344,1.,-4.120629196238));
#58321=CARTESIAN_POINT('Ctrl Pts',(0.734698226764092,1.,-4.12666277570844));
#58322=CARTESIAN_POINT('Ctrl Pts',(0.733376589323546,1.,-4.13118752795207));
#58323=CARTESIAN_POINT('Ctrl Pts',(0.732488575135159,1.,-4.1342038373684));
#58324=CARTESIAN_POINT('Ctrl Pts',(0.73204283740062,1.,-4.13571194405636));
#58325=CARTESIAN_POINT('Origin',(0.73204283740062,0.,-4.13571194405636));
#58326=CARTESIAN_POINT('',(0.581791163835815,1.,-4.15950947128175));
#58327=CARTESIAN_POINT('Origin',(0.,0.,0.));
#58328=CARTESIAN_POINT('',(0.963899035117248,1.,-3.62400312501245));
#58329=CARTESIAN_POINT('Origin',(0.,1.,0.));
#58330=CARTESIAN_POINT('Ctrl Pts',(0.963899035117248,1.,-3.62400312501246));
#58331=CARTESIAN_POINT('Ctrl Pts',(0.963899035117248,0.666666666666667,
-3.62400312501246));
#58332=CARTESIAN_POINT('Ctrl Pts',(0.963899035117248,0.333333333333333,
-3.62400312501246));
#58333=CARTESIAN_POINT('Ctrl Pts',(0.963899035117248,-0.333333333333333,
-3.62400312501246));
#58334=CARTESIAN_POINT('Ctrl Pts',(0.963899035117249,-0.666666666666667,
-3.62400312501246));
#58335=CARTESIAN_POINT('Ctrl Pts',(0.963899035117249,-1.,-3.62400312501246));
#58336=CARTESIAN_POINT('Ctrl Pts',(1.22531898815164,-1.,-4.01728681790024));
#58337=CARTESIAN_POINT('Ctrl Pts',(1.22531898815164,1.,-4.01728681790024));
#58338=CARTESIAN_POINT('Ctrl Pts',(1.22423716681447,-1.,-4.0161454457032));
#58339=CARTESIAN_POINT('Ctrl Pts',(1.22423716681447,1.,-4.0161454457032));
#58340=CARTESIAN_POINT('Ctrl Pts',(1.22207656456199,-1.,-4.01386104434674));
#58341=CARTESIAN_POINT('Ctrl Pts',(1.22207656456199,1.,-4.01386104434674));
#58342=CARTESIAN_POINT('Ctrl Pts',(1.21884478244983,-1.,-4.01042947142681));
#58343=CARTESIAN_POINT('Ctrl Pts',(1.21884478244983,1.,-4.01042947142681));
#58344=CARTESIAN_POINT('Ctrl Pts',(1.21455398918813,-1.,-4.00584409524937));
#58345=CARTESIAN_POINT('Ctrl Pts',(1.21455398918813,1.,-4.00584409524937));
#58346=CARTESIAN_POINT('Ctrl Pts',(1.20922097030107,-1.,-4.00009577952534));
#58347=CARTESIAN_POINT('Ctrl Pts',(1.20922097030107,1.,-4.00009577952534));
#58348=CARTESIAN_POINT('Ctrl Pts',(1.2039185237544,-1.,-3.99433084800649));
#58349=CARTESIAN_POINT('Ctrl Pts',(1.2039185237544,1.,-3.99433084800649));
#58350=CARTESIAN_POINT('Ctrl Pts',(1.19864679609596,-1.,-3.98854928957287));
#58351=CARTESIAN_POINT('Ctrl Pts',(1.19864679609596,1.,-3.98854928957287));
#58352=CARTESIAN_POINT('Ctrl Pts',(1.19340598349307,-1.,-3.98275111052015));
#58353=CARTESIAN_POINT('Ctrl Pts',(1.19340598349307,1.,-3.98275111052015));
#58354=CARTESIAN_POINT('Ctrl Pts',(1.18819633715285,-1.,-3.97693634766926));
#58355=CARTESIAN_POINT('Ctrl Pts',(1.18819633715285,1.,-3.97693634766926));
#58356=CARTESIAN_POINT('Ctrl Pts',(1.18301815039596,-1.,-3.9711050516465));
#58357=CARTESIAN_POINT('Ctrl Pts',(1.18301815039596,1.,-3.9711050516465));
#58358=CARTESIAN_POINT('Ctrl Pts',(1.17787174135445,-1.,-3.96525726357682));
#58359=CARTESIAN_POINT('Ctrl Pts',(1.17787174135445,1.,-3.96525726357682));
#58360=CARTESIAN_POINT('Ctrl Pts',(1.17275743590327,-1.,-3.95939299213164));
#58361=CARTESIAN_POINT('Ctrl Pts',(1.17275743590327,1.,-3.95939299213164));
#58362=CARTESIAN_POINT('Ctrl Pts',(1.16767555244495,-1.,-3.95351219510062));
#58363=CARTESIAN_POINT('Ctrl Pts',(1.16767555244495,1.,-3.95351219510062));
#58364=CARTESIAN_POINT('Ctrl Pts',(1.16262637999261,-1.,-3.9476147478092));
#58365=CARTESIAN_POINT('Ctrl Pts',(1.16262637999261,1.,-3.9476147478092));
#58366=CARTESIAN_POINT('Ctrl Pts',(1.1576101834106,-1.,-3.94170046685542));
#58367=CARTESIAN_POINT('Ctrl Pts',(1.1576101834106,1.,-3.94170046685542));
#58368=CARTESIAN_POINT('Ctrl Pts',(1.1526272271639,-1.,-3.9357691705651));
#58369=CARTESIAN_POINT('Ctrl Pts',(1.1526272271639,1.,-3.9357691705651));
#58370=CARTESIAN_POINT('Ctrl Pts',(1.14767779451147,-1.,-3.92982073294334));
#58371=CARTESIAN_POINT('Ctrl Pts',(1.14767779451147,1.,-3.92982073294334));
#58372=CARTESIAN_POINT('Ctrl Pts',(1.14276220561575,-1.,-3.92385513133937));
#58373=CARTESIAN_POINT('Ctrl Pts',(1.14276220561575,1.,-3.92385513133937));
#58374=CARTESIAN_POINT('Ctrl Pts',(1.13788084225511,-1.,-3.91787251936688));
#58375=CARTESIAN_POINT('Ctrl Pts',(1.13788084225511,1.,-3.91787251936688));
#58376=CARTESIAN_POINT('Ctrl Pts',(1.13303414693849,-1.,-3.91187321145495));
#58377=CARTESIAN_POINT('Ctrl Pts',(1.13303414693849,1.,-3.91187321145495));
#58378=CARTESIAN_POINT('Ctrl Pts',(1.12822258281518,-1.,-3.90585753318622));
#58379=CARTESIAN_POINT('Ctrl Pts',(1.12822258281518,1.,-3.90585753318622));
#58380=CARTESIAN_POINT('Ctrl Pts',(1.12344660099029,-1.,-3.89982569749978));
#58381=CARTESIAN_POINT('Ctrl Pts',(1.12344660099029,1.,-3.89982569749978));
#58382=CARTESIAN_POINT('Ctrl Pts',(1.11870660794609,-1.,-3.89377768340362));
#58383=CARTESIAN_POINT('Ctrl Pts',(1.11870660794609,1.,-3.89377768340362));
#58384=CARTESIAN_POINT('Ctrl Pts',(1.11400292434447,-1.,-3.88771308285229));
#58385=CARTESIAN_POINT('Ctrl Pts',(1.11400292434447,1.,-3.88771308285229));
#58386=CARTESIAN_POINT('Ctrl Pts',(1.10933577224029,-1.,-3.88163105531791));
#58387=CARTESIAN_POINT('Ctrl Pts',(1.10933577224029,1.,-3.88163105531791));
#58388=CARTESIAN_POINT('Ctrl Pts',(1.10470536603303,-1.,-3.87553067187566));
#58389=CARTESIAN_POINT('Ctrl Pts',(1.10470536603303,1.,-3.87553067187566));
#58390=CARTESIAN_POINT('Ctrl Pts',(1.10011198761202,-1.,-3.86941120134872));
#58391=CARTESIAN_POINT('Ctrl Pts',(1.10011198761202,1.,-3.86941120134872));
#58392=CARTESIAN_POINT('Ctrl Pts',(1.09555606505012,-1.,-3.86327241021242));
#58393=CARTESIAN_POINT('Ctrl Pts',(1.09555606505012,1.,-3.86327241021242));
#58394=CARTESIAN_POINT('Ctrl Pts',(1.09103825516288,-1.,-3.85711487933911));
#58395=CARTESIAN_POINT('Ctrl Pts',(1.09103825516288,1.,-3.85711487933911));
#58396=CARTESIAN_POINT('Ctrl Pts',(1.08655950846377,-1.,-3.85094025222691));
#58397=CARTESIAN_POINT('Ctrl Pts',(1.08655950846377,1.,-3.85094025222691));
#58398=CARTESIAN_POINT('Ctrl Pts',(1.08212087917986,-1.,-3.84475048030615));
#58399=CARTESIAN_POINT('Ctrl Pts',(1.08212087917986,1.,-3.84475048030615));
#58400=CARTESIAN_POINT('Ctrl Pts',(1.07772335353856,-1.,-3.83854714117486));
#58401=CARTESIAN_POINT('Ctrl Pts',(1.07772335353856,1.,-3.83854714117486));
#58402=CARTESIAN_POINT('Ctrl Pts',(1.0733676663346,-1.,-3.83233071195145));
#58403=CARTESIAN_POINT('Ctrl Pts',(1.0733676663346,1.,-3.83233071195145));
#58404=CARTESIAN_POINT('Ctrl Pts',(1.0690541318036,-1.,-3.82609989967278));
#58405=CARTESIAN_POINT('Ctrl Pts',(1.0690541318036,1.,-3.82609989967278));
#58406=CARTESIAN_POINT('Ctrl Pts',(1.06478244038931,-1.,-3.81985083953012));
#58407=CARTESIAN_POINT('Ctrl Pts',(1.06478244038931,1.,-3.81985083953012));
#58408=CARTESIAN_POINT('Ctrl Pts',(1.06055206187298,-1.,-3.81357866117485));
#58409=CARTESIAN_POINT('Ctrl Pts',(1.06055206187298,1.,-3.81357866117485));
#58410=CARTESIAN_POINT('Ctrl Pts',(1.05636266918643,-1.,-3.80727913637784));
#58411=CARTESIAN_POINT('Ctrl Pts',(1.05636266918643,1.,-3.80727913637784));
#58412=CARTESIAN_POINT('Ctrl Pts',(1.05221457990015,-1.,-3.80095039790678));
#58413=CARTESIAN_POINT('Ctrl Pts',(1.05221457990015,1.,-3.80095039790678));
#58414=CARTESIAN_POINT('Ctrl Pts',(1.04810913267641,-1.,-3.79459440308793));
#58415=CARTESIAN_POINT('Ctrl Pts',(1.04810913267641,1.,-3.79459440308793));
#58416=CARTESIAN_POINT('Ctrl Pts',(1.04404924374426,-1.,-3.78821910787195));
#58417=CARTESIAN_POINT('Ctrl Pts',(1.04404924374426,1.,-3.78821910787195));
#58418=CARTESIAN_POINT('Ctrl Pts',(1.04003862055804,-1.,-3.78183535008192));
#58419=CARTESIAN_POINT('Ctrl Pts',(1.04003862055804,1.,-3.78183535008192));
#58420=CARTESIAN_POINT('Ctrl Pts',(1.03608074678013,-1.,-3.77545283140445));
#58421=CARTESIAN_POINT('Ctrl Pts',(1.03608074678013,1.,-3.77545283140445));
#58422=CARTESIAN_POINT('Ctrl Pts',(1.0321778660492,-1.,-3.76907609832522));
#58423=CARTESIAN_POINT('Ctrl Pts',(1.0321778660492,1.,-3.76907609832522));
#58424=CARTESIAN_POINT('Ctrl Pts',(1.02833014458181,-1.,-3.76270122291232));
#58425=CARTESIAN_POINT('Ctrl Pts',(1.02833014458181,1.,-3.76270122291232));
#58426=CARTESIAN_POINT('Ctrl Pts',(1.0245342944466,-1.,-3.75631037456194));
#58427=CARTESIAN_POINT('Ctrl Pts',(1.0245342944466,1.,-3.75631037456194));
#58428=CARTESIAN_POINT('Ctrl Pts',(1.02078510487428,-1.,-3.74987777155834));
#58429=CARTESIAN_POINT('Ctrl Pts',(1.02078510487428,1.,-3.74987777155834));
#58430=CARTESIAN_POINT('Ctrl Pts',(1.01707794311079,-1.,-3.74337942504959));
#58431=CARTESIAN_POINT('Ctrl Pts',(1.01707794311079,1.,-3.74337942504959));
#58432=CARTESIAN_POINT('Ctrl Pts',(1.01341114319903,-1.,-3.73680245055734));
#58433=CARTESIAN_POINT('Ctrl Pts',(1.01341114319903,1.,-3.73680245055734));
#58434=CARTESIAN_POINT('Ctrl Pts',(1.00978798539496,-1.,-3.73015276704426));
#58435=CARTESIAN_POINT('Ctrl Pts',(1.00978798539496,1.,-3.73015276704426));
#58436=CARTESIAN_POINT('Ctrl Pts',(1.0062200073571,-1.,-3.72346803750596));
#58437=CARTESIAN_POINT('Ctrl Pts',(1.0062200073571,1.,-3.72346803750596));
#58438=CARTESIAN_POINT('Ctrl Pts',(1.00272423396822,-1.,-3.71680667125119));
#58439=CARTESIAN_POINT('Ctrl Pts',(1.00272423396822,1.,-3.71680667125119));
#58440=CARTESIAN_POINT('Ctrl Pts',(0.99931726075653,-1.,-3.71022439713938));
#58441=CARTESIAN_POINT('Ctrl Pts',(0.99931726075653,1.,-3.71022439713938));
#58442=CARTESIAN_POINT('Ctrl Pts',(0.996009819772518,-1.,-3.70375282282138));
#58443=CARTESIAN_POINT('Ctrl Pts',(0.996009819772518,1.,-3.70375282282138));
#58444=CARTESIAN_POINT('Ctrl Pts',(0.99280221833201,-1.,-3.69738123415662));
#58445=CARTESIAN_POINT('Ctrl Pts',(0.99280221833201,1.,-3.69738123415662));
#58446=CARTESIAN_POINT('Ctrl Pts',(0.989676715398558,-1.,-3.69102682138847));
#58447=CARTESIAN_POINT('Ctrl Pts',(0.989676715398558,1.,-3.69102682138847));
#58448=CARTESIAN_POINT('Ctrl Pts',(0.986602639863837,-1.,-3.68455317926068));
#58449=CARTESIAN_POINT('Ctrl Pts',(0.986602639863837,1.,-3.68455317926068));
#58450=CARTESIAN_POINT('Ctrl Pts',(0.983550791470419,-1.,-3.67782408841715));
#58451=CARTESIAN_POINT('Ctrl Pts',(0.983550791470419,1.,-3.67782408841715));
#58452=CARTESIAN_POINT('Ctrl Pts',(0.980505922458267,-1.,-3.67074983340361));
#58453=CARTESIAN_POINT('Ctrl Pts',(0.980505922458267,1.,-3.67074983340361));
#58454=CARTESIAN_POINT('Ctrl Pts',(0.977478312751618,-1.,-3.66333049637475));
#58455=CARTESIAN_POINT('Ctrl Pts',(0.977478312751618,1.,-3.66333049637475));
#58456=CARTESIAN_POINT('Ctrl Pts',(0.974519971354848,-1.,-3.65571576735126));
#58457=CARTESIAN_POINT('Ctrl Pts',(0.974519971354848,1.,-3.65571576735126));
#58458=CARTESIAN_POINT('Ctrl Pts',(0.971722122061341,-1.,-3.64819756447455));
#58459=CARTESIAN_POINT('Ctrl Pts',(0.971722122061341,1.,-3.64819756447455));
#58460=CARTESIAN_POINT('Ctrl Pts',(0.969195124675865,-1.,-3.64113946505766));
#58461=CARTESIAN_POINT('Ctrl Pts',(0.969195124675865,1.,-3.64113946505766));
#58462=CARTESIAN_POINT('Ctrl Pts',(0.967052554541385,-1.,-3.63492122081143));
#58463=CARTESIAN_POINT('Ctrl Pts',(0.967052554541385,1.,-3.63492122081143));
#58464=CARTESIAN_POINT('Ctrl Pts',(0.965395153165293,-1.,-3.62988252139846));
#58465=CARTESIAN_POINT('Ctrl Pts',(0.965395153165293,1.,-3.62988252139846));
#58466=CARTESIAN_POINT('Ctrl Pts',(0.964291001273287,-1.,-3.62625391254797));
#58467=CARTESIAN_POINT('Ctrl Pts',(0.964291001273287,1.,-3.62625391254797));
#58468=CARTESIAN_POINT('Ctrl Pts',(0.963875774530619,-1.,-3.6245656860652));
#58469=CARTESIAN_POINT('Ctrl Pts',(0.963875774530619,1.,-3.6245656860652));
#58470=CARTESIAN_POINT('Ctrl Pts',(0.963832486395051,-1.,-3.62399933639915));
#58471=CARTESIAN_POINT('Ctrl Pts',(0.963832486395051,1.,-3.62399933639915));
#58472=CARTESIAN_POINT('Ctrl Pts',(0.963922720982193,-1.,-3.62393257642052));
#58473=CARTESIAN_POINT('Ctrl Pts',(0.963922720982193,1.,-3.62393257642052));
#58474=CARTESIAN_POINT('Ctrl Pts',(0.963997613369571,-1.,-3.62397690409552));
#58475=CARTESIAN_POINT('Ctrl Pts',(0.963997613369571,1.,-3.62397690409552));
#58476=CARTESIAN_POINT('',(1.22531898815164,1.,-4.01728681790024));
#58477=CARTESIAN_POINT('Ctrl Pts',(1.22531898815164,1.,-4.01728681790024));
#58478=CARTESIAN_POINT('Ctrl Pts',(1.22423716681447,1.,-4.0161454457032));
#58479=CARTESIAN_POINT('Ctrl Pts',(1.22207656456199,1.,-4.01386104434674));
#58480=CARTESIAN_POINT('Ctrl Pts',(1.21884478244983,1.,-4.01042947142681));
#58481=CARTESIAN_POINT('Ctrl Pts',(1.21455398918813,1.,-4.00584409524937));
#58482=CARTESIAN_POINT('Ctrl Pts',(1.20922097030107,1.,-4.00009577952534));
#58483=CARTESIAN_POINT('Ctrl Pts',(1.2039185237544,1.,-3.99433084800649));
#58484=CARTESIAN_POINT('Ctrl Pts',(1.19864679609596,1.,-3.98854928957287));
#58485=CARTESIAN_POINT('Ctrl Pts',(1.19340598349307,1.,-3.98275111052015));
#58486=CARTESIAN_POINT('Ctrl Pts',(1.18819633715285,1.,-3.97693634766926));
#58487=CARTESIAN_POINT('Ctrl Pts',(1.18301815039596,1.,-3.9711050516465));
#58488=CARTESIAN_POINT('Ctrl Pts',(1.17787174135445,1.,-3.96525726357682));
#58489=CARTESIAN_POINT('Ctrl Pts',(1.17275743590327,1.,-3.95939299213164));
#58490=CARTESIAN_POINT('Ctrl Pts',(1.16767555244495,1.,-3.95351219510062));
#58491=CARTESIAN_POINT('Ctrl Pts',(1.16262637999261,1.,-3.9476147478092));
#58492=CARTESIAN_POINT('Ctrl Pts',(1.1576101834106,1.,-3.94170046685542));
#58493=CARTESIAN_POINT('Ctrl Pts',(1.1526272271639,1.,-3.9357691705651));
#58494=CARTESIAN_POINT('Ctrl Pts',(1.14767779451147,1.,-3.92982073294334));
#58495=CARTESIAN_POINT('Ctrl Pts',(1.14276220561575,1.,-3.92385513133937));
#58496=CARTESIAN_POINT('Ctrl Pts',(1.13788084225511,1.,-3.91787251936688));
#58497=CARTESIAN_POINT('Ctrl Pts',(1.13303414693849,1.,-3.91187321145495));
#58498=CARTESIAN_POINT('Ctrl Pts',(1.12822258281518,1.,-3.90585753318622));
#58499=CARTESIAN_POINT('Ctrl Pts',(1.12344660099029,1.,-3.89982569749978));
#58500=CARTESIAN_POINT('Ctrl Pts',(1.11870660794609,1.,-3.89377768340362));
#58501=CARTESIAN_POINT('Ctrl Pts',(1.11400292434447,1.,-3.88771308285229));
#58502=CARTESIAN_POINT('Ctrl Pts',(1.10933577224029,1.,-3.88163105531791));
#58503=CARTESIAN_POINT('Ctrl Pts',(1.10470536603303,1.,-3.87553067187566));
#58504=CARTESIAN_POINT('Ctrl Pts',(1.10011198761202,1.,-3.86941120134872));
#58505=CARTESIAN_POINT('Ctrl Pts',(1.09555606505012,1.,-3.86327241021242));
#58506=CARTESIAN_POINT('Ctrl Pts',(1.09103825516288,1.,-3.85711487933911));
#58507=CARTESIAN_POINT('Ctrl Pts',(1.08655950846377,1.,-3.85094025222691));
#58508=CARTESIAN_POINT('Ctrl Pts',(1.08212087917986,1.,-3.84475048030615));
#58509=CARTESIAN_POINT('Ctrl Pts',(1.07772335353856,1.,-3.83854714117486));
#58510=CARTESIAN_POINT('Ctrl Pts',(1.0733676663346,1.,-3.83233071195145));
#58511=CARTESIAN_POINT('Ctrl Pts',(1.0690541318036,1.,-3.82609989967278));
#58512=CARTESIAN_POINT('Ctrl Pts',(1.06478244038931,1.,-3.81985083953012));
#58513=CARTESIAN_POINT('Ctrl Pts',(1.06055206187298,1.,-3.81357866117485));
#58514=CARTESIAN_POINT('Ctrl Pts',(1.05636266918643,1.,-3.80727913637784));
#58515=CARTESIAN_POINT('Ctrl Pts',(1.05221457990015,1.,-3.80095039790678));
#58516=CARTESIAN_POINT('Ctrl Pts',(1.04810913267641,1.,-3.79459440308793));
#58517=CARTESIAN_POINT('Ctrl Pts',(1.04404924374426,1.,-3.78821910787195));
#58518=CARTESIAN_POINT('Ctrl Pts',(1.04003862055804,1.,-3.78183535008192));
#58519=CARTESIAN_POINT('Ctrl Pts',(1.03608074678013,1.,-3.77545283140445));
#58520=CARTESIAN_POINT('Ctrl Pts',(1.0321778660492,1.,-3.76907609832522));
#58521=CARTESIAN_POINT('Ctrl Pts',(1.02833014458181,1.,-3.76270122291232));
#58522=CARTESIAN_POINT('Ctrl Pts',(1.0245342944466,1.,-3.75631037456194));
#58523=CARTESIAN_POINT('Ctrl Pts',(1.02078510487428,1.,-3.74987777155834));
#58524=CARTESIAN_POINT('Ctrl Pts',(1.01707794311079,1.,-3.74337942504959));
#58525=CARTESIAN_POINT('Ctrl Pts',(1.01341114319903,1.,-3.73680245055734));
#58526=CARTESIAN_POINT('Ctrl Pts',(1.00978798539496,1.,-3.73015276704426));
#58527=CARTESIAN_POINT('Ctrl Pts',(1.0062200073571,1.,-3.72346803750596));
#58528=CARTESIAN_POINT('Ctrl Pts',(1.00272423396822,1.,-3.71680667125119));
#58529=CARTESIAN_POINT('Ctrl Pts',(0.99931726075653,1.,-3.71022439713938));
#58530=CARTESIAN_POINT('Ctrl Pts',(0.996009819772518,1.,-3.70375282282138));
#58531=CARTESIAN_POINT('Ctrl Pts',(0.99280221833201,1.,-3.69738123415662));
#58532=CARTESIAN_POINT('Ctrl Pts',(0.989676715398558,1.,-3.69102682138847));
#58533=CARTESIAN_POINT('Ctrl Pts',(0.986602639863837,1.,-3.68455317926068));
#58534=CARTESIAN_POINT('Ctrl Pts',(0.983550791470419,1.,-3.67782408841715));
#58535=CARTESIAN_POINT('Ctrl Pts',(0.980505922458267,1.,-3.67074983340361));
#58536=CARTESIAN_POINT('Ctrl Pts',(0.977478312751618,1.,-3.66333049637475));
#58537=CARTESIAN_POINT('Ctrl Pts',(0.974519971354848,1.,-3.65571576735126));
#58538=CARTESIAN_POINT('Ctrl Pts',(0.971722122061341,1.,-3.64819756447455));
#58539=CARTESIAN_POINT('Ctrl Pts',(0.969195124675865,1.,-3.64113946505766));
#58540=CARTESIAN_POINT('Ctrl Pts',(0.967052554541385,1.,-3.63492122081143));
#58541=CARTESIAN_POINT('Ctrl Pts',(0.965395153165293,1.,-3.62988252139846));
#58542=CARTESIAN_POINT('Ctrl Pts',(0.964373850166457,1.,-3.62652618145335));
#58543=CARTESIAN_POINT('Ctrl Pts',(0.963957782642843,1.,-3.62489305727662));
#58544=CARTESIAN_POINT('Ctrl Pts',(0.963861297423241,1.,-3.62424461507588));
#58545=CARTESIAN_POINT('Ctrl Pts',(0.963880158555582,1.,-3.6240482887845));
#58546=CARTESIAN_POINT('Ctrl Pts',(0.963899035117249,1.,-3.62400312501246));
#58547=CARTESIAN_POINT('',(1.22531898815164,0.,-4.01728681790024));
#58548=CARTESIAN_POINT('Ctrl Pts',(1.35022972712301,-1.,-3.49848248301936));
#58549=CARTESIAN_POINT('Ctrl Pts',(1.35022972712301,1.,-3.49848248301936));
#58550=CARTESIAN_POINT('Ctrl Pts',(1.35026426118402,-1.,-3.4984026005375));
#58551=CARTESIAN_POINT('Ctrl Pts',(1.35026426118402,1.,-3.4984026005375));
#58552=CARTESIAN_POINT('Ctrl Pts',(1.35037650303019,-1.,-3.49840357193736));
#58553=CARTESIAN_POINT('Ctrl Pts',(1.35037650303019,1.,-3.49840357193736));
#58554=CARTESIAN_POINT('Ctrl Pts',(1.35067437417483,-1.,-3.49888720257132));
#58555=CARTESIAN_POINT('Ctrl Pts',(1.35067437417483,1.,-3.49888720257132));
#58556=CARTESIAN_POINT('Ctrl Pts',(1.3513307633124,-1.,-3.5004970706414));
#58557=CARTESIAN_POINT('Ctrl Pts',(1.3513307633124,1.,-3.5004970706414));
#58558=CARTESIAN_POINT('Ctrl Pts',(1.35257032843486,-1.,-3.50408168106261));
#58559=CARTESIAN_POINT('Ctrl Pts',(1.35257032843486,1.,-3.50408168106261));
#58560=CARTESIAN_POINT('Ctrl Pts',(1.35419113575956,-1.,-3.50913227059999));
#58561=CARTESIAN_POINT('Ctrl Pts',(1.35419113575956,1.,-3.50913227059999));
#58562=CARTESIAN_POINT('Ctrl Pts',(1.35611275237152,-1.,-3.51542230699556));
#58563=CARTESIAN_POINT('Ctrl Pts',(1.35611275237152,1.,-3.51542230699556));
#58564=CARTESIAN_POINT('Ctrl Pts',(1.35821701528836,-1.,-3.52261776116748));
#58565=CARTESIAN_POINT('Ctrl Pts',(1.35821701528836,1.,-3.52261776116748));
#58566=CARTESIAN_POINT('Ctrl Pts',(1.36037259643734,-1.,-3.530344649616));
#58567=CARTESIAN_POINT('Ctrl Pts',(1.36037259643734,1.,-3.530344649616));
#58568=CARTESIAN_POINT('Ctrl Pts',(1.36245507339307,-1.,-3.53824396424961));
#58569=CARTESIAN_POINT('Ctrl Pts',(1.36245507339307,1.,-3.53824396424961));
#58570=CARTESIAN_POINT('Ctrl Pts',(1.36436666257597,-1.,-3.54602591832973));
#58571=CARTESIAN_POINT('Ctrl Pts',(1.36436666257597,1.,-3.54602591832973));
#58572=CARTESIAN_POINT('Ctrl Pts',(1.3660614545677,-1.,-3.55353883995949));
#58573=CARTESIAN_POINT('Ctrl Pts',(1.3660614545677,1.,-3.55353883995949));
#58574=CARTESIAN_POINT('Ctrl Pts',(1.36754771771233,-1.,-3.56077662028649));
#58575=CARTESIAN_POINT('Ctrl Pts',(1.36754771771233,1.,-3.56077662028649));
#58576=CARTESIAN_POINT('Ctrl Pts',(1.36886584973389,-1.,-3.5678208030466));
#58577=CARTESIAN_POINT('Ctrl Pts',(1.36886584973389,1.,-3.5678208030466));
#58578=CARTESIAN_POINT('Ctrl Pts',(1.37007229485659,-1.,-3.57479875549486));
#58579=CARTESIAN_POINT('Ctrl Pts',(1.37007229485659,1.,-3.57479875549486));
#58580=CARTESIAN_POINT('Ctrl Pts',(1.37122241663062,-1.,-3.58183885982715));
#58581=CARTESIAN_POINT('Ctrl Pts',(1.37122241663062,1.,-3.58183885982715));
#58582=CARTESIAN_POINT('Ctrl Pts',(1.37235053660976,-1.,-3.58901853846365));
#58583=CARTESIAN_POINT('Ctrl Pts',(1.37235053660976,1.,-3.58901853846365));
#58584=CARTESIAN_POINT('Ctrl Pts',(1.37346320103157,-1.,-3.59634627869048));
#58585=CARTESIAN_POINT('Ctrl Pts',(1.37346320103157,1.,-3.59634627869048));
#58586=CARTESIAN_POINT('Ctrl Pts',(1.37455051379623,-1.,-3.60379020123988));
#58587=CARTESIAN_POINT('Ctrl Pts',(1.37455051379623,1.,-3.60379020123988));
#58588=CARTESIAN_POINT('Ctrl Pts',(1.37559314436634,-1.,-3.61129546591064));
#58589=CARTESIAN_POINT('Ctrl Pts',(1.37559314436634,1.,-3.61129546591064));
#58590=CARTESIAN_POINT('Ctrl Pts',(1.37657053403107,-1.,-3.61880481160421));
#58591=CARTESIAN_POINT('Ctrl Pts',(1.37657053403107,1.,-3.61880481160421));
#58592=CARTESIAN_POINT('Ctrl Pts',(1.37746987919881,-1.,-3.62628098665145));
#58593=CARTESIAN_POINT('Ctrl Pts',(1.37746987919881,1.,-3.62628098665145));
#58594=CARTESIAN_POINT('Ctrl Pts',(1.37829035457339,-1.,-3.63371727442486));
#58595=CARTESIAN_POINT('Ctrl Pts',(1.37829035457339,1.,-3.63371727442486));
#58596=CARTESIAN_POINT('Ctrl Pts',(1.37903818567359,-1.,-3.64112507791141));
#58597=CARTESIAN_POINT('Ctrl Pts',(1.37903818567359,1.,-3.64112507791141));
#58598=CARTESIAN_POINT('Ctrl Pts',(1.37972372481603,-1.,-3.64852652756456));
#58599=CARTESIAN_POINT('Ctrl Pts',(1.37972372481603,1.,-3.64852652756456));
#58600=CARTESIAN_POINT('Ctrl Pts',(1.38035791051212,-1.,-3.6559455440439));
#58601=CARTESIAN_POINT('Ctrl Pts',(1.38035791051212,1.,-3.6559455440439));
#58602=CARTESIAN_POINT('Ctrl Pts',(1.38094856333552,-1.,-3.66339848520857));
#58603=CARTESIAN_POINT('Ctrl Pts',(1.38094856333552,1.,-3.66339848520857));
#58604=CARTESIAN_POINT('Ctrl Pts',(1.38149812653868,-1.,-3.67088843112262));
#58605=CARTESIAN_POINT('Ctrl Pts',(1.38149812653868,1.,-3.67088843112262));
#58606=CARTESIAN_POINT('Ctrl Pts',(1.3820057429062,-1.,-3.67841038482414));
#58607=CARTESIAN_POINT('Ctrl Pts',(1.3820057429062,1.,-3.67841038482414));
#58608=CARTESIAN_POINT('Ctrl Pts',(1.38246852827182,-1.,-3.68595444983838));
#58609=CARTESIAN_POINT('Ctrl Pts',(1.38246852827182,1.,-3.68595444983838));
#58610=CARTESIAN_POINT('Ctrl Pts',(1.3828831117165,-1.,-3.69350967899526));
#58611=CARTESIAN_POINT('Ctrl Pts',(1.3828831117165,1.,-3.69350967899526));
#58612=CARTESIAN_POINT('Ctrl Pts',(1.38324717612865,-1.,-3.701067921679));
#58613=CARTESIAN_POINT('Ctrl Pts',(1.38324717612865,1.,-3.701067921679));
#58614=CARTESIAN_POINT('Ctrl Pts',(1.38356065402124,-1.,-3.70862680753347));
#58615=CARTESIAN_POINT('Ctrl Pts',(1.38356065402124,1.,-3.70862680753347));
#58616=CARTESIAN_POINT('Ctrl Pts',(1.38382489984586,-1.,-3.7161876605181));
#58617=CARTESIAN_POINT('Ctrl Pts',(1.38382489984586,1.,-3.7161876605181));
#58618=CARTESIAN_POINT('Ctrl Pts',(1.3840421342895,-1.,-3.72375409358803));
#58619=CARTESIAN_POINT('Ctrl Pts',(1.3840421342895,1.,-3.72375409358803));
#58620=CARTESIAN_POINT('Ctrl Pts',(1.38421479111531,-1.,-3.73133035859282));
#58621=CARTESIAN_POINT('Ctrl Pts',(1.38421479111531,1.,-3.73133035859282));
#58622=CARTESIAN_POINT('Ctrl Pts',(1.38434489156458,-1.,-3.73891976418104));
#58623=CARTESIAN_POINT('Ctrl Pts',(1.38434489156458,1.,-3.73891976418104));
#58624=CARTESIAN_POINT('Ctrl Pts',(1.38443344984394,-1.,-3.74652317167876));
#58625=CARTESIAN_POINT('Ctrl Pts',(1.38443344984394,1.,-3.74652317167876));
#58626=CARTESIAN_POINT('Ctrl Pts',(1.38448077997163,-1.,-3.7541397631875));
#58627=CARTESIAN_POINT('Ctrl Pts',(1.38448077997163,1.,-3.7541397631875));
#58628=CARTESIAN_POINT('Ctrl Pts',(1.3844867525335,-1.,-3.76176768271367));
#58629=CARTESIAN_POINT('Ctrl Pts',(1.3844867525335,1.,-3.76176768271367));
#58630=CARTESIAN_POINT('Ctrl Pts',(1.38445107339518,-1.,-3.76940473185779));
#58631=CARTESIAN_POINT('Ctrl Pts',(1.38445107339518,1.,-3.76940473185779));
#58632=CARTESIAN_POINT('Ctrl Pts',(1.38437354551428,-1.,-3.77704902230418));
#58633=CARTESIAN_POINT('Ctrl Pts',(1.38437354551428,1.,-3.77704902230418));
#58634=CARTESIAN_POINT('Ctrl Pts',(1.38425435883756,-1.,-3.78469969805082));
#58635=CARTESIAN_POINT('Ctrl Pts',(1.38425435883756,1.,-3.78469969805082));
#58636=CARTESIAN_POINT('Ctrl Pts',(1.38409399694566,-1.,-3.79235669640841));
#58637=CARTESIAN_POINT('Ctrl Pts',(1.38409399694566,1.,-3.79235669640841));
#58638=CARTESIAN_POINT('Ctrl Pts',(1.38389311766682,-1.,-3.80002044322111));
#58639=CARTESIAN_POINT('Ctrl Pts',(1.38389311766682,1.,-3.80002044322111));
#58640=CARTESIAN_POINT('Ctrl Pts',(1.3836524404622,-1.,-3.80769156398411));
#58641=CARTESIAN_POINT('Ctrl Pts',(1.3836524404622,1.,-3.80769156398411));
#58642=CARTESIAN_POINT('Ctrl Pts',(1.38337263902782,-1.,-3.81537060817811));
#58643=CARTESIAN_POINT('Ctrl Pts',(1.38337263902782,1.,-3.81537060817811));
#58644=CARTESIAN_POINT('Ctrl Pts',(1.38305421262763,-1.,-3.82305771743829));
#58645=CARTESIAN_POINT('Ctrl Pts',(1.38305421262763,1.,-3.82305771743829));
#58646=CARTESIAN_POINT('Ctrl Pts',(1.38269750245138,-1.,-3.8307526698229));
#58647=CARTESIAN_POINT('Ctrl Pts',(1.38269750245138,1.,-3.8307526698229));
#58648=CARTESIAN_POINT('Ctrl Pts',(1.38230274828821,-1.,-3.83845502790746));
#58649=CARTESIAN_POINT('Ctrl Pts',(1.38230274828821,1.,-3.83845502790746));
#58650=CARTESIAN_POINT('Ctrl Pts',(1.38187013346109,-1.,-3.84616425605764));
#58651=CARTESIAN_POINT('Ctrl Pts',(1.38187013346109,1.,-3.84616425605764));
#58652=CARTESIAN_POINT('Ctrl Pts',(1.38139983115049,-1.,-3.85387983979481));
#58653=CARTESIAN_POINT('Ctrl Pts',(1.38139983115049,1.,-3.85387983979481));
#58654=CARTESIAN_POINT('Ctrl Pts',(1.38089205992989,-1.,-3.86160143043959));
#58655=CARTESIAN_POINT('Ctrl Pts',(1.38089205992989,1.,-3.86160143043959));
#58656=CARTESIAN_POINT('Ctrl Pts',(1.38034709213014,-1.,-3.86932885813068));
#58657=CARTESIAN_POINT('Ctrl Pts',(1.38034709213014,1.,-3.86932885813068));
#58658=CARTESIAN_POINT('Ctrl Pts',(1.37976523097073,-1.,-3.87706205830532));
#58659=CARTESIAN_POINT('Ctrl Pts',(1.37976523097073,1.,-3.87706205830532));
#58660=CARTESIAN_POINT('Ctrl Pts',(1.37914679719383,-1.,-3.88480102249278));
#58661=CARTESIAN_POINT('Ctrl Pts',(1.37914679719383,1.,-3.88480102249278));
#58662=CARTESIAN_POINT('Ctrl Pts',(1.3784921128802,-1.,-3.89254574338496));
#58663=CARTESIAN_POINT('Ctrl Pts',(1.3784921128802,1.,-3.89254574338496));
#58664=CARTESIAN_POINT('Ctrl Pts',(1.37780148512792,-1.,-3.90029615196727));
#58665=CARTESIAN_POINT('Ctrl Pts',(1.37780148512792,1.,-3.90029615196727));
#58666=CARTESIAN_POINT('Ctrl Pts',(1.3770751963402,-1.,-3.90805209523486));
#58667=CARTESIAN_POINT('Ctrl Pts',(1.3770751963402,1.,-3.90805209523486));
#58668=CARTESIAN_POINT('Ctrl Pts',(1.37631350505797,-1.,-3.91581337462644));
#58669=CARTESIAN_POINT('Ctrl Pts',(1.37631350505797,1.,-3.91581337462644));
#58670=CARTESIAN_POINT('Ctrl Pts',(1.37551664448242,-1.,-3.92357976987672));
#58671=CARTESIAN_POINT('Ctrl Pts',(1.37551664448242,1.,-3.92357976987672));
#58672=CARTESIAN_POINT('Ctrl Pts',(1.37468482215751,-1.,-3.93135106761844));
#58673=CARTESIAN_POINT('Ctrl Pts',(1.37468482215751,1.,-3.93135106761844));
#58674=CARTESIAN_POINT('Ctrl Pts',(1.37381821967165,-1.,-3.93912709040818));
#58675=CARTESIAN_POINT('Ctrl Pts',(1.37381821967165,1.,-3.93912709040818));
#58676=CARTESIAN_POINT('Ctrl Pts',(1.37291699202807,-1.,-3.94690771785133));
#58677=CARTESIAN_POINT('Ctrl Pts',(1.37291699202807,1.,-3.94690771785133));
#58678=CARTESIAN_POINT('Ctrl Pts',(1.37198126432386,-1.,-3.95469287280914));
#58679=CARTESIAN_POINT('Ctrl Pts',(1.37198126432386,1.,-3.95469287280914));
#58680=CARTESIAN_POINT('Ctrl Pts',(1.3712051561502,-1.,-3.96092458506535));
#58681=CARTESIAN_POINT('Ctrl Pts',(1.3712051561502,1.,-3.96092458506535));
#58682=CARTESIAN_POINT('Ctrl Pts',(1.37060761745635,-1.,-3.96560037974645));
#58683=CARTESIAN_POINT('Ctrl Pts',(1.37060761745635,1.,-3.96560037974645));
#58684=CARTESIAN_POINT('Ctrl Pts',(1.37020239094614,-1.,-3.9687184694131));
#58685=CARTESIAN_POINT('Ctrl Pts',(1.37020239094614,1.,-3.9687184694131));
#58686=CARTESIAN_POINT('Ctrl Pts',(1.36999806084572,-1.,-3.97027773754922));
#58687=CARTESIAN_POINT('Ctrl Pts',(1.36999806084572,1.,-3.97027773754922));
#58688=CARTESIAN_POINT('',(1.35032489087101,1.,-3.4984457533445));
#58689=CARTESIAN_POINT('Ctrl Pts',(1.35032489087101,-1.,-3.4984457533445));
#58690=CARTESIAN_POINT('Ctrl Pts',(1.35032489087101,-0.666666666666667,
-3.4984457533445));
#58691=CARTESIAN_POINT('Ctrl Pts',(1.35032489087101,-0.333333333333333,
-3.4984457533445));
#58692=CARTESIAN_POINT('Ctrl Pts',(1.35032489087101,0.333333333333333,-3.4984457533445));
#58693=CARTESIAN_POINT('Ctrl Pts',(1.35032489087101,0.666666666666667,-3.4984457533445));
#58694=CARTESIAN_POINT('Ctrl Pts',(1.35032489087101,1.,-3.4984457533445));
#58695=CARTESIAN_POINT('',(1.36999806084572,1.,-3.97027773754922));
#58696=CARTESIAN_POINT('',(1.36999806084572,0.,-3.97027773754922));
#58697=CARTESIAN_POINT('Ctrl Pts',(1.35032489087101,1.,-3.49844575334451));
#58698=CARTESIAN_POINT('Ctrl Pts',(1.35036670892966,1.,-3.49847119623846));
#58699=CARTESIAN_POINT('Ctrl Pts',(1.35049736560527,1.,-3.49861894124827));
#58700=CARTESIAN_POINT('Ctrl Pts',(1.35080045218587,1.,-3.49920025459723));
#58701=CARTESIAN_POINT('Ctrl Pts',(1.35142377279517,1.,-3.50076603816491));
#58702=CARTESIAN_POINT('Ctrl Pts',(1.35257032843486,1.,-3.50408168106261));
#58703=CARTESIAN_POINT('Ctrl Pts',(1.35419113575956,1.,-3.50913227059999));
#58704=CARTESIAN_POINT('Ctrl Pts',(1.35611275237152,1.,-3.51542230699556));
#58705=CARTESIAN_POINT('Ctrl Pts',(1.35821701528836,1.,-3.52261776116748));
#58706=CARTESIAN_POINT('Ctrl Pts',(1.36037259643734,1.,-3.530344649616));
#58707=CARTESIAN_POINT('Ctrl Pts',(1.36245507339307,1.,-3.53824396424961));
#58708=CARTESIAN_POINT('Ctrl Pts',(1.36436666257597,1.,-3.54602591832973));
#58709=CARTESIAN_POINT('Ctrl Pts',(1.3660614545677,1.,-3.55353883995949));
#58710=CARTESIAN_POINT('Ctrl Pts',(1.36754771771233,1.,-3.56077662028649));
#58711=CARTESIAN_POINT('Ctrl Pts',(1.36886584973389,1.,-3.5678208030466));
#58712=CARTESIAN_POINT('Ctrl Pts',(1.37007229485659,1.,-3.57479875549486));
#58713=CARTESIAN_POINT('Ctrl Pts',(1.37122241663062,1.,-3.58183885982715));
#58714=CARTESIAN_POINT('Ctrl Pts',(1.37235053660976,1.,-3.58901853846365));
#58715=CARTESIAN_POINT('Ctrl Pts',(1.37346320103157,1.,-3.59634627869048));
#58716=CARTESIAN_POINT('Ctrl Pts',(1.37455051379623,1.,-3.60379020123988));
#58717=CARTESIAN_POINT('Ctrl Pts',(1.37559314436634,1.,-3.61129546591064));
#58718=CARTESIAN_POINT('Ctrl Pts',(1.37657053403107,1.,-3.61880481160421));
#58719=CARTESIAN_POINT('Ctrl Pts',(1.37746987919881,1.,-3.62628098665145));
#58720=CARTESIAN_POINT('Ctrl Pts',(1.37829035457339,1.,-3.63371727442486));
#58721=CARTESIAN_POINT('Ctrl Pts',(1.37903818567359,1.,-3.64112507791141));
#58722=CARTESIAN_POINT('Ctrl Pts',(1.37972372481603,1.,-3.64852652756456));
#58723=CARTESIAN_POINT('Ctrl Pts',(1.38035791051212,1.,-3.6559455440439));
#58724=CARTESIAN_POINT('Ctrl Pts',(1.38094856333552,1.,-3.66339848520857));
#58725=CARTESIAN_POINT('Ctrl Pts',(1.38149812653868,1.,-3.67088843112262));
#58726=CARTESIAN_POINT('Ctrl Pts',(1.3820057429062,1.,-3.67841038482414));
#58727=CARTESIAN_POINT('Ctrl Pts',(1.38246852827182,1.,-3.68595444983838));
#58728=CARTESIAN_POINT('Ctrl Pts',(1.3828831117165,1.,-3.69350967899526));
#58729=CARTESIAN_POINT('Ctrl Pts',(1.38324717612865,1.,-3.701067921679));
#58730=CARTESIAN_POINT('Ctrl Pts',(1.38356065402124,1.,-3.70862680753347));
#58731=CARTESIAN_POINT('Ctrl Pts',(1.38382489984586,1.,-3.7161876605181));
#58732=CARTESIAN_POINT('Ctrl Pts',(1.3840421342895,1.,-3.72375409358803));
#58733=CARTESIAN_POINT('Ctrl Pts',(1.38421479111531,1.,-3.73133035859282));
#58734=CARTESIAN_POINT('Ctrl Pts',(1.38434489156458,1.,-3.73891976418104));
#58735=CARTESIAN_POINT('Ctrl Pts',(1.38443344984394,1.,-3.74652317167876));
#58736=CARTESIAN_POINT('Ctrl Pts',(1.38448077997163,1.,-3.7541397631875));
#58737=CARTESIAN_POINT('Ctrl Pts',(1.3844867525335,1.,-3.76176768271367));
#58738=CARTESIAN_POINT('Ctrl Pts',(1.38445107339518,1.,-3.76940473185779));
#58739=CARTESIAN_POINT('Ctrl Pts',(1.38437354551428,1.,-3.77704902230418));
#58740=CARTESIAN_POINT('Ctrl Pts',(1.38425435883756,1.,-3.78469969805082));
#58741=CARTESIAN_POINT('Ctrl Pts',(1.38409399694566,1.,-3.79235669640841));
#58742=CARTESIAN_POINT('Ctrl Pts',(1.38389311766682,1.,-3.80002044322111));
#58743=CARTESIAN_POINT('Ctrl Pts',(1.3836524404622,1.,-3.80769156398411));
#58744=CARTESIAN_POINT('Ctrl Pts',(1.38337263902782,1.,-3.81537060817811));
#58745=CARTESIAN_POINT('Ctrl Pts',(1.38305421262763,1.,-3.82305771743829));
#58746=CARTESIAN_POINT('Ctrl Pts',(1.38269750245138,1.,-3.8307526698229));
#58747=CARTESIAN_POINT('Ctrl Pts',(1.38230274828821,1.,-3.83845502790746));
#58748=CARTESIAN_POINT('Ctrl Pts',(1.38187013346109,1.,-3.84616425605764));
#58749=CARTESIAN_POINT('Ctrl Pts',(1.38139983115049,1.,-3.85387983979481));
#58750=CARTESIAN_POINT('Ctrl Pts',(1.38089205992989,1.,-3.86160143043959));
#58751=CARTESIAN_POINT('Ctrl Pts',(1.38034709213014,1.,-3.86932885813068));
#58752=CARTESIAN_POINT('Ctrl Pts',(1.37976523097073,1.,-3.87706205830532));
#58753=CARTESIAN_POINT('Ctrl Pts',(1.37914679719383,1.,-3.88480102249278));
#58754=CARTESIAN_POINT('Ctrl Pts',(1.3784921128802,1.,-3.89254574338496));
#58755=CARTESIAN_POINT('Ctrl Pts',(1.37780148512792,1.,-3.90029615196727));
#58756=CARTESIAN_POINT('Ctrl Pts',(1.3770751963402,1.,-3.90805209523486));
#58757=CARTESIAN_POINT('Ctrl Pts',(1.37631350505797,1.,-3.91581337462644));
#58758=CARTESIAN_POINT('Ctrl Pts',(1.37551664448242,1.,-3.92357976987672));
#58759=CARTESIAN_POINT('Ctrl Pts',(1.37468482215751,1.,-3.93135106761844));
#58760=CARTESIAN_POINT('Ctrl Pts',(1.37381821967165,1.,-3.93912709040818));
#58761=CARTESIAN_POINT('Ctrl Pts',(1.37291699202807,1.,-3.94690771785133));
#58762=CARTESIAN_POINT('Ctrl Pts',(1.37198126432386,1.,-3.95469287280914));
#58763=CARTESIAN_POINT('Ctrl Pts',(1.3712051561502,1.,-3.96092458506535));
#58764=CARTESIAN_POINT('Ctrl Pts',(1.37060761745635,1.,-3.96560037974645));
#58765=CARTESIAN_POINT('Ctrl Pts',(1.37020239094614,1.,-3.9687184694131));
#58766=CARTESIAN_POINT('Ctrl Pts',(1.36999806084572,1.,-3.97027773754922));
#58767=CARTESIAN_POINT('Origin',(1.36999806084572,0.,-3.97027773754922));
#58768=CARTESIAN_POINT('',(1.22531898815164,1.,-4.01728681790024));
#58769=CARTESIAN_POINT('Origin',(0.,0.,0.));
#58770=CARTESIAN_POINT('',(1.51895082866166,1.,-3.42859860294378));
#58771=CARTESIAN_POINT('Origin',(0.,1.,0.));
#58772=CARTESIAN_POINT('Ctrl Pts',(1.51895082866166,1.,-3.42859860294378));
#58773=CARTESIAN_POINT('Ctrl Pts',(1.51895082866166,0.666666666666667,-3.42859860294378));
#58774=CARTESIAN_POINT('Ctrl Pts',(1.51895082866166,0.333333333333333,-3.42859860294378));
#58775=CARTESIAN_POINT('Ctrl Pts',(1.51895082866166,-0.333333333333333,
-3.42859860294378));
#58776=CARTESIAN_POINT('Ctrl Pts',(1.51895082866166,-0.666666666666667,
-3.42859860294378));
#58777=CARTESIAN_POINT('Ctrl Pts',(1.51895082866166,-1.,-3.42859860294378));
#58778=CARTESIAN_POINT('Ctrl Pts',(1.83867539237861,-1.,-3.77614523045147));
#58779=CARTESIAN_POINT('Ctrl Pts',(1.83867539237861,1.,-3.77614523045147));
#58780=CARTESIAN_POINT('Ctrl Pts',(1.83742834010821,-1.,-3.77518714458232));
#58781=CARTESIAN_POINT('Ctrl Pts',(1.83742834010821,1.,-3.77518714458232));
#58782=CARTESIAN_POINT('Ctrl Pts',(1.83493697935064,-1.,-3.77326886065484));
#58783=CARTESIAN_POINT('Ctrl Pts',(1.83493697935064,1.,-3.77326886065484));
#58784=CARTESIAN_POINT('Ctrl Pts',(1.83120816956515,-1.,-3.77038509819777));
#58785=CARTESIAN_POINT('Ctrl Pts',(1.83120816956515,1.,-3.77038509819777));
#58786=CARTESIAN_POINT('Ctrl Pts',(1.82625289221933,-1.,-3.76652740355856));
#58787=CARTESIAN_POINT('Ctrl Pts',(1.82625289221933,1.,-3.76652740355856));
#58788=CARTESIAN_POINT('Ctrl Pts',(1.82008629694924,-1.,-3.76168412709652));
#58789=CARTESIAN_POINT('Ctrl Pts',(1.82008629694924,1.,-3.76168412709652));
#58790=CARTESIAN_POINT('Ctrl Pts',(1.81394729834032,-1.,-3.75681965683995));
#58791=CARTESIAN_POINT('Ctrl Pts',(1.81394729834032,1.,-3.75681965683995));
#58792=CARTESIAN_POINT('Ctrl Pts',(1.80783603939662,-1.,-3.75193395888069));
#58793=CARTESIAN_POINT('Ctrl Pts',(1.80783603939662,1.,-3.75193395888069));
#58794=CARTESIAN_POINT('Ctrl Pts',(1.80175271485519,-1.,-3.74702700874954));
#58795=CARTESIAN_POINT('Ctrl Pts',(1.80175271485519,1.,-3.74702700874954));
#58796=CARTESIAN_POINT('Ctrl Pts',(1.79569757859041,-1.,-3.74209880351667));
#58797=CARTESIAN_POINT('Ctrl Pts',(1.79569757859041,1.,-3.74209880351667));
#58798=CARTESIAN_POINT('Ctrl Pts',(1.78967092823139,-1.,-3.73714934729962));
#58799=CARTESIAN_POINT('Ctrl Pts',(1.78967092823139,1.,-3.73714934729962));
#58800=CARTESIAN_POINT('Ctrl Pts',(1.78367308442682,-1.,-3.73217863095022));
#58801=CARTESIAN_POINT('Ctrl Pts',(1.78367308442682,1.,-3.73217863095022));
#58802=CARTESIAN_POINT('Ctrl Pts',(1.77770437039606,-1.,-3.72718661205504));
#58803=CARTESIAN_POINT('Ctrl Pts',(1.77770437039606,1.,-3.72718661205504));
#58804=CARTESIAN_POINT('Ctrl Pts',(1.77176509401846,-1.,-3.72217319911429));
#58805=CARTESIAN_POINT('Ctrl Pts',(1.77176509401846,1.,-3.72217319911429));
#58806=CARTESIAN_POINT('Ctrl Pts',(1.76585552124549,-1.,-3.71713822377676));
#58807=CARTESIAN_POINT('Ctrl Pts',(1.76585552124549,1.,-3.71713822377676));
#58808=CARTESIAN_POINT('Ctrl Pts',(1.75997588499021,-1.,-3.71208146346455));
#58809=CARTESIAN_POINT('Ctrl Pts',(1.75997588499021,1.,-3.71208146346455));
#58810=CARTESIAN_POINT('Ctrl Pts',(1.75412641804148,-1.,-3.70700269736876));
#58811=CARTESIAN_POINT('Ctrl Pts',(1.75412641804148,1.,-3.70700269736876));
#58812=CARTESIAN_POINT('Ctrl Pts',(1.74830738046092,-1.,-3.70190175673422));
#58813=CARTESIAN_POINT('Ctrl Pts',(1.74830738046092,1.,-3.70190175673422));
#58814=CARTESIAN_POINT('Ctrl Pts',(1.74251908492589,-1.,-3.6967785691046));
#58815=CARTESIAN_POINT('Ctrl Pts',(1.74251908492589,1.,-3.6967785691046));
#58816=CARTESIAN_POINT('Ctrl Pts',(1.73676193254493,-1.,-3.69163322647906));
#58817=CARTESIAN_POINT('Ctrl Pts',(1.73676193254493,1.,-3.69163322647906));
#58818=CARTESIAN_POINT('Ctrl Pts',(1.73103640956647,-1.,-3.68646597019188));
#58819=CARTESIAN_POINT('Ctrl Pts',(1.73103640956647,1.,-3.68646597019188));
#58820=CARTESIAN_POINT('Ctrl Pts',(1.72534302437003,-1.,-3.68127704936472));
#58821=CARTESIAN_POINT('Ctrl Pts',(1.72534302437003,1.,-3.68127704936472));
#58822=CARTESIAN_POINT('Ctrl Pts',(1.71968225581787,-1.,-3.67606660374665));
#58823=CARTESIAN_POINT('Ctrl Pts',(1.71968225581787,1.,-3.67606660374665));
#58824=CARTESIAN_POINT('Ctrl Pts',(1.71405450210392,-1.,-3.67083454901629));
#58825=CARTESIAN_POINT('Ctrl Pts',(1.71405450210392,1.,-3.67083454901629));
#58826=CARTESIAN_POINT('Ctrl Pts',(1.70846001610983,-1.,-3.6655804319893));
#58827=CARTESIAN_POINT('Ctrl Pts',(1.70846001610983,1.,-3.6655804319893));
#58828=CARTESIAN_POINT('Ctrl Pts',(1.70289888566904,-1.,-3.6603033877491));
#58829=CARTESIAN_POINT('Ctrl Pts',(1.70289888566904,1.,-3.6603033877491));
#58830=CARTESIAN_POINT('Ctrl Pts',(1.69737117722558,-1.,-3.65500246526798));
#58831=CARTESIAN_POINT('Ctrl Pts',(1.69737117722558,1.,-3.65500246526798));
#58832=CARTESIAN_POINT('Ctrl Pts',(1.691877054817,-1.,-3.64967689827393));
#58833=CARTESIAN_POINT('Ctrl Pts',(1.691877054817,1.,-3.64967689827393));
#58834=CARTESIAN_POINT('Ctrl Pts',(1.68641690471455,-1.,-3.64432638915199));
#58835=CARTESIAN_POINT('Ctrl Pts',(1.68641690471455,1.,-3.64432638915199));
#58836=CARTESIAN_POINT('Ctrl Pts',(1.68099146651577,-1.,-3.63895140887443));
#58837=CARTESIAN_POINT('Ctrl Pts',(1.68099146651577,1.,-3.63895140887443));
#58838=CARTESIAN_POINT('Ctrl Pts',(1.67560193613145,-1.,-3.63355343201211));
#58839=CARTESIAN_POINT('Ctrl Pts',(1.67560193613145,1.,-3.63355343201211));
#58840=CARTESIAN_POINT('Ctrl Pts',(1.67024966008037,-1.,-3.62813422105257));
#58841=CARTESIAN_POINT('Ctrl Pts',(1.67024966008037,1.,-3.62813422105257));
#58842=CARTESIAN_POINT('Ctrl Pts',(1.66493585923853,-1.,-3.62269517989104));
#58843=CARTESIAN_POINT('Ctrl Pts',(1.66493585923853,1.,-3.62269517989104));
#58844=CARTESIAN_POINT('Ctrl Pts',(1.65966133399186,-1.,-3.61723666482457));
#58845=CARTESIAN_POINT('Ctrl Pts',(1.65966133399186,1.,-3.61723666482457));
#58846=CARTESIAN_POINT('Ctrl Pts',(1.65442619244327,-1.,-3.61175734965129));
#58847=CARTESIAN_POINT('Ctrl Pts',(1.65442619244327,1.,-3.61175734965129));
#58848=CARTESIAN_POINT('Ctrl Pts',(1.64922952425833,-1.,-3.60625346556992));
#58849=CARTESIAN_POINT('Ctrl Pts',(1.64922952425833,1.,-3.60625346556992));
#58850=CARTESIAN_POINT('Ctrl Pts',(1.6440700438558,-1.,-3.6007202851384));
#58851=CARTESIAN_POINT('Ctrl Pts',(1.6440700438558,1.,-3.6007202851384));
#58852=CARTESIAN_POINT('Ctrl Pts',(1.63894676675349,-1.,-3.59515368334887));
#58853=CARTESIAN_POINT('Ctrl Pts',(1.63894676675349,1.,-3.59515368334887));
#58854=CARTESIAN_POINT('Ctrl Pts',(1.63385971451259,-1.,-3.58955176627876));
#58855=CARTESIAN_POINT('Ctrl Pts',(1.63385971451259,1.,-3.58955176627876));
#58856=CARTESIAN_POINT('Ctrl Pts',(1.62881051550748,-1.,-3.5839162577435));
#58857=CARTESIAN_POINT('Ctrl Pts',(1.62881051550748,1.,-3.5839162577435));
#58858=CARTESIAN_POINT('Ctrl Pts',(1.62380329464851,-1.,-3.57825455954405));
#58859=CARTESIAN_POINT('Ctrl Pts',(1.62380329464851,1.,-3.57825455954405));
#58860=CARTESIAN_POINT('Ctrl Pts',(1.61884340915412,-1.,-3.57257679609826));
#58861=CARTESIAN_POINT('Ctrl Pts',(1.61884340915412,1.,-3.57257679609826));
#58862=CARTESIAN_POINT('Ctrl Pts',(1.61393581747522,-1.,-3.56689200468404));
#58863=CARTESIAN_POINT('Ctrl Pts',(1.61393581747522,1.,-3.56689200468404));
#58864=CARTESIAN_POINT('Ctrl Pts',(1.60908344685459,-1.,-3.56120432482986));
#58865=CARTESIAN_POINT('Ctrl Pts',(1.60908344685459,1.,-3.56120432482986));
#58866=CARTESIAN_POINT('Ctrl Pts',(1.60428584699848,-1.,-3.55550985096117));
#58867=CARTESIAN_POINT('Ctrl Pts',(1.60428584699848,1.,-3.55550985096117));
#58868=CARTESIAN_POINT('Ctrl Pts',(1.59953698113444,-1.,-3.54979148634426));
#58869=CARTESIAN_POINT('Ctrl Pts',(1.59953698113444,1.,-3.54979148634426));
#58870=CARTESIAN_POINT('Ctrl Pts',(1.5948276694975,-1.,-3.544024581823));
#58871=CARTESIAN_POINT('Ctrl Pts',(1.5948276694975,1.,-3.544024581823));
#58872=CARTESIAN_POINT('Ctrl Pts',(1.59014958368725,-1.,-3.53818616861045));
#58873=CARTESIAN_POINT('Ctrl Pts',(1.59014958368725,1.,-3.53818616861045));
#58874=CARTESIAN_POINT('Ctrl Pts',(1.58549906268083,-1.,-3.53226378147068));
#58875=CARTESIAN_POINT('Ctrl Pts',(1.58549906268083,1.,-3.53226378147068));
#58876=CARTESIAN_POINT('Ctrl Pts',(1.58088027227856,-1.,-3.52626275334899));
#58877=CARTESIAN_POINT('Ctrl Pts',(1.58088027227856,1.,-3.52626275334899));
#58878=CARTESIAN_POINT('Ctrl Pts',(1.5763104998818,-1.,-3.52021847865961));
#58879=CARTESIAN_POINT('Ctrl Pts',(1.5763104998818,1.,-3.52021847865961));
#58880=CARTESIAN_POINT('Ctrl Pts',(1.57181569799774,-1.,-3.51418598431733));
#58881=CARTESIAN_POINT('Ctrl Pts',(1.57181569799774,1.,-3.51418598431733));
#58882=CARTESIAN_POINT('Ctrl Pts',(1.56742097575041,-1.,-3.50821771695427));
#58883=CARTESIAN_POINT('Ctrl Pts',(1.56742097575041,1.,-3.50821771695427));
#58884=CARTESIAN_POINT('Ctrl Pts',(1.56314187758689,-1.,-3.50234321621607));
#58885=CARTESIAN_POINT('Ctrl Pts',(1.56314187758689,1.,-3.50234321621607));
#58886=CARTESIAN_POINT('Ctrl Pts',(1.55897703097859,-1.,-3.49655185179623));
#58887=CARTESIAN_POINT('Ctrl Pts',(1.55897703097859,1.,-3.49655185179623));
#58888=CARTESIAN_POINT('Ctrl Pts',(1.5548959590107,-1.,-3.49076460877317));
#58889=CARTESIAN_POINT('Ctrl Pts',(1.5548959590107,1.,-3.49076460877317));
#58890=CARTESIAN_POINT('Ctrl Pts',(1.55084702970382,-1.,-3.48485155928414));
#58891=CARTESIAN_POINT('Ctrl Pts',(1.55084702970382,1.,-3.48485155928414));
#58892=CARTESIAN_POINT('Ctrl Pts',(1.54678009290206,-1.,-3.47868272898599));
#58893=CARTESIAN_POINT('Ctrl Pts',(1.54678009290206,1.,-3.47868272898599));
#58894=CARTESIAN_POINT('Ctrl Pts',(1.54266605398152,-1.,-3.47217189224576));
#58895=CARTESIAN_POINT('Ctrl Pts',(1.54266605398152,1.,-3.47217189224576));
#58896=CARTESIAN_POINT('Ctrl Pts',(1.53851507915533,-1.,-3.46531752207222));
#58897=CARTESIAN_POINT('Ctrl Pts',(1.53851507915533,1.,-3.46531752207222));
#58898=CARTESIAN_POINT('Ctrl Pts',(1.53440195378902,-1.,-3.45825932955273));
#58899=CARTESIAN_POINT('Ctrl Pts',(1.53440195378902,1.,-3.45825932955273));
#58900=CARTESIAN_POINT('Ctrl Pts',(1.530462444618,-1.,-3.45127136828667));
#58901=CARTESIAN_POINT('Ctrl Pts',(1.530462444618,1.,-3.45127136828667));
#58902=CARTESIAN_POINT('Ctrl Pts',(1.52686242875717,-1.,-3.44469547527));
#58903=CARTESIAN_POINT('Ctrl Pts',(1.52686242875717,1.,-3.44469547527));
#58904=CARTESIAN_POINT('Ctrl Pts',(1.52377348950429,-1.,-3.43888895974182));
#58905=CARTESIAN_POINT('Ctrl Pts',(1.52377348950429,1.,-3.43888895974182));
#58906=CARTESIAN_POINT('Ctrl Pts',(1.52134826724227,-1.,-3.43417156977749));
#58907=CARTESIAN_POINT('Ctrl Pts',(1.52134826724227,1.,-3.43417156977749));
#58908=CARTESIAN_POINT('Ctrl Pts',(1.51969006980792,-1.,-3.43076036253384));
#58909=CARTESIAN_POINT('Ctrl Pts',(1.51969006980792,1.,-3.43076036253384));
#58910=CARTESIAN_POINT('Ctrl Pts',(1.51901585838879,-1.,-3.42915787669388));
#58911=CARTESIAN_POINT('Ctrl Pts',(1.51901585838879,1.,-3.42915787669388));
#58912=CARTESIAN_POINT('Ctrl Pts',(1.51888450659497,-1.,-3.42860527148835));
#58913=CARTESIAN_POINT('Ctrl Pts',(1.51888450659497,1.,-3.42860527148835));
#58914=CARTESIAN_POINT('Ctrl Pts',(1.51896318668306,-1.,-3.42852521763648));
#58915=CARTESIAN_POINT('Ctrl Pts',(1.51896318668306,1.,-3.42852521763648));
#58916=CARTESIAN_POINT('Ctrl Pts',(1.519044091397,-1.,-3.42855728381368));
#58917=CARTESIAN_POINT('Ctrl Pts',(1.519044091397,1.,-3.42855728381368));
#58918=CARTESIAN_POINT('',(1.83867539237861,1.,-3.77614523045147));
#58919=CARTESIAN_POINT('Ctrl Pts',(1.83867539237861,1.,-3.77614523045147));
#58920=CARTESIAN_POINT('Ctrl Pts',(1.83742834010821,1.,-3.77518714458232));
#58921=CARTESIAN_POINT('Ctrl Pts',(1.83493697935064,1.,-3.77326886065484));
#58922=CARTESIAN_POINT('Ctrl Pts',(1.83120816956515,1.,-3.77038509819777));
#58923=CARTESIAN_POINT('Ctrl Pts',(1.82625289221933,1.,-3.76652740355856));
#58924=CARTESIAN_POINT('Ctrl Pts',(1.82008629694924,1.,-3.76168412709652));
#58925=CARTESIAN_POINT('Ctrl Pts',(1.81394729834032,1.,-3.75681965683995));
#58926=CARTESIAN_POINT('Ctrl Pts',(1.80783603939662,1.,-3.75193395888069));
#58927=CARTESIAN_POINT('Ctrl Pts',(1.80175271485519,1.,-3.74702700874954));
#58928=CARTESIAN_POINT('Ctrl Pts',(1.79569757859041,1.,-3.74209880351667));
#58929=CARTESIAN_POINT('Ctrl Pts',(1.78967092823139,1.,-3.73714934729962));
#58930=CARTESIAN_POINT('Ctrl Pts',(1.78367308442682,1.,-3.73217863095022));
#58931=CARTESIAN_POINT('Ctrl Pts',(1.77770437039606,1.,-3.72718661205504));
#58932=CARTESIAN_POINT('Ctrl Pts',(1.77176509401846,1.,-3.72217319911429));
#58933=CARTESIAN_POINT('Ctrl Pts',(1.76585552124549,1.,-3.71713822377676));
#58934=CARTESIAN_POINT('Ctrl Pts',(1.75997588499021,1.,-3.71208146346455));
#58935=CARTESIAN_POINT('Ctrl Pts',(1.75412641804148,1.,-3.70700269736876));
#58936=CARTESIAN_POINT('Ctrl Pts',(1.74830738046092,1.,-3.70190175673422));
#58937=CARTESIAN_POINT('Ctrl Pts',(1.74251908492589,1.,-3.6967785691046));
#58938=CARTESIAN_POINT('Ctrl Pts',(1.73676193254493,1.,-3.69163322647906));
#58939=CARTESIAN_POINT('Ctrl Pts',(1.73103640956647,1.,-3.68646597019188));
#58940=CARTESIAN_POINT('Ctrl Pts',(1.72534302437003,1.,-3.68127704936472));
#58941=CARTESIAN_POINT('Ctrl Pts',(1.71968225581787,1.,-3.67606660374665));
#58942=CARTESIAN_POINT('Ctrl Pts',(1.71405450210392,1.,-3.67083454901629));
#58943=CARTESIAN_POINT('Ctrl Pts',(1.70846001610983,1.,-3.6655804319893));
#58944=CARTESIAN_POINT('Ctrl Pts',(1.70289888566904,1.,-3.6603033877491));
#58945=CARTESIAN_POINT('Ctrl Pts',(1.69737117722558,1.,-3.65500246526798));
#58946=CARTESIAN_POINT('Ctrl Pts',(1.691877054817,1.,-3.64967689827393));
#58947=CARTESIAN_POINT('Ctrl Pts',(1.68641690471455,1.,-3.64432638915199));
#58948=CARTESIAN_POINT('Ctrl Pts',(1.68099146651577,1.,-3.63895140887443));
#58949=CARTESIAN_POINT('Ctrl Pts',(1.67560193613145,1.,-3.63355343201211));
#58950=CARTESIAN_POINT('Ctrl Pts',(1.67024966008037,1.,-3.62813422105257));
#58951=CARTESIAN_POINT('Ctrl Pts',(1.66493585923853,1.,-3.62269517989104));
#58952=CARTESIAN_POINT('Ctrl Pts',(1.65966133399186,1.,-3.61723666482457));
#58953=CARTESIAN_POINT('Ctrl Pts',(1.65442619244327,1.,-3.61175734965129));
#58954=CARTESIAN_POINT('Ctrl Pts',(1.64922952425833,1.,-3.60625346556992));
#58955=CARTESIAN_POINT('Ctrl Pts',(1.6440700438558,1.,-3.6007202851384));
#58956=CARTESIAN_POINT('Ctrl Pts',(1.63894676675349,1.,-3.59515368334887));
#58957=CARTESIAN_POINT('Ctrl Pts',(1.63385971451259,1.,-3.58955176627876));
#58958=CARTESIAN_POINT('Ctrl Pts',(1.62881051550748,1.,-3.5839162577435));
#58959=CARTESIAN_POINT('Ctrl Pts',(1.62380329464851,1.,-3.57825455954405));
#58960=CARTESIAN_POINT('Ctrl Pts',(1.61884340915412,1.,-3.57257679609826));
#58961=CARTESIAN_POINT('Ctrl Pts',(1.61393581747522,1.,-3.56689200468404));
#58962=CARTESIAN_POINT('Ctrl Pts',(1.60908344685459,1.,-3.56120432482986));
#58963=CARTESIAN_POINT('Ctrl Pts',(1.60428584699848,1.,-3.55550985096117));
#58964=CARTESIAN_POINT('Ctrl Pts',(1.59953698113444,1.,-3.54979148634426));
#58965=CARTESIAN_POINT('Ctrl Pts',(1.5948276694975,1.,-3.544024581823));
#58966=CARTESIAN_POINT('Ctrl Pts',(1.59014958368725,1.,-3.53818616861045));
#58967=CARTESIAN_POINT('Ctrl Pts',(1.58549906268083,1.,-3.53226378147068));
#58968=CARTESIAN_POINT('Ctrl Pts',(1.58088027227856,1.,-3.52626275334899));
#58969=CARTESIAN_POINT('Ctrl Pts',(1.5763104998818,1.,-3.52021847865961));
#58970=CARTESIAN_POINT('Ctrl Pts',(1.57181569799774,1.,-3.51418598431733));
#58971=CARTESIAN_POINT('Ctrl Pts',(1.56742097575041,1.,-3.50821771695427));
#58972=CARTESIAN_POINT('Ctrl Pts',(1.56314187758689,1.,-3.50234321621607));
#58973=CARTESIAN_POINT('Ctrl Pts',(1.55897703097859,1.,-3.49655185179623));
#58974=CARTESIAN_POINT('Ctrl Pts',(1.5548959590107,1.,-3.49076460877317));
#58975=CARTESIAN_POINT('Ctrl Pts',(1.55084702970382,1.,-3.48485155928414));
#58976=CARTESIAN_POINT('Ctrl Pts',(1.54678009290206,1.,-3.47868272898599));
#58977=CARTESIAN_POINT('Ctrl Pts',(1.54266605398152,1.,-3.47217189224576));
#58978=CARTESIAN_POINT('Ctrl Pts',(1.53851507915533,1.,-3.46531752207222));
#58979=CARTESIAN_POINT('Ctrl Pts',(1.53440195378902,1.,-3.45825932955273));
#58980=CARTESIAN_POINT('Ctrl Pts',(1.530462444618,1.,-3.45127136828667));
#58981=CARTESIAN_POINT('Ctrl Pts',(1.52686242875717,1.,-3.44469547527));
#58982=CARTESIAN_POINT('Ctrl Pts',(1.52377348950429,1.,-3.43888895974182));
#58983=CARTESIAN_POINT('Ctrl Pts',(1.52134826724227,1.,-3.43417156977749));
#58984=CARTESIAN_POINT('Ctrl Pts',(1.5198144909343,1.,-3.43101631893491));
#58985=CARTESIAN_POINT('Ctrl Pts',(1.51914806898539,1.,-3.42946838852728));
#58986=CARTESIAN_POINT('Ctrl Pts',(1.51895133295017,1.,-3.42884302333978));
#58987=CARTESIAN_POINT('Ctrl Pts',(1.51893924967231,1.,-3.42864616361967));
#58988=CARTESIAN_POINT('Ctrl Pts',(1.51895082866166,1.,-3.42859860294378));
#58989=CARTESIAN_POINT('',(1.83867539237861,0.,-3.77614523045147));
#58990=CARTESIAN_POINT('Ctrl Pts',(1.8808893942881,-1.,-3.24418789321065));
#58991=CARTESIAN_POINT('Ctrl Pts',(1.8808893942881,1.,-3.24418789321065));
#58992=CARTESIAN_POINT('Ctrl Pts',(1.8809110068042,-1.,-3.24410359189733));
#58993=CARTESIAN_POINT('Ctrl Pts',(1.8809110068042,1.,-3.24410359189733));
#58994=CARTESIAN_POINT('Ctrl Pts',(1.8810220187274,-1.,-3.24408699284449));
#58995=CARTESIAN_POINT('Ctrl Pts',(1.8810220187274,1.,-3.24408699284449));
#58996=CARTESIAN_POINT('Ctrl Pts',(1.88139187908347,-1.,-3.24451807186964));
#58997=CARTESIAN_POINT('Ctrl Pts',(1.88139187908347,1.,-3.24451807186964));
#58998=CARTESIAN_POINT('Ctrl Pts',(1.88229202583187,-1.,-3.24600543790876));
#58999=CARTESIAN_POINT('Ctrl Pts',(1.88229202583187,1.,-3.24600543790876));
#59000=CARTESIAN_POINT('Ctrl Pts',(1.88407708646435,-1.,-3.24935200512055));
#59001=CARTESIAN_POINT('Ctrl Pts',(1.88407708646435,1.,-3.24935200512055));
#59002=CARTESIAN_POINT('Ctrl Pts',(1.88646802523372,-1.,-3.25408686339298));
#59003=CARTESIAN_POINT('Ctrl Pts',(1.88646802523372,1.,-3.25408686339298));
#59004=CARTESIAN_POINT('Ctrl Pts',(1.88934996203508,-1.,-3.2599988519361));
#59005=CARTESIAN_POINT('Ctrl Pts',(1.88934996203508,1.,-3.2599988519361));
#59006=CARTESIAN_POINT('Ctrl Pts',(1.89255393500769,-1.,-3.2667765388833));
#59007=CARTESIAN_POINT('Ctrl Pts',(1.89255393500769,1.,-3.2667765388833));
#59008=CARTESIAN_POINT('Ctrl Pts',(1.89589172903662,-1.,-3.27407108932908));
#59009=CARTESIAN_POINT('Ctrl Pts',(1.89589172903662,1.,-3.27407108932908));
#59010=CARTESIAN_POINT('Ctrl Pts',(1.89918429230424,-1.,-3.28154737912287));
#59011=CARTESIAN_POINT('Ctrl Pts',(1.89918429230424,1.,-3.28154737912287));
#59012=CARTESIAN_POINT('Ctrl Pts',(1.9022897124757,-1.,-3.28893448600364));
#59013=CARTESIAN_POINT('Ctrl Pts',(1.9022897124757,1.,-3.28893448600364));
#59014=CARTESIAN_POINT('Ctrl Pts',(1.9051389186417,-1.,-3.29608978722258));
#59015=CARTESIAN_POINT('Ctrl Pts',(1.9051389186417,1.,-3.29608978722258));
#59016=CARTESIAN_POINT('Ctrl Pts',(1.90773912171424,-1.,-3.30300595568341));
#59017=CARTESIAN_POINT('Ctrl Pts',(1.90773912171424,1.,-3.30300595568341));
#59018=CARTESIAN_POINT('Ctrl Pts',(1.91014297830502,-1.,-3.30975721158694));
#59019=CARTESIAN_POINT('Ctrl Pts',(1.91014297830502,1.,-3.30975721158694));
#59020=CARTESIAN_POINT('Ctrl Pts',(1.91242616234459,-1.,-3.31646052426395));
#59021=CARTESIAN_POINT('Ctrl Pts',(1.91242616234459,1.,-3.31646052426395));
#59022=CARTESIAN_POINT('Ctrl Pts',(1.91466343916612,-1.,-3.32323403454507));
#59023=CARTESIAN_POINT('Ctrl Pts',(1.91466343916612,1.,-3.32323403454507));
#59024=CARTESIAN_POINT('Ctrl Pts',(1.91690081930297,-1.,-3.33014884257812));
#59025=CARTESIAN_POINT('Ctrl Pts',(1.91690081930297,1.,-3.33014884257812));
#59026=CARTESIAN_POINT('Ctrl Pts',(1.91914609610173,-1.,-3.33721230709948));
#59027=CARTESIAN_POINT('Ctrl Pts',(1.91914609610173,1.,-3.33721230709948));
#59028=CARTESIAN_POINT('Ctrl Pts',(1.92138450828378,-1.,-3.34439448941915));
#59029=CARTESIAN_POINT('Ctrl Pts',(1.92138450828378,1.,-3.34439448941915));
#59030=CARTESIAN_POINT('Ctrl Pts',(1.92358838440518,-1.,-3.35164424847207));
#59031=CARTESIAN_POINT('Ctrl Pts',(1.92358838440518,1.,-3.35164424847207));
#59032=CARTESIAN_POINT('Ctrl Pts',(1.92572846125763,-1.,-3.35890824422976));
#59033=CARTESIAN_POINT('Ctrl Pts',(1.92572846125763,1.,-3.35890824422976));
#59034=CARTESIAN_POINT('Ctrl Pts',(1.92778626543803,-1.,-3.36615168657597));
#59035=CARTESIAN_POINT('Ctrl Pts',(1.92778626543803,1.,-3.36615168657597));
#59036=CARTESIAN_POINT('Ctrl Pts',(1.92975993109897,-1.,-3.37336807068078));
#59037=CARTESIAN_POINT('Ctrl Pts',(1.92975993109897,1.,-3.37336807068078));
#59038=CARTESIAN_POINT('Ctrl Pts',(1.93165739093292,-1.,-3.38056768525577));
#59039=CARTESIAN_POINT('Ctrl Pts',(1.93165739093292,1.,-3.38056768525577));
#59040=CARTESIAN_POINT('Ctrl Pts',(1.93349233176794,-1.,-3.38777076883267));
#59041=CARTESIAN_POINT('Ctrl Pts',(1.93349233176794,1.,-3.38777076883267));
#59042=CARTESIAN_POINT('Ctrl Pts',(1.93527929945982,-1.,-3.39499923640789));
#59043=CARTESIAN_POINT('Ctrl Pts',(1.93527929945982,1.,-3.39499923640789));
#59044=CARTESIAN_POINT('Ctrl Pts',(1.93702857723089,-1.,-3.40226802104093));
#59045=CARTESIAN_POINT('Ctrl Pts',(1.93702857723089,1.,-3.40226802104093));
#59046=CARTESIAN_POINT('Ctrl Pts',(1.93874306008132,-1.,-3.40957978266623));
#59047=CARTESIAN_POINT('Ctrl Pts',(1.93874306008132,1.,-3.40957978266623));
#59048=CARTESIAN_POINT('Ctrl Pts',(1.94042111965237,-1.,-3.41692971994082));
#59049=CARTESIAN_POINT('Ctrl Pts',(1.94042111965237,1.,-3.41692971994082));
#59050=CARTESIAN_POINT('Ctrl Pts',(1.94205835913692,-1.,-3.42430850941497));
#59051=CARTESIAN_POINT('Ctrl Pts',(1.94205835913692,1.,-3.42430850941497));
#59052=CARTESIAN_POINT('Ctrl Pts',(1.94364973660285,-1.,-3.43170586602436));
#59053=CARTESIAN_POINT('Ctrl Pts',(1.94364973660285,1.,-3.43170586602436));
#59054=CARTESIAN_POINT('Ctrl Pts',(1.94519168842883,-1.,-3.43911410197693));
#59055=CARTESIAN_POINT('Ctrl Pts',(1.94519168842883,1.,-3.43911410197693));
#59056=CARTESIAN_POINT('Ctrl Pts',(1.94668377715332,-1.,-3.44653088665685));
#59057=CARTESIAN_POINT('Ctrl Pts',(1.94668377715332,1.,-3.44653088665685));
#59058=CARTESIAN_POINT('Ctrl Pts',(1.94812754766524,-1.,-3.45395731584051));
#59059=CARTESIAN_POINT('Ctrl Pts',(1.94812754766524,1.,-3.45395731584051));
#59060=CARTESIAN_POINT('Ctrl Pts',(1.94952575850196,-1.,-3.46139661060959));
#59061=CARTESIAN_POINT('Ctrl Pts',(1.94952575850196,1.,-3.46139661060959));
#59062=CARTESIAN_POINT('Ctrl Pts',(1.95088147859876,-1.,-3.4688525897419));
#59063=CARTESIAN_POINT('Ctrl Pts',(1.95088147859876,1.,-3.4688525897419));
#59064=CARTESIAN_POINT('Ctrl Pts',(1.95219722189878,-1.,-3.47632820495926));
#59065=CARTESIAN_POINT('Ctrl Pts',(1.95219722189878,1.,-3.47632820495926));
#59066=CARTESIAN_POINT('Ctrl Pts',(1.95347412486316,-1.,-3.48382414832649));
#59067=CARTESIAN_POINT('Ctrl Pts',(1.95347412486316,1.,-3.48382414832649));
#59068=CARTESIAN_POINT('Ctrl Pts',(1.95471236969653,-1.,-3.49133956289154));
#59069=CARTESIAN_POINT('Ctrl Pts',(1.95471236969653,1.,-3.49133956289154));
#59070=CARTESIAN_POINT('Ctrl Pts',(1.9559115382367,-1.,-3.49887263575602));
#59071=CARTESIAN_POINT('Ctrl Pts',(1.9559115382367,1.,-3.49887263575602));
#59072=CARTESIAN_POINT('Ctrl Pts',(1.95707099606513,-1.,-3.50642124159913));
#59073=CARTESIAN_POINT('Ctrl Pts',(1.95707099606513,1.,-3.50642124159913));
#59074=CARTESIAN_POINT('Ctrl Pts',(1.95819025316768,-1.,-3.51398354617773));
#59075=CARTESIAN_POINT('Ctrl Pts',(1.95819025316768,1.,-3.51398354617773));
#59076=CARTESIAN_POINT('Ctrl Pts',(1.95926936324436,-1.,-3.52155867431438));
#59077=CARTESIAN_POINT('Ctrl Pts',(1.95926936324436,1.,-3.52155867431438));
#59078=CARTESIAN_POINT('Ctrl Pts',(1.96030879411534,-1.,-3.52914648844289));
#59079=CARTESIAN_POINT('Ctrl Pts',(1.96030879411534,1.,-3.52914648844289));
#59080=CARTESIAN_POINT('Ctrl Pts',(1.96130926212661,-1.,-3.53674730625759));
#59081=CARTESIAN_POINT('Ctrl Pts',(1.96130926212661,1.,-3.53674730625759));
#59082=CARTESIAN_POINT('Ctrl Pts',(1.96227157573058,-1.,-3.54436163300425));
#59083=CARTESIAN_POINT('Ctrl Pts',(1.96227157573058,1.,-3.54436163300425));
#59084=CARTESIAN_POINT('Ctrl Pts',(1.96319648628667,-1.,-3.55198990600929));
#59085=CARTESIAN_POINT('Ctrl Pts',(1.96319648628667,1.,-3.55198990600929));
#59086=CARTESIAN_POINT('Ctrl Pts',(1.96408450906868,-1.,-3.55963218706201));
#59087=CARTESIAN_POINT('Ctrl Pts',(1.96408450906868,1.,-3.55963218706201));
#59088=CARTESIAN_POINT('Ctrl Pts',(1.96493594634643,-1.,-3.56728820357933));
#59089=CARTESIAN_POINT('Ctrl Pts',(1.96493594634643,1.,-3.56728820357933));
#59090=CARTESIAN_POINT('Ctrl Pts',(1.96575096652857,-1.,-3.57495748601088));
#59091=CARTESIAN_POINT('Ctrl Pts',(1.96575096652857,1.,-3.57495748601088));
#59092=CARTESIAN_POINT('Ctrl Pts',(1.9665296668894,-1.,-3.58263947663884));
#59093=CARTESIAN_POINT('Ctrl Pts',(1.9665296668894,1.,-3.58263947663884));
#59094=CARTESIAN_POINT('Ctrl Pts',(1.96727213799507,-1.,-3.5903336402273));
#59095=CARTESIAN_POINT('Ctrl Pts',(1.96727213799507,1.,-3.5903336402273));
#59096=CARTESIAN_POINT('Ctrl Pts',(1.96797854118257,-1.,-3.59803959819725));
#59097=CARTESIAN_POINT('Ctrl Pts',(1.96797854118257,1.,-3.59803959819725));
#59098=CARTESIAN_POINT('Ctrl Pts',(1.96864911885775,-1.,-3.60575714017676));
#59099=CARTESIAN_POINT('Ctrl Pts',(1.96864911885775,1.,-3.60575714017676));
#59100=CARTESIAN_POINT('Ctrl Pts',(1.96928416040712,-1.,-3.61348615496393));
#59101=CARTESIAN_POINT('Ctrl Pts',(1.96928416040712,1.,-3.61348615496393));
#59102=CARTESIAN_POINT('Ctrl Pts',(1.96988398129888,-1.,-3.62122658401722));
#59103=CARTESIAN_POINT('Ctrl Pts',(1.96988398129888,1.,-3.62122658401722));
#59104=CARTESIAN_POINT('Ctrl Pts',(1.97044889850518,-1.,-3.62897836973397));
#59105=CARTESIAN_POINT('Ctrl Pts',(1.97044889850518,1.,-3.62897836973397));
#59106=CARTESIAN_POINT('Ctrl Pts',(1.97097920454698,-1.,-3.63674139590853));
#59107=CARTESIAN_POINT('Ctrl Pts',(1.97097920454698,1.,-3.63674139590853));
#59108=CARTESIAN_POINT('Ctrl Pts',(1.97147515441539,-1.,-3.64451546724222));
#59109=CARTESIAN_POINT('Ctrl Pts',(1.97147515441539,1.,-3.64451546724222));
#59110=CARTESIAN_POINT('Ctrl Pts',(1.97193697240645,-1.,-3.65230034717364));
#59111=CARTESIAN_POINT('Ctrl Pts',(1.97193697240645,1.,-3.65230034717364));
#59112=CARTESIAN_POINT('Ctrl Pts',(1.97236485439317,-1.,-3.66009578166865));
#59113=CARTESIAN_POINT('Ctrl Pts',(1.97236485439317,1.,-3.66009578166865));
#59114=CARTESIAN_POINT('Ctrl Pts',(1.9727589719863,-1.,-3.66790152751984));
#59115=CARTESIAN_POINT('Ctrl Pts',(1.9727589719863,1.,-3.66790152751984));
#59116=CARTESIAN_POINT('Ctrl Pts',(1.97311947678035,-1.,-3.67571738106175));
#59117=CARTESIAN_POINT('Ctrl Pts',(1.97311947678035,1.,-3.67571738106175));
#59118=CARTESIAN_POINT('Ctrl Pts',(1.9734465030363,-1.,-3.68354319913416));
#59119=CARTESIAN_POINT('Ctrl Pts',(1.9734465030363,1.,-3.68354319913416));
#59120=CARTESIAN_POINT('Ctrl Pts',(1.97374016224397,-1.,-3.69137888597855));
#59121=CARTESIAN_POINT('Ctrl Pts',(1.97374016224397,1.,-3.69137888597855));
#59122=CARTESIAN_POINT('Ctrl Pts',(1.97394846382288,-1.,-3.69765528558292));
#59123=CARTESIAN_POINT('Ctrl Pts',(1.97394846382288,1.,-3.69765528558292));
#59124=CARTESIAN_POINT('Ctrl Pts',(1.97408973726149,-1.,-3.70236698911837));
#59125=CARTESIAN_POINT('Ctrl Pts',(1.97408973726149,1.,-3.70236698911837));
#59126=CARTESIAN_POINT('Ctrl Pts',(1.974177276451,-1.,-3.7055100813194));
#59127=CARTESIAN_POINT('Ctrl Pts',(1.974177276451,1.,-3.7055100813194));
#59128=CARTESIAN_POINT('Ctrl Pts',(1.97421938526992,-1.,-3.70708211654725));
#59129=CARTESIAN_POINT('Ctrl Pts',(1.97421938526992,1.,-3.70708211654725));
#59130=CARTESIAN_POINT('',(1.88097764062542,1.,-3.24413672884902));
#59131=CARTESIAN_POINT('Ctrl Pts',(1.88097764062541,-1.,-3.24413672884902));
#59132=CARTESIAN_POINT('Ctrl Pts',(1.88097764062541,-0.666666666666667,
-3.24413672884902));
#59133=CARTESIAN_POINT('Ctrl Pts',(1.88097764062541,-0.333333333333333,
-3.24413672884902));
#59134=CARTESIAN_POINT('Ctrl Pts',(1.88097764062541,0.333333333333333,-3.24413672884902));
#59135=CARTESIAN_POINT('Ctrl Pts',(1.88097764062541,0.666666666666667,-3.24413672884902));
#59136=CARTESIAN_POINT('Ctrl Pts',(1.88097764062541,1.,-3.24413672884902));
#59137=CARTESIAN_POINT('',(1.97421938526992,1.,-3.70708211654725));
#59138=CARTESIAN_POINT('',(1.97421938526992,0.,-3.70708211654725));
#59139=CARTESIAN_POINT('Ctrl Pts',(1.88097764062542,1.,-3.24413672884902));
#59140=CARTESIAN_POINT('Ctrl Pts',(1.88102292397987,1.,-3.24415531671311));
#59141=CARTESIAN_POINT('Ctrl Pts',(1.88117508446657,1.,-3.24428080352952));
#59142=CARTESIAN_POINT('Ctrl Pts',(1.88156537699118,1.,-3.24480754675942));
#59143=CARTESIAN_POINT('Ctrl Pts',(1.88242596600422,1.,-3.24625654410705));
#59144=CARTESIAN_POINT('Ctrl Pts',(1.88407708646435,1.,-3.24935200512055));
#59145=CARTESIAN_POINT('Ctrl Pts',(1.88646802523372,1.,-3.25408686339298));
#59146=CARTESIAN_POINT('Ctrl Pts',(1.88934996203508,1.,-3.2599988519361));
#59147=CARTESIAN_POINT('Ctrl Pts',(1.89255393500769,1.,-3.2667765388833));
#59148=CARTESIAN_POINT('Ctrl Pts',(1.89589172903662,1.,-3.27407108932908));
#59149=CARTESIAN_POINT('Ctrl Pts',(1.89918429230424,1.,-3.28154737912287));
#59150=CARTESIAN_POINT('Ctrl Pts',(1.9022897124757,1.,-3.28893448600364));
#59151=CARTESIAN_POINT('Ctrl Pts',(1.9051389186417,1.,-3.29608978722258));
#59152=CARTESIAN_POINT('Ctrl Pts',(1.90773912171424,1.,-3.30300595568341));
#59153=CARTESIAN_POINT('Ctrl Pts',(1.91014297830502,1.,-3.30975721158694));
#59154=CARTESIAN_POINT('Ctrl Pts',(1.91242616234459,1.,-3.31646052426395));
#59155=CARTESIAN_POINT('Ctrl Pts',(1.91466343916612,1.,-3.32323403454507));
#59156=CARTESIAN_POINT('Ctrl Pts',(1.91690081930297,1.,-3.33014884257812));
#59157=CARTESIAN_POINT('Ctrl Pts',(1.91914609610173,1.,-3.33721230709948));
#59158=CARTESIAN_POINT('Ctrl Pts',(1.92138450828378,1.,-3.34439448941915));
#59159=CARTESIAN_POINT('Ctrl Pts',(1.92358838440518,1.,-3.35164424847207));
#59160=CARTESIAN_POINT('Ctrl Pts',(1.92572846125763,1.,-3.35890824422976));
#59161=CARTESIAN_POINT('Ctrl Pts',(1.92778626543803,1.,-3.36615168657597));
#59162=CARTESIAN_POINT('Ctrl Pts',(1.92975993109897,1.,-3.37336807068078));
#59163=CARTESIAN_POINT('Ctrl Pts',(1.93165739093292,1.,-3.38056768525577));
#59164=CARTESIAN_POINT('Ctrl Pts',(1.93349233176794,1.,-3.38777076883267));
#59165=CARTESIAN_POINT('Ctrl Pts',(1.93527929945982,1.,-3.39499923640789));
#59166=CARTESIAN_POINT('Ctrl Pts',(1.93702857723089,1.,-3.40226802104093));
#59167=CARTESIAN_POINT('Ctrl Pts',(1.93874306008132,1.,-3.40957978266623));
#59168=CARTESIAN_POINT('Ctrl Pts',(1.94042111965237,1.,-3.41692971994082));
#59169=CARTESIAN_POINT('Ctrl Pts',(1.94205835913692,1.,-3.42430850941497));
#59170=CARTESIAN_POINT('Ctrl Pts',(1.94364973660285,1.,-3.43170586602436));
#59171=CARTESIAN_POINT('Ctrl Pts',(1.94519168842883,1.,-3.43911410197693));
#59172=CARTESIAN_POINT('Ctrl Pts',(1.94668377715332,1.,-3.44653088665685));
#59173=CARTESIAN_POINT('Ctrl Pts',(1.94812754766524,1.,-3.45395731584051));
#59174=CARTESIAN_POINT('Ctrl Pts',(1.94952575850196,1.,-3.46139661060959));
#59175=CARTESIAN_POINT('Ctrl Pts',(1.95088147859876,1.,-3.4688525897419));
#59176=CARTESIAN_POINT('Ctrl Pts',(1.95219722189878,1.,-3.47632820495926));
#59177=CARTESIAN_POINT('Ctrl Pts',(1.95347412486316,1.,-3.48382414832649));
#59178=CARTESIAN_POINT('Ctrl Pts',(1.95471236969653,1.,-3.49133956289154));
#59179=CARTESIAN_POINT('Ctrl Pts',(1.9559115382367,1.,-3.49887263575602));
#59180=CARTESIAN_POINT('Ctrl Pts',(1.95707099606513,1.,-3.50642124159913));
#59181=CARTESIAN_POINT('Ctrl Pts',(1.95819025316768,1.,-3.51398354617773));
#59182=CARTESIAN_POINT('Ctrl Pts',(1.95926936324436,1.,-3.52155867431438));
#59183=CARTESIAN_POINT('Ctrl Pts',(1.96030879411534,1.,-3.52914648844289));
#59184=CARTESIAN_POINT('Ctrl Pts',(1.96130926212661,1.,-3.53674730625759));
#59185=CARTESIAN_POINT('Ctrl Pts',(1.96227157573058,1.,-3.54436163300425));
#59186=CARTESIAN_POINT('Ctrl Pts',(1.96319648628667,1.,-3.55198990600929));
#59187=CARTESIAN_POINT('Ctrl Pts',(1.96408450906868,1.,-3.55963218706201));
#59188=CARTESIAN_POINT('Ctrl Pts',(1.96493594634643,1.,-3.56728820357933));
#59189=CARTESIAN_POINT('Ctrl Pts',(1.96575096652857,1.,-3.57495748601088));
#59190=CARTESIAN_POINT('Ctrl Pts',(1.9665296668894,1.,-3.58263947663884));
#59191=CARTESIAN_POINT('Ctrl Pts',(1.96727213799507,1.,-3.5903336402273));
#59192=CARTESIAN_POINT('Ctrl Pts',(1.96797854118257,1.,-3.59803959819725));
#59193=CARTESIAN_POINT('Ctrl Pts',(1.96864911885775,1.,-3.60575714017676));
#59194=CARTESIAN_POINT('Ctrl Pts',(1.96928416040712,1.,-3.61348615496393));
#59195=CARTESIAN_POINT('Ctrl Pts',(1.96988398129888,1.,-3.62122658401722));
#59196=CARTESIAN_POINT('Ctrl Pts',(1.97044889850518,1.,-3.62897836973397));
#59197=CARTESIAN_POINT('Ctrl Pts',(1.97097920454698,1.,-3.63674139590853));
#59198=CARTESIAN_POINT('Ctrl Pts',(1.97147515441539,1.,-3.64451546724222));
#59199=CARTESIAN_POINT('Ctrl Pts',(1.97193697240645,1.,-3.65230034717364));
#59200=CARTESIAN_POINT('Ctrl Pts',(1.97236485439317,1.,-3.66009578166865));
#59201=CARTESIAN_POINT('Ctrl Pts',(1.9727589719863,1.,-3.66790152751984));
#59202=CARTESIAN_POINT('Ctrl Pts',(1.97311947678035,1.,-3.67571738106175));
#59203=CARTESIAN_POINT('Ctrl Pts',(1.9734465030363,1.,-3.68354319913416));
#59204=CARTESIAN_POINT('Ctrl Pts',(1.97374016224397,1.,-3.69137888597855));
#59205=CARTESIAN_POINT('Ctrl Pts',(1.97394846382288,1.,-3.69765528558292));
#59206=CARTESIAN_POINT('Ctrl Pts',(1.97408973726149,1.,-3.70236698911837));
#59207=CARTESIAN_POINT('Ctrl Pts',(1.974177276451,1.,-3.7055100813194));
#59208=CARTESIAN_POINT('Ctrl Pts',(1.97421938526992,1.,-3.70708211654725));
#59209=CARTESIAN_POINT('Origin',(1.97421938526992,0.,-3.70708211654725));
#59210=CARTESIAN_POINT('',(1.83867539237861,1.,-3.77614523045147));
#59211=CARTESIAN_POINT('Origin',(0.,0.,0.));
#59212=CARTESIAN_POINT('',(2.03660101169564,1.,-3.14877060440425));
#59213=CARTESIAN_POINT('Origin',(0.,1.,0.));
#59214=CARTESIAN_POINT('Ctrl Pts',(2.03660101169564,1.,-3.14877060440425));
#59215=CARTESIAN_POINT('Ctrl Pts',(2.03660101169564,0.666666666666667,-3.14877060440425));
#59216=CARTESIAN_POINT('Ctrl Pts',(2.03660101169564,0.333333333333333,-3.14877060440425));
#59217=CARTESIAN_POINT('Ctrl Pts',(2.03660101169564,-0.333333333333333,
-3.14877060440425));
#59218=CARTESIAN_POINT('Ctrl Pts',(2.03660101169564,-0.666666666666667,
-3.14877060440425));
#59219=CARTESIAN_POINT('Ctrl Pts',(2.03660101169564,-1.,-3.14877060440425));
#59220=CARTESIAN_POINT('Ctrl Pts',(2.40675750623143,-1.,-3.44202241512147));
#59221=CARTESIAN_POINT('Ctrl Pts',(2.40675750623143,1.,-3.44202241512147));
#59222=CARTESIAN_POINT('Ctrl Pts',(2.40537592959345,-1.,-3.44127120683402));
#59223=CARTESIAN_POINT('Ctrl Pts',(2.40537592959345,1.,-3.44127120683402));
#59224=CARTESIAN_POINT('Ctrl Pts',(2.40261515590099,-1.,-3.43976627485223));
#59225=CARTESIAN_POINT('Ctrl Pts',(2.40261515590099,1.,-3.43976627485223));
#59226=CARTESIAN_POINT('Ctrl Pts',(2.39848113411428,-1.,-3.43750133066037));
#59227=CARTESIAN_POINT('Ctrl Pts',(2.39848113411428,1.,-3.43750133066037));
#59228=CARTESIAN_POINT('Ctrl Pts',(2.39298338805823,-1.,-3.43446630680436));
#59229=CARTESIAN_POINT('Ctrl Pts',(2.39298338805823,1.,-3.43446630680436));
#59230=CARTESIAN_POINT('Ctrl Pts',(2.38613505844641,-1.,-3.43064732714472));
#59231=CARTESIAN_POINT('Ctrl Pts',(2.38613505844641,1.,-3.43064732714472));
#59232=CARTESIAN_POINT('Ctrl Pts',(2.37931067029517,-1.,-3.42680309755241));
#59233=CARTESIAN_POINT('Ctrl Pts',(2.37931067029517,1.,-3.42680309755241));
#59234=CARTESIAN_POINT('Ctrl Pts',(2.37251035954351,-1.,-3.42293356216595));
#59235=CARTESIAN_POINT('Ctrl Pts',(2.37251035954351,1.,-3.42293356216595));
#59236=CARTESIAN_POINT('Ctrl Pts',(2.36573431470313,-1.,-3.41903866635384));
#59237=CARTESIAN_POINT('Ctrl Pts',(2.36573431470313,1.,-3.41903866635384));
#59238=CARTESIAN_POINT('Ctrl Pts',(2.35898278606449,-1.,-3.4151183675076));
#59239=CARTESIAN_POINT('Ctrl Pts',(2.35898278606449,1.,-3.4151183675076));
#59240=CARTESIAN_POINT('Ctrl Pts',(2.35225606823649,-1.,-3.41117262313464));
#59241=CARTESIAN_POINT('Ctrl Pts',(2.35225606823649,1.,-3.41117262313464));
#59242=CARTESIAN_POINT('Ctrl Pts',(2.34555447648901,-1.,-3.40720137403888));
#59243=CARTESIAN_POINT('Ctrl Pts',(2.34555447648901,1.,-3.40720137403888));
#59244=CARTESIAN_POINT('Ctrl Pts',(2.33887832342715,-1.,-3.40320452776646));
#59245=CARTESIAN_POINT('Ctrl Pts',(2.33887832342715,1.,-3.40320452776646));
#59246=CARTESIAN_POINT('Ctrl Pts',(2.33222789882601,-1.,-3.39918194578115));
#59247=CARTESIAN_POINT('Ctrl Pts',(2.33222789882601,1.,-3.39918194578115));
#59248=CARTESIAN_POINT('Ctrl Pts',(2.32560343902683,-1.,-3.39513342020045));
#59249=CARTESIAN_POINT('Ctrl Pts',(2.32560343902683,1.,-3.39513342020045));
#59250=CARTESIAN_POINT('Ctrl Pts',(2.31900513925627,-1.,-3.39105869475112));
#59251=CARTESIAN_POINT('Ctrl Pts',(2.31900513925627,1.,-3.39105869475112));
#59252=CARTESIAN_POINT('Ctrl Pts',(2.31243319489505,-1.,-3.38695751492659));
#59253=CARTESIAN_POINT('Ctrl Pts',(2.31243319489505,1.,-3.38695751492659));
#59254=CARTESIAN_POINT('Ctrl Pts',(2.30588783640389,-1.,-3.38282967336676));
#59255=CARTESIAN_POINT('Ctrl Pts',(2.30588783640389,1.,-3.38282967336676));
#59256=CARTESIAN_POINT('Ctrl Pts',(2.29936936127588,-1.,-3.37867504959382));
#59257=CARTESIAN_POINT('Ctrl Pts',(2.29936936127588,1.,-3.37867504959382));
#59258=CARTESIAN_POINT('Ctrl Pts',(2.2928781800731,-1.,-3.37449367172707));
#59259=CARTESIAN_POINT('Ctrl Pts',(2.2928781800731,1.,-3.37449367172707));
#59260=CARTESIAN_POINT('Ctrl Pts',(2.28641481081045,-1.,-3.37028570206357));
#59261=CARTESIAN_POINT('Ctrl Pts',(2.28641481081045,1.,-3.37028570206357));
#59262=CARTESIAN_POINT('Ctrl Pts',(2.27997979457968,-1.,-3.36605130712978));
#59263=CARTESIAN_POINT('Ctrl Pts',(2.27997979457968,1.,-3.36605130712978));
#59264=CARTESIAN_POINT('Ctrl Pts',(2.27357362620902,-1.,-3.36179055004369));
#59265=CARTESIAN_POINT('Ctrl Pts',(2.27357362620902,1.,-3.36179055004369));
#59266=CARTESIAN_POINT('Ctrl Pts',(2.26719668579921,-1.,-3.35750328523077));
#59267=CARTESIAN_POINT('Ctrl Pts',(2.26719668579921,1.,-3.35750328523077));
#59268=CARTESIAN_POINT('Ctrl Pts',(2.26084915222484,-1.,-3.35318902552676));
#59269=CARTESIAN_POINT('Ctrl Pts',(2.26084915222484,1.,-3.35318902552676));
#59270=CARTESIAN_POINT('Ctrl Pts',(2.25453097693524,-1.,-3.34884690292342));
#59271=CARTESIAN_POINT('Ctrl Pts',(2.25453097693524,1.,-3.34884690292342));
#59272=CARTESIAN_POINT('Ctrl Pts',(2.24824207678287,-1.,-3.34447596770768));
#59273=CARTESIAN_POINT('Ctrl Pts',(2.24824207678287,1.,-3.34447596770768));
#59274=CARTESIAN_POINT('Ctrl Pts',(2.24198249391437,-1.,-3.34007543738044));
#59275=CARTESIAN_POINT('Ctrl Pts',(2.24198249391437,1.,-3.34007543738044));
#59276=CARTESIAN_POINT('Ctrl Pts',(2.23575256328809,-1.,-3.33564495756478));
#59277=CARTESIAN_POINT('Ctrl Pts',(2.23575256328809,1.,-3.33564495756478));
#59278=CARTESIAN_POINT('Ctrl Pts',(2.22955308907221,-1.,-3.33118487773593));
#59279=CARTESIAN_POINT('Ctrl Pts',(2.22955308907221,1.,-3.33118487773593));
#59280=CARTESIAN_POINT('Ctrl Pts',(2.22338548312758,-1.,-3.32669646722871));
#59281=CARTESIAN_POINT('Ctrl Pts',(2.22338548312758,1.,-3.32669646722871));
#59282=CARTESIAN_POINT('Ctrl Pts',(2.21725135110889,-1.,-3.32218125618955));
#59283=CARTESIAN_POINT('Ctrl Pts',(2.21725135110889,1.,-3.32218125618955));
#59284=CARTESIAN_POINT('Ctrl Pts',(2.21115211847872,-1.,-3.31764044024231));
#59285=CARTESIAN_POINT('Ctrl Pts',(2.21115211847872,1.,-3.31764044024231));
#59286=CARTESIAN_POINT('Ctrl Pts',(2.20508863150608,-1.,-3.3130742460895));
#59287=CARTESIAN_POINT('Ctrl Pts',(2.20508863150608,1.,-3.3130742460895));
#59288=CARTESIAN_POINT('Ctrl Pts',(2.19906078949924,-1.,-3.30848134694597));
#59289=CARTESIAN_POINT('Ctrl Pts',(2.19906078949924,1.,-3.30848134694597));
#59290=CARTESIAN_POINT('Ctrl Pts',(2.19306710376112,-1.,-3.30385816281831));
#59291=CARTESIAN_POINT('Ctrl Pts',(2.19306710376112,1.,-3.30385816281831));
#59292=CARTESIAN_POINT('Ctrl Pts',(2.18710556500325,-1.,-3.29920022557635));
#59293=CARTESIAN_POINT('Ctrl Pts',(2.18710556500325,1.,-3.29920022557635));
#59294=CARTESIAN_POINT('Ctrl Pts',(2.18117455557062,-1.,-3.29450361500484));
#59295=CARTESIAN_POINT('Ctrl Pts',(2.18117455557062,1.,-3.29450361500484));
#59296=CARTESIAN_POINT('Ctrl Pts',(2.17527380048422,-1.,-3.28976645712566));
#59297=CARTESIAN_POINT('Ctrl Pts',(2.17527380048422,1.,-3.28976645712566));
#59298=CARTESIAN_POINT('Ctrl Pts',(2.16940517773459,-1.,-3.2849901997973));
#59299=CARTESIAN_POINT('Ctrl Pts',(2.16940517773459,1.,-3.2849901997973));
#59300=CARTESIAN_POINT('Ctrl Pts',(2.16357391934434,-1.,-3.28018150841414));
#59301=CARTESIAN_POINT('Ctrl Pts',(2.16357391934434,1.,-3.28018150841414));
#59302=CARTESIAN_POINT('Ctrl Pts',(2.15778690038359,-1.,-3.27534954469206));
#59303=CARTESIAN_POINT('Ctrl Pts',(2.15778690038359,1.,-3.27534954469206));
#59304=CARTESIAN_POINT('Ctrl Pts',(2.15205043199818,-1.,-3.27050245897244));
#59305=CARTESIAN_POINT('Ctrl Pts',(2.15205043199818,1.,-3.27050245897244));
#59306=CARTESIAN_POINT('Ctrl Pts',(2.14636805295663,-1.,-3.26564388189764));
#59307=CARTESIAN_POINT('Ctrl Pts',(2.14636805295663,1.,-3.26564388189764));
#59308=CARTESIAN_POINT('Ctrl Pts',(2.14073870754257,-1.,-3.26077002641868));
#59309=CARTESIAN_POINT('Ctrl Pts',(2.14073870754257,1.,-3.26077002641868));
#59310=CARTESIAN_POINT('Ctrl Pts',(2.13515375878786,-1.,-3.25586495065027));
#59311=CARTESIAN_POINT('Ctrl Pts',(2.13515375878786,1.,-3.25586495065027));
#59312=CARTESIAN_POINT('Ctrl Pts',(2.1296002839681,-1.,-3.25090574493994));
#59313=CARTESIAN_POINT('Ctrl Pts',(2.1296002839681,1.,-3.25090574493994));
#59314=CARTESIAN_POINT('Ctrl Pts',(2.12406646410943,-1.,-3.24587102613347));
#59315=CARTESIAN_POINT('Ctrl Pts',(2.12406646410943,1.,-3.24587102613347));
#59316=CARTESIAN_POINT('Ctrl Pts',(2.11854673326972,-1.,-3.24074905517282));
#59317=CARTESIAN_POINT('Ctrl Pts',(2.11854673326972,1.,-3.24074905517282));
#59318=CARTESIAN_POINT('Ctrl Pts',(2.11304604021784,-1.,-3.23554444767115));
#59319=CARTESIAN_POINT('Ctrl Pts',(2.11304604021784,1.,-3.23554444767115));
#59320=CARTESIAN_POINT('Ctrl Pts',(2.1075869964248,-1.,-3.23028945793334));
#59321=CARTESIAN_POINT('Ctrl Pts',(2.1075869964248,1.,-3.23028945793334));
#59322=CARTESIAN_POINT('Ctrl Pts',(2.10220384298533,-1.,-3.22503437553496));
#59323=CARTESIAN_POINT('Ctrl Pts',(2.10220384298533,1.,-3.22503437553496));
#59324=CARTESIAN_POINT('Ctrl Pts',(2.09692958434933,-1.,-3.21982707347067));
#59325=CARTESIAN_POINT('Ctrl Pts',(2.09692958434933,1.,-3.21982707347067));
#59326=CARTESIAN_POINT('Ctrl Pts',(2.0917841946046,-1.,-3.2146942960168));
#59327=CARTESIAN_POINT('Ctrl Pts',(2.0917841946046,1.,-3.2146942960168));
#59328=CARTESIAN_POINT('Ctrl Pts',(2.08676465517435,-1.,-3.20962575845433));
#59329=CARTESIAN_POINT('Ctrl Pts',(2.08676465517435,1.,-3.20962575845433));
#59330=CARTESIAN_POINT('Ctrl Pts',(2.08182850370816,-1.,-3.20454818630635));
#59331=CARTESIAN_POINT('Ctrl Pts',(2.08182850370816,1.,-3.20454818630635));
#59332=CARTESIAN_POINT('Ctrl Pts',(2.0769044187063,-1.,-3.19934132835879));
#59333=CARTESIAN_POINT('Ctrl Pts',(2.0769044187063,1.,-3.19934132835879));
#59334=CARTESIAN_POINT('Ctrl Pts',(2.07192253497765,-1.,-3.19388465568113));
#59335=CARTESIAN_POINT('Ctrl Pts',(2.07192253497765,1.,-3.19388465568113));
#59336=CARTESIAN_POINT('Ctrl Pts',(2.06684062744065,-1.,-3.18809755562297));
#59337=CARTESIAN_POINT('Ctrl Pts',(2.06684062744065,1.,-3.18809755562297));
#59338=CARTESIAN_POINT('Ctrl Pts',(2.06166849827143,-1.,-3.18197692964677));
#59339=CARTESIAN_POINT('Ctrl Pts',(2.06166849827143,1.,-3.18197692964677));
#59340=CARTESIAN_POINT('Ctrl Pts',(2.05650186773279,-1.,-3.17564906975592));
#59341=CARTESIAN_POINT('Ctrl Pts',(2.05650186773279,1.,-3.17564906975592));
#59342=CARTESIAN_POINT('Ctrl Pts',(2.05151770247452,-1.,-3.16936341689859));
#59343=CARTESIAN_POINT('Ctrl Pts',(2.05151770247452,1.,-3.16936341689859));
#59344=CARTESIAN_POINT('Ctrl Pts',(2.0469333124766,-1.,-3.16343165059235));
#59345=CARTESIAN_POINT('Ctrl Pts',(2.0469333124766,1.,-3.16343165059235));
#59346=CARTESIAN_POINT('Ctrl Pts',(2.04297406404132,-1.,-3.15817983946525));
#59347=CARTESIAN_POINT('Ctrl Pts',(2.04297406404132,1.,-3.15817983946525));
#59348=CARTESIAN_POINT('Ctrl Pts',(2.03984073791432,-1.,-3.1538999167466));
#59349=CARTESIAN_POINT('Ctrl Pts',(2.03984073791432,1.,-3.1538999167466));
#59350=CARTESIAN_POINT('Ctrl Pts',(2.03766932526171,-1.,-3.15079010635326));
#59351=CARTESIAN_POINT('Ctrl Pts',(2.03766932526171,1.,-3.15079010635326));
#59352=CARTESIAN_POINT('Ctrl Pts',(2.03675273048882,-1.,-3.14931281967585));
#59353=CARTESIAN_POINT('Ctrl Pts',(2.03675273048882,1.,-3.14931281967585));
#59354=CARTESIAN_POINT('Ctrl Pts',(2.03653654935384,-1.,-3.14878756590499));
#59355=CARTESIAN_POINT('Ctrl Pts',(2.03653654935384,1.,-3.14878756590499));
#59356=CARTESIAN_POINT('Ctrl Pts',(2.036601737578,-1.,-3.14869618937139));
#59357=CARTESIAN_POINT('Ctrl Pts',(2.036601737578,1.,-3.14869618937139));
#59358=CARTESIAN_POINT('Ctrl Pts',(2.03668666247593,-1.,-3.1487152044751));
#59359=CARTESIAN_POINT('Ctrl Pts',(2.03668666247593,1.,-3.1487152044751));
#59360=CARTESIAN_POINT('',(2.40675750623143,1.,-3.44202241512147));
#59361=CARTESIAN_POINT('Ctrl Pts',(2.40675750623143,1.,-3.44202241512147));
#59362=CARTESIAN_POINT('Ctrl Pts',(2.40537592959345,1.,-3.44127120683402));
#59363=CARTESIAN_POINT('Ctrl Pts',(2.40261515590099,1.,-3.43976627485223));
#59364=CARTESIAN_POINT('Ctrl Pts',(2.39848113411428,1.,-3.43750133066037));
#59365=CARTESIAN_POINT('Ctrl Pts',(2.39298338805823,1.,-3.43446630680436));
#59366=CARTESIAN_POINT('Ctrl Pts',(2.38613505844641,1.,-3.43064732714472));
#59367=CARTESIAN_POINT('Ctrl Pts',(2.37931067029517,1.,-3.42680309755241));
#59368=CARTESIAN_POINT('Ctrl Pts',(2.37251035954351,1.,-3.42293356216595));
#59369=CARTESIAN_POINT('Ctrl Pts',(2.36573431470313,1.,-3.41903866635384));
#59370=CARTESIAN_POINT('Ctrl Pts',(2.35898278606449,1.,-3.4151183675076));
#59371=CARTESIAN_POINT('Ctrl Pts',(2.35225606823649,1.,-3.41117262313464));
#59372=CARTESIAN_POINT('Ctrl Pts',(2.34555447648901,1.,-3.40720137403888));
#59373=CARTESIAN_POINT('Ctrl Pts',(2.33887832342715,1.,-3.40320452776646));
#59374=CARTESIAN_POINT('Ctrl Pts',(2.33222789882601,1.,-3.39918194578115));
#59375=CARTESIAN_POINT('Ctrl Pts',(2.32560343902683,1.,-3.39513342020045));
#59376=CARTESIAN_POINT('Ctrl Pts',(2.31900513925627,1.,-3.39105869475112));
#59377=CARTESIAN_POINT('Ctrl Pts',(2.31243319489505,1.,-3.38695751492659));
#59378=CARTESIAN_POINT('Ctrl Pts',(2.30588783640389,1.,-3.38282967336676));
#59379=CARTESIAN_POINT('Ctrl Pts',(2.29936936127588,1.,-3.37867504959382));
#59380=CARTESIAN_POINT('Ctrl Pts',(2.2928781800731,1.,-3.37449367172707));
#59381=CARTESIAN_POINT('Ctrl Pts',(2.28641481081045,1.,-3.37028570206357));
#59382=CARTESIAN_POINT('Ctrl Pts',(2.27997979457968,1.,-3.36605130712978));
#59383=CARTESIAN_POINT('Ctrl Pts',(2.27357362620902,1.,-3.36179055004369));
#59384=CARTESIAN_POINT('Ctrl Pts',(2.26719668579921,1.,-3.35750328523077));
#59385=CARTESIAN_POINT('Ctrl Pts',(2.26084915222484,1.,-3.35318902552676));
#59386=CARTESIAN_POINT('Ctrl Pts',(2.25453097693524,1.,-3.34884690292342));
#59387=CARTESIAN_POINT('Ctrl Pts',(2.24824207678287,1.,-3.34447596770768));
#59388=CARTESIAN_POINT('Ctrl Pts',(2.24198249391437,1.,-3.34007543738044));
#59389=CARTESIAN_POINT('Ctrl Pts',(2.23575256328809,1.,-3.33564495756478));
#59390=CARTESIAN_POINT('Ctrl Pts',(2.22955308907221,1.,-3.33118487773593));
#59391=CARTESIAN_POINT('Ctrl Pts',(2.22338548312758,1.,-3.32669646722871));
#59392=CARTESIAN_POINT('Ctrl Pts',(2.21725135110889,1.,-3.32218125618955));
#59393=CARTESIAN_POINT('Ctrl Pts',(2.21115211847872,1.,-3.31764044024231));
#59394=CARTESIAN_POINT('Ctrl Pts',(2.20508863150608,1.,-3.3130742460895));
#59395=CARTESIAN_POINT('Ctrl Pts',(2.19906078949924,1.,-3.30848134694597));
#59396=CARTESIAN_POINT('Ctrl Pts',(2.19306710376112,1.,-3.30385816281831));
#59397=CARTESIAN_POINT('Ctrl Pts',(2.18710556500325,1.,-3.29920022557635));
#59398=CARTESIAN_POINT('Ctrl Pts',(2.18117455557062,1.,-3.29450361500484));
#59399=CARTESIAN_POINT('Ctrl Pts',(2.17527380048422,1.,-3.28976645712566));
#59400=CARTESIAN_POINT('Ctrl Pts',(2.16940517773459,1.,-3.2849901997973));
#59401=CARTESIAN_POINT('Ctrl Pts',(2.16357391934434,1.,-3.28018150841414));
#59402=CARTESIAN_POINT('Ctrl Pts',(2.15778690038359,1.,-3.27534954469206));
#59403=CARTESIAN_POINT('Ctrl Pts',(2.15205043199818,1.,-3.27050245897244));
#59404=CARTESIAN_POINT('Ctrl Pts',(2.14636805295663,1.,-3.26564388189764));
#59405=CARTESIAN_POINT('Ctrl Pts',(2.14073870754257,1.,-3.26077002641868));
#59406=CARTESIAN_POINT('Ctrl Pts',(2.13515375878786,1.,-3.25586495065027));
#59407=CARTESIAN_POINT('Ctrl Pts',(2.1296002839681,1.,-3.25090574493994));
#59408=CARTESIAN_POINT('Ctrl Pts',(2.12406646410943,1.,-3.24587102613347));
#59409=CARTESIAN_POINT('Ctrl Pts',(2.11854673326972,1.,-3.24074905517282));
#59410=CARTESIAN_POINT('Ctrl Pts',(2.11304604021784,1.,-3.23554444767115));
#59411=CARTESIAN_POINT('Ctrl Pts',(2.1075869964248,1.,-3.23028945793334));
#59412=CARTESIAN_POINT('Ctrl Pts',(2.10220384298533,1.,-3.22503437553496));
#59413=CARTESIAN_POINT('Ctrl Pts',(2.09692958434933,1.,-3.21982707347067));
#59414=CARTESIAN_POINT('Ctrl Pts',(2.0917841946046,1.,-3.2146942960168));
#59415=CARTESIAN_POINT('Ctrl Pts',(2.08676465517435,1.,-3.20962575845433));
#59416=CARTESIAN_POINT('Ctrl Pts',(2.08182850370816,1.,-3.20454818630635));
#59417=CARTESIAN_POINT('Ctrl Pts',(2.0769044187063,1.,-3.19934132835879));
#59418=CARTESIAN_POINT('Ctrl Pts',(2.07192253497765,1.,-3.19388465568113));
#59419=CARTESIAN_POINT('Ctrl Pts',(2.06684062744065,1.,-3.18809755562297));
#59420=CARTESIAN_POINT('Ctrl Pts',(2.06166849827143,1.,-3.18197692964677));
#59421=CARTESIAN_POINT('Ctrl Pts',(2.05650186773279,1.,-3.17564906975592));
#59422=CARTESIAN_POINT('Ctrl Pts',(2.05151770247452,1.,-3.16936341689859));
#59423=CARTESIAN_POINT('Ctrl Pts',(2.0469333124766,1.,-3.16343165059235));
#59424=CARTESIAN_POINT('Ctrl Pts',(2.04297406404132,1.,-3.15817983946525));
#59425=CARTESIAN_POINT('Ctrl Pts',(2.03984073791432,1.,-3.1538999167466));
#59426=CARTESIAN_POINT('Ctrl Pts',(2.03783225496023,1.,-3.15102344775396));
#59427=CARTESIAN_POINT('Ctrl Pts',(2.03693188810614,1.,-3.14959882629936));
#59428=CARTESIAN_POINT('Ctrl Pts',(2.03663974554941,1.,-3.14901193669147));
#59429=CARTESIAN_POINT('Ctrl Pts',(2.03659701539175,1.,-3.1488193908823));
#59430=CARTESIAN_POINT('Ctrl Pts',(2.03660101169564,1.,-3.14877060440425));
#59431=CARTESIAN_POINT('',(2.40675750623143,0.,-3.44202241512147));
#59432=CARTESIAN_POINT('Ctrl Pts',(2.36523532225181,-1.,-2.91001063062876));
#59433=CARTESIAN_POINT('Ctrl Pts',(2.36523532225181,1.,-2.91001063062876));
#59434=CARTESIAN_POINT('Ctrl Pts',(2.36524348105112,-1.,-2.90992398626211));
#59435=CARTESIAN_POINT('Ctrl Pts',(2.36524348105112,1.,-2.90992398626211));
#59436=CARTESIAN_POINT('Ctrl Pts',(2.36535052956938,-1.,-2.90989022548032));
#59437=CARTESIAN_POINT('Ctrl Pts',(2.36535052956938,1.,-2.90989022548032));
#59438=CARTESIAN_POINT('Ctrl Pts',(2.36578327194741,-1.,-2.91025813830041));
#59439=CARTESIAN_POINT('Ctrl Pts',(2.36578327194741,1.,-2.91025813830041));
#59440=CARTESIAN_POINT('Ctrl Pts',(2.36690501170627,-1.,-2.9115863784204));
#59441=CARTESIAN_POINT('Ctrl Pts',(2.36690501170627,1.,-2.9115863784204));
#59442=CARTESIAN_POINT('Ctrl Pts',(2.36919161373173,-1.,-2.9146124988314));
#59443=CARTESIAN_POINT('Ctrl Pts',(2.36919161373173,1.,-2.9146124988314));
#59444=CARTESIAN_POINT('Ctrl Pts',(2.37229381109821,-1.,-2.91891503791411));
#59445=CARTESIAN_POINT('Ctrl Pts',(2.37229381109821,1.,-2.91891503791411));
#59446=CARTESIAN_POINT('Ctrl Pts',(2.3760651052403,-1.,-2.92430340582608));
#59447=CARTESIAN_POINT('Ctrl Pts',(2.3760651052403,1.,-2.92430340582608));
#59448=CARTESIAN_POINT('Ctrl Pts',(2.38028989582073,-1.,-2.93049643640206));
#59449=CARTESIAN_POINT('Ctrl Pts',(2.38028989582073,1.,-2.93049643640206));
#59450=CARTESIAN_POINT('Ctrl Pts',(2.38472771516311,-1.,-2.93717903280391));
#59451=CARTESIAN_POINT('Ctrl Pts',(2.38472771516311,1.,-2.93717903280391));
#59452=CARTESIAN_POINT('Ctrl Pts',(2.38914929090759,-1.,-2.94404820669076));
#59453=CARTESIAN_POINT('Ctrl Pts',(2.38914929090759,1.,-2.94404820669076));
#59454=CARTESIAN_POINT('Ctrl Pts',(2.39337207631667,-1.,-2.95085857128439));
#59455=CARTESIAN_POINT('Ctrl Pts',(2.39337207631667,1.,-2.95085857128439));
#59456=CARTESIAN_POINT('Ctrl Pts',(2.39730553974516,-1.,-2.95748006482942));
#59457=CARTESIAN_POINT('Ctrl Pts',(2.39730553974516,1.,-2.95748006482942));
#59458=CARTESIAN_POINT('Ctrl Pts',(2.4009556571164,-1.,-2.96390432240312));
#59459=CARTESIAN_POINT('Ctrl Pts',(2.4009556571164,1.,-2.96390432240312));
#59460=CARTESIAN_POINT('Ctrl Pts',(2.40438604734919,-1.,-2.9701964131236));
#59461=CARTESIAN_POINT('Ctrl Pts',(2.40438604734919,1.,-2.9701964131236));
#59462=CARTESIAN_POINT('Ctrl Pts',(2.40768975073713,-1.,-2.97646002822422));
#59463=CARTESIAN_POINT('Ctrl Pts',(2.40768975073713,1.,-2.97646002822422));
#59464=CARTESIAN_POINT('Ctrl Pts',(2.41095909342571,-1.,-2.98280015815107));
#59465=CARTESIAN_POINT('Ctrl Pts',(2.41095909342571,1.,-2.98280015815107));
#59466=CARTESIAN_POINT('Ctrl Pts',(2.41425064199586,-1.,-2.98927983005796));
#59467=CARTESIAN_POINT('Ctrl Pts',(2.41425064199586,1.,-2.98927983005796));
#59468=CARTESIAN_POINT('Ctrl Pts',(2.41757324500514,-1.,-2.99590509293503));
#59469=CARTESIAN_POINT('Ctrl Pts',(2.41757324500514,1.,-2.99590509293503));
#59470=CARTESIAN_POINT('Ctrl Pts',(2.42090763946779,-1.,-3.00264868585996));
#59471=CARTESIAN_POINT('Ctrl Pts',(2.42090763946779,1.,-3.00264868585996));
#59472=CARTESIAN_POINT('Ctrl Pts',(2.42421849439613,-1.,-3.00946442616659));
#59473=CARTESIAN_POINT('Ctrl Pts',(2.42421849439613,1.,-3.00946442616659));
#59474=CARTESIAN_POINT('Ctrl Pts',(2.42746856264168,-1.,-3.01630420830504));
#59475=CARTESIAN_POINT('Ctrl Pts',(2.42746856264168,1.,-3.01630420830504));
#59476=CARTESIAN_POINT('Ctrl Pts',(2.43063415586637,-1.,-3.02313656036004));
#59477=CARTESIAN_POINT('Ctrl Pts',(2.43063415586637,1.,-3.02313656036004));
#59478=CARTESIAN_POINT('Ctrl Pts',(2.43371241361488,-1.,-3.02995534946978));
#59479=CARTESIAN_POINT('Ctrl Pts',(2.43371241361488,1.,-3.02995534946978));
#59480=CARTESIAN_POINT('Ctrl Pts',(2.43671278042414,-1.,-3.03676949672822));
#59481=CARTESIAN_POINT('Ctrl Pts',(2.43671278042414,1.,-3.03676949672822));
#59482=CARTESIAN_POINT('Ctrl Pts',(2.43965194061857,-1.,-3.04359685040555));
#59483=CARTESIAN_POINT('Ctrl Pts',(2.43965194061857,1.,-3.04359685040555));
#59484=CARTESIAN_POINT('Ctrl Pts',(2.44254768923105,-1.,-3.05045678021504));
#59485=CARTESIAN_POINT('Ctrl Pts',(2.44254768923105,1.,-3.05045678021504));
#59486=CARTESIAN_POINT('Ctrl Pts',(2.44541251892556,-1.,-3.05736242671506));
#59487=CARTESIAN_POINT('Ctrl Pts',(2.44541251892556,1.,-3.05736242671506));
#59488=CARTESIAN_POINT('Ctrl Pts',(2.44824970516543,-1.,-3.06431596421405));
#59489=CARTESIAN_POINT('Ctrl Pts',(2.44824970516543,1.,-3.06431596421405));
#59490=CARTESIAN_POINT('Ctrl Pts',(2.45105688854422,-1.,-3.07131290521297));
#59491=CARTESIAN_POINT('Ctrl Pts',(2.45105688854422,1.,-3.07131290521297));
#59492=CARTESIAN_POINT('Ctrl Pts',(2.4538282678779,-1.,-3.07834472886139));
#59493=CARTESIAN_POINT('Ctrl Pts',(2.4538282678779,1.,-3.07834472886139));
#59494=CARTESIAN_POINT('Ctrl Pts',(2.45655725437039,-1.,-3.08540206545315));
#59495=CARTESIAN_POINT('Ctrl Pts',(2.45655725437039,1.,-3.08540206545315));
#59496=CARTESIAN_POINT('Ctrl Pts',(2.4592391256388,-1.,-3.09247787931887));
#59497=CARTESIAN_POINT('Ctrl Pts',(2.4592391256388,1.,-3.09247787931887));
#59498=CARTESIAN_POINT('Ctrl Pts',(2.46187308501884,-1.,-3.09956993697052));
#59499=CARTESIAN_POINT('Ctrl Pts',(2.46187308501884,1.,-3.09956993697052));
#59500=CARTESIAN_POINT('Ctrl Pts',(2.46446082979646,-1.,-3.1066790790198));
#59501=CARTESIAN_POINT('Ctrl Pts',(2.46446082979646,1.,-3.1066790790198));
#59502=CARTESIAN_POINT('Ctrl Pts',(2.46700558843506,-1.,-3.11380805536122));
#59503=CARTESIAN_POINT('Ctrl Pts',(2.46700558843506,1.,-3.11380805536122));
#59504=CARTESIAN_POINT('Ctrl Pts',(2.46951098947469,-1.,-3.12096015766983));
#59505=CARTESIAN_POINT('Ctrl Pts',(2.46951098947469,1.,-3.12096015766983));
#59506=CARTESIAN_POINT('Ctrl Pts',(2.47197997765871,-1.,-3.12813790805952));
#59507=CARTESIAN_POINT('Ctrl Pts',(2.47197997765871,1.,-3.12813790805952));
#59508=CARTESIAN_POINT('Ctrl Pts',(2.47441378371932,-1.,-3.13534181229295));
#59509=CARTESIAN_POINT('Ctrl Pts',(2.47441378371932,1.,-3.13534181229295));
#59510=CARTESIAN_POINT('Ctrl Pts',(2.47681245356109,-1.,-3.1425709954655));
#59511=CARTESIAN_POINT('Ctrl Pts',(2.47681245356109,1.,-3.1425709954655));
#59512=CARTESIAN_POINT('Ctrl Pts',(2.47917529057029,-1.,-3.14982373241352));
#59513=CARTESIAN_POINT('Ctrl Pts',(2.47917529057029,1.,-3.14982373241352));
#59514=CARTESIAN_POINT('Ctrl Pts',(2.48150133566571,-1.,-3.15709802322739));
#59515=CARTESIAN_POINT('Ctrl Pts',(2.48150133566571,1.,-3.15709802322739));
#59516=CARTESIAN_POINT('Ctrl Pts',(2.48378981792725,-1.,-3.16439213290161));
#59517=CARTESIAN_POINT('Ctrl Pts',(2.48378981792725,1.,-3.16439213290161));
#59518=CARTESIAN_POINT('Ctrl Pts',(2.48604065348587,-1.,-3.17170518863313));
#59519=CARTESIAN_POINT('Ctrl Pts',(2.48604065348587,1.,-3.17170518863313));
#59520=CARTESIAN_POINT('Ctrl Pts',(2.48825428288201,-1.,-3.17903698136622));
#59521=CARTESIAN_POINT('Ctrl Pts',(2.48825428288201,1.,-3.17903698136622));
#59522=CARTESIAN_POINT('Ctrl Pts',(2.49043146334059,-1.,-3.18638771282266));
#59523=CARTESIAN_POINT('Ctrl Pts',(2.49043146334059,1.,-3.18638771282266));
#59524=CARTESIAN_POINT('Ctrl Pts',(2.49257307239848,-1.,-3.19375775555798));
#59525=CARTESIAN_POINT('Ctrl Pts',(2.49257307239848,1.,-3.19375775555798));
#59526=CARTESIAN_POINT('Ctrl Pts',(2.49467992057755,-1.,-3.20114742397588));
#59527=CARTESIAN_POINT('Ctrl Pts',(2.49467992057755,1.,-3.20114742397588));
#59528=CARTESIAN_POINT('Ctrl Pts',(2.4967525264737,-1.,-3.20855669849836));
#59529=CARTESIAN_POINT('Ctrl Pts',(2.4967525264737,1.,-3.20855669849836));
#59530=CARTESIAN_POINT('Ctrl Pts',(2.4987911459939,-1.,-3.21598526261286));
#59531=CARTESIAN_POINT('Ctrl Pts',(2.4987911459939,1.,-3.21598526261286));
#59532=CARTESIAN_POINT('Ctrl Pts',(2.50079587201957,-1.,-3.22343262620503));
#59533=CARTESIAN_POINT('Ctrl Pts',(2.50079587201957,1.,-3.22343262620503));
#59534=CARTESIAN_POINT('Ctrl Pts',(2.50276671338111,-1.,-3.23089822320646));
#59535=CARTESIAN_POINT('Ctrl Pts',(2.50276671338111,1.,-3.23089822320646));
#59536=CARTESIAN_POINT('Ctrl Pts',(2.5047036758003,-1.,-3.23838151080319));
#59537=CARTESIAN_POINT('Ctrl Pts',(2.5047036758003,1.,-3.23838151080319));
#59538=CARTESIAN_POINT('Ctrl Pts',(2.506606859405,-1.,-3.24588208983849));
#59539=CARTESIAN_POINT('Ctrl Pts',(2.506606859405,1.,-3.24588208983849));
#59540=CARTESIAN_POINT('Ctrl Pts',(2.50847647070723,-1.,-3.25339971460982));
#59541=CARTESIAN_POINT('Ctrl Pts',(2.50847647070723,1.,-3.25339971460982));
#59542=CARTESIAN_POINT('Ctrl Pts',(2.51031277813486,-1.,-3.26093423001434));
#59543=CARTESIAN_POINT('Ctrl Pts',(2.51031277813486,1.,-3.26093423001434));
#59544=CARTESIAN_POINT('Ctrl Pts',(2.51211608411423,-1.,-3.26848552888116));
#59545=CARTESIAN_POINT('Ctrl Pts',(2.51211608411423,1.,-3.26848552888116));
#59546=CARTESIAN_POINT('Ctrl Pts',(2.513886692704,-1.,-3.27605350473142));
#59547=CARTESIAN_POINT('Ctrl Pts',(2.513886692704,1.,-3.27605350473142));
#59548=CARTESIAN_POINT('Ctrl Pts',(2.51562487464514,-1.,-3.28363799702982));
#59549=CARTESIAN_POINT('Ctrl Pts',(2.51562487464514,1.,-3.28363799702982));
#59550=CARTESIAN_POINT('Ctrl Pts',(2.51733085123797,-1.,-3.2912387729927));
#59551=CARTESIAN_POINT('Ctrl Pts',(2.51733085123797,1.,-3.2912387729927));
#59552=CARTESIAN_POINT('Ctrl Pts',(2.51900480701068,-1.,-3.29885556388353));
#59553=CARTESIAN_POINT('Ctrl Pts',(2.51900480701068,1.,-3.29885556388353));
#59554=CARTESIAN_POINT('Ctrl Pts',(2.52064689568511,-1.,-3.30648808815443));
#59555=CARTESIAN_POINT('Ctrl Pts',(2.52064689568511,1.,-3.30648808815443));
#59556=CARTESIAN_POINT('Ctrl Pts',(2.52225724871313,-1.,-3.31413607874645));
#59557=CARTESIAN_POINT('Ctrl Pts',(2.52225724871313,1.,-3.31413607874645));
#59558=CARTESIAN_POINT('Ctrl Pts',(2.5238359839626,-1.,-3.32179931078699));
#59559=CARTESIAN_POINT('Ctrl Pts',(2.5238359839626,1.,-3.32179931078699));
#59560=CARTESIAN_POINT('Ctrl Pts',(2.52538321164634,-1.,-3.32947762187533));
#59561=CARTESIAN_POINT('Ctrl Pts',(2.52538321164634,1.,-3.32947762187533));
#59562=CARTESIAN_POINT('Ctrl Pts',(2.52689902690158,-1.,-3.33717089999103));
#59563=CARTESIAN_POINT('Ctrl Pts',(2.52689902690158,1.,-3.33717089999103));
#59564=CARTESIAN_POINT('Ctrl Pts',(2.52808660915689,-1.,-3.34333744115511));
#59565=CARTESIAN_POINT('Ctrl Pts',(2.52808660915689,1.,-3.34333744115511));
#59566=CARTESIAN_POINT('Ctrl Pts',(2.52896321610703,-1.,-3.34796903576663));
#59567=CARTESIAN_POINT('Ctrl Pts',(2.52896321610703,1.,-3.34796903576663));
#59568=CARTESIAN_POINT('Ctrl Pts',(2.5295413654909,-1.,-3.35105973714072));
#59569=CARTESIAN_POINT('Ctrl Pts',(2.5295413654909,1.,-3.35105973714072));
#59570=CARTESIAN_POINT('Ctrl Pts',(2.52982887637028,-1.,-3.35260583073571));
#59571=CARTESIAN_POINT('Ctrl Pts',(2.52982887637028,1.,-3.35260583073571));
#59572=CARTESIAN_POINT('',(2.36531447826073,1.,-2.90994629141676));
#59573=CARTESIAN_POINT('Ctrl Pts',(2.36531447826073,-1.,-2.90994629141676));
#59574=CARTESIAN_POINT('Ctrl Pts',(2.36531447826073,-0.666666666666667,
-2.90994629141676));
#59575=CARTESIAN_POINT('Ctrl Pts',(2.36531447826073,-0.333333333333333,
-2.90994629141676));
#59576=CARTESIAN_POINT('Ctrl Pts',(2.36531447826073,0.333333333333333,-2.90994629141676));
#59577=CARTESIAN_POINT('Ctrl Pts',(2.36531447826074,0.666666666666667,-2.90994629141676));
#59578=CARTESIAN_POINT('Ctrl Pts',(2.36531447826074,1.,-2.90994629141676));
#59579=CARTESIAN_POINT('',(2.52982887637028,1.,-3.35260583073571));
#59580=CARTESIAN_POINT('',(2.52982887637028,0.,-3.35260583073571));
#59581=CARTESIAN_POINT('Ctrl Pts',(2.36531447826073,1.,-2.90994629141676));
#59582=CARTESIAN_POINT('Ctrl Pts',(2.36536211188453,1.,-2.90995756655606));
#59583=CARTESIAN_POINT('Ctrl Pts',(2.36553202948613,1.,-2.91005770527719));
#59584=CARTESIAN_POINT('Ctrl Pts',(2.36599991765749,1.,-2.91051690822156));
#59585=CARTESIAN_POINT('Ctrl Pts',(2.36707658451664,1.,-2.91181344022548));
#59586=CARTESIAN_POINT('Ctrl Pts',(2.36919161373173,1.,-2.9146124988314));
#59587=CARTESIAN_POINT('Ctrl Pts',(2.37229381109821,1.,-2.91891503791411));
#59588=CARTESIAN_POINT('Ctrl Pts',(2.3760651052403,1.,-2.92430340582608));
#59589=CARTESIAN_POINT('Ctrl Pts',(2.38028989582073,1.,-2.93049643640206));
#59590=CARTESIAN_POINT('Ctrl Pts',(2.38472771516311,1.,-2.93717903280391));
#59591=CARTESIAN_POINT('Ctrl Pts',(2.38914929090759,1.,-2.94404820669076));
#59592=CARTESIAN_POINT('Ctrl Pts',(2.39337207631667,1.,-2.95085857128439));
#59593=CARTESIAN_POINT('Ctrl Pts',(2.39730553974516,1.,-2.95748006482942));
#59594=CARTESIAN_POINT('Ctrl Pts',(2.4009556571164,1.,-2.96390432240312));
#59595=CARTESIAN_POINT('Ctrl Pts',(2.40438604734919,1.,-2.9701964131236));
#59596=CARTESIAN_POINT('Ctrl Pts',(2.40768975073713,1.,-2.97646002822422));
#59597=CARTESIAN_POINT('Ctrl Pts',(2.41095909342571,1.,-2.98280015815107));
#59598=CARTESIAN_POINT('Ctrl Pts',(2.41425064199586,1.,-2.98927983005796));
#59599=CARTESIAN_POINT('Ctrl Pts',(2.41757324500514,1.,-2.99590509293503));
#59600=CARTESIAN_POINT('Ctrl Pts',(2.42090763946779,1.,-3.00264868585996));
#59601=CARTESIAN_POINT('Ctrl Pts',(2.42421849439613,1.,-3.00946442616659));
#59602=CARTESIAN_POINT('Ctrl Pts',(2.42746856264168,1.,-3.01630420830504));
#59603=CARTESIAN_POINT('Ctrl Pts',(2.43063415586637,1.,-3.02313656036004));
#59604=CARTESIAN_POINT('Ctrl Pts',(2.43371241361488,1.,-3.02995534946978));
#59605=CARTESIAN_POINT('Ctrl Pts',(2.43671278042414,1.,-3.03676949672822));
#59606=CARTESIAN_POINT('Ctrl Pts',(2.43965194061857,1.,-3.04359685040555));
#59607=CARTESIAN_POINT('Ctrl Pts',(2.44254768923105,1.,-3.05045678021504));
#59608=CARTESIAN_POINT('Ctrl Pts',(2.44541251892556,1.,-3.05736242671506));
#59609=CARTESIAN_POINT('Ctrl Pts',(2.44824970516543,1.,-3.06431596421405));
#59610=CARTESIAN_POINT('Ctrl Pts',(2.45105688854422,1.,-3.07131290521297));
#59611=CARTESIAN_POINT('Ctrl Pts',(2.4538282678779,1.,-3.07834472886139));
#59612=CARTESIAN_POINT('Ctrl Pts',(2.45655725437039,1.,-3.08540206545315));
#59613=CARTESIAN_POINT('Ctrl Pts',(2.4592391256388,1.,-3.09247787931887));
#59614=CARTESIAN_POINT('Ctrl Pts',(2.46187308501884,1.,-3.09956993697052));
#59615=CARTESIAN_POINT('Ctrl Pts',(2.46446082979646,1.,-3.1066790790198));
#59616=CARTESIAN_POINT('Ctrl Pts',(2.46700558843506,1.,-3.11380805536122));
#59617=CARTESIAN_POINT('Ctrl Pts',(2.46951098947469,1.,-3.12096015766983));
#59618=CARTESIAN_POINT('Ctrl Pts',(2.47197997765871,1.,-3.12813790805952));
#59619=CARTESIAN_POINT('Ctrl Pts',(2.47441378371932,1.,-3.13534181229295));
#59620=CARTESIAN_POINT('Ctrl Pts',(2.47681245356109,1.,-3.1425709954655));
#59621=CARTESIAN_POINT('Ctrl Pts',(2.47917529057029,1.,-3.14982373241352));
#59622=CARTESIAN_POINT('Ctrl Pts',(2.48150133566571,1.,-3.15709802322739));
#59623=CARTESIAN_POINT('Ctrl Pts',(2.48378981792725,1.,-3.16439213290161));
#59624=CARTESIAN_POINT('Ctrl Pts',(2.48604065348587,1.,-3.17170518863313));
#59625=CARTESIAN_POINT('Ctrl Pts',(2.48825428288201,1.,-3.17903698136622));
#59626=CARTESIAN_POINT('Ctrl Pts',(2.49043146334059,1.,-3.18638771282266));
#59627=CARTESIAN_POINT('Ctrl Pts',(2.49257307239848,1.,-3.19375775555798));
#59628=CARTESIAN_POINT('Ctrl Pts',(2.49467992057755,1.,-3.20114742397588));
#59629=CARTESIAN_POINT('Ctrl Pts',(2.4967525264737,1.,-3.20855669849836));
#59630=CARTESIAN_POINT('Ctrl Pts',(2.4987911459939,1.,-3.21598526261286));
#59631=CARTESIAN_POINT('Ctrl Pts',(2.50079587201957,1.,-3.22343262620503));
#59632=CARTESIAN_POINT('Ctrl Pts',(2.50276671338111,1.,-3.23089822320646));
#59633=CARTESIAN_POINT('Ctrl Pts',(2.5047036758003,1.,-3.23838151080319));
#59634=CARTESIAN_POINT('Ctrl Pts',(2.506606859405,1.,-3.24588208983849));
#59635=CARTESIAN_POINT('Ctrl Pts',(2.50847647070723,1.,-3.25339971460982));
#59636=CARTESIAN_POINT('Ctrl Pts',(2.51031277813486,1.,-3.26093423001434));
#59637=CARTESIAN_POINT('Ctrl Pts',(2.51211608411423,1.,-3.26848552888116));
#59638=CARTESIAN_POINT('Ctrl Pts',(2.513886692704,1.,-3.27605350473142));
#59639=CARTESIAN_POINT('Ctrl Pts',(2.51562487464514,1.,-3.28363799702982));
#59640=CARTESIAN_POINT('Ctrl Pts',(2.51733085123797,1.,-3.2912387729927));
#59641=CARTESIAN_POINT('Ctrl Pts',(2.51900480701068,1.,-3.29885556388353));
#59642=CARTESIAN_POINT('Ctrl Pts',(2.52064689568511,1.,-3.30648808815443));
#59643=CARTESIAN_POINT('Ctrl Pts',(2.52225724871313,1.,-3.31413607874645));
#59644=CARTESIAN_POINT('Ctrl Pts',(2.5238359839626,1.,-3.32179931078699));
#59645=CARTESIAN_POINT('Ctrl Pts',(2.52538321164634,1.,-3.32947762187533));
#59646=CARTESIAN_POINT('Ctrl Pts',(2.52689902690158,1.,-3.33717089999103));
#59647=CARTESIAN_POINT('Ctrl Pts',(2.52808660915689,1.,-3.34333744115511));
#59648=CARTESIAN_POINT('Ctrl Pts',(2.52896321610703,1.,-3.34796903576663));
#59649=CARTESIAN_POINT('Ctrl Pts',(2.5295413654909,1.,-3.35105973714072));
#59650=CARTESIAN_POINT('Ctrl Pts',(2.52982887637028,1.,-3.35260583073571));
#59651=CARTESIAN_POINT('Origin',(2.52982887637028,0.,-3.35260583073571));
#59652=CARTESIAN_POINT('',(2.40675750623143,1.,-3.44202241512147));
#59653=CARTESIAN_POINT('Origin',(0.,0.,0.));
#59654=CARTESIAN_POINT('',(2.50410331873042,1.,-2.79140942341378));
#59655=CARTESIAN_POINT('Origin',(0.,1.,0.));
#59656=CARTESIAN_POINT('Ctrl Pts',(2.50410331873042,1.,-2.79140942341378));
#59657=CARTESIAN_POINT('Ctrl Pts',(2.50410331873042,0.666666666666667,-2.79140942341378));
#59658=CARTESIAN_POINT('Ctrl Pts',(2.50410331873042,0.333333333333333,-2.79140942341378));
#59659=CARTESIAN_POINT('Ctrl Pts',(2.50410331873042,-0.333333333333333,
-2.79140942341378));
#59660=CARTESIAN_POINT('Ctrl Pts',(2.50410331873042,-0.666666666666667,
-2.79140942341378));
#59661=CARTESIAN_POINT('Ctrl Pts',(2.50410331873042,-1.,-2.79140942341378));
#59662=CARTESIAN_POINT('Ctrl Pts',(2.91557726271063,-1.,-3.02314558451372));
#59663=CARTESIAN_POINT('Ctrl Pts',(2.91557726271063,1.,-3.02314558451372));
#59664=CARTESIAN_POINT('Ctrl Pts',(2.91409518070707,-1.,-3.02261975104912));
#59665=CARTESIAN_POINT('Ctrl Pts',(2.91409518070707,1.,-3.02261975104912));
#59666=CARTESIAN_POINT('Ctrl Pts',(2.91113297349052,-1.,-3.02156522743299));
#59667=CARTESIAN_POINT('Ctrl Pts',(2.91113297349052,1.,-3.02156522743299));
#59668=CARTESIAN_POINT('Ctrl Pts',(2.90669553303902,-1.,-3.01997487194926));
#59669=CARTESIAN_POINT('Ctrl Pts',(2.90669553303902,1.,-3.01997487194926));
#59670=CARTESIAN_POINT('Ctrl Pts',(2.90079069102661,-1.,-3.01783725123646));
#59671=CARTESIAN_POINT('Ctrl Pts',(2.90079069102661,1.,-3.01783725123646));
#59672=CARTESIAN_POINT('Ctrl Pts',(2.8934292556764,-1.,-3.01513660433291));
#59673=CARTESIAN_POINT('Ctrl Pts',(2.8934292556764,1.,-3.01513660433291));
#59674=CARTESIAN_POINT('Ctrl Pts',(2.88608751706796,-1.,-3.01240727309568));
#59675=CARTESIAN_POINT('Ctrl Pts',(2.88608751706796,1.,-3.01240727309568));
#59676=CARTESIAN_POINT('Ctrl Pts',(2.87876560072799,-1.,-3.0096491810855));
#59677=CARTESIAN_POINT('Ctrl Pts',(2.87876560072799,1.,-3.0096491810855));
#59678=CARTESIAN_POINT('Ctrl Pts',(2.87146368430104,-1.,-3.00686224485374));
#59679=CARTESIAN_POINT('Ctrl Pts',(2.87146368430104,1.,-3.00686224485374));
#59680=CARTESIAN_POINT('Ctrl Pts',(2.86418200833065,-1.,-3.00404638316245));
#59681=CARTESIAN_POINT('Ctrl Pts',(2.86418200833065,1.,-3.00404638316245));
#59682=CARTESIAN_POINT('Ctrl Pts',(2.85692085715129,-1.,-3.0012015079552));
#59683=CARTESIAN_POINT('Ctrl Pts',(2.85692085715129,1.,-3.0012015079552));
#59684=CARTESIAN_POINT('Ctrl Pts',(2.84968053289104,-1.,-2.99832751144566));
#59685=CARTESIAN_POINT('Ctrl Pts',(2.84968053289104,1.,-2.99832751144566));
#59686=CARTESIAN_POINT('Ctrl Pts',(2.84246132984334,-1.,-2.995424253416));
#59687=CARTESIAN_POINT('Ctrl Pts',(2.84246132984334,1.,-2.995424253416));
#59688=CARTESIAN_POINT('Ctrl Pts',(2.83526351254383,-1.,-2.99249155170479));
#59689=CARTESIAN_POINT('Ctrl Pts',(2.83526351254383,1.,-2.99249155170479));
#59690=CARTESIAN_POINT('Ctrl Pts',(2.82808728190402,-1.,-2.98952916401699));
#59691=CARTESIAN_POINT('Ctrl Pts',(2.82808728190402,1.,-2.98952916401699));
#59692=CARTESIAN_POINT('Ctrl Pts',(2.82093279065704,-1.,-2.98653680669434));
#59693=CARTESIAN_POINT('Ctrl Pts',(2.82093279065704,1.,-2.98653680669434));
#59694=CARTESIAN_POINT('Ctrl Pts',(2.81380019196454,-1.,-2.9835141977994));
#59695=CARTESIAN_POINT('Ctrl Pts',(2.81380019196454,1.,-2.9835141977994));
#59696=CARTESIAN_POINT('Ctrl Pts',(2.80668968101162,-1.,-2.98046109647299));
#59697=CARTESIAN_POINT('Ctrl Pts',(2.80668968101162,1.,-2.98046109647299));
#59698=CARTESIAN_POINT('Ctrl Pts',(2.79960153278186,-1.,-2.97737733718242));
#59699=CARTESIAN_POINT('Ctrl Pts',(2.79960153278186,1.,-2.97737733718242));
#59700=CARTESIAN_POINT('Ctrl Pts',(2.79253615718147,-1.,-2.97426288347475));
#59701=CARTESIAN_POINT('Ctrl Pts',(2.79253615718147,1.,-2.97426288347475));
#59702=CARTESIAN_POINT('Ctrl Pts',(2.78549409123657,-1.,-2.97111781461349));
#59703=CARTESIAN_POINT('Ctrl Pts',(2.78549409123657,1.,-2.97111781461349));
#59704=CARTESIAN_POINT('Ctrl Pts',(2.77847589542767,-1.,-2.9679422104295));
#59705=CARTESIAN_POINT('Ctrl Pts',(2.77847589542767,1.,-2.9679422104295));
#59706=CARTESIAN_POINT('Ctrl Pts',(2.77148206836464,-1.,-2.96473605585548));
#59707=CARTESIAN_POINT('Ctrl Pts',(2.77148206836464,1.,-2.96473605585548));
#59708=CARTESIAN_POINT('Ctrl Pts',(2.76451296269571,-1.,-2.96149914764832));
#59709=CARTESIAN_POINT('Ctrl Pts',(2.76451296269571,1.,-2.96149914764832));
#59710=CARTESIAN_POINT('Ctrl Pts',(2.75756867888393,-1.,-2.9582309766594));
#59711=CARTESIAN_POINT('Ctrl Pts',(2.75756867888393,1.,-2.9582309766594));
#59712=CARTESIAN_POINT('Ctrl Pts',(2.75064903318996,-1.,-2.95493069316211));
#59713=CARTESIAN_POINT('Ctrl Pts',(2.75064903318996,1.,-2.95493069316211));
#59714=CARTESIAN_POINT('Ctrl Pts',(2.7437537949221,-1.,-2.95159737214305));
#59715=CARTESIAN_POINT('Ctrl Pts',(2.7437537949221,1.,-2.95159737214305));
#59716=CARTESIAN_POINT('Ctrl Pts',(2.73688288329825,-1.,-2.94823023414381));
#59717=CARTESIAN_POINT('Ctrl Pts',(2.73688288329825,1.,-2.94823023414381));
#59718=CARTESIAN_POINT('Ctrl Pts',(2.73003657371613,-1.,-2.94482887675139));
#59719=CARTESIAN_POINT('Ctrl Pts',(2.73003657371613,1.,-2.94482887675139));
#59720=CARTESIAN_POINT('Ctrl Pts',(2.72321571511322,-1.,-2.94139351933882));
#59721=CARTESIAN_POINT('Ctrl Pts',(2.72321571511322,1.,-2.94139351933882));
#59722=CARTESIAN_POINT('Ctrl Pts',(2.71642190053575,-1.,-2.93792519474955));
#59723=CARTESIAN_POINT('Ctrl Pts',(2.71642190053575,1.,-2.93792519474955));
#59724=CARTESIAN_POINT('Ctrl Pts',(2.70965695523776,-1.,-2.93442516311168));
#59725=CARTESIAN_POINT('Ctrl Pts',(2.70965695523776,1.,-2.93442516311168));
#59726=CARTESIAN_POINT('Ctrl Pts',(2.70292247416881,-1.,-2.93089438233746));
#59727=CARTESIAN_POINT('Ctrl Pts',(2.70292247416881,1.,-2.93089438233746));
#59728=CARTESIAN_POINT('Ctrl Pts',(2.69621932864302,-1.,-2.92733294395268));
#59729=CARTESIAN_POINT('Ctrl Pts',(2.69621932864302,1.,-2.92733294395268));
#59730=CARTESIAN_POINT('Ctrl Pts',(2.68954721165342,-1.,-2.92373955325876));
#59731=CARTESIAN_POINT('Ctrl Pts',(2.68954721165342,1.,-2.92373955325876));
#59732=CARTESIAN_POINT('Ctrl Pts',(2.68290409279689,-1.,-2.92011090722152));
#59733=CARTESIAN_POINT('Ctrl Pts',(2.68290409279689,1.,-2.92011090722152));
#59734=CARTESIAN_POINT('Ctrl Pts',(2.67628728855309,-1.,-2.91644290704281));
#59735=CARTESIAN_POINT('Ctrl Pts',(2.67628728855309,1.,-2.91644290704281));
#59736=CARTESIAN_POINT('Ctrl Pts',(2.66969458792627,-1.,-2.91273193382876));
#59737=CARTESIAN_POINT('Ctrl Pts',(2.66969458792627,1.,-2.91273193382876));
#59738=CARTESIAN_POINT('Ctrl Pts',(2.66312542616808,-1.,-2.90897617968921));
#59739=CARTESIAN_POINT('Ctrl Pts',(2.66312542616808,1.,-2.90897617968921));
#59740=CARTESIAN_POINT('Ctrl Pts',(2.65658188464287,-1.,-2.90517678087467));
#59741=CARTESIAN_POINT('Ctrl Pts',(2.65658188464287,1.,-2.90517678087467));
#59742=CARTESIAN_POINT('Ctrl Pts',(2.65007017365576,-1.,-2.90133950224879));
#59743=CARTESIAN_POINT('Ctrl Pts',(2.65007017365576,1.,-2.90133950224879));
#59744=CARTESIAN_POINT('Ctrl Pts',(2.64359851684146,-1.,-2.89747231723361));
#59745=CARTESIAN_POINT('Ctrl Pts',(2.64359851684146,1.,-2.89747231723361));
#59746=CARTESIAN_POINT('Ctrl Pts',(2.63717442263944,-1.,-2.89358228854557));
#59747=CARTESIAN_POINT('Ctrl Pts',(2.63717442263944,1.,-2.89358228854557));
#59748=CARTESIAN_POINT('Ctrl Pts',(2.63080195420771,-1.,-2.88967244854243));
#59749=CARTESIAN_POINT('Ctrl Pts',(2.63080195420771,1.,-2.88967244854243));
#59750=CARTESIAN_POINT('Ctrl Pts',(2.62447947640253,-1.,-2.88573922195049));
#59751=CARTESIAN_POINT('Ctrl Pts',(2.62447947640253,1.,-2.88573922195049));
#59752=CARTESIAN_POINT('Ctrl Pts',(2.61819596473087,-1.,-2.88176821427502));
#59753=CARTESIAN_POINT('Ctrl Pts',(2.61819596473087,1.,-2.88176821427502));
#59754=CARTESIAN_POINT('Ctrl Pts',(2.61193507170928,-1.,-2.87773881947885));
#59755=CARTESIAN_POINT('Ctrl Pts',(2.61193507170928,1.,-2.87773881947885));
#59756=CARTESIAN_POINT('Ctrl Pts',(2.6056817788128,-1.,-2.87363176656475));
#59757=CARTESIAN_POINT('Ctrl Pts',(2.6056817788128,1.,-2.87363176656475));
#59758=CARTESIAN_POINT('Ctrl Pts',(2.59942875223202,-1.,-2.86943633170712));
#59759=CARTESIAN_POINT('Ctrl Pts',(2.59942875223202,1.,-2.86943633170712));
#59760=CARTESIAN_POINT('Ctrl Pts',(2.59318160184921,-1.,-2.86515629953528));
#59761=CARTESIAN_POINT('Ctrl Pts',(2.59318160184921,1.,-2.86515629953528));
#59762=CARTESIAN_POINT('Ctrl Pts',(2.5869677064356,-1.,-2.86081999003668));
#59763=CARTESIAN_POINT('Ctrl Pts',(2.5869677064356,1.,-2.86081999003668));
#59764=CARTESIAN_POINT('Ctrl Pts',(2.58082875254407,-1.,-2.85647171715147));
#59765=CARTESIAN_POINT('Ctrl Pts',(2.58082875254407,1.,-2.85647171715147));
#59766=CARTESIAN_POINT('Ctrl Pts',(2.57480482727128,-1.,-2.85215360144483));
#59767=CARTESIAN_POINT('Ctrl Pts',(2.57480482727128,1.,-2.85215360144483));
#59768=CARTESIAN_POINT('Ctrl Pts',(2.56891984251743,-1.,-2.84788893329091));
#59769=CARTESIAN_POINT('Ctrl Pts',(2.56891984251743,1.,-2.84788893329091));
#59770=CARTESIAN_POINT('Ctrl Pts',(2.56316920798489,-1.,-2.84366802680211));
#59771=CARTESIAN_POINT('Ctrl Pts',(2.56316920798489,1.,-2.84366802680211));
#59772=CARTESIAN_POINT('Ctrl Pts',(2.55749952145165,-1.,-2.83942515220699));
#59773=CARTESIAN_POINT('Ctrl Pts',(2.55749952145165,1.,-2.83942515220699));
#59774=CARTESIAN_POINT('Ctrl Pts',(2.55182152806964,-1.,-2.83505269592412));
#59775=CARTESIAN_POINT('Ctrl Pts',(2.55182152806964,1.,-2.83505269592412));
#59776=CARTESIAN_POINT('Ctrl Pts',(2.54604736792542,-1.,-2.83044254225794));
#59777=CARTESIAN_POINT('Ctrl Pts',(2.54604736792542,1.,-2.83044254225794));
#59778=CARTESIAN_POINT('Ctrl Pts',(2.54012272520141,-1.,-2.82552167649157));
#59779=CARTESIAN_POINT('Ctrl Pts',(2.54012272520141,1.,-2.82552167649157));
#59780=CARTESIAN_POINT('Ctrl Pts',(2.53405679667463,-1.,-2.82028550483744));
#59781=CARTESIAN_POINT('Ctrl Pts',(2.53405679667463,1.,-2.82028550483744));
#59782=CARTESIAN_POINT('Ctrl Pts',(2.52796388055457,-1.,-2.8148437904867));
#59783=CARTESIAN_POINT('Ctrl Pts',(2.52796388055457,1.,-2.8148437904867));
#59784=CARTESIAN_POINT('Ctrl Pts',(2.52205778589922,-1.,-2.80941521967234));
#59785=CARTESIAN_POINT('Ctrl Pts',(2.52205778589922,1.,-2.80941521967234));
#59786=CARTESIAN_POINT('Ctrl Pts',(2.51660190466067,-1.,-2.80427363984939));
#59787=CARTESIAN_POINT('Ctrl Pts',(2.51660190466067,1.,-2.80427363984939));
#59788=CARTESIAN_POINT('Ctrl Pts',(2.51186983687947,-1.,-2.79970585014308));
#59789=CARTESIAN_POINT('Ctrl Pts',(2.51186983687947,1.,-2.79970585014308));
#59790=CARTESIAN_POINT('Ctrl Pts',(2.50810555977564,-1.,-2.7959687805717));
#59791=CARTESIAN_POINT('Ctrl Pts',(2.50810555977564,1.,-2.7959687805717));
#59792=CARTESIAN_POINT('Ctrl Pts',(2.50547439929077,-1.,-2.79323694088143));
#59793=CARTESIAN_POINT('Ctrl Pts',(2.50547439929077,1.,-2.79323694088143));
#59794=CARTESIAN_POINT('Ctrl Pts',(2.50433799076945,-1.,-2.79192122906739));
#59795=CARTESIAN_POINT('Ctrl Pts',(2.50433799076945,1.,-2.79192122906739));
#59796=CARTESIAN_POINT('Ctrl Pts',(2.50404230339032,-1.,-2.79143626022225));
#59797=CARTESIAN_POINT('Ctrl Pts',(2.50404230339032,1.,-2.79143626022225));
#59798=CARTESIAN_POINT('Ctrl Pts',(2.50409239460011,-1.,-2.79133581100044));
#59799=CARTESIAN_POINT('Ctrl Pts',(2.50409239460011,1.,-2.79133581100044));
#59800=CARTESIAN_POINT('Ctrl Pts',(2.50417924854921,-1.,-2.79134130681569));
#59801=CARTESIAN_POINT('Ctrl Pts',(2.50417924854921,1.,-2.79134130681569));
#59802=CARTESIAN_POINT('',(2.91557726271063,1.,-3.02314558451372));
#59803=CARTESIAN_POINT('Ctrl Pts',(2.91557726271063,1.,-3.02314558451372));
#59804=CARTESIAN_POINT('Ctrl Pts',(2.91409518070707,1.,-3.02261975104912));
#59805=CARTESIAN_POINT('Ctrl Pts',(2.91113297349052,1.,-3.02156522743299));
#59806=CARTESIAN_POINT('Ctrl Pts',(2.90669553303902,1.,-3.01997487194926));
#59807=CARTESIAN_POINT('Ctrl Pts',(2.90079069102661,1.,-3.01783725123646));
#59808=CARTESIAN_POINT('Ctrl Pts',(2.8934292556764,1.,-3.01513660433291));
#59809=CARTESIAN_POINT('Ctrl Pts',(2.88608751706796,1.,-3.01240727309568));
#59810=CARTESIAN_POINT('Ctrl Pts',(2.87876560072799,1.,-3.0096491810855));
#59811=CARTESIAN_POINT('Ctrl Pts',(2.87146368430104,1.,-3.00686224485374));
#59812=CARTESIAN_POINT('Ctrl Pts',(2.86418200833065,1.,-3.00404638316245));
#59813=CARTESIAN_POINT('Ctrl Pts',(2.85692085715129,1.,-3.0012015079552));
#59814=CARTESIAN_POINT('Ctrl Pts',(2.84968053289104,1.,-2.99832751144566));
#59815=CARTESIAN_POINT('Ctrl Pts',(2.84246132984334,1.,-2.995424253416));
#59816=CARTESIAN_POINT('Ctrl Pts',(2.83526351254383,1.,-2.99249155170479));
#59817=CARTESIAN_POINT('Ctrl Pts',(2.82808728190402,1.,-2.98952916401699));
#59818=CARTESIAN_POINT('Ctrl Pts',(2.82093279065704,1.,-2.98653680669434));
#59819=CARTESIAN_POINT('Ctrl Pts',(2.81380019196454,1.,-2.9835141977994));
#59820=CARTESIAN_POINT('Ctrl Pts',(2.80668968101162,1.,-2.98046109647299));
#59821=CARTESIAN_POINT('Ctrl Pts',(2.79960153278186,1.,-2.97737733718242));
#59822=CARTESIAN_POINT('Ctrl Pts',(2.79253615718147,1.,-2.97426288347475));
#59823=CARTESIAN_POINT('Ctrl Pts',(2.78549409123657,1.,-2.97111781461349));
#59824=CARTESIAN_POINT('Ctrl Pts',(2.77847589542767,1.,-2.9679422104295));
#59825=CARTESIAN_POINT('Ctrl Pts',(2.77148206836464,1.,-2.96473605585548));
#59826=CARTESIAN_POINT('Ctrl Pts',(2.76451296269571,1.,-2.96149914764832));
#59827=CARTESIAN_POINT('Ctrl Pts',(2.75756867888393,1.,-2.9582309766594));
#59828=CARTESIAN_POINT('Ctrl Pts',(2.75064903318996,1.,-2.95493069316211));
#59829=CARTESIAN_POINT('Ctrl Pts',(2.7437537949221,1.,-2.95159737214305));
#59830=CARTESIAN_POINT('Ctrl Pts',(2.73688288329825,1.,-2.94823023414381));
#59831=CARTESIAN_POINT('Ctrl Pts',(2.73003657371613,1.,-2.94482887675139));
#59832=CARTESIAN_POINT('Ctrl Pts',(2.72321571511322,1.,-2.94139351933882));
#59833=CARTESIAN_POINT('Ctrl Pts',(2.71642190053575,1.,-2.93792519474955));
#59834=CARTESIAN_POINT('Ctrl Pts',(2.70965695523776,1.,-2.93442516311168));
#59835=CARTESIAN_POINT('Ctrl Pts',(2.70292247416881,1.,-2.93089438233746));
#59836=CARTESIAN_POINT('Ctrl Pts',(2.69621932864302,1.,-2.92733294395268));
#59837=CARTESIAN_POINT('Ctrl Pts',(2.68954721165342,1.,-2.92373955325876));
#59838=CARTESIAN_POINT('Ctrl Pts',(2.68290409279689,1.,-2.92011090722152));
#59839=CARTESIAN_POINT('Ctrl Pts',(2.67628728855309,1.,-2.91644290704281));
#59840=CARTESIAN_POINT('Ctrl Pts',(2.66969458792627,1.,-2.91273193382876));
#59841=CARTESIAN_POINT('Ctrl Pts',(2.66312542616808,1.,-2.90897617968921));
#59842=CARTESIAN_POINT('Ctrl Pts',(2.65658188464287,1.,-2.90517678087467));
#59843=CARTESIAN_POINT('Ctrl Pts',(2.65007017365576,1.,-2.90133950224879));
#59844=CARTESIAN_POINT('Ctrl Pts',(2.64359851684146,1.,-2.89747231723361));
#59845=CARTESIAN_POINT('Ctrl Pts',(2.63717442263944,1.,-2.89358228854557));
#59846=CARTESIAN_POINT('Ctrl Pts',(2.63080195420771,1.,-2.88967244854243));
#59847=CARTESIAN_POINT('Ctrl Pts',(2.62447947640253,1.,-2.88573922195049));
#59848=CARTESIAN_POINT('Ctrl Pts',(2.61819596473087,1.,-2.88176821427502));
#59849=CARTESIAN_POINT('Ctrl Pts',(2.61193507170928,1.,-2.87773881947885));
#59850=CARTESIAN_POINT('Ctrl Pts',(2.6056817788128,1.,-2.87363176656475));
#59851=CARTESIAN_POINT('Ctrl Pts',(2.59942875223202,1.,-2.86943633170712));
#59852=CARTESIAN_POINT('Ctrl Pts',(2.59318160184921,1.,-2.86515629953528));
#59853=CARTESIAN_POINT('Ctrl Pts',(2.5869677064356,1.,-2.86081999003668));
#59854=CARTESIAN_POINT('Ctrl Pts',(2.58082875254407,1.,-2.85647171715147));
#59855=CARTESIAN_POINT('Ctrl Pts',(2.57480482727128,1.,-2.85215360144483));
#59856=CARTESIAN_POINT('Ctrl Pts',(2.56891984251743,1.,-2.84788893329091));
#59857=CARTESIAN_POINT('Ctrl Pts',(2.56316920798489,1.,-2.84366802680211));
#59858=CARTESIAN_POINT('Ctrl Pts',(2.55749952145165,1.,-2.83942515220699));
#59859=CARTESIAN_POINT('Ctrl Pts',(2.55182152806964,1.,-2.83505269592412));
#59860=CARTESIAN_POINT('Ctrl Pts',(2.54604736792542,1.,-2.83044254225794));
#59861=CARTESIAN_POINT('Ctrl Pts',(2.54012272520141,1.,-2.82552167649157));
#59862=CARTESIAN_POINT('Ctrl Pts',(2.53405679667463,1.,-2.82028550483744));
#59863=CARTESIAN_POINT('Ctrl Pts',(2.52796388055457,1.,-2.8148437904867));
#59864=CARTESIAN_POINT('Ctrl Pts',(2.52205778589922,1.,-2.80941521967234));
#59865=CARTESIAN_POINT('Ctrl Pts',(2.51660190466067,1.,-2.80427363984939));
#59866=CARTESIAN_POINT('Ctrl Pts',(2.51186983687947,1.,-2.79970585014308));
#59867=CARTESIAN_POINT('Ctrl Pts',(2.50810555977564,1.,-2.7959687805717));
#59868=CARTESIAN_POINT('Ctrl Pts',(2.50567182569153,1.,-2.79344192164204));
#59869=CARTESIAN_POINT('Ctrl Pts',(2.50455968395235,1.,-2.79217568804874));
#59870=CARTESIAN_POINT('Ctrl Pts',(2.50417932839344,1.,-2.79164172519039));
#59871=CARTESIAN_POINT('Ctrl Pts',(2.50410700351427,1.,-2.79145823440899));
#59872=CARTESIAN_POINT('Ctrl Pts',(2.50410331873043,1.,-2.79140942341378));
#59873=CARTESIAN_POINT('',(2.91557726271063,0.,-3.02314558451372));
#59874=CARTESIAN_POINT('Ctrl Pts',(2.79134130681569,-1.,-2.50417924854921));
#59875=CARTESIAN_POINT('Ctrl Pts',(2.79134130681569,1.,-2.50417924854921));
#59876=CARTESIAN_POINT('Ctrl Pts',(2.7913358110015,-1.,-2.50409239460108));
#59877=CARTESIAN_POINT('Ctrl Pts',(2.7913358110015,1.,-2.50409239460108));
#59878=CARTESIAN_POINT('Ctrl Pts',(2.79143626022503,-1.,-2.50404230339286));
#59879=CARTESIAN_POINT('Ctrl Pts',(2.79143626022503,1.,-2.50404230339286));
#59880=CARTESIAN_POINT('Ctrl Pts',(2.79192122907148,-1.,-2.5043379907732));
#59881=CARTESIAN_POINT('Ctrl Pts',(2.79192122907148,1.,-2.5043379907732));
#59882=CARTESIAN_POINT('Ctrl Pts',(2.7932369408851,-1.,-2.50547439929414));
#59883=CARTESIAN_POINT('Ctrl Pts',(2.7932369408851,1.,-2.50547439929414));
#59884=CARTESIAN_POINT('Ctrl Pts',(2.79596878057287,-1.,-2.50810555977671));
#59885=CARTESIAN_POINT('Ctrl Pts',(2.79596878057287,1.,-2.50810555977671));
#59886=CARTESIAN_POINT('Ctrl Pts',(2.79970585014168,-1.,-2.51186983687818));
#59887=CARTESIAN_POINT('Ctrl Pts',(2.79970585014168,1.,-2.51186983687818));
#59888=CARTESIAN_POINT('Ctrl Pts',(2.80427363984653,-1.,-2.51660190465805));
#59889=CARTESIAN_POINT('Ctrl Pts',(2.80427363984653,1.,-2.51660190465805));
#59890=CARTESIAN_POINT('Ctrl Pts',(2.80941521966941,-1.,-2.52205778589653));
#59891=CARTESIAN_POINT('Ctrl Pts',(2.80941521966941,1.,-2.52205778589653));
#59892=CARTESIAN_POINT('Ctrl Pts',(2.81484379048475,-1.,-2.52796388055278));
#59893=CARTESIAN_POINT('Ctrl Pts',(2.81484379048475,1.,-2.52796388055278));
#59894=CARTESIAN_POINT('Ctrl Pts',(2.82028550483689,-1.,-2.53405679667412));
#59895=CARTESIAN_POINT('Ctrl Pts',(2.82028550483689,1.,-2.53405679667412));
#59896=CARTESIAN_POINT('Ctrl Pts',(2.8255216764922,-1.,-2.54012272520199));
#59897=CARTESIAN_POINT('Ctrl Pts',(2.8255216764922,1.,-2.54012272520199));
#59898=CARTESIAN_POINT('Ctrl Pts',(2.83044254225917,-1.,-2.54604736792655));
#59899=CARTESIAN_POINT('Ctrl Pts',(2.83044254225917,1.,-2.54604736792655));
#59900=CARTESIAN_POINT('Ctrl Pts',(2.83505269592536,-1.,-2.55182152807077));
#59901=CARTESIAN_POINT('Ctrl Pts',(2.83505269592536,1.,-2.55182152807077));
#59902=CARTESIAN_POINT('Ctrl Pts',(2.83942515220782,-1.,-2.55749952145241));
#59903=CARTESIAN_POINT('Ctrl Pts',(2.83942515220782,1.,-2.55749952145241));
#59904=CARTESIAN_POINT('Ctrl Pts',(2.84366802680237,-1.,-2.56316920798513));
#59905=CARTESIAN_POINT('Ctrl Pts',(2.84366802680237,1.,-2.56316920798513));
#59906=CARTESIAN_POINT('Ctrl Pts',(2.84788893329067,-1.,-2.56891984251721));
#59907=CARTESIAN_POINT('Ctrl Pts',(2.84788893329067,1.,-2.56891984251721));
#59908=CARTESIAN_POINT('Ctrl Pts',(2.85215360144431,-1.,-2.57480482727081));
#59909=CARTESIAN_POINT('Ctrl Pts',(2.85215360144431,1.,-2.57480482727081));
#59910=CARTESIAN_POINT('Ctrl Pts',(2.85647171715092,-1.,-2.58082875254357));
#59911=CARTESIAN_POINT('Ctrl Pts',(2.85647171715092,1.,-2.58082875254357));
#59912=CARTESIAN_POINT('Ctrl Pts',(2.86081999003629,-1.,-2.58696770643524));
#59913=CARTESIAN_POINT('Ctrl Pts',(2.86081999003629,1.,-2.58696770643524));
#59914=CARTESIAN_POINT('Ctrl Pts',(2.86515629953513,-1.,-2.59318160184908));
#59915=CARTESIAN_POINT('Ctrl Pts',(2.86515629953513,1.,-2.59318160184908));
#59916=CARTESIAN_POINT('Ctrl Pts',(2.86943633170722,-1.,-2.5994287522321));
#59917=CARTESIAN_POINT('Ctrl Pts',(2.86943633170722,1.,-2.5994287522321));
#59918=CARTESIAN_POINT('Ctrl Pts',(2.87363176656501,-1.,-2.60568177881303));
#59919=CARTESIAN_POINT('Ctrl Pts',(2.87363176656501,1.,-2.60568177881303));
#59920=CARTESIAN_POINT('Ctrl Pts',(2.87773881947915,-1.,-2.61193507170955));
#59921=CARTESIAN_POINT('Ctrl Pts',(2.87773881947915,1.,-2.61193507170955));
#59922=CARTESIAN_POINT('Ctrl Pts',(2.88176821427525,-1.,-2.61819596473108));
#59923=CARTESIAN_POINT('Ctrl Pts',(2.88176821427525,1.,-2.61819596473108));
#59924=CARTESIAN_POINT('Ctrl Pts',(2.88573922195059,-1.,-2.62447947640262));
#59925=CARTESIAN_POINT('Ctrl Pts',(2.88573922195059,1.,-2.62447947640262));
#59926=CARTESIAN_POINT('Ctrl Pts',(2.88967244854239,-1.,-2.63080195420767));
#59927=CARTESIAN_POINT('Ctrl Pts',(2.88967244854239,1.,-2.63080195420767));
#59928=CARTESIAN_POINT('Ctrl Pts',(2.89358228854544,-1.,-2.63717442263932));
#59929=CARTESIAN_POINT('Ctrl Pts',(2.89358228854544,1.,-2.63717442263932));
#59930=CARTESIAN_POINT('Ctrl Pts',(2.89747231723345,-1.,-2.64359851684131));
#59931=CARTESIAN_POINT('Ctrl Pts',(2.89747231723345,1.,-2.64359851684131));
#59932=CARTESIAN_POINT('Ctrl Pts',(2.90133950224867,-1.,-2.65007017365564));
#59933=CARTESIAN_POINT('Ctrl Pts',(2.90133950224867,1.,-2.65007017365564));
#59934=CARTESIAN_POINT('Ctrl Pts',(2.90517678087461,-1.,-2.65658188464282));
#59935=CARTESIAN_POINT('Ctrl Pts',(2.90517678087461,1.,-2.65658188464282));
#59936=CARTESIAN_POINT('Ctrl Pts',(2.90897617968923,-1.,-2.6631254261681));
#59937=CARTESIAN_POINT('Ctrl Pts',(2.90897617968923,1.,-2.6631254261681));
#59938=CARTESIAN_POINT('Ctrl Pts',(2.91273193382882,-1.,-2.66969458792631));
#59939=CARTESIAN_POINT('Ctrl Pts',(2.91273193382882,1.,-2.66969458792631));
#59940=CARTESIAN_POINT('Ctrl Pts',(2.91644290704285,-1.,-2.67628728855312));
#59941=CARTESIAN_POINT('Ctrl Pts',(2.91644290704285,1.,-2.67628728855312));
#59942=CARTESIAN_POINT('Ctrl Pts',(2.92011090722152,-1.,-2.68290409279688));
#59943=CARTESIAN_POINT('Ctrl Pts',(2.92011090722152,1.,-2.68290409279688));
#59944=CARTESIAN_POINT('Ctrl Pts',(2.92373955325875,-1.,-2.68954721165339));
#59945=CARTESIAN_POINT('Ctrl Pts',(2.92373955325875,1.,-2.68954721165339));
#59946=CARTESIAN_POINT('Ctrl Pts',(2.92733294395267,-1.,-2.69621932864301));
#59947=CARTESIAN_POINT('Ctrl Pts',(2.92733294395267,1.,-2.69621932864301));
#59948=CARTESIAN_POINT('Ctrl Pts',(2.93089438233749,-1.,-2.70292247416885));
#59949=CARTESIAN_POINT('Ctrl Pts',(2.93089438233749,1.,-2.70292247416885));
#59950=CARTESIAN_POINT('Ctrl Pts',(2.93442516311179,-1.,-2.70965695523787));
#59951=CARTESIAN_POINT('Ctrl Pts',(2.93442516311179,1.,-2.70965695523787));
#59952=CARTESIAN_POINT('Ctrl Pts',(2.93792519474972,-1.,-2.71642190053592));
#59953=CARTESIAN_POINT('Ctrl Pts',(2.93792519474972,1.,-2.71642190053592));
#59954=CARTESIAN_POINT('Ctrl Pts',(2.94139351933897,-1.,-2.72321571511337));
#59955=CARTESIAN_POINT('Ctrl Pts',(2.94139351933897,1.,-2.72321571511337));
#59956=CARTESIAN_POINT('Ctrl Pts',(2.94482887675143,-1.,-2.73003657371617));
#59957=CARTESIAN_POINT('Ctrl Pts',(2.94482887675143,1.,-2.73003657371617));
#59958=CARTESIAN_POINT('Ctrl Pts',(2.94823023414364,-1.,-2.73688288329808));
#59959=CARTESIAN_POINT('Ctrl Pts',(2.94823023414364,1.,-2.73688288329808));
#59960=CARTESIAN_POINT('Ctrl Pts',(2.95159737214266,-1.,-2.74375379492172));
#59961=CARTESIAN_POINT('Ctrl Pts',(2.95159737214266,1.,-2.74375379492172));
#59962=CARTESIAN_POINT('Ctrl Pts',(2.95493069316161,-1.,-2.75064903318947));
#59963=CARTESIAN_POINT('Ctrl Pts',(2.95493069316161,1.,-2.75064903318947));
#59964=CARTESIAN_POINT('Ctrl Pts',(2.95823097665896,-1.,-2.7575686788835));
#59965=CARTESIAN_POINT('Ctrl Pts',(2.95823097665896,1.,-2.7575686788835));
#59966=CARTESIAN_POINT('Ctrl Pts',(2.96149914764818,-1.,-2.76451296269557));
#59967=CARTESIAN_POINT('Ctrl Pts',(2.96149914764818,1.,-2.76451296269557));
#59968=CARTESIAN_POINT('Ctrl Pts',(2.96473605585583,-1.,-2.77148206836498));
#59969=CARTESIAN_POINT('Ctrl Pts',(2.96473605585583,1.,-2.77148206836498));
#59970=CARTESIAN_POINT('Ctrl Pts',(2.96794221043036,-1.,-2.7784758954285));
#59971=CARTESIAN_POINT('Ctrl Pts',(2.96794221043036,1.,-2.7784758954285));
#59972=CARTESIAN_POINT('Ctrl Pts',(2.97111781461465,-1.,-2.78549409123769));
#59973=CARTESIAN_POINT('Ctrl Pts',(2.97111781461465,1.,-2.78549409123769));
#59974=CARTESIAN_POINT('Ctrl Pts',(2.9742628834758,-1.,-2.79253615718248));
#59975=CARTESIAN_POINT('Ctrl Pts',(2.9742628834758,1.,-2.79253615718248));
#59976=CARTESIAN_POINT('Ctrl Pts',(2.97737733718287,-1.,-2.7996015327823));
#59977=CARTESIAN_POINT('Ctrl Pts',(2.97737733718287,1.,-2.7996015327823));
#59978=CARTESIAN_POINT('Ctrl Pts',(2.98046109647241,-1.,-2.80668968101106));
#59979=CARTESIAN_POINT('Ctrl Pts',(2.98046109647241,1.,-2.80668968101106));
#59980=CARTESIAN_POINT('Ctrl Pts',(2.98351419779767,-1.,-2.81380019196286));
#59981=CARTESIAN_POINT('Ctrl Pts',(2.98351419779767,1.,-2.81380019196286));
#59982=CARTESIAN_POINT('Ctrl Pts',(2.9865368066918,-1.,-2.82093279065457));
#59983=CARTESIAN_POINT('Ctrl Pts',(2.9865368066918,1.,-2.82093279065457));
#59984=CARTESIAN_POINT('Ctrl Pts',(2.98952916401446,-1.,-2.82808728190157));
#59985=CARTESIAN_POINT('Ctrl Pts',(2.98952916401446,1.,-2.82808728190157));
#59986=CARTESIAN_POINT('Ctrl Pts',(2.99249155170339,-1.,-2.83526351254248));
#59987=CARTESIAN_POINT('Ctrl Pts',(2.99249155170339,1.,-2.83526351254248));
#59988=CARTESIAN_POINT('Ctrl Pts',(2.99542425341685,-1.,-2.84246132984415));
#59989=CARTESIAN_POINT('Ctrl Pts',(2.99542425341685,1.,-2.84246132984415));
#59990=CARTESIAN_POINT('Ctrl Pts',(2.99832751144925,-1.,-2.84968053289451));
#59991=CARTESIAN_POINT('Ctrl Pts',(2.99832751144925,1.,-2.84968053289451));
#59992=CARTESIAN_POINT('Ctrl Pts',(3.00120150796095,-1.,-2.85692085715686));
#59993=CARTESIAN_POINT('Ctrl Pts',(3.00120150796095,1.,-2.85692085715686));
#59994=CARTESIAN_POINT('Ctrl Pts',(3.00404638316867,-1.,-2.86418200833667));
#59995=CARTESIAN_POINT('Ctrl Pts',(3.00404638316867,1.,-2.86418200833667));
#59996=CARTESIAN_POINT('Ctrl Pts',(3.00686224485784,-1.,-2.87146368430502));
#59997=CARTESIAN_POINT('Ctrl Pts',(3.00686224485784,1.,-2.87146368430502));
#59998=CARTESIAN_POINT('Ctrl Pts',(3.00964918108476,-1.,-2.87876560072727));
#59999=CARTESIAN_POINT('Ctrl Pts',(3.00964918108476,1.,-2.87876560072727));
#60000=CARTESIAN_POINT('Ctrl Pts',(3.01240727308829,-1.,-2.8860875170608));
#60001=CARTESIAN_POINT('Ctrl Pts',(3.01240727308829,1.,-2.8860875170608));
#60002=CARTESIAN_POINT('Ctrl Pts',(3.01513660431928,-1.,-2.89342925566321));
#60003=CARTESIAN_POINT('Ctrl Pts',(3.01513660431928,1.,-2.89342925566321));
#60004=CARTESIAN_POINT('Ctrl Pts',(3.01783725121981,-1.,-2.9007906910105));
#60005=CARTESIAN_POINT('Ctrl Pts',(3.01783725121981,1.,-2.9007906910105));
#60006=CARTESIAN_POINT('Ctrl Pts',(3.01997487193503,-1.,-2.90669553302526));
#60007=CARTESIAN_POINT('Ctrl Pts',(3.01997487193503,1.,-2.90669553302526));
#60008=CARTESIAN_POINT('Ctrl Pts',(3.02156522742431,-1.,-2.91113297348212));
#60009=CARTESIAN_POINT('Ctrl Pts',(3.02156522742431,1.,-2.91113297348212));
#60010=CARTESIAN_POINT('Ctrl Pts',(3.02261975104593,-1.,-2.91409518070399));
#60011=CARTESIAN_POINT('Ctrl Pts',(3.02261975104593,1.,-2.91409518070399));
#60012=CARTESIAN_POINT('Ctrl Pts',(3.02314558451372,-1.,-2.91557726271063));
#60013=CARTESIAN_POINT('Ctrl Pts',(3.02314558451372,1.,-2.91557726271063));
#60014=CARTESIAN_POINT('',(2.79140942341258,1.,-2.50410331873176));
#60015=CARTESIAN_POINT('Ctrl Pts',(2.79140942341258,-1.,-2.50410331873176));
#60016=CARTESIAN_POINT('Ctrl Pts',(2.79140942341258,-0.666666666666667,
-2.50410331873176));
#60017=CARTESIAN_POINT('Ctrl Pts',(2.79140942341258,-0.333333333333333,
-2.50410331873176));
#60018=CARTESIAN_POINT('Ctrl Pts',(2.79140942341258,0.333333333333333,-2.50410331873176));
#60019=CARTESIAN_POINT('Ctrl Pts',(2.79140942341258,0.666666666666667,-2.50410331873176));
#60020=CARTESIAN_POINT('Ctrl Pts',(2.79140942341258,1.,-2.50410331873176));
#60021=CARTESIAN_POINT('',(3.02314558451372,1.,-2.91557726271063));
#60022=CARTESIAN_POINT('',(3.02314558451372,0.,-2.91557726271063));
#60023=CARTESIAN_POINT('Ctrl Pts',(2.79140942341258,1.,-2.50410331873176));
#60024=CARTESIAN_POINT('Ctrl Pts',(2.79145823440781,1.,-2.50410700351493));
#60025=CARTESIAN_POINT('Ctrl Pts',(2.79164172518905,1.,-2.50417932839313));
#60026=CARTESIAN_POINT('Ctrl Pts',(2.79217568804755,1.,-2.50455968395146));
#60027=CARTESIAN_POINT('Ctrl Pts',(2.79344192164147,1.,-2.50567182569081));
#60028=CARTESIAN_POINT('Ctrl Pts',(2.79596878057287,1.,-2.50810555977671));
#60029=CARTESIAN_POINT('Ctrl Pts',(2.79970585014168,1.,-2.51186983687818));
#60030=CARTESIAN_POINT('Ctrl Pts',(2.80427363984653,1.,-2.51660190465805));
#60031=CARTESIAN_POINT('Ctrl Pts',(2.80941521966941,1.,-2.52205778589653));
#60032=CARTESIAN_POINT('Ctrl Pts',(2.81484379048475,1.,-2.52796388055278));
#60033=CARTESIAN_POINT('Ctrl Pts',(2.82028550483689,1.,-2.53405679667412));
#60034=CARTESIAN_POINT('Ctrl Pts',(2.8255216764922,1.,-2.54012272520199));
#60035=CARTESIAN_POINT('Ctrl Pts',(2.83044254225917,1.,-2.54604736792655));
#60036=CARTESIAN_POINT('Ctrl Pts',(2.83505269592536,1.,-2.55182152807077));
#60037=CARTESIAN_POINT('Ctrl Pts',(2.83942515220782,1.,-2.55749952145241));
#60038=CARTESIAN_POINT('Ctrl Pts',(2.84366802680237,1.,-2.56316920798513));
#60039=CARTESIAN_POINT('Ctrl Pts',(2.84788893329067,1.,-2.56891984251721));
#60040=CARTESIAN_POINT('Ctrl Pts',(2.85215360144431,1.,-2.57480482727081));
#60041=CARTESIAN_POINT('Ctrl Pts',(2.85647171715092,1.,-2.58082875254357));
#60042=CARTESIAN_POINT('Ctrl Pts',(2.86081999003629,1.,-2.58696770643524));
#60043=CARTESIAN_POINT('Ctrl Pts',(2.86515629953513,1.,-2.59318160184908));
#60044=CARTESIAN_POINT('Ctrl Pts',(2.86943633170722,1.,-2.5994287522321));
#60045=CARTESIAN_POINT('Ctrl Pts',(2.87363176656501,1.,-2.60568177881303));
#60046=CARTESIAN_POINT('Ctrl Pts',(2.87773881947915,1.,-2.61193507170955));
#60047=CARTESIAN_POINT('Ctrl Pts',(2.88176821427525,1.,-2.61819596473108));
#60048=CARTESIAN_POINT('Ctrl Pts',(2.88573922195059,1.,-2.62447947640262));
#60049=CARTESIAN_POINT('Ctrl Pts',(2.88967244854239,1.,-2.63080195420767));
#60050=CARTESIAN_POINT('Ctrl Pts',(2.89358228854544,1.,-2.63717442263932));
#60051=CARTESIAN_POINT('Ctrl Pts',(2.89747231723345,1.,-2.64359851684131));
#60052=CARTESIAN_POINT('Ctrl Pts',(2.90133950224867,1.,-2.65007017365564));
#60053=CARTESIAN_POINT('Ctrl Pts',(2.90517678087461,1.,-2.65658188464282));
#60054=CARTESIAN_POINT('Ctrl Pts',(2.90897617968923,1.,-2.6631254261681));
#60055=CARTESIAN_POINT('Ctrl Pts',(2.91273193382882,1.,-2.66969458792631));
#60056=CARTESIAN_POINT('Ctrl Pts',(2.91644290704285,1.,-2.67628728855312));
#60057=CARTESIAN_POINT('Ctrl Pts',(2.92011090722152,1.,-2.68290409279688));
#60058=CARTESIAN_POINT('Ctrl Pts',(2.92373955325875,1.,-2.68954721165339));
#60059=CARTESIAN_POINT('Ctrl Pts',(2.92733294395267,1.,-2.69621932864301));
#60060=CARTESIAN_POINT('Ctrl Pts',(2.93089438233749,1.,-2.70292247416885));
#60061=CARTESIAN_POINT('Ctrl Pts',(2.93442516311179,1.,-2.70965695523787));
#60062=CARTESIAN_POINT('Ctrl Pts',(2.93792519474972,1.,-2.71642190053592));
#60063=CARTESIAN_POINT('Ctrl Pts',(2.94139351933897,1.,-2.72321571511337));
#60064=CARTESIAN_POINT('Ctrl Pts',(2.94482887675143,1.,-2.73003657371617));
#60065=CARTESIAN_POINT('Ctrl Pts',(2.94823023414364,1.,-2.73688288329808));
#60066=CARTESIAN_POINT('Ctrl Pts',(2.95159737214266,1.,-2.74375379492172));
#60067=CARTESIAN_POINT('Ctrl Pts',(2.95493069316161,1.,-2.75064903318947));
#60068=CARTESIAN_POINT('Ctrl Pts',(2.95823097665896,1.,-2.7575686788835));
#60069=CARTESIAN_POINT('Ctrl Pts',(2.96149914764818,1.,-2.76451296269557));
#60070=CARTESIAN_POINT('Ctrl Pts',(2.96473605585583,1.,-2.77148206836498));
#60071=CARTESIAN_POINT('Ctrl Pts',(2.96794221043036,1.,-2.7784758954285));
#60072=CARTESIAN_POINT('Ctrl Pts',(2.97111781461465,1.,-2.78549409123769));
#60073=CARTESIAN_POINT('Ctrl Pts',(2.9742628834758,1.,-2.79253615718248));
#60074=CARTESIAN_POINT('Ctrl Pts',(2.97737733718287,1.,-2.7996015327823));
#60075=CARTESIAN_POINT('Ctrl Pts',(2.98046109647241,1.,-2.80668968101106));
#60076=CARTESIAN_POINT('Ctrl Pts',(2.98351419779767,1.,-2.81380019196286));
#60077=CARTESIAN_POINT('Ctrl Pts',(2.9865368066918,1.,-2.82093279065457));
#60078=CARTESIAN_POINT('Ctrl Pts',(2.98952916401446,1.,-2.82808728190157));
#60079=CARTESIAN_POINT('Ctrl Pts',(2.99249155170339,1.,-2.83526351254248));
#60080=CARTESIAN_POINT('Ctrl Pts',(2.99542425341685,1.,-2.84246132984415));
#60081=CARTESIAN_POINT('Ctrl Pts',(2.99832751144925,1.,-2.84968053289451));
#60082=CARTESIAN_POINT('Ctrl Pts',(3.00120150796095,1.,-2.85692085715686));
#60083=CARTESIAN_POINT('Ctrl Pts',(3.00404638316867,1.,-2.86418200833667));
#60084=CARTESIAN_POINT('Ctrl Pts',(3.00686224485784,1.,-2.87146368430502));
#60085=CARTESIAN_POINT('Ctrl Pts',(3.00964918108476,1.,-2.87876560072727));
#60086=CARTESIAN_POINT('Ctrl Pts',(3.01240727308829,1.,-2.8860875170608));
#60087=CARTESIAN_POINT('Ctrl Pts',(3.01513660431928,1.,-2.89342925566321));
#60088=CARTESIAN_POINT('Ctrl Pts',(3.01783725121981,1.,-2.9007906910105));
#60089=CARTESIAN_POINT('Ctrl Pts',(3.01997487193503,1.,-2.90669553302526));
#60090=CARTESIAN_POINT('Ctrl Pts',(3.02156522742431,1.,-2.91113297348212));
#60091=CARTESIAN_POINT('Ctrl Pts',(3.02261975104593,1.,-2.91409518070399));
#60092=CARTESIAN_POINT('Ctrl Pts',(3.02314558451372,1.,-2.91557726271063));
#60093=CARTESIAN_POINT('Origin',(3.02314558451372,0.,-2.91557726271063));
#60094=CARTESIAN_POINT('',(2.91557726271063,1.,-3.02314558451372));
#60095=CARTESIAN_POINT('Origin',(0.,0.,0.));
#60096=CARTESIAN_POINT('',(2.90994629141562,1.,-2.36531447826213));
#60097=CARTESIAN_POINT('Origin',(0.,1.,0.));
#60098=CARTESIAN_POINT('Ctrl Pts',(2.90994629141562,1.,-2.36531447826213));
#60099=CARTESIAN_POINT('Ctrl Pts',(2.90994629141562,0.666666666666667,-2.36531447826213));
#60100=CARTESIAN_POINT('Ctrl Pts',(2.90994629141562,0.333333333333333,-2.36531447826213));
#60101=CARTESIAN_POINT('Ctrl Pts',(2.90994629141562,-0.333333333333333,
-2.36531447826213));
#60102=CARTESIAN_POINT('Ctrl Pts',(2.90994629141562,-0.666666666666667,
-2.36531447826213));
#60103=CARTESIAN_POINT('Ctrl Pts',(2.90994629141562,-1.,-2.36531447826213));
#60104=CARTESIAN_POINT('Ctrl Pts',(3.35260583073571,-1.,-2.52982887637028));
#60105=CARTESIAN_POINT('Ctrl Pts',(3.35260583073571,1.,-2.52982887637028));
#60106=CARTESIAN_POINT('Ctrl Pts',(3.35105973714426,-1.,-2.52954136549357));
#60107=CARTESIAN_POINT('Ctrl Pts',(3.35105973714426,1.,-2.52954136549357));
#60108=CARTESIAN_POINT('Ctrl Pts',(3.34796903577628,-1.,-2.5289632161143));
#60109=CARTESIAN_POINT('Ctrl Pts',(3.34796903577628,1.,-2.5289632161143));
#60110=CARTESIAN_POINT('Ctrl Pts',(3.34333744117093,-1.,-2.52808660916879));
#60111=CARTESIAN_POINT('Ctrl Pts',(3.34333744117093,1.,-2.52808660916879));
#60112=CARTESIAN_POINT('Ctrl Pts',(3.33717090000955,-1.,-2.52689902691551));
#60113=CARTESIAN_POINT('Ctrl Pts',(3.33717090000955,1.,-2.52689902691551));
#60114=CARTESIAN_POINT('Ctrl Pts',(3.32947762189049,-1.,-2.52538321165774));
#60115=CARTESIAN_POINT('Ctrl Pts',(3.32947762189049,1.,-2.52538321165774));
#60116=CARTESIAN_POINT('Ctrl Pts',(3.32179931079521,-1.,-2.52383598396878));
#60117=CARTESIAN_POINT('Ctrl Pts',(3.32179931079521,1.,-2.52383598396878));
#60118=CARTESIAN_POINT('Ctrl Pts',(3.31413607874727,-1.,-2.52225724871375));
#60119=CARTESIAN_POINT('Ctrl Pts',(3.31413607874727,1.,-2.52225724871375));
#60120=CARTESIAN_POINT('Ctrl Pts',(3.30648808814986,-1.,-2.52064689568167));
#60121=CARTESIAN_POINT('Ctrl Pts',(3.30648808814986,1.,-2.52064689568167));
#60122=CARTESIAN_POINT('Ctrl Pts',(3.29885556387661,-1.,-2.51900480700548));
#60123=CARTESIAN_POINT('Ctrl Pts',(3.29885556387661,1.,-2.51900480700548));
#60124=CARTESIAN_POINT('Ctrl Pts',(3.2912387729863,-1.,-2.51733085123316));
#60125=CARTESIAN_POINT('Ctrl Pts',(3.2912387729863,1.,-2.51733085123316));
#60126=CARTESIAN_POINT('Ctrl Pts',(3.28363799702583,-1.,-2.51562487464215));
#60127=CARTESIAN_POINT('Ctrl Pts',(3.28363799702583,1.,-2.51562487464215));
#60128=CARTESIAN_POINT('Ctrl Pts',(3.27605350473048,-1.,-2.51388669270329));
#60129=CARTESIAN_POINT('Ctrl Pts',(3.27605350473048,1.,-2.51388669270329));
#60130=CARTESIAN_POINT('Ctrl Pts',(3.26848552888271,-1.,-2.51211608411539));
#60131=CARTESIAN_POINT('Ctrl Pts',(3.26848552888271,1.,-2.51211608411539));
#60132=CARTESIAN_POINT('Ctrl Pts',(3.26093423001716,-1.,-2.51031277813697));
#60133=CARTESIAN_POINT('Ctrl Pts',(3.26093423001716,1.,-2.51031277813697));
#60134=CARTESIAN_POINT('Ctrl Pts',(3.25339971461265,-1.,-2.50847647070936));
#60135=CARTESIAN_POINT('Ctrl Pts',(3.25339971461265,1.,-2.50847647070936));
#60136=CARTESIAN_POINT('Ctrl Pts',(3.24588208984042,-1.,-2.50660685940645));
#60137=CARTESIAN_POINT('Ctrl Pts',(3.24588208984042,1.,-2.50660685940645));
#60138=CARTESIAN_POINT('Ctrl Pts',(3.23838151080383,-1.,-2.50470367580078));
#60139=CARTESIAN_POINT('Ctrl Pts',(3.23838151080383,1.,-2.50470367580078));
#60140=CARTESIAN_POINT('Ctrl Pts',(3.23089822320596,-1.,-2.50276671338074));
#60141=CARTESIAN_POINT('Ctrl Pts',(3.23089822320596,1.,-2.50276671338074));
#60142=CARTESIAN_POINT('Ctrl Pts',(3.22343262620387,-1.,-2.5007958720187));
#60143=CARTESIAN_POINT('Ctrl Pts',(3.22343262620387,1.,-2.5007958720187));
#60144=CARTESIAN_POINT('Ctrl Pts',(3.21598526261157,-1.,-2.49879114599293));
#60145=CARTESIAN_POINT('Ctrl Pts',(3.21598526261157,1.,-2.49879114599293));
#60146=CARTESIAN_POINT('Ctrl Pts',(3.2085566984974,-1.,-2.49675252647298));
#60147=CARTESIAN_POINT('Ctrl Pts',(3.2085566984974,1.,-2.49675252647298));
#60148=CARTESIAN_POINT('Ctrl Pts',(3.20114742397549,-1.,-2.49467992057726));
#60149=CARTESIAN_POINT('Ctrl Pts',(3.20114742397549,1.,-2.49467992057726));
#60150=CARTESIAN_POINT('Ctrl Pts',(3.19375775555814,-1.,-2.4925730723986));
#60151=CARTESIAN_POINT('Ctrl Pts',(3.19375775555814,1.,-2.4925730723986));
#60152=CARTESIAN_POINT('Ctrl Pts',(3.18638771282315,-1.,-2.49043146334095));
#60153=CARTESIAN_POINT('Ctrl Pts',(3.18638771282315,1.,-2.49043146334095));
#60154=CARTESIAN_POINT('Ctrl Pts',(3.17903698136678,-1.,-2.48825428288243));
#60155=CARTESIAN_POINT('Ctrl Pts',(3.17903698136678,1.,-2.48825428288243));
#60156=CARTESIAN_POINT('Ctrl Pts',(3.17170518863357,-1.,-2.48604065348619));
#60157=CARTESIAN_POINT('Ctrl Pts',(3.17170518863357,1.,-2.48604065348619));
#60158=CARTESIAN_POINT('Ctrl Pts',(3.16439213290181,-1.,-2.48378981792739));
#60159=CARTESIAN_POINT('Ctrl Pts',(3.16439213290181,1.,-2.48378981792739));
#60160=CARTESIAN_POINT('Ctrl Pts',(3.15709802322735,-1.,-2.48150133566568));
#60161=CARTESIAN_POINT('Ctrl Pts',(3.15709802322735,1.,-2.48150133566568));
#60162=CARTESIAN_POINT('Ctrl Pts',(3.14982373241335,-1.,-2.47917529057016));
#60163=CARTESIAN_POINT('Ctrl Pts',(3.14982373241335,1.,-2.47917529057016));
#60164=CARTESIAN_POINT('Ctrl Pts',(3.14257099546531,-1.,-2.47681245356095));
#60165=CARTESIAN_POINT('Ctrl Pts',(3.14257099546531,1.,-2.47681245356095));
#60166=CARTESIAN_POINT('Ctrl Pts',(3.13534181229282,-1.,-2.47441378371923));
#60167=CARTESIAN_POINT('Ctrl Pts',(3.13534181229282,1.,-2.47441378371923));
#60168=CARTESIAN_POINT('Ctrl Pts',(3.12813790805948,-1.,-2.47197997765868));
#60169=CARTESIAN_POINT('Ctrl Pts',(3.12813790805948,1.,-2.47197997765868));
#60170=CARTESIAN_POINT('Ctrl Pts',(3.12096015766984,-1.,-2.4695109894747));
#60171=CARTESIAN_POINT('Ctrl Pts',(3.12096015766984,1.,-2.4695109894747));
#60172=CARTESIAN_POINT('Ctrl Pts',(3.11380805536124,-1.,-2.46700558843507));
#60173=CARTESIAN_POINT('Ctrl Pts',(3.11380805536124,1.,-2.46700558843507));
#60174=CARTESIAN_POINT('Ctrl Pts',(3.10667907901981,-1.,-2.46446082979645));
#60175=CARTESIAN_POINT('Ctrl Pts',(3.10667907901981,1.,-2.46446082979645));
#60176=CARTESIAN_POINT('Ctrl Pts',(3.09956993697048,-1.,-2.4618730850188));
#60177=CARTESIAN_POINT('Ctrl Pts',(3.09956993697048,1.,-2.4618730850188));
#60178=CARTESIAN_POINT('Ctrl Pts',(3.09247787931881,-1.,-2.45923912563875));
#60179=CARTESIAN_POINT('Ctrl Pts',(3.09247787931881,1.,-2.45923912563875));
#60180=CARTESIAN_POINT('Ctrl Pts',(3.08540206545313,-1.,-2.45655725437037));
#60181=CARTESIAN_POINT('Ctrl Pts',(3.08540206545313,1.,-2.45655725437037));
#60182=CARTESIAN_POINT('Ctrl Pts',(3.07834472886145,-1.,-2.45382826787795));
#60183=CARTESIAN_POINT('Ctrl Pts',(3.07834472886145,1.,-2.45382826787795));
#60184=CARTESIAN_POINT('Ctrl Pts',(3.0713129052131,-1.,-2.45105688854432));
#60185=CARTESIAN_POINT('Ctrl Pts',(3.0713129052131,1.,-2.45105688854432));
#60186=CARTESIAN_POINT('Ctrl Pts',(3.06431596421422,-1.,-2.44824970516558));
#60187=CARTESIAN_POINT('Ctrl Pts',(3.06431596421422,1.,-2.44824970516558));
#60188=CARTESIAN_POINT('Ctrl Pts',(3.05736242671521,-1.,-2.44541251892568));
#60189=CARTESIAN_POINT('Ctrl Pts',(3.05736242671521,1.,-2.44541251892568));
#60190=CARTESIAN_POINT('Ctrl Pts',(3.05045678021509,-1.,-2.44254768923109));
#60191=CARTESIAN_POINT('Ctrl Pts',(3.05045678021509,1.,-2.44254768923109));
#60192=CARTESIAN_POINT('Ctrl Pts',(3.04359685040545,-1.,-2.43965194061849));
#60193=CARTESIAN_POINT('Ctrl Pts',(3.04359685040545,1.,-2.43965194061849));
#60194=CARTESIAN_POINT('Ctrl Pts',(3.03676949672797,-1.,-2.43671278042394));
#60195=CARTESIAN_POINT('Ctrl Pts',(3.03676949672797,1.,-2.43671278042394));
#60196=CARTESIAN_POINT('Ctrl Pts',(3.02995534946946,-1.,-2.43371241361462));
#60197=CARTESIAN_POINT('Ctrl Pts',(3.02995534946946,1.,-2.43371241361462));
#60198=CARTESIAN_POINT('Ctrl Pts',(3.02313656035977,-1.,-2.43063415586615));
#60199=CARTESIAN_POINT('Ctrl Pts',(3.02313656035977,1.,-2.43063415586615));
#60200=CARTESIAN_POINT('Ctrl Pts',(3.01630420830493,-1.,-2.4274685626416));
#60201=CARTESIAN_POINT('Ctrl Pts',(3.01630420830493,1.,-2.4274685626416));
#60202=CARTESIAN_POINT('Ctrl Pts',(3.00946442616674,-1.,-2.42421849439625));
#60203=CARTESIAN_POINT('Ctrl Pts',(3.00946442616674,1.,-2.42421849439625));
#60204=CARTESIAN_POINT('Ctrl Pts',(3.00264868586038,-1.,-2.42090763946812));
#60205=CARTESIAN_POINT('Ctrl Pts',(3.00264868586038,1.,-2.42090763946812));
#60206=CARTESIAN_POINT('Ctrl Pts',(2.99590509293561,-1.,-2.4175732450056));
#60207=CARTESIAN_POINT('Ctrl Pts',(2.99590509293561,1.,-2.4175732450056));
#60208=CARTESIAN_POINT('Ctrl Pts',(2.98927983005851,-1.,-2.4142506419963));
#60209=CARTESIAN_POINT('Ctrl Pts',(2.98927983005851,1.,-2.4142506419963));
#60210=CARTESIAN_POINT('Ctrl Pts',(2.98280015815132,-1.,-2.41095909342591));
#60211=CARTESIAN_POINT('Ctrl Pts',(2.98280015815132,1.,-2.41095909342591));
#60212=CARTESIAN_POINT('Ctrl Pts',(2.97646002822395,-1.,-2.40768975073691));
#60213=CARTESIAN_POINT('Ctrl Pts',(2.97646002822395,1.,-2.40768975073691));
#60214=CARTESIAN_POINT('Ctrl Pts',(2.97019641312272,-1.,-2.40438604734848));
#60215=CARTESIAN_POINT('Ctrl Pts',(2.97019641312272,1.,-2.40438604734848));
#60216=CARTESIAN_POINT('Ctrl Pts',(2.9639043224018,-1.,-2.40095565711535));
#60217=CARTESIAN_POINT('Ctrl Pts',(2.9639043224018,1.,-2.40095565711535));
#60218=CARTESIAN_POINT('Ctrl Pts',(2.95748006482811,-1.,-2.39730553974412));
#60219=CARTESIAN_POINT('Ctrl Pts',(2.95748006482811,1.,-2.39730553974412));
#60220=CARTESIAN_POINT('Ctrl Pts',(2.95085857128372,-1.,-2.39337207631613));
#60221=CARTESIAN_POINT('Ctrl Pts',(2.95085857128372,1.,-2.39337207631613));
#60222=CARTESIAN_POINT('Ctrl Pts',(2.94404820669135,-1.,-2.38914929090806));
#60223=CARTESIAN_POINT('Ctrl Pts',(2.94404820669135,1.,-2.38914929090806));
#60224=CARTESIAN_POINT('Ctrl Pts',(2.93717903280599,-1.,-2.38472771516476));
#60225=CARTESIAN_POINT('Ctrl Pts',(2.93717903280599,1.,-2.38472771516476));
#60226=CARTESIAN_POINT('Ctrl Pts',(2.93049643640517,-1.,-2.3802898958232));
#60227=CARTESIAN_POINT('Ctrl Pts',(2.93049643640517,1.,-2.3802898958232));
#60228=CARTESIAN_POINT('Ctrl Pts',(2.92430340582912,-1.,-2.37606510524271));
#60229=CARTESIAN_POINT('Ctrl Pts',(2.92430340582912,1.,-2.37606510524271));
#60230=CARTESIAN_POINT('Ctrl Pts',(2.9189150379156,-1.,-2.37229381109939));
#60231=CARTESIAN_POINT('Ctrl Pts',(2.9189150379156,1.,-2.37229381109939));
#60232=CARTESIAN_POINT('Ctrl Pts',(2.91461249883016,-1.,-2.36919161373074));
#60233=CARTESIAN_POINT('Ctrl Pts',(2.91461249883016,1.,-2.36919161373074));
#60234=CARTESIAN_POINT('Ctrl Pts',(2.9115863784165,-1.,-2.36690501170317));
#60235=CARTESIAN_POINT('Ctrl Pts',(2.9115863784165,1.,-2.36690501170317));
#60236=CARTESIAN_POINT('Ctrl Pts',(2.91025813829606,-1.,-2.36578327194396));
#60237=CARTESIAN_POINT('Ctrl Pts',(2.91025813829606,1.,-2.36578327194396));
#60238=CARTESIAN_POINT('Ctrl Pts',(2.90989022547738,-1.,-2.36535052956704));
#60239=CARTESIAN_POINT('Ctrl Pts',(2.90989022547738,1.,-2.36535052956704));
#60240=CARTESIAN_POINT('Ctrl Pts',(2.90992398626098,-1.,-2.36524348105023));
#60241=CARTESIAN_POINT('Ctrl Pts',(2.90992398626098,1.,-2.36524348105023));
#60242=CARTESIAN_POINT('Ctrl Pts',(2.91001063062876,-1.,-2.36523532225181));
#60243=CARTESIAN_POINT('Ctrl Pts',(2.91001063062876,1.,-2.36523532225181));
#60244=CARTESIAN_POINT('',(3.35260583073571,1.,-2.52982887637028));
#60245=CARTESIAN_POINT('Ctrl Pts',(3.35260583073571,1.,-2.52982887637028));
#60246=CARTESIAN_POINT('Ctrl Pts',(3.35105973714426,1.,-2.52954136549357));
#60247=CARTESIAN_POINT('Ctrl Pts',(3.34796903577628,1.,-2.5289632161143));
#60248=CARTESIAN_POINT('Ctrl Pts',(3.34333744117093,1.,-2.52808660916879));
#60249=CARTESIAN_POINT('Ctrl Pts',(3.33717090000955,1.,-2.52689902691551));
#60250=CARTESIAN_POINT('Ctrl Pts',(3.32947762189049,1.,-2.52538321165774));
#60251=CARTESIAN_POINT('Ctrl Pts',(3.32179931079521,1.,-2.52383598396878));
#60252=CARTESIAN_POINT('Ctrl Pts',(3.31413607874727,1.,-2.52225724871375));
#60253=CARTESIAN_POINT('Ctrl Pts',(3.30648808814986,1.,-2.52064689568167));
#60254=CARTESIAN_POINT('Ctrl Pts',(3.29885556387661,1.,-2.51900480700548));
#60255=CARTESIAN_POINT('Ctrl Pts',(3.2912387729863,1.,-2.51733085123316));
#60256=CARTESIAN_POINT('Ctrl Pts',(3.28363799702583,1.,-2.51562487464215));
#60257=CARTESIAN_POINT('Ctrl Pts',(3.27605350473048,1.,-2.51388669270329));
#60258=CARTESIAN_POINT('Ctrl Pts',(3.26848552888271,1.,-2.51211608411539));
#60259=CARTESIAN_POINT('Ctrl Pts',(3.26093423001716,1.,-2.51031277813697));
#60260=CARTESIAN_POINT('Ctrl Pts',(3.25339971461265,1.,-2.50847647070936));
#60261=CARTESIAN_POINT('Ctrl Pts',(3.24588208984042,1.,-2.50660685940645));
#60262=CARTESIAN_POINT('Ctrl Pts',(3.23838151080383,1.,-2.50470367580078));
#60263=CARTESIAN_POINT('Ctrl Pts',(3.23089822320596,1.,-2.50276671338074));
#60264=CARTESIAN_POINT('Ctrl Pts',(3.22343262620387,1.,-2.5007958720187));
#60265=CARTESIAN_POINT('Ctrl Pts',(3.21598526261157,1.,-2.49879114599293));
#60266=CARTESIAN_POINT('Ctrl Pts',(3.2085566984974,1.,-2.49675252647298));
#60267=CARTESIAN_POINT('Ctrl Pts',(3.20114742397549,1.,-2.49467992057726));
#60268=CARTESIAN_POINT('Ctrl Pts',(3.19375775555814,1.,-2.4925730723986));
#60269=CARTESIAN_POINT('Ctrl Pts',(3.18638771282315,1.,-2.49043146334095));
#60270=CARTESIAN_POINT('Ctrl Pts',(3.17903698136678,1.,-2.48825428288243));
#60271=CARTESIAN_POINT('Ctrl Pts',(3.17170518863357,1.,-2.48604065348619));
#60272=CARTESIAN_POINT('Ctrl Pts',(3.16439213290181,1.,-2.48378981792739));
#60273=CARTESIAN_POINT('Ctrl Pts',(3.15709802322735,1.,-2.48150133566568));
#60274=CARTESIAN_POINT('Ctrl Pts',(3.14982373241335,1.,-2.47917529057016));
#60275=CARTESIAN_POINT('Ctrl Pts',(3.14257099546531,1.,-2.47681245356095));
#60276=CARTESIAN_POINT('Ctrl Pts',(3.13534181229282,1.,-2.47441378371923));
#60277=CARTESIAN_POINT('Ctrl Pts',(3.12813790805948,1.,-2.47197997765868));
#60278=CARTESIAN_POINT('Ctrl Pts',(3.12096015766984,1.,-2.4695109894747));
#60279=CARTESIAN_POINT('Ctrl Pts',(3.11380805536124,1.,-2.46700558843507));
#60280=CARTESIAN_POINT('Ctrl Pts',(3.10667907901981,1.,-2.46446082979645));
#60281=CARTESIAN_POINT('Ctrl Pts',(3.09956993697048,1.,-2.4618730850188));
#60282=CARTESIAN_POINT('Ctrl Pts',(3.09247787931881,1.,-2.45923912563875));
#60283=CARTESIAN_POINT('Ctrl Pts',(3.08540206545313,1.,-2.45655725437037));
#60284=CARTESIAN_POINT('Ctrl Pts',(3.07834472886145,1.,-2.45382826787795));
#60285=CARTESIAN_POINT('Ctrl Pts',(3.0713129052131,1.,-2.45105688854432));
#60286=CARTESIAN_POINT('Ctrl Pts',(3.06431596421422,1.,-2.44824970516558));
#60287=CARTESIAN_POINT('Ctrl Pts',(3.05736242671521,1.,-2.44541251892568));
#60288=CARTESIAN_POINT('Ctrl Pts',(3.05045678021509,1.,-2.44254768923109));
#60289=CARTESIAN_POINT('Ctrl Pts',(3.04359685040545,1.,-2.43965194061849));
#60290=CARTESIAN_POINT('Ctrl Pts',(3.03676949672797,1.,-2.43671278042394));
#60291=CARTESIAN_POINT('Ctrl Pts',(3.02995534946946,1.,-2.43371241361462));
#60292=CARTESIAN_POINT('Ctrl Pts',(3.02313656035977,1.,-2.43063415586615));
#60293=CARTESIAN_POINT('Ctrl Pts',(3.01630420830493,1.,-2.4274685626416));
#60294=CARTESIAN_POINT('Ctrl Pts',(3.00946442616674,1.,-2.42421849439625));
#60295=CARTESIAN_POINT('Ctrl Pts',(3.00264868586038,1.,-2.42090763946812));
#60296=CARTESIAN_POINT('Ctrl Pts',(2.99590509293561,1.,-2.4175732450056));
#60297=CARTESIAN_POINT('Ctrl Pts',(2.98927983005851,1.,-2.4142506419963));
#60298=CARTESIAN_POINT('Ctrl Pts',(2.98280015815132,1.,-2.41095909342591));
#60299=CARTESIAN_POINT('Ctrl Pts',(2.97646002822395,1.,-2.40768975073691));
#60300=CARTESIAN_POINT('Ctrl Pts',(2.97019641312272,1.,-2.40438604734848));
#60301=CARTESIAN_POINT('Ctrl Pts',(2.9639043224018,1.,-2.40095565711535));
#60302=CARTESIAN_POINT('Ctrl Pts',(2.95748006482811,1.,-2.39730553974412));
#60303=CARTESIAN_POINT('Ctrl Pts',(2.95085857128372,1.,-2.39337207631613));
#60304=CARTESIAN_POINT('Ctrl Pts',(2.94404820669135,1.,-2.38914929090806));
#60305=CARTESIAN_POINT('Ctrl Pts',(2.93717903280599,1.,-2.38472771516476));
#60306=CARTESIAN_POINT('Ctrl Pts',(2.93049643640517,1.,-2.3802898958232));
#60307=CARTESIAN_POINT('Ctrl Pts',(2.92430340582912,1.,-2.37606510524271));
#60308=CARTESIAN_POINT('Ctrl Pts',(2.9189150379156,1.,-2.37229381109939));
#60309=CARTESIAN_POINT('Ctrl Pts',(2.91461249883016,1.,-2.36919161373074));
#60310=CARTESIAN_POINT('Ctrl Pts',(2.91181344022628,1.,-2.36707658451709));
#60311=CARTESIAN_POINT('Ctrl Pts',(2.91051690822262,1.,-2.36599991765853));
#60312=CARTESIAN_POINT('Ctrl Pts',(2.9100577052777,1.,-2.36553202948741));
#60313=CARTESIAN_POINT('Ctrl Pts',(2.90995756655558,1.,-2.3653621118858));
#60314=CARTESIAN_POINT('Ctrl Pts',(2.90994629141562,1.,-2.36531447826213));
#60315=CARTESIAN_POINT('',(3.35260583073571,0.,-2.52982887637028));
#60316=CARTESIAN_POINT('Ctrl Pts',(3.1487152044751,-1.,-2.03668666247593));
#60317=CARTESIAN_POINT('Ctrl Pts',(3.1487152044751,1.,-2.03668666247593));
#60318=CARTESIAN_POINT('Ctrl Pts',(3.14869618937258,-1.,-2.03660173757879));
#60319=CARTESIAN_POINT('Ctrl Pts',(3.14869618937258,1.,-2.03660173757879));
#60320=CARTESIAN_POINT('Ctrl Pts',(3.14878756590812,-1.,-2.03653654935592));
#60321=CARTESIAN_POINT('Ctrl Pts',(3.14878756590812,1.,-2.03653654935592));
#60322=CARTESIAN_POINT('Ctrl Pts',(3.14931281968048,-1.,-2.03675273049189));
#60323=CARTESIAN_POINT('Ctrl Pts',(3.14931281968048,1.,-2.03675273049189));
#60324=CARTESIAN_POINT('Ctrl Pts',(3.15079010635742,-1.,-2.03766932526445));
#60325=CARTESIAN_POINT('Ctrl Pts',(3.15079010635742,1.,-2.03766932526445));
#60326=CARTESIAN_POINT('Ctrl Pts',(3.15389991674792,-1.,-2.03984073791519));
#60327=CARTESIAN_POINT('Ctrl Pts',(3.15389991674792,1.,-2.03984073791519));
#60328=CARTESIAN_POINT('Ctrl Pts',(3.15817983946367,-1.,-2.04297406404027));
#60329=CARTESIAN_POINT('Ctrl Pts',(3.15817983946367,1.,-2.04297406404027));
#60330=CARTESIAN_POINT('Ctrl Pts',(3.16343165058912,-1.,-2.04693331247446));
#60331=CARTESIAN_POINT('Ctrl Pts',(3.16343165058912,1.,-2.04693331247446));
#60332=CARTESIAN_POINT('Ctrl Pts',(3.16936341689527,-1.,-2.05151770247233));
#60333=CARTESIAN_POINT('Ctrl Pts',(3.16936341689527,1.,-2.05151770247233));
#60334=CARTESIAN_POINT('Ctrl Pts',(3.17564906975371,-1.,-2.05650186773132));
#60335=CARTESIAN_POINT('Ctrl Pts',(3.17564906975371,1.,-2.05650186773132));
#60336=CARTESIAN_POINT('Ctrl Pts',(3.18197692964614,-1.,-2.06166849827101));
#60337=CARTESIAN_POINT('Ctrl Pts',(3.18197692964614,1.,-2.06166849827101));
#60338=CARTESIAN_POINT('Ctrl Pts',(3.18809755562368,-1.,-2.06684062744112));
#60339=CARTESIAN_POINT('Ctrl Pts',(3.18809755562368,1.,-2.06684062744112));
#60340=CARTESIAN_POINT('Ctrl Pts',(3.19388465568252,-1.,-2.07192253497857));
#60341=CARTESIAN_POINT('Ctrl Pts',(3.19388465568252,1.,-2.07192253497857));
#60342=CARTESIAN_POINT('Ctrl Pts',(3.19934132836019,-1.,-2.07690441870722));
#60343=CARTESIAN_POINT('Ctrl Pts',(3.19934132836019,1.,-2.07690441870722));
#60344=CARTESIAN_POINT('Ctrl Pts',(3.2045481863073,-1.,-2.08182850370878));
#60345=CARTESIAN_POINT('Ctrl Pts',(3.2045481863073,1.,-2.08182850370878));
#60346=CARTESIAN_POINT('Ctrl Pts',(3.20962575845463,-1.,-2.08676465517455));
#60347=CARTESIAN_POINT('Ctrl Pts',(3.20962575845463,1.,-2.08676465517455));
#60348=CARTESIAN_POINT('Ctrl Pts',(3.21469429601654,-1.,-2.09178419460443));
#60349=CARTESIAN_POINT('Ctrl Pts',(3.21469429601654,1.,-2.09178419460443));
#60350=CARTESIAN_POINT('Ctrl Pts',(3.21982707347009,-1.,-2.09692958434895));
#60351=CARTESIAN_POINT('Ctrl Pts',(3.21982707347009,1.,-2.09692958434895));
#60352=CARTESIAN_POINT('Ctrl Pts',(3.22503437553434,-1.,-2.10220384298492));
#60353=CARTESIAN_POINT('Ctrl Pts',(3.22503437553434,1.,-2.10220384298492));
#60354=CARTESIAN_POINT('Ctrl Pts',(3.23028945793289,-1.,-2.10758699642451));
#60355=CARTESIAN_POINT('Ctrl Pts',(3.23028945793289,1.,-2.10758699642451));
#60356=CARTESIAN_POINT('Ctrl Pts',(3.23554444767099,-1.,-2.11304604021773));
#60357=CARTESIAN_POINT('Ctrl Pts',(3.23554444767099,1.,-2.11304604021773));
#60358=CARTESIAN_POINT('Ctrl Pts',(3.24074905517293,-1.,-2.11854673326979));
#60359=CARTESIAN_POINT('Ctrl Pts',(3.24074905517293,1.,-2.11854673326979));
#60360=CARTESIAN_POINT('Ctrl Pts',(3.24587102613376,-1.,-2.12406646410962));
#60361=CARTESIAN_POINT('Ctrl Pts',(3.24587102613376,1.,-2.12406646410962));
#60362=CARTESIAN_POINT('Ctrl Pts',(3.25090574494028,-1.,-2.12960028396832));
#60363=CARTESIAN_POINT('Ctrl Pts',(3.25090574494028,1.,-2.12960028396832));
#60364=CARTESIAN_POINT('Ctrl Pts',(3.25586495065054,-1.,-2.13515375878803));
#60365=CARTESIAN_POINT('Ctrl Pts',(3.25586495065054,1.,-2.13515375878803));
#60366=CARTESIAN_POINT('Ctrl Pts',(3.26077002641879,-1.,-2.14073870754264));
#60367=CARTESIAN_POINT('Ctrl Pts',(3.26077002641879,1.,-2.14073870754264));
#60368=CARTESIAN_POINT('Ctrl Pts',(3.26564388189759,-1.,-2.1463680529566));
#60369=CARTESIAN_POINT('Ctrl Pts',(3.26564388189759,1.,-2.1463680529566));
#60370=CARTESIAN_POINT('Ctrl Pts',(3.27050245897228,-1.,-2.15205043199808));
#60371=CARTESIAN_POINT('Ctrl Pts',(3.27050245897228,1.,-2.15205043199808));
#60372=CARTESIAN_POINT('Ctrl Pts',(3.27534954469187,-1.,-2.15778690038347));
#60373=CARTESIAN_POINT('Ctrl Pts',(3.27534954469187,1.,-2.15778690038347));
#60374=CARTESIAN_POINT('Ctrl Pts',(3.280181508414,-1.,-2.16357391934425));
#60375=CARTESIAN_POINT('Ctrl Pts',(3.280181508414,1.,-2.16357391934425));
#60376=CARTESIAN_POINT('Ctrl Pts',(3.28499019979724,-1.,-2.16940517773455));
#60377=CARTESIAN_POINT('Ctrl Pts',(3.28499019979724,1.,-2.16940517773455));
#60378=CARTESIAN_POINT('Ctrl Pts',(3.28976645712568,-1.,-2.17527380048423));
#60379=CARTESIAN_POINT('Ctrl Pts',(3.28976645712568,1.,-2.17527380048423));
#60380=CARTESIAN_POINT('Ctrl Pts',(3.2945036150049,-1.,-2.18117455557065));
#60381=CARTESIAN_POINT('Ctrl Pts',(3.2945036150049,1.,-2.18117455557065));
#60382=CARTESIAN_POINT('Ctrl Pts',(3.29920022557639,-1.,-2.18710556500327));
#60383=CARTESIAN_POINT('Ctrl Pts',(3.29920022557639,1.,-2.18710556500327));
#60384=CARTESIAN_POINT('Ctrl Pts',(3.30385816281831,-1.,-2.19306710376111));
#60385=CARTESIAN_POINT('Ctrl Pts',(3.30385816281831,1.,-2.19306710376111));
#60386=CARTESIAN_POINT('Ctrl Pts',(3.30848134694595,-1.,-2.19906078949923));
#60387=CARTESIAN_POINT('Ctrl Pts',(3.30848134694595,1.,-2.19906078949923));
#60388=CARTESIAN_POINT('Ctrl Pts',(3.31307424608949,-1.,-2.20508863150607));
#60389=CARTESIAN_POINT('Ctrl Pts',(3.31307424608949,1.,-2.20508863150607));
#60390=CARTESIAN_POINT('Ctrl Pts',(3.31764044024235,-1.,-2.21115211847875));
#60391=CARTESIAN_POINT('Ctrl Pts',(3.31764044024235,1.,-2.21115211847875));
#60392=CARTESIAN_POINT('Ctrl Pts',(3.32218125618968,-1.,-2.21725135110898));
#60393=CARTESIAN_POINT('Ctrl Pts',(3.32218125618968,1.,-2.21725135110898));
#60394=CARTESIAN_POINT('Ctrl Pts',(3.3266964672289,-1.,-2.22338548312772));
#60395=CARTESIAN_POINT('Ctrl Pts',(3.3266964672289,1.,-2.22338548312772));
#60396=CARTESIAN_POINT('Ctrl Pts',(3.33118487773611,-1.,-2.22955308907233));
#60397=CARTESIAN_POINT('Ctrl Pts',(3.33118487773611,1.,-2.22955308907233));
#60398=CARTESIAN_POINT('Ctrl Pts',(3.33564495756481,-1.,-2.23575256328812));
#60399=CARTESIAN_POINT('Ctrl Pts',(3.33564495756481,1.,-2.23575256328812));
#60400=CARTESIAN_POINT('Ctrl Pts',(3.34007543738025,-1.,-2.24198249391422));
#60401=CARTESIAN_POINT('Ctrl Pts',(3.34007543738025,1.,-2.24198249391422));
#60402=CARTESIAN_POINT('Ctrl Pts',(3.34447596770723,-1.,-2.24824207678256));
#60403=CARTESIAN_POINT('Ctrl Pts',(3.34447596770723,1.,-2.24824207678256));
#60404=CARTESIAN_POINT('Ctrl Pts',(3.34884690292285,-1.,-2.25453097693483));
#60405=CARTESIAN_POINT('Ctrl Pts',(3.34884690292285,1.,-2.25453097693483));
#60406=CARTESIAN_POINT('Ctrl Pts',(3.35318902552626,-1.,-2.26084915222449));
#60407=CARTESIAN_POINT('Ctrl Pts',(3.35318902552626,1.,-2.26084915222449));
#60408=CARTESIAN_POINT('Ctrl Pts',(3.35750328523061,-1.,-2.2671966857991));
#60409=CARTESIAN_POINT('Ctrl Pts',(3.35750328523061,1.,-2.2671966857991));
#60410=CARTESIAN_POINT('Ctrl Pts',(3.36179055004409,-1.,-2.2735736262093));
#60411=CARTESIAN_POINT('Ctrl Pts',(3.36179055004409,1.,-2.2735736262093));
#60412=CARTESIAN_POINT('Ctrl Pts',(3.36605130713076,-1.,-2.27997979458037));
#60413=CARTESIAN_POINT('Ctrl Pts',(3.36605130713076,1.,-2.27997979458037));
#60414=CARTESIAN_POINT('Ctrl Pts',(3.37028570206488,-1.,-2.28641481081137));
#60415=CARTESIAN_POINT('Ctrl Pts',(3.37028570206488,1.,-2.28641481081137));
#60416=CARTESIAN_POINT('Ctrl Pts',(3.37449367172826,-1.,-2.29287818007393));
#60417=CARTESIAN_POINT('Ctrl Pts',(3.37449367172826,1.,-2.29287818007393));
#60418=CARTESIAN_POINT('Ctrl Pts',(3.37867504959433,-1.,-2.29936936127624));
#60419=CARTESIAN_POINT('Ctrl Pts',(3.37867504959433,1.,-2.29936936127624));
#60420=CARTESIAN_POINT('Ctrl Pts',(3.3828296733661,-1.,-2.30588783640343));
#60421=CARTESIAN_POINT('Ctrl Pts',(3.3828296733661,1.,-2.30588783640343));
#60422=CARTESIAN_POINT('Ctrl Pts',(3.38695751492462,-1.,-2.31243319489367));
#60423=CARTESIAN_POINT('Ctrl Pts',(3.38695751492462,1.,-2.31243319489367));
#60424=CARTESIAN_POINT('Ctrl Pts',(3.39105869474822,-1.,-2.31900513925424));
#60425=CARTESIAN_POINT('Ctrl Pts',(3.39105869474822,1.,-2.31900513925424));
#60426=CARTESIAN_POINT('Ctrl Pts',(3.39513342019756,-1.,-2.3256034390248));
#60427=CARTESIAN_POINT('Ctrl Pts',(3.39513342019756,1.,-2.3256034390248));
#60428=CARTESIAN_POINT('Ctrl Pts',(3.39918194577956,-1.,-2.33222789882489));
#60429=CARTESIAN_POINT('Ctrl Pts',(3.39918194577956,1.,-2.33222789882489));
#60430=CARTESIAN_POINT('Ctrl Pts',(3.40320452776743,-1.,-2.33887832342782));
#60431=CARTESIAN_POINT('Ctrl Pts',(3.40320452776743,1.,-2.33887832342782));
#60432=CARTESIAN_POINT('Ctrl Pts',(3.40720137404297,-1.,-2.34555447649188));
#60433=CARTESIAN_POINT('Ctrl Pts',(3.40720137404297,1.,-2.34555447649188));
#60434=CARTESIAN_POINT('Ctrl Pts',(3.41117262314119,-1.,-2.35225606824109));
#60435=CARTESIAN_POINT('Ctrl Pts',(3.41117262314119,1.,-2.35225606824109));
#60436=CARTESIAN_POINT('Ctrl Pts',(3.41511836751469,-1.,-2.35898278606946));
#60437=CARTESIAN_POINT('Ctrl Pts',(3.41511836751469,1.,-2.35898278606946));
#60438=CARTESIAN_POINT('Ctrl Pts',(3.41903866635852,-1.,-2.36573431470642));
#60439=CARTESIAN_POINT('Ctrl Pts',(3.41903866635852,1.,-2.36573431470642));
#60440=CARTESIAN_POINT('Ctrl Pts',(3.42293356216511,-1.,-2.37251035954292));
#60441=CARTESIAN_POINT('Ctrl Pts',(3.42293356216511,1.,-2.37251035954292));
#60442=CARTESIAN_POINT('Ctrl Pts',(3.42680309754399,-1.,-2.37931067028926));
#60443=CARTESIAN_POINT('Ctrl Pts',(3.42680309754399,1.,-2.37931067028926));
#60444=CARTESIAN_POINT('Ctrl Pts',(3.43064732712919,-1.,-2.38613505843552));
#60445=CARTESIAN_POINT('Ctrl Pts',(3.43064732712919,1.,-2.38613505843552));
#60446=CARTESIAN_POINT('Ctrl Pts',(3.4344663067854,-1.,-2.39298338804493));
#60447=CARTESIAN_POINT('Ctrl Pts',(3.4344663067854,1.,-2.39298338804493));
#60448=CARTESIAN_POINT('Ctrl Pts',(3.43750133064416,-1.,-2.39848113410292));
#60449=CARTESIAN_POINT('Ctrl Pts',(3.43750133064416,1.,-2.39848113410292));
#60450=CARTESIAN_POINT('Ctrl Pts',(3.43976627484234,-1.,-2.40261515589405));
#60451=CARTESIAN_POINT('Ctrl Pts',(3.43976627484234,1.,-2.40261515589405));
#60452=CARTESIAN_POINT('Ctrl Pts',(3.44127120683039,-1.,-2.4053759295909));
#60453=CARTESIAN_POINT('Ctrl Pts',(3.44127120683039,1.,-2.4053759295909));
#60454=CARTESIAN_POINT('Ctrl Pts',(3.44202241512147,-1.,-2.40675750623143));
#60455=CARTESIAN_POINT('Ctrl Pts',(3.44202241512147,1.,-2.40675750623143));
#60456=CARTESIAN_POINT('',(3.14877060440327,1.,-2.03660101169715));
#60457=CARTESIAN_POINT('Ctrl Pts',(3.14877060440327,-1.,-2.03660101169715));
#60458=CARTESIAN_POINT('Ctrl Pts',(3.14877060440327,-0.666666666666667,
-2.03660101169715));
#60459=CARTESIAN_POINT('Ctrl Pts',(3.14877060440327,-0.333333333333333,
-2.03660101169715));
#60460=CARTESIAN_POINT('Ctrl Pts',(3.14877060440327,0.333333333333333,-2.03660101169715));
#60461=CARTESIAN_POINT('Ctrl Pts',(3.14877060440328,0.666666666666667,-2.03660101169714));
#60462=CARTESIAN_POINT('Ctrl Pts',(3.14877060440328,1.,-2.03660101169714));
#60463=CARTESIAN_POINT('',(3.44202241512147,1.,-2.40675750623143));
#60464=CARTESIAN_POINT('',(3.44202241512147,0.,-2.40675750623143));
#60465=CARTESIAN_POINT('Ctrl Pts',(3.14877060440327,1.,-2.03660101169715));
#60466=CARTESIAN_POINT('Ctrl Pts',(3.14881939088124,1.,-2.03659701539259));
#60467=CARTESIAN_POINT('Ctrl Pts',(3.1490119366901,1.,-2.03663974554932));
#60468=CARTESIAN_POINT('Ctrl Pts',(3.14959882629804,1.,-2.03693188810544));
#60469=CARTESIAN_POINT('Ctrl Pts',(3.15102344775328,1.,-2.03783225495961));
#60470=CARTESIAN_POINT('Ctrl Pts',(3.15389991674792,1.,-2.03984073791519));
#60471=CARTESIAN_POINT('Ctrl Pts',(3.15817983946367,1.,-2.04297406404027));
#60472=CARTESIAN_POINT('Ctrl Pts',(3.16343165058912,1.,-2.04693331247446));
#60473=CARTESIAN_POINT('Ctrl Pts',(3.16936341689527,1.,-2.05151770247233));
#60474=CARTESIAN_POINT('Ctrl Pts',(3.17564906975371,1.,-2.05650186773132));
#60475=CARTESIAN_POINT('Ctrl Pts',(3.18197692964614,1.,-2.06166849827101));
#60476=CARTESIAN_POINT('Ctrl Pts',(3.18809755562368,1.,-2.06684062744112));
#60477=CARTESIAN_POINT('Ctrl Pts',(3.19388465568252,1.,-2.07192253497857));
#60478=CARTESIAN_POINT('Ctrl Pts',(3.19934132836019,1.,-2.07690441870722));
#60479=CARTESIAN_POINT('Ctrl Pts',(3.2045481863073,1.,-2.08182850370878));
#60480=CARTESIAN_POINT('Ctrl Pts',(3.20962575845463,1.,-2.08676465517455));
#60481=CARTESIAN_POINT('Ctrl Pts',(3.21469429601654,1.,-2.09178419460443));
#60482=CARTESIAN_POINT('Ctrl Pts',(3.21982707347009,1.,-2.09692958434895));
#60483=CARTESIAN_POINT('Ctrl Pts',(3.22503437553434,1.,-2.10220384298492));
#60484=CARTESIAN_POINT('Ctrl Pts',(3.23028945793289,1.,-2.10758699642451));
#60485=CARTESIAN_POINT('Ctrl Pts',(3.23554444767099,1.,-2.11304604021773));
#60486=CARTESIAN_POINT('Ctrl Pts',(3.24074905517293,1.,-2.11854673326979));
#60487=CARTESIAN_POINT('Ctrl Pts',(3.24587102613376,1.,-2.12406646410962));
#60488=CARTESIAN_POINT('Ctrl Pts',(3.25090574494028,1.,-2.12960028396832));
#60489=CARTESIAN_POINT('Ctrl Pts',(3.25586495065054,1.,-2.13515375878803));
#60490=CARTESIAN_POINT('Ctrl Pts',(3.26077002641879,1.,-2.14073870754264));
#60491=CARTESIAN_POINT('Ctrl Pts',(3.26564388189759,1.,-2.1463680529566));
#60492=CARTESIAN_POINT('Ctrl Pts',(3.27050245897228,1.,-2.15205043199808));
#60493=CARTESIAN_POINT('Ctrl Pts',(3.27534954469187,1.,-2.15778690038347));
#60494=CARTESIAN_POINT('Ctrl Pts',(3.280181508414,1.,-2.16357391934425));
#60495=CARTESIAN_POINT('Ctrl Pts',(3.28499019979724,1.,-2.16940517773455));
#60496=CARTESIAN_POINT('Ctrl Pts',(3.28976645712568,1.,-2.17527380048423));
#60497=CARTESIAN_POINT('Ctrl Pts',(3.2945036150049,1.,-2.18117455557065));
#60498=CARTESIAN_POINT('Ctrl Pts',(3.29920022557639,1.,-2.18710556500327));
#60499=CARTESIAN_POINT('Ctrl Pts',(3.30385816281831,1.,-2.19306710376111));
#60500=CARTESIAN_POINT('Ctrl Pts',(3.30848134694595,1.,-2.19906078949923));
#60501=CARTESIAN_POINT('Ctrl Pts',(3.31307424608949,1.,-2.20508863150607));
#60502=CARTESIAN_POINT('Ctrl Pts',(3.31764044024235,1.,-2.21115211847875));
#60503=CARTESIAN_POINT('Ctrl Pts',(3.32218125618968,1.,-2.21725135110898));
#60504=CARTESIAN_POINT('Ctrl Pts',(3.3266964672289,1.,-2.22338548312772));
#60505=CARTESIAN_POINT('Ctrl Pts',(3.33118487773611,1.,-2.22955308907233));
#60506=CARTESIAN_POINT('Ctrl Pts',(3.33564495756481,1.,-2.23575256328812));
#60507=CARTESIAN_POINT('Ctrl Pts',(3.34007543738025,1.,-2.24198249391422));
#60508=CARTESIAN_POINT('Ctrl Pts',(3.34447596770723,1.,-2.24824207678256));
#60509=CARTESIAN_POINT('Ctrl Pts',(3.34884690292285,1.,-2.25453097693483));
#60510=CARTESIAN_POINT('Ctrl Pts',(3.35318902552626,1.,-2.26084915222449));
#60511=CARTESIAN_POINT('Ctrl Pts',(3.35750328523061,1.,-2.2671966857991));
#60512=CARTESIAN_POINT('Ctrl Pts',(3.36179055004409,1.,-2.2735736262093));
#60513=CARTESIAN_POINT('Ctrl Pts',(3.36605130713076,1.,-2.27997979458037));
#60514=CARTESIAN_POINT('Ctrl Pts',(3.37028570206488,1.,-2.28641481081137));
#60515=CARTESIAN_POINT('Ctrl Pts',(3.37449367172826,1.,-2.29287818007393));
#60516=CARTESIAN_POINT('Ctrl Pts',(3.37867504959433,1.,-2.29936936127624));
#60517=CARTESIAN_POINT('Ctrl Pts',(3.3828296733661,1.,-2.30588783640343));
#60518=CARTESIAN_POINT('Ctrl Pts',(3.38695751492462,1.,-2.31243319489367));
#60519=CARTESIAN_POINT('Ctrl Pts',(3.39105869474822,1.,-2.31900513925424));
#60520=CARTESIAN_POINT('Ctrl Pts',(3.39513342019756,1.,-2.3256034390248));
#60521=CARTESIAN_POINT('Ctrl Pts',(3.39918194577956,1.,-2.33222789882489));
#60522=CARTESIAN_POINT('Ctrl Pts',(3.40320452776743,1.,-2.33887832342782));
#60523=CARTESIAN_POINT('Ctrl Pts',(3.40720137404297,1.,-2.34555447649188));
#60524=CARTESIAN_POINT('Ctrl Pts',(3.41117262314119,1.,-2.35225606824109));
#60525=CARTESIAN_POINT('Ctrl Pts',(3.41511836751469,1.,-2.35898278606946));
#60526=CARTESIAN_POINT('Ctrl Pts',(3.41903866635852,1.,-2.36573431470642));
#60527=CARTESIAN_POINT('Ctrl Pts',(3.42293356216511,1.,-2.37251035954292));
#60528=CARTESIAN_POINT('Ctrl Pts',(3.42680309754399,1.,-2.37931067028926));
#60529=CARTESIAN_POINT('Ctrl Pts',(3.43064732712919,1.,-2.38613505843552));
#60530=CARTESIAN_POINT('Ctrl Pts',(3.4344663067854,1.,-2.39298338804493));
#60531=CARTESIAN_POINT('Ctrl Pts',(3.43750133064416,1.,-2.39848113410292));
#60532=CARTESIAN_POINT('Ctrl Pts',(3.43976627484234,1.,-2.40261515589405));
#60533=CARTESIAN_POINT('Ctrl Pts',(3.44127120683039,1.,-2.4053759295909));
#60534=CARTESIAN_POINT('Ctrl Pts',(3.44202241512147,1.,-2.40675750623143));
#60535=CARTESIAN_POINT('Origin',(3.44202241512147,0.,-2.40675750623143));
#60536=CARTESIAN_POINT('',(3.35260583073571,1.,-2.52982887637028));
#60537=CARTESIAN_POINT('Origin',(0.,0.,0.));
#60538=CARTESIAN_POINT('',(3.24413672884812,1.,-1.88097764062697));
#60539=CARTESIAN_POINT('Origin',(0.,1.,0.));
#60540=CARTESIAN_POINT('Ctrl Pts',(3.24413672884812,1.,-1.88097764062697));
#60541=CARTESIAN_POINT('Ctrl Pts',(3.24413672884812,0.666666666666667,-1.88097764062697));
#60542=CARTESIAN_POINT('Ctrl Pts',(3.24413672884812,0.333333333333333,-1.88097764062697));
#60543=CARTESIAN_POINT('Ctrl Pts',(3.24413672884812,-0.333333333333333,
-1.88097764062697));
#60544=CARTESIAN_POINT('Ctrl Pts',(3.24413672884812,-0.666666666666667,
-1.88097764062697));
#60545=CARTESIAN_POINT('Ctrl Pts',(3.24413672884812,-1.,-1.88097764062697));
#60546=CARTESIAN_POINT('Ctrl Pts',(3.70708211654725,-1.,-1.97421938526992));
#60547=CARTESIAN_POINT('Ctrl Pts',(3.70708211654725,1.,-1.97421938526992));
#60548=CARTESIAN_POINT('Ctrl Pts',(3.70551008132332,-1.,-1.97417727645308));
#60549=CARTESIAN_POINT('Ctrl Pts',(3.70551008132332,1.,-1.97417727645308));
#60550=CARTESIAN_POINT('Ctrl Pts',(3.70236698912904,-1.,-1.97408973726715));
#60551=CARTESIAN_POINT('Ctrl Pts',(3.70236698912904,1.,-1.97408973726715));
#60552=CARTESIAN_POINT('Ctrl Pts',(3.6976552856004,-1.,-1.97394846383216));
#60553=CARTESIAN_POINT('Ctrl Pts',(3.6976552856004,1.,-1.97394846383216));
#60554=CARTESIAN_POINT('Ctrl Pts',(3.69137888599902,-1.,-1.97374016225483));
#60555=CARTESIAN_POINT('Ctrl Pts',(3.69137888599902,1.,-1.97374016225483));
#60556=CARTESIAN_POINT('Ctrl Pts',(3.68354319915092,-1.,-1.97344650304519));
#60557=CARTESIAN_POINT('Ctrl Pts',(3.68354319915092,1.,-1.97344650304519));
#60558=CARTESIAN_POINT('Ctrl Pts',(3.67571738107084,-1.,-1.97311947678517));
#60559=CARTESIAN_POINT('Ctrl Pts',(3.67571738107084,1.,-1.97311947678517));
#60560=CARTESIAN_POINT('Ctrl Pts',(3.66790152752075,-1.,-1.97275897198678));
#60561=CARTESIAN_POINT('Ctrl Pts',(3.66790152752075,1.,-1.97275897198678));
#60562=CARTESIAN_POINT('Ctrl Pts',(3.6600957816636,-1.,-1.9723648543905));
#60563=CARTESIAN_POINT('Ctrl Pts',(3.6600957816636,1.,-1.9723648543905));
#60564=CARTESIAN_POINT('Ctrl Pts',(3.652300347166,-1.,-1.9719369724024));
#60565=CARTESIAN_POINT('Ctrl Pts',(3.652300347166,1.,-1.9719369724024));
#60566=CARTESIAN_POINT('Ctrl Pts',(3.64451546723514,-1.,-1.97147515441164));
#60567=CARTESIAN_POINT('Ctrl Pts',(3.64451546723514,1.,-1.97147515441164));
#60568=CARTESIAN_POINT('Ctrl Pts',(3.63674139590412,-1.,-1.97097920454464));
#60569=CARTESIAN_POINT('Ctrl Pts',(3.63674139590412,1.,-1.97097920454464));
#60570=CARTESIAN_POINT('Ctrl Pts',(3.62897836973293,-1.,-1.97044889850463));
#60571=CARTESIAN_POINT('Ctrl Pts',(3.62897836973293,1.,-1.97044889850463));
#60572=CARTESIAN_POINT('Ctrl Pts',(3.62122658401893,-1.,-1.96988398129978));
#60573=CARTESIAN_POINT('Ctrl Pts',(3.62122658401893,1.,-1.96988398129978));
#60574=CARTESIAN_POINT('Ctrl Pts',(3.61348615496704,-1.,-1.96928416040877));
#60575=CARTESIAN_POINT('Ctrl Pts',(3.61348615496704,1.,-1.96928416040877));
#60576=CARTESIAN_POINT('Ctrl Pts',(3.60575714017989,-1.,-1.9686491188594));
#60577=CARTESIAN_POINT('Ctrl Pts',(3.60575714017989,1.,-1.9686491188594));
#60578=CARTESIAN_POINT('Ctrl Pts',(3.59803959819938,-1.,-1.96797854118369));
#60579=CARTESIAN_POINT('Ctrl Pts',(3.59803959819938,1.,-1.96797854118369));
#60580=CARTESIAN_POINT('Ctrl Pts',(3.59033364022801,-1.,-1.96727213799544));
#60581=CARTESIAN_POINT('Ctrl Pts',(3.59033364022801,1.,-1.96727213799544));
#60582=CARTESIAN_POINT('Ctrl Pts',(3.58263947663829,-1.,-1.96652966688911));
#60583=CARTESIAN_POINT('Ctrl Pts',(3.58263947663829,1.,-1.96652966688911));
#60584=CARTESIAN_POINT('Ctrl Pts',(3.57495748600959,-1.,-1.96575096652789));
#60585=CARTESIAN_POINT('Ctrl Pts',(3.57495748600959,1.,-1.96575096652789));
#60586=CARTESIAN_POINT('Ctrl Pts',(3.56728820357791,-1.,-1.96493594634567));
#60587=CARTESIAN_POINT('Ctrl Pts',(3.56728820357791,1.,-1.96493594634567));
#60588=CARTESIAN_POINT('Ctrl Pts',(3.55963218706096,-1.,-1.96408450906812));
#60589=CARTESIAN_POINT('Ctrl Pts',(3.55963218706096,1.,-1.96408450906812));
#60590=CARTESIAN_POINT('Ctrl Pts',(3.55198990600886,-1.,-1.96319648628644));
#60591=CARTESIAN_POINT('Ctrl Pts',(3.55198990600886,1.,-1.96319648628644));
#60592=CARTESIAN_POINT('Ctrl Pts',(3.54436163300443,-1.,-1.96227157573067));
#60593=CARTESIAN_POINT('Ctrl Pts',(3.54436163300443,1.,-1.96227157573067));
#60594=CARTESIAN_POINT('Ctrl Pts',(3.53674730625813,-1.,-1.96130926212689));
#60595=CARTESIAN_POINT('Ctrl Pts',(3.53674730625813,1.,-1.96130926212689));
#60596=CARTESIAN_POINT('Ctrl Pts',(3.52914648844351,-1.,-1.96030879411566));
#60597=CARTESIAN_POINT('Ctrl Pts',(3.52914648844351,1.,-1.96030879411566));
#60598=CARTESIAN_POINT('Ctrl Pts',(3.52155867431486,-1.,-1.95926936324461));
#60599=CARTESIAN_POINT('Ctrl Pts',(3.52155867431486,1.,-1.95926936324461));
#60600=CARTESIAN_POINT('Ctrl Pts',(3.51398354617794,-1.,-1.95819025316779));
#60601=CARTESIAN_POINT('Ctrl Pts',(3.51398354617794,1.,-1.95819025316779));
#60602=CARTESIAN_POINT('Ctrl Pts',(3.50642124159909,-1.,-1.95707099606511));
#60603=CARTESIAN_POINT('Ctrl Pts',(3.50642124159909,1.,-1.95707099606511));
#60604=CARTESIAN_POINT('Ctrl Pts',(3.49887263575583,-1.,-1.95591153823661));
#60605=CARTESIAN_POINT('Ctrl Pts',(3.49887263575583,1.,-1.95591153823661));
#60606=CARTESIAN_POINT('Ctrl Pts',(3.49133956289133,-1.,-1.95471236969643));
#60607=CARTESIAN_POINT('Ctrl Pts',(3.49133956289133,1.,-1.95471236969643));
#60608=CARTESIAN_POINT('Ctrl Pts',(3.48382414832634,-1.,-1.95347412486309));
#60609=CARTESIAN_POINT('Ctrl Pts',(3.48382414832634,1.,-1.95347412486309));
#60610=CARTESIAN_POINT('Ctrl Pts',(3.47632820495921,-1.,-1.95219722189876));
#60611=CARTESIAN_POINT('Ctrl Pts',(3.47632820495921,1.,-1.95219722189876));
#60612=CARTESIAN_POINT('Ctrl Pts',(3.46885258974191,-1.,-1.95088147859877));
#60613=CARTESIAN_POINT('Ctrl Pts',(3.46885258974191,1.,-1.95088147859877));
#60614=CARTESIAN_POINT('Ctrl Pts',(3.46139661060962,-1.,-1.94952575850197));
#60615=CARTESIAN_POINT('Ctrl Pts',(3.46139661060962,1.,-1.94952575850197));
#60616=CARTESIAN_POINT('Ctrl Pts',(3.45395731584051,-1.,-1.94812754766524));
#60617=CARTESIAN_POINT('Ctrl Pts',(3.45395731584051,1.,-1.94812754766524));
#60618=CARTESIAN_POINT('Ctrl Pts',(3.44653088665681,-1.,-1.94668377715329));
#60619=CARTESIAN_POINT('Ctrl Pts',(3.44653088665681,1.,-1.94668377715329));
#60620=CARTESIAN_POINT('Ctrl Pts',(3.43911410197687,-1.,-1.94519168842879));
#60621=CARTESIAN_POINT('Ctrl Pts',(3.43911410197687,1.,-1.94519168842879));
#60622=CARTESIAN_POINT('Ctrl Pts',(3.43170586602434,-1.,-1.94364973660284));
#60623=CARTESIAN_POINT('Ctrl Pts',(3.43170586602434,1.,-1.94364973660284));
#60624=CARTESIAN_POINT('Ctrl Pts',(3.42430850941503,-1.,-1.94205835913696));
#60625=CARTESIAN_POINT('Ctrl Pts',(3.42430850941503,1.,-1.94205835913696));
#60626=CARTESIAN_POINT('Ctrl Pts',(3.41692971994096,-1.,-1.94042111965246));
#60627=CARTESIAN_POINT('Ctrl Pts',(3.41692971994096,1.,-1.94042111965246));
#60628=CARTESIAN_POINT('Ctrl Pts',(3.40957978266642,-1.,-1.93874306008143));
#60629=CARTESIAN_POINT('Ctrl Pts',(3.40957978266642,1.,-1.93874306008143));
#60630=CARTESIAN_POINT('Ctrl Pts',(3.40226802104109,-1.,-1.93702857723098));
#60631=CARTESIAN_POINT('Ctrl Pts',(3.40226802104109,1.,-1.93702857723098));
#60632=CARTESIAN_POINT('Ctrl Pts',(3.39499923640795,-1.,-1.93527929945985));
#60633=CARTESIAN_POINT('Ctrl Pts',(3.39499923640795,1.,-1.93527929945985));
#60634=CARTESIAN_POINT('Ctrl Pts',(3.38777076883256,-1.,-1.93349233176788));
#60635=CARTESIAN_POINT('Ctrl Pts',(3.38777076883256,1.,-1.93349233176788));
#60636=CARTESIAN_POINT('Ctrl Pts',(3.3805676852555,-1.,-1.93165739093276));
#60637=CARTESIAN_POINT('Ctrl Pts',(3.3805676852555,1.,-1.93165739093276));
#60638=CARTESIAN_POINT('Ctrl Pts',(3.37336807068043,-1.,-1.92975993109877));
#60639=CARTESIAN_POINT('Ctrl Pts',(3.37336807068043,1.,-1.92975993109877));
#60640=CARTESIAN_POINT('Ctrl Pts',(3.36615168657567,-1.,-1.92778626543786));
#60641=CARTESIAN_POINT('Ctrl Pts',(3.36615168657567,1.,-1.92778626543786));
#60642=CARTESIAN_POINT('Ctrl Pts',(3.35890824422965,-1.,-1.92572846125756));
#60643=CARTESIAN_POINT('Ctrl Pts',(3.35890824422965,1.,-1.92572846125756));
#60644=CARTESIAN_POINT('Ctrl Pts',(3.35164424847223,-1.,-1.92358838440528));
#60645=CARTESIAN_POINT('Ctrl Pts',(3.35164424847223,1.,-1.92358838440528));
#60646=CARTESIAN_POINT('Ctrl Pts',(3.34439448941961,-1.,-1.92138450828404));
#60647=CARTESIAN_POINT('Ctrl Pts',(3.34439448941961,1.,-1.92138450828404));
#60648=CARTESIAN_POINT('Ctrl Pts',(3.33721230710012,-1.,-1.9191460961021));
#60649=CARTESIAN_POINT('Ctrl Pts',(3.33721230710012,1.,-1.9191460961021));
#60650=CARTESIAN_POINT('Ctrl Pts',(3.33014884257873,-1.,-1.91690081930332));
#60651=CARTESIAN_POINT('Ctrl Pts',(3.33014884257873,1.,-1.91690081930332));
#60652=CARTESIAN_POINT('Ctrl Pts',(3.32323403454535,-1.,-1.91466343916628));
#60653=CARTESIAN_POINT('Ctrl Pts',(3.32323403454535,1.,-1.91466343916628));
#60654=CARTESIAN_POINT('Ctrl Pts',(3.31646052426364,-1.,-1.91242616234442));
#60655=CARTESIAN_POINT('Ctrl Pts',(3.31646052426364,1.,-1.91242616234442));
#60656=CARTESIAN_POINT('Ctrl Pts',(3.30975721158596,-1.,-1.91014297830446));
#60657=CARTESIAN_POINT('Ctrl Pts',(3.30975721158596,1.,-1.91014297830446));
#60658=CARTESIAN_POINT('Ctrl Pts',(3.30300595568195,-1.,-1.90773912171341));
#60659=CARTESIAN_POINT('Ctrl Pts',(3.30300595568195,1.,-1.90773912171341));
#60660=CARTESIAN_POINT('Ctrl Pts',(3.29608978722113,-1.,-1.90513891864087));
#60661=CARTESIAN_POINT('Ctrl Pts',(3.29608978722113,1.,-1.90513891864087));
#60662=CARTESIAN_POINT('Ctrl Pts',(3.2889344860029,-1.,-1.90228971247527));
#60663=CARTESIAN_POINT('Ctrl Pts',(3.2889344860029,1.,-1.90228971247527));
#60664=CARTESIAN_POINT('Ctrl Pts',(3.28154737912352,-1.,-1.89918429230462));
#60665=CARTESIAN_POINT('Ctrl Pts',(3.28154737912352,1.,-1.89918429230462));
#60666=CARTESIAN_POINT('Ctrl Pts',(3.27407108933139,-1.,-1.89589172903793));
#60667=CARTESIAN_POINT('Ctrl Pts',(3.27407108933139,1.,-1.89589172903793));
#60668=CARTESIAN_POINT('Ctrl Pts',(3.26677653888676,-1.,-1.89255393500965));
#60669=CARTESIAN_POINT('Ctrl Pts',(3.26677653888676,1.,-1.89255393500965));
#60670=CARTESIAN_POINT('Ctrl Pts',(3.25999885193947,-1.,-1.88934996203698));
#60671=CARTESIAN_POINT('Ctrl Pts',(3.25999885193947,1.,-1.88934996203698));
#60672=CARTESIAN_POINT('Ctrl Pts',(3.25408686339463,-1.,-1.88646802523466));
#60673=CARTESIAN_POINT('Ctrl Pts',(3.25408686339463,1.,-1.88646802523466));
#60674=CARTESIAN_POINT('Ctrl Pts',(3.24935200511918,-1.,-1.88407708646357));
#60675=CARTESIAN_POINT('Ctrl Pts',(3.24935200511918,1.,-1.88407708646357));
#60676=CARTESIAN_POINT('Ctrl Pts',(3.24600543790443,-1.,-1.88229202582941));
#60677=CARTESIAN_POINT('Ctrl Pts',(3.24600543790443,1.,-1.88229202582941));
#60678=CARTESIAN_POINT('Ctrl Pts',(3.24451807186481,-1.,-1.88139187908074));
#60679=CARTESIAN_POINT('Ctrl Pts',(3.24451807186481,1.,-1.88139187908074));
#60680=CARTESIAN_POINT('Ctrl Pts',(3.24408699284121,-1.,-1.88102201872555));
#60681=CARTESIAN_POINT('Ctrl Pts',(3.24408699284121,1.,-1.88102201872555));
#60682=CARTESIAN_POINT('Ctrl Pts',(3.24410359189609,-1.,-1.88091100680349));
#60683=CARTESIAN_POINT('Ctrl Pts',(3.24410359189609,1.,-1.88091100680349));
#60684=CARTESIAN_POINT('Ctrl Pts',(3.24418789321065,-1.,-1.8808893942881));
#60685=CARTESIAN_POINT('Ctrl Pts',(3.24418789321065,1.,-1.8808893942881));
#60686=CARTESIAN_POINT('',(3.70708211654725,1.,-1.97421938526992));
#60687=CARTESIAN_POINT('Ctrl Pts',(3.70708211654725,1.,-1.97421938526992));
#60688=CARTESIAN_POINT('Ctrl Pts',(3.70551008132332,1.,-1.97417727645308));
#60689=CARTESIAN_POINT('Ctrl Pts',(3.70236698912904,1.,-1.97408973726715));
#60690=CARTESIAN_POINT('Ctrl Pts',(3.6976552856004,1.,-1.97394846383216));
#60691=CARTESIAN_POINT('Ctrl Pts',(3.69137888599902,1.,-1.97374016225483));
#60692=CARTESIAN_POINT('Ctrl Pts',(3.68354319915092,1.,-1.97344650304519));
#60693=CARTESIAN_POINT('Ctrl Pts',(3.67571738107084,1.,-1.97311947678517));
#60694=CARTESIAN_POINT('Ctrl Pts',(3.66790152752075,1.,-1.97275897198678));
#60695=CARTESIAN_POINT('Ctrl Pts',(3.6600957816636,1.,-1.9723648543905));
#60696=CARTESIAN_POINT('Ctrl Pts',(3.652300347166,1.,-1.9719369724024));
#60697=CARTESIAN_POINT('Ctrl Pts',(3.64451546723514,1.,-1.97147515441164));
#60698=CARTESIAN_POINT('Ctrl Pts',(3.63674139590412,1.,-1.97097920454464));
#60699=CARTESIAN_POINT('Ctrl Pts',(3.62897836973293,1.,-1.97044889850463));
#60700=CARTESIAN_POINT('Ctrl Pts',(3.62122658401893,1.,-1.96988398129978));
#60701=CARTESIAN_POINT('Ctrl Pts',(3.61348615496704,1.,-1.96928416040877));
#60702=CARTESIAN_POINT('Ctrl Pts',(3.60575714017989,1.,-1.9686491188594));
#60703=CARTESIAN_POINT('Ctrl Pts',(3.59803959819938,1.,-1.96797854118369));
#60704=CARTESIAN_POINT('Ctrl Pts',(3.59033364022801,1.,-1.96727213799544));
#60705=CARTESIAN_POINT('Ctrl Pts',(3.58263947663829,1.,-1.96652966688911));
#60706=CARTESIAN_POINT('Ctrl Pts',(3.57495748600959,1.,-1.96575096652789));
#60707=CARTESIAN_POINT('Ctrl Pts',(3.56728820357791,1.,-1.96493594634567));
#60708=CARTESIAN_POINT('Ctrl Pts',(3.55963218706096,1.,-1.96408450906812));
#60709=CARTESIAN_POINT('Ctrl Pts',(3.55198990600886,1.,-1.96319648628644));
#60710=CARTESIAN_POINT('Ctrl Pts',(3.54436163300443,1.,-1.96227157573067));
#60711=CARTESIAN_POINT('Ctrl Pts',(3.53674730625813,1.,-1.96130926212689));
#60712=CARTESIAN_POINT('Ctrl Pts',(3.52914648844351,1.,-1.96030879411566));
#60713=CARTESIAN_POINT('Ctrl Pts',(3.52155867431486,1.,-1.95926936324461));
#60714=CARTESIAN_POINT('Ctrl Pts',(3.51398354617794,1.,-1.95819025316779));
#60715=CARTESIAN_POINT('Ctrl Pts',(3.50642124159909,1.,-1.95707099606511));
#60716=CARTESIAN_POINT('Ctrl Pts',(3.49887263575583,1.,-1.95591153823661));
#60717=CARTESIAN_POINT('Ctrl Pts',(3.49133956289133,1.,-1.95471236969643));
#60718=CARTESIAN_POINT('Ctrl Pts',(3.48382414832634,1.,-1.95347412486309));
#60719=CARTESIAN_POINT('Ctrl Pts',(3.47632820495921,1.,-1.95219722189876));
#60720=CARTESIAN_POINT('Ctrl Pts',(3.46885258974191,1.,-1.95088147859877));
#60721=CARTESIAN_POINT('Ctrl Pts',(3.46139661060962,1.,-1.94952575850197));
#60722=CARTESIAN_POINT('Ctrl Pts',(3.45395731584051,1.,-1.94812754766524));
#60723=CARTESIAN_POINT('Ctrl Pts',(3.44653088665681,1.,-1.94668377715329));
#60724=CARTESIAN_POINT('Ctrl Pts',(3.43911410197687,1.,-1.94519168842879));
#60725=CARTESIAN_POINT('Ctrl Pts',(3.43170586602434,1.,-1.94364973660284));
#60726=CARTESIAN_POINT('Ctrl Pts',(3.42430850941503,1.,-1.94205835913696));
#60727=CARTESIAN_POINT('Ctrl Pts',(3.41692971994096,1.,-1.94042111965246));
#60728=CARTESIAN_POINT('Ctrl Pts',(3.40957978266642,1.,-1.93874306008143));
#60729=CARTESIAN_POINT('Ctrl Pts',(3.40226802104109,1.,-1.93702857723098));
#60730=CARTESIAN_POINT('Ctrl Pts',(3.39499923640795,1.,-1.93527929945985));
#60731=CARTESIAN_POINT('Ctrl Pts',(3.38777076883256,1.,-1.93349233176788));
#60732=CARTESIAN_POINT('Ctrl Pts',(3.3805676852555,1.,-1.93165739093276));
#60733=CARTESIAN_POINT('Ctrl Pts',(3.37336807068043,1.,-1.92975993109877));
#60734=CARTESIAN_POINT('Ctrl Pts',(3.36615168657567,1.,-1.92778626543786));
#60735=CARTESIAN_POINT('Ctrl Pts',(3.35890824422965,1.,-1.92572846125756));
#60736=CARTESIAN_POINT('Ctrl Pts',(3.35164424847223,1.,-1.92358838440528));
#60737=CARTESIAN_POINT('Ctrl Pts',(3.34439448941961,1.,-1.92138450828404));
#60738=CARTESIAN_POINT('Ctrl Pts',(3.33721230710012,1.,-1.9191460961021));
#60739=CARTESIAN_POINT('Ctrl Pts',(3.33014884257873,1.,-1.91690081930332));
#60740=CARTESIAN_POINT('Ctrl Pts',(3.32323403454535,1.,-1.91466343916628));
#60741=CARTESIAN_POINT('Ctrl Pts',(3.31646052426364,1.,-1.91242616234442));
#60742=CARTESIAN_POINT('Ctrl Pts',(3.30975721158596,1.,-1.91014297830446));
#60743=CARTESIAN_POINT('Ctrl Pts',(3.30300595568195,1.,-1.90773912171341));
#60744=CARTESIAN_POINT('Ctrl Pts',(3.29608978722113,1.,-1.90513891864087));
#60745=CARTESIAN_POINT('Ctrl Pts',(3.2889344860029,1.,-1.90228971247527));
#60746=CARTESIAN_POINT('Ctrl Pts',(3.28154737912352,1.,-1.89918429230462));
#60747=CARTESIAN_POINT('Ctrl Pts',(3.27407108933139,1.,-1.89589172903793));
#60748=CARTESIAN_POINT('Ctrl Pts',(3.26677653888676,1.,-1.89255393500965));
#60749=CARTESIAN_POINT('Ctrl Pts',(3.25999885193947,1.,-1.88934996203698));
#60750=CARTESIAN_POINT('Ctrl Pts',(3.25408686339463,1.,-1.88646802523466));
#60751=CARTESIAN_POINT('Ctrl Pts',(3.24935200511918,1.,-1.88407708646357));
#60752=CARTESIAN_POINT('Ctrl Pts',(3.2462565441079,1.,-1.88242596600454));
#60753=CARTESIAN_POINT('Ctrl Pts',(3.24480754676064,1.,-1.88156537699203));
#60754=CARTESIAN_POINT('Ctrl Pts',(3.24428080353022,1.,-1.88117508446775));
#60755=CARTESIAN_POINT('Ctrl Pts',(3.24415531671284,1.,-1.8810229239812));
#60756=CARTESIAN_POINT('Ctrl Pts',(3.24413672884812,1.,-1.88097764062697));
#60757=CARTESIAN_POINT('',(3.70708211654725,0.,-1.97421938526992));
#60758=CARTESIAN_POINT('Ctrl Pts',(3.42855728381368,-1.,-1.519044091397));
#60759=CARTESIAN_POINT('Ctrl Pts',(3.42855728381368,1.,-1.519044091397));
#60760=CARTESIAN_POINT('Ctrl Pts',(3.42852521763778,-1.,-1.51896318668366));
#60761=CARTESIAN_POINT('Ctrl Pts',(3.42852521763778,1.,-1.51896318668366));
#60762=CARTESIAN_POINT('Ctrl Pts',(3.42860527149177,-1.,-1.51888450659652));
#60763=CARTESIAN_POINT('Ctrl Pts',(3.42860527149177,1.,-1.51888450659652));
#60764=CARTESIAN_POINT('Ctrl Pts',(3.42915787669893,-1.,-1.51901585839109));
#60765=CARTESIAN_POINT('Ctrl Pts',(3.42915787669893,1.,-1.51901585839109));
#60766=CARTESIAN_POINT('Ctrl Pts',(3.43076036253837,-1.,-1.51969006980999));
#60767=CARTESIAN_POINT('Ctrl Pts',(3.43076036253837,1.,-1.51969006980999));
#60768=CARTESIAN_POINT('Ctrl Pts',(3.43417156977893,-1.,-1.52134826724293));
#60769=CARTESIAN_POINT('Ctrl Pts',(3.43417156977893,1.,-1.52134826724293));
#60770=CARTESIAN_POINT('Ctrl Pts',(3.4388889597401,-1.,-1.5237734895035));
#60771=CARTESIAN_POINT('Ctrl Pts',(3.4388889597401,1.,-1.5237734895035));
#60772=CARTESIAN_POINT('Ctrl Pts',(3.44469547526647,-1.,-1.52686242875556));
#60773=CARTESIAN_POINT('Ctrl Pts',(3.44469547526647,1.,-1.52686242875556));
#60774=CARTESIAN_POINT('Ctrl Pts',(3.45127136828305,-1.,-1.53046244461635));
#60775=CARTESIAN_POINT('Ctrl Pts',(3.45127136828305,1.,-1.53046244461635));
#60776=CARTESIAN_POINT('Ctrl Pts',(3.45825932955032,-1.,-1.53440195378792));
#60777=CARTESIAN_POINT('Ctrl Pts',(3.45825932955032,1.,-1.53440195378792));
#60778=CARTESIAN_POINT('Ctrl Pts',(3.46531752207153,-1.,-1.53851507915502));
#60779=CARTESIAN_POINT('Ctrl Pts',(3.46531752207153,1.,-1.53851507915502));
#60780=CARTESIAN_POINT('Ctrl Pts',(3.47217189224653,-1.,-1.54266605398188));
#60781=CARTESIAN_POINT('Ctrl Pts',(3.47217189224653,1.,-1.54266605398188));
#60782=CARTESIAN_POINT('Ctrl Pts',(3.47868272898751,-1.,-1.54678009290276));
#60783=CARTESIAN_POINT('Ctrl Pts',(3.47868272898751,1.,-1.54678009290276));
#60784=CARTESIAN_POINT('Ctrl Pts',(3.48485155928567,-1.,-1.55084702970452));
#60785=CARTESIAN_POINT('Ctrl Pts',(3.48485155928567,1.,-1.55084702970452));
#60786=CARTESIAN_POINT('Ctrl Pts',(3.4907646087742,-1.,-1.55489595901116));
#60787=CARTESIAN_POINT('Ctrl Pts',(3.4907646087742,1.,-1.55489595901116));
#60788=CARTESIAN_POINT('Ctrl Pts',(3.49655185179655,-1.,-1.55897703097874));
#60789=CARTESIAN_POINT('Ctrl Pts',(3.49655185179655,1.,-1.55897703097874));
#60790=CARTESIAN_POINT('Ctrl Pts',(3.50234321621578,-1.,-1.56314187758675));
#60791=CARTESIAN_POINT('Ctrl Pts',(3.50234321621578,1.,-1.56314187758675));
#60792=CARTESIAN_POINT('Ctrl Pts',(3.50821771695363,-1.,-1.56742097575012));
#60793=CARTESIAN_POINT('Ctrl Pts',(3.50821771695363,1.,-1.56742097575012));
#60794=CARTESIAN_POINT('Ctrl Pts',(3.51418598431665,-1.,-1.57181569799743));
#60795=CARTESIAN_POINT('Ctrl Pts',(3.51418598431665,1.,-1.57181569799743));
#60796=CARTESIAN_POINT('Ctrl Pts',(3.52021847865912,-1.,-1.57631049988158));
#60797=CARTESIAN_POINT('Ctrl Pts',(3.52021847865912,1.,-1.57631049988158));
#60798=CARTESIAN_POINT('Ctrl Pts',(3.52626275334881,-1.,-1.58088027227848));
#60799=CARTESIAN_POINT('Ctrl Pts',(3.52626275334881,1.,-1.58088027227848));
#60800=CARTESIAN_POINT('Ctrl Pts',(3.5322637814708,-1.,-1.58549906268088));
#60801=CARTESIAN_POINT('Ctrl Pts',(3.5322637814708,1.,-1.58549906268088));
#60802=CARTESIAN_POINT('Ctrl Pts',(3.53818616861077,-1.,-1.59014958368739));
#60803=CARTESIAN_POINT('Ctrl Pts',(3.53818616861077,1.,-1.59014958368739));
#60804=CARTESIAN_POINT('Ctrl Pts',(3.54402458182337,-1.,-1.59482766949766));
#60805=CARTESIAN_POINT('Ctrl Pts',(3.54402458182337,1.,-1.59482766949766));
#60806=CARTESIAN_POINT('Ctrl Pts',(3.54979148634454,-1.,-1.59953698113457));
#60807=CARTESIAN_POINT('Ctrl Pts',(3.54979148634454,1.,-1.59953698113457));
#60808=CARTESIAN_POINT('Ctrl Pts',(3.55550985096129,-1.,-1.60428584699853));
#60809=CARTESIAN_POINT('Ctrl Pts',(3.55550985096129,1.,-1.60428584699853));
#60810=CARTESIAN_POINT('Ctrl Pts',(3.5612043248298,-1.,-1.60908344685457));
#60811=CARTESIAN_POINT('Ctrl Pts',(3.5612043248298,1.,-1.60908344685457));
#60812=CARTESIAN_POINT('Ctrl Pts',(3.56689200468387,-1.,-1.61393581747514));
#60813=CARTESIAN_POINT('Ctrl Pts',(3.56689200468387,1.,-1.61393581747514));
#60814=CARTESIAN_POINT('Ctrl Pts',(3.57257679609806,-1.,-1.61884340915404));
#60815=CARTESIAN_POINT('Ctrl Pts',(3.57257679609806,1.,-1.61884340915404));
#60816=CARTESIAN_POINT('Ctrl Pts',(3.5782545595439,-1.,-1.62380329464844));
#60817=CARTESIAN_POINT('Ctrl Pts',(3.5782545595439,1.,-1.62380329464844));
#60818=CARTESIAN_POINT('Ctrl Pts',(3.58391625774343,-1.,-1.62881051550745));
#60819=CARTESIAN_POINT('Ctrl Pts',(3.58391625774343,1.,-1.62881051550745));
#60820=CARTESIAN_POINT('Ctrl Pts',(3.58955176627879,-1.,-1.6338597145126));
#60821=CARTESIAN_POINT('Ctrl Pts',(3.58955176627879,1.,-1.6338597145126));
#60822=CARTESIAN_POINT('Ctrl Pts',(3.59515368334893,-1.,-1.63894676675352));
#60823=CARTESIAN_POINT('Ctrl Pts',(3.59515368334893,1.,-1.63894676675352));
#60824=CARTESIAN_POINT('Ctrl Pts',(3.60072028513845,-1.,-1.64407004385582));
#60825=CARTESIAN_POINT('Ctrl Pts',(3.60072028513845,1.,-1.64407004385582));
#60826=CARTESIAN_POINT('Ctrl Pts',(3.60625346556992,-1.,-1.64922952425832));
#60827=CARTESIAN_POINT('Ctrl Pts',(3.60625346556992,1.,-1.64922952425832));
#60828=CARTESIAN_POINT('Ctrl Pts',(3.61175734965127,-1.,-1.65442619244325));
#60829=CARTESIAN_POINT('Ctrl Pts',(3.61175734965127,1.,-1.65442619244325));
#60830=CARTESIAN_POINT('Ctrl Pts',(3.61723666482456,-1.,-1.65966133399186));
#60831=CARTESIAN_POINT('Ctrl Pts',(3.61723666482456,1.,-1.65966133399186));
#60832=CARTESIAN_POINT('Ctrl Pts',(3.62269517989109,-1.,-1.66493585923855));
#60833=CARTESIAN_POINT('Ctrl Pts',(3.62269517989109,1.,-1.66493585923855));
#60834=CARTESIAN_POINT('Ctrl Pts',(3.62813422105271,-1.,-1.67024966008045));
#60835=CARTESIAN_POINT('Ctrl Pts',(3.62813422105271,1.,-1.67024966008045));
#60836=CARTESIAN_POINT('Ctrl Pts',(3.63355343201232,-1.,-1.67560193613156));
#60837=CARTESIAN_POINT('Ctrl Pts',(3.63355343201232,1.,-1.67560193613156));
#60838=CARTESIAN_POINT('Ctrl Pts',(3.63895140887462,-1.,-1.68099146651586));
#60839=CARTESIAN_POINT('Ctrl Pts',(3.63895140887462,1.,-1.68099146651586));
#60840=CARTESIAN_POINT('Ctrl Pts',(3.64432638915203,-1.,-1.68641690471457));
#60841=CARTESIAN_POINT('Ctrl Pts',(3.64432638915203,1.,-1.68641690471457));
#60842=CARTESIAN_POINT('Ctrl Pts',(3.64967689827371,-1.,-1.69187705481689));
#60843=CARTESIAN_POINT('Ctrl Pts',(3.64967689827371,1.,-1.69187705481689));
#60844=CARTESIAN_POINT('Ctrl Pts',(3.65500246526749,-1.,-1.69737117722534));
#60845=CARTESIAN_POINT('Ctrl Pts',(3.65500246526749,1.,-1.69737117722534));
#60846=CARTESIAN_POINT('Ctrl Pts',(3.66030338774847,-1.,-1.70289888566873));
#60847=CARTESIAN_POINT('Ctrl Pts',(3.66030338774847,1.,-1.70289888566873));
#60848=CARTESIAN_POINT('Ctrl Pts',(3.66558043198876,-1.,-1.70846001610956));
#60849=CARTESIAN_POINT('Ctrl Pts',(3.66558043198876,1.,-1.70846001610956));
#60850=CARTESIAN_POINT('Ctrl Pts',(3.67083454901611,-1.,-1.71405450210384));
#60851=CARTESIAN_POINT('Ctrl Pts',(3.67083454901611,1.,-1.71405450210384));
#60852=CARTESIAN_POINT('Ctrl Pts',(3.67606660374709,-1.,-1.71968225581808));
#60853=CARTESIAN_POINT('Ctrl Pts',(3.67606660374709,1.,-1.71968225581808));
#60854=CARTESIAN_POINT('Ctrl Pts',(3.68127704936579,-1.,-1.72534302437056));
#60855=CARTESIAN_POINT('Ctrl Pts',(3.68127704936579,1.,-1.72534302437056));
#60856=CARTESIAN_POINT('Ctrl Pts',(3.68646597019332,-1.,-1.73103640956717));
#60857=CARTESIAN_POINT('Ctrl Pts',(3.68646597019332,1.,-1.73103640956717));
#60858=CARTESIAN_POINT('Ctrl Pts',(3.69163322648036,-1.,-1.73676193254557));
#60859=CARTESIAN_POINT('Ctrl Pts',(3.69163322648036,1.,-1.73676193254557));
#60860=CARTESIAN_POINT('Ctrl Pts',(3.69677856910517,-1.,-1.74251908492617));
#60861=CARTESIAN_POINT('Ctrl Pts',(3.69677856910517,1.,-1.74251908492617));
#60862=CARTESIAN_POINT('Ctrl Pts',(3.7019017567335,-1.,-1.74830738046057));
#60863=CARTESIAN_POINT('Ctrl Pts',(3.7019017567335,1.,-1.74830738046057));
#60864=CARTESIAN_POINT('Ctrl Pts',(3.70700269736659,-1.,-1.75412641804042));
#60865=CARTESIAN_POINT('Ctrl Pts',(3.70700269736659,1.,-1.75412641804042));
#60866=CARTESIAN_POINT('Ctrl Pts',(3.71208146346136,-1.,-1.75997588498865));
#60867=CARTESIAN_POINT('Ctrl Pts',(3.71208146346136,1.,-1.75997588498865));
#60868=CARTESIAN_POINT('Ctrl Pts',(3.71713822377359,-1.,-1.76585552124394));
#60869=CARTESIAN_POINT('Ctrl Pts',(3.71713822377359,1.,-1.76585552124394));
#60870=CARTESIAN_POINT('Ctrl Pts',(3.72217319911254,-1.,-1.77176509401761));
#60871=CARTESIAN_POINT('Ctrl Pts',(3.72217319911254,1.,-1.77176509401761));
#60872=CARTESIAN_POINT('Ctrl Pts',(3.72718661205609,-1.,-1.77770437039658));
#60873=CARTESIAN_POINT('Ctrl Pts',(3.72718661205609,1.,-1.77770437039658));
#60874=CARTESIAN_POINT('Ctrl Pts',(3.7321786309547,-1.,-1.78367308442901));
#60875=CARTESIAN_POINT('Ctrl Pts',(3.7321786309547,1.,-1.78367308442901));
#60876=CARTESIAN_POINT('Ctrl Pts',(3.73714934730681,-1.,-1.78967092823491));
#60877=CARTESIAN_POINT('Ctrl Pts',(3.73714934730681,1.,-1.78967092823491));
#60878=CARTESIAN_POINT('Ctrl Pts',(3.74209880352445,-1.,-1.79569757859422));
#60879=CARTESIAN_POINT('Ctrl Pts',(3.74209880352445,1.,-1.79569757859422));
#60880=CARTESIAN_POINT('Ctrl Pts',(3.74702700875467,-1.,-1.8017527148577));
#60881=CARTESIAN_POINT('Ctrl Pts',(3.74702700875467,1.,-1.8017527148577));
#60882=CARTESIAN_POINT('Ctrl Pts',(3.75193395887977,-1.,-1.80783603939617));
#60883=CARTESIAN_POINT('Ctrl Pts',(3.75193395887977,1.,-1.80783603939617));
#60884=CARTESIAN_POINT('Ctrl Pts',(3.75681965683071,-1.,-1.8139472983358));
#60885=CARTESIAN_POINT('Ctrl Pts',(3.75681965683071,1.,-1.8139472983358));
#60886=CARTESIAN_POINT('Ctrl Pts',(3.76168412707948,-1.,-1.82008629694091));
#60887=CARTESIAN_POINT('Ctrl Pts',(3.76168412707948,1.,-1.82008629694091));
#60888=CARTESIAN_POINT('Ctrl Pts',(3.76652740353775,-1.,-1.82625289220915));
#60889=CARTESIAN_POINT('Ctrl Pts',(3.76652740353775,1.,-1.82625289220915));
#60890=CARTESIAN_POINT('Ctrl Pts',(3.77038509817999,-1.,-1.83120816955646));
#60891=CARTESIAN_POINT('Ctrl Pts',(3.77038509817999,1.,-1.83120816955646));
#60892=CARTESIAN_POINT('Ctrl Pts',(3.77326886064398,-1.,-1.83493697934534));
#60893=CARTESIAN_POINT('Ctrl Pts',(3.77326886064398,1.,-1.83493697934534));
#60894=CARTESIAN_POINT('Ctrl Pts',(3.77518714457833,-1.,-1.83742834010626));
#60895=CARTESIAN_POINT('Ctrl Pts',(3.77518714457833,1.,-1.83742834010626));
#60896=CARTESIAN_POINT('Ctrl Pts',(3.77614523045147,-1.,-1.83867539237861));
#60897=CARTESIAN_POINT('Ctrl Pts',(3.77614523045147,1.,-1.83867539237861));
#60898=CARTESIAN_POINT('',(3.42859860294306,1.,-1.5189508286633));
#60899=CARTESIAN_POINT('Ctrl Pts',(3.42859860294306,-1.,-1.5189508286633));
#60900=CARTESIAN_POINT('Ctrl Pts',(3.42859860294306,-0.666666666666667,
-1.5189508286633));
#60901=CARTESIAN_POINT('Ctrl Pts',(3.42859860294306,-0.333333333333333,
-1.5189508286633));
#60902=CARTESIAN_POINT('Ctrl Pts',(3.42859860294306,0.333333333333333,-1.5189508286633));
#60903=CARTESIAN_POINT('Ctrl Pts',(3.42859860294306,0.666666666666667,-1.5189508286633));
#60904=CARTESIAN_POINT('Ctrl Pts',(3.42859860294306,1.,-1.5189508286633));
#60905=CARTESIAN_POINT('',(3.77614523045147,1.,-1.83867539237861));
#60906=CARTESIAN_POINT('',(3.77614523045147,0.,-1.83867539237861));
#60907=CARTESIAN_POINT('Ctrl Pts',(3.42859860294306,1.,-1.5189508286633));
#60908=CARTESIAN_POINT('Ctrl Pts',(3.42864616361875,1.,-1.51893924967331));
#60909=CARTESIAN_POINT('Ctrl Pts',(3.42884302333841,1.,-1.5189513329503));
#60910=CARTESIAN_POINT('Ctrl Pts',(3.42946838852588,1.,-1.51914806898491));
#60911=CARTESIAN_POINT('Ctrl Pts',(3.43101631893414,1.,-1.5198144909338));
#60912=CARTESIAN_POINT('Ctrl Pts',(3.43417156977893,1.,-1.52134826724293));
#60913=CARTESIAN_POINT('Ctrl Pts',(3.4388889597401,1.,-1.5237734895035));
#60914=CARTESIAN_POINT('Ctrl Pts',(3.44469547526647,1.,-1.52686242875556));
#60915=CARTESIAN_POINT('Ctrl Pts',(3.45127136828305,1.,-1.53046244461635));
#60916=CARTESIAN_POINT('Ctrl Pts',(3.45825932955032,1.,-1.53440195378792));
#60917=CARTESIAN_POINT('Ctrl Pts',(3.46531752207153,1.,-1.53851507915502));
#60918=CARTESIAN_POINT('Ctrl Pts',(3.47217189224653,1.,-1.54266605398188));
#60919=CARTESIAN_POINT('Ctrl Pts',(3.47868272898751,1.,-1.54678009290276));
#60920=CARTESIAN_POINT('Ctrl Pts',(3.48485155928567,1.,-1.55084702970452));
#60921=CARTESIAN_POINT('Ctrl Pts',(3.4907646087742,1.,-1.55489595901116));
#60922=CARTESIAN_POINT('Ctrl Pts',(3.49655185179655,1.,-1.55897703097874));
#60923=CARTESIAN_POINT('Ctrl Pts',(3.50234321621578,1.,-1.56314187758675));
#60924=CARTESIAN_POINT('Ctrl Pts',(3.50821771695363,1.,-1.56742097575012));
#60925=CARTESIAN_POINT('Ctrl Pts',(3.51418598431665,1.,-1.57181569799743));
#60926=CARTESIAN_POINT('Ctrl Pts',(3.52021847865912,1.,-1.57631049988158));
#60927=CARTESIAN_POINT('Ctrl Pts',(3.52626275334881,1.,-1.58088027227848));
#60928=CARTESIAN_POINT('Ctrl Pts',(3.5322637814708,1.,-1.58549906268088));
#60929=CARTESIAN_POINT('Ctrl Pts',(3.53818616861077,1.,-1.59014958368739));
#60930=CARTESIAN_POINT('Ctrl Pts',(3.54402458182337,1.,-1.59482766949766));
#60931=CARTESIAN_POINT('Ctrl Pts',(3.54979148634454,1.,-1.59953698113457));
#60932=CARTESIAN_POINT('Ctrl Pts',(3.55550985096129,1.,-1.60428584699853));
#60933=CARTESIAN_POINT('Ctrl Pts',(3.5612043248298,1.,-1.60908344685457));
#60934=CARTESIAN_POINT('Ctrl Pts',(3.56689200468387,1.,-1.61393581747514));
#60935=CARTESIAN_POINT('Ctrl Pts',(3.57257679609806,1.,-1.61884340915404));
#60936=CARTESIAN_POINT('Ctrl Pts',(3.5782545595439,1.,-1.62380329464844));
#60937=CARTESIAN_POINT('Ctrl Pts',(3.58391625774343,1.,-1.62881051550745));
#60938=CARTESIAN_POINT('Ctrl Pts',(3.58955176627879,1.,-1.6338597145126));
#60939=CARTESIAN_POINT('Ctrl Pts',(3.59515368334893,1.,-1.63894676675352));
#60940=CARTESIAN_POINT('Ctrl Pts',(3.60072028513845,1.,-1.64407004385582));
#60941=CARTESIAN_POINT('Ctrl Pts',(3.60625346556992,1.,-1.64922952425832));
#60942=CARTESIAN_POINT('Ctrl Pts',(3.61175734965127,1.,-1.65442619244325));
#60943=CARTESIAN_POINT('Ctrl Pts',(3.61723666482456,1.,-1.65966133399186));
#60944=CARTESIAN_POINT('Ctrl Pts',(3.62269517989109,1.,-1.66493585923855));
#60945=CARTESIAN_POINT('Ctrl Pts',(3.62813422105271,1.,-1.67024966008045));
#60946=CARTESIAN_POINT('Ctrl Pts',(3.63355343201232,1.,-1.67560193613156));
#60947=CARTESIAN_POINT('Ctrl Pts',(3.63895140887462,1.,-1.68099146651586));
#60948=CARTESIAN_POINT('Ctrl Pts',(3.64432638915203,1.,-1.68641690471457));
#60949=CARTESIAN_POINT('Ctrl Pts',(3.64967689827371,1.,-1.69187705481689));
#60950=CARTESIAN_POINT('Ctrl Pts',(3.65500246526749,1.,-1.69737117722534));
#60951=CARTESIAN_POINT('Ctrl Pts',(3.66030338774847,1.,-1.70289888566873));
#60952=CARTESIAN_POINT('Ctrl Pts',(3.66558043198876,1.,-1.70846001610956));
#60953=CARTESIAN_POINT('Ctrl Pts',(3.67083454901611,1.,-1.71405450210384));
#60954=CARTESIAN_POINT('Ctrl Pts',(3.67606660374709,1.,-1.71968225581808));
#60955=CARTESIAN_POINT('Ctrl Pts',(3.68127704936579,1.,-1.72534302437056));
#60956=CARTESIAN_POINT('Ctrl Pts',(3.68646597019332,1.,-1.73103640956717));
#60957=CARTESIAN_POINT('Ctrl Pts',(3.69163322648036,1.,-1.73676193254557));
#60958=CARTESIAN_POINT('Ctrl Pts',(3.69677856910517,1.,-1.74251908492617));
#60959=CARTESIAN_POINT('Ctrl Pts',(3.7019017567335,1.,-1.74830738046057));
#60960=CARTESIAN_POINT('Ctrl Pts',(3.70700269736659,1.,-1.75412641804042));
#60961=CARTESIAN_POINT('Ctrl Pts',(3.71208146346136,1.,-1.75997588498865));
#60962=CARTESIAN_POINT('Ctrl Pts',(3.71713822377359,1.,-1.76585552124394));
#60963=CARTESIAN_POINT('Ctrl Pts',(3.72217319911254,1.,-1.77176509401761));
#60964=CARTESIAN_POINT('Ctrl Pts',(3.72718661205609,1.,-1.77770437039658));
#60965=CARTESIAN_POINT('Ctrl Pts',(3.7321786309547,1.,-1.78367308442901));
#60966=CARTESIAN_POINT('Ctrl Pts',(3.73714934730681,1.,-1.78967092823491));
#60967=CARTESIAN_POINT('Ctrl Pts',(3.74209880352445,1.,-1.79569757859422));
#60968=CARTESIAN_POINT('Ctrl Pts',(3.74702700875467,1.,-1.8017527148577));
#60969=CARTESIAN_POINT('Ctrl Pts',(3.75193395887977,1.,-1.80783603939617));
#60970=CARTESIAN_POINT('Ctrl Pts',(3.75681965683071,1.,-1.8139472983358));
#60971=CARTESIAN_POINT('Ctrl Pts',(3.76168412707948,1.,-1.82008629694091));
#60972=CARTESIAN_POINT('Ctrl Pts',(3.76652740353775,1.,-1.82625289220915));
#60973=CARTESIAN_POINT('Ctrl Pts',(3.77038509817999,1.,-1.83120816955646));
#60974=CARTESIAN_POINT('Ctrl Pts',(3.77326886064398,1.,-1.83493697934534));
#60975=CARTESIAN_POINT('Ctrl Pts',(3.77518714457833,1.,-1.83742834010626));
#60976=CARTESIAN_POINT('Ctrl Pts',(3.77614523045147,1.,-1.83867539237861));
#60977=CARTESIAN_POINT('Origin',(3.77614523045147,0.,-1.83867539237861));
#60978=CARTESIAN_POINT('',(3.70708211654725,1.,-1.97421938526992));
#60979=CARTESIAN_POINT('Origin',(0.,0.,0.));
#60980=CARTESIAN_POINT('',(3.49844575334386,1.,-1.35032489087269));
#60981=CARTESIAN_POINT('Origin',(0.,1.,0.));
#60982=CARTESIAN_POINT('Ctrl Pts',(3.49844575334386,1.,-1.35032489087269));
#60983=CARTESIAN_POINT('Ctrl Pts',(3.49844575334386,0.666666666666667,-1.35032489087269));
#60984=CARTESIAN_POINT('Ctrl Pts',(3.49844575334386,0.333333333333333,-1.35032489087269));
#60985=CARTESIAN_POINT('Ctrl Pts',(3.49844575334386,-0.333333333333333,
-1.35032489087269));
#60986=CARTESIAN_POINT('Ctrl Pts',(3.49844575334386,-0.666666666666667,
-1.35032489087269));
#60987=CARTESIAN_POINT('Ctrl Pts',(3.49844575334386,-1.,-1.35032489087269));
#60988=CARTESIAN_POINT('Ctrl Pts',(3.97027773754922,-1.,-1.36999806084572));
#60989=CARTESIAN_POINT('Ctrl Pts',(3.97027773754922,1.,-1.36999806084572));
#60990=CARTESIAN_POINT('Ctrl Pts',(3.9687184694173,-1.,-1.37020239094758));
#60991=CARTESIAN_POINT('Ctrl Pts',(3.9687184694173,1.,-1.37020239094758));
#60992=CARTESIAN_POINT('Ctrl Pts',(3.96560037975788,-1.,-1.37060761746027));
#60993=CARTESIAN_POINT('Ctrl Pts',(3.96560037975788,1.,-1.37060761746027));
#60994=CARTESIAN_POINT('Ctrl Pts',(3.96092458508407,-1.,-1.37120515615663));
#60995=CARTESIAN_POINT('Ctrl Pts',(3.96092458508407,1.,-1.37120515615663));
#60996=CARTESIAN_POINT('Ctrl Pts',(3.95469287283105,-1.,-1.37198126433139));
#60997=CARTESIAN_POINT('Ctrl Pts',(3.95469287283105,1.,-1.37198126433139));
#60998=CARTESIAN_POINT('Ctrl Pts',(3.94690771786926,-1.,-1.37291699203423));
#60999=CARTESIAN_POINT('Ctrl Pts',(3.94690771786926,1.,-1.37291699203423));
#61000=CARTESIAN_POINT('Ctrl Pts',(3.93912709041791,-1.,-1.37381821967499));
#61001=CARTESIAN_POINT('Ctrl Pts',(3.93912709041791,1.,-1.37381821967499));
#61002=CARTESIAN_POINT('Ctrl Pts',(3.93135106761941,-1.,-1.37468482215784));
#61003=CARTESIAN_POINT('Ctrl Pts',(3.93135106761941,1.,-1.37468482215784));
#61004=CARTESIAN_POINT('Ctrl Pts',(3.92357976987132,-1.,-1.37551664448057));
#61005=CARTESIAN_POINT('Ctrl Pts',(3.92357976987132,1.,-1.37551664448057));
#61006=CARTESIAN_POINT('Ctrl Pts',(3.91581337461825,-1.,-1.37631350505516));
#61007=CARTESIAN_POINT('Ctrl Pts',(3.91581337461825,1.,-1.37631350505516));
#61008=CARTESIAN_POINT('Ctrl Pts',(3.90805209522729,-1.,-1.3770751963376));
#61009=CARTESIAN_POINT('Ctrl Pts',(3.90805209522729,1.,-1.3770751963376));
#61010=CARTESIAN_POINT('Ctrl Pts',(3.90029615196255,-1.,-1.3778014851263));
#61011=CARTESIAN_POINT('Ctrl Pts',(3.90029615196255,1.,-1.3778014851263));
#61012=CARTESIAN_POINT('Ctrl Pts',(3.89254574338385,-1.,-1.37849211287981));
#61013=CARTESIAN_POINT('Ctrl Pts',(3.89254574338385,1.,-1.37849211287981));
#61014=CARTESIAN_POINT('Ctrl Pts',(3.88480102249461,-1.,-1.37914679719446));
#61015=CARTESIAN_POINT('Ctrl Pts',(3.88480102249461,1.,-1.37914679719446));
#61016=CARTESIAN_POINT('Ctrl Pts',(3.87706205830865,-1.,-1.37976523097187));
#61017=CARTESIAN_POINT('Ctrl Pts',(3.87706205830865,1.,-1.37976523097187));
#61018=CARTESIAN_POINT('Ctrl Pts',(3.86932885813403,-1.,-1.38034709213129));
#61019=CARTESIAN_POINT('Ctrl Pts',(3.86932885813403,1.,-1.38034709213129));
#61020=CARTESIAN_POINT('Ctrl Pts',(3.86160143044187,-1.,-1.38089205993068));
#61021=CARTESIAN_POINT('Ctrl Pts',(3.86160143044187,1.,-1.38089205993068));
#61022=CARTESIAN_POINT('Ctrl Pts',(3.85387983979557,-1.,-1.38139983115075));
#61023=CARTESIAN_POINT('Ctrl Pts',(3.85387983979557,1.,-1.38139983115075));
#61024=CARTESIAN_POINT('Ctrl Pts',(3.84616425605705,-1.,-1.38187013346089));
#61025=CARTESIAN_POINT('Ctrl Pts',(3.84616425605705,1.,-1.38187013346089));
#61026=CARTESIAN_POINT('Ctrl Pts',(3.83845502790609,-1.,-1.38230274828774));
#61027=CARTESIAN_POINT('Ctrl Pts',(3.83845502790609,1.,-1.38230274828774));
#61028=CARTESIAN_POINT('Ctrl Pts',(3.83075266982138,-1.,-1.38269750245086));
#61029=CARTESIAN_POINT('Ctrl Pts',(3.83075266982138,1.,-1.38269750245086));
#61030=CARTESIAN_POINT('Ctrl Pts',(3.82305771743715,-1.,-1.38305421262724));
#61031=CARTESIAN_POINT('Ctrl Pts',(3.82305771743715,1.,-1.38305421262724));
#61032=CARTESIAN_POINT('Ctrl Pts',(3.81537060817765,-1.,-1.38337263902766));
#61033=CARTESIAN_POINT('Ctrl Pts',(3.81537060817765,1.,-1.38337263902766));
#61034=CARTESIAN_POINT('Ctrl Pts',(3.80769156398429,-1.,-1.38365244046226));
#61035=CARTESIAN_POINT('Ctrl Pts',(3.80769156398429,1.,-1.38365244046226));
#61036=CARTESIAN_POINT('Ctrl Pts',(3.80002044322169,-1.,-1.38389311766701));
#61037=CARTESIAN_POINT('Ctrl Pts',(3.80002044322169,1.,-1.38389311766701));
#61038=CARTESIAN_POINT('Ctrl Pts',(3.79235669640907,-1.,-1.38409399694589));
#61039=CARTESIAN_POINT('Ctrl Pts',(3.79235669640907,1.,-1.38409399694589));
#61040=CARTESIAN_POINT('Ctrl Pts',(3.78469969805134,-1.,-1.38425435883773));
#61041=CARTESIAN_POINT('Ctrl Pts',(3.78469969805134,1.,-1.38425435883773));
#61042=CARTESIAN_POINT('Ctrl Pts',(3.77704902230441,-1.,-1.38437354551435));
#61043=CARTESIAN_POINT('Ctrl Pts',(3.77704902230441,1.,-1.38437354551435));
#61044=CARTESIAN_POINT('Ctrl Pts',(3.76940473185775,-1.,-1.38445107339517));
#61045=CARTESIAN_POINT('Ctrl Pts',(3.76940473185775,1.,-1.38445107339517));
#61046=CARTESIAN_POINT('Ctrl Pts',(3.76176768271347,-1.,-1.38448675253343));
#61047=CARTESIAN_POINT('Ctrl Pts',(3.76176768271347,1.,-1.38448675253343));
#61048=CARTESIAN_POINT('Ctrl Pts',(3.75413976318727,-1.,-1.38448077997155));
#61049=CARTESIAN_POINT('Ctrl Pts',(3.75413976318727,1.,-1.38448077997155));
#61050=CARTESIAN_POINT('Ctrl Pts',(3.7465231716786,-1.,-1.38443344984389));
#61051=CARTESIAN_POINT('Ctrl Pts',(3.7465231716786,1.,-1.38443344984389));
#61052=CARTESIAN_POINT('Ctrl Pts',(3.73891976418099,-1.,-1.38434489156456));
#61053=CARTESIAN_POINT('Ctrl Pts',(3.73891976418099,1.,-1.38434489156456));
#61054=CARTESIAN_POINT('Ctrl Pts',(3.73133035859283,-1.,-1.38421479111531));
#61055=CARTESIAN_POINT('Ctrl Pts',(3.73133035859283,1.,-1.38421479111531));
#61056=CARTESIAN_POINT('Ctrl Pts',(3.72375409358805,-1.,-1.3840421342895));
#61057=CARTESIAN_POINT('Ctrl Pts',(3.72375409358805,1.,-1.3840421342895));
#61058=CARTESIAN_POINT('Ctrl Pts',(3.7161876605181,-1.,-1.38382489984585));
#61059=CARTESIAN_POINT('Ctrl Pts',(3.7161876605181,1.,-1.38382489984585));
#61060=CARTESIAN_POINT('Ctrl Pts',(3.70862680753343,-1.,-1.38356065402122));
#61061=CARTESIAN_POINT('Ctrl Pts',(3.70862680753343,1.,-1.38356065402122));
#61062=CARTESIAN_POINT('Ctrl Pts',(3.70106792167894,-1.,-1.38324717612862));
#61063=CARTESIAN_POINT('Ctrl Pts',(3.70106792167894,1.,-1.38324717612862));
#61064=CARTESIAN_POINT('Ctrl Pts',(3.69350967899523,-1.,-1.38288311171649));
#61065=CARTESIAN_POINT('Ctrl Pts',(3.69350967899523,1.,-1.38288311171649));
#61066=CARTESIAN_POINT('Ctrl Pts',(3.68595444983844,-1.,-1.38246852827185));
#61067=CARTESIAN_POINT('Ctrl Pts',(3.68595444983844,1.,-1.38246852827185));
#61068=CARTESIAN_POINT('Ctrl Pts',(3.6784103848243,-1.,-1.38200574290626));
#61069=CARTESIAN_POINT('Ctrl Pts',(3.6784103848243,1.,-1.38200574290626));
#61070=CARTESIAN_POINT('Ctrl Pts',(3.67088843112282,-1.,-1.38149812653876));
#61071=CARTESIAN_POINT('Ctrl Pts',(3.67088843112282,1.,-1.38149812653876));
#61072=CARTESIAN_POINT('Ctrl Pts',(3.66339848520874,-1.,-1.38094856333558));
#61073=CARTESIAN_POINT('Ctrl Pts',(3.66339848520874,1.,-1.38094856333558));
#61074=CARTESIAN_POINT('Ctrl Pts',(3.65594554404396,-1.,-1.38035791051215));
#61075=CARTESIAN_POINT('Ctrl Pts',(3.65594554404396,1.,-1.38035791051215));
#61076=CARTESIAN_POINT('Ctrl Pts',(3.64852652756444,-1.,-1.37972372481598));
#61077=CARTESIAN_POINT('Ctrl Pts',(3.64852652756444,1.,-1.37972372481598));
#61078=CARTESIAN_POINT('Ctrl Pts',(3.64112507791112,-1.,-1.37903818567347));
#61079=CARTESIAN_POINT('Ctrl Pts',(3.64112507791112,1.,-1.37903818567347));
#61080=CARTESIAN_POINT('Ctrl Pts',(3.63371727442448,-1.,-1.37829035457325));
#61081=CARTESIAN_POINT('Ctrl Pts',(3.63371727442448,1.,-1.37829035457325));
#61082=CARTESIAN_POINT('Ctrl Pts',(3.62628098665112,-1.,-1.37746987919868));
#61083=CARTESIAN_POINT('Ctrl Pts',(3.62628098665112,1.,-1.37746987919868));
#61084=CARTESIAN_POINT('Ctrl Pts',(3.61880481160408,-1.,-1.37657053403102));
#61085=CARTESIAN_POINT('Ctrl Pts',(3.61880481160408,1.,-1.37657053403102));
#61086=CARTESIAN_POINT('Ctrl Pts',(3.61129546591082,-1.,-1.37559314436641));
#61087=CARTESIAN_POINT('Ctrl Pts',(3.61129546591082,1.,-1.37559314436641));
#61088=CARTESIAN_POINT('Ctrl Pts',(3.60379020124038,-1.,-1.37455051379642));
#61089=CARTESIAN_POINT('Ctrl Pts',(3.60379020124038,1.,-1.37455051379642));
#61090=CARTESIAN_POINT('Ctrl Pts',(3.59634627869117,-1.,-1.37346320103184));
#61091=CARTESIAN_POINT('Ctrl Pts',(3.59634627869117,1.,-1.37346320103184));
#61092=CARTESIAN_POINT('Ctrl Pts',(3.5890185384643,-1.,-1.37235053661));
#61093=CARTESIAN_POINT('Ctrl Pts',(3.5890185384643,1.,-1.37235053661));
#61094=CARTESIAN_POINT('Ctrl Pts',(3.58183885982745,-1.,-1.37122241663073));
#61095=CARTESIAN_POINT('Ctrl Pts',(3.58183885982745,1.,-1.37122241663073));
#61096=CARTESIAN_POINT('Ctrl Pts',(3.57479875549453,-1.,-1.37007229485646));
#61097=CARTESIAN_POINT('Ctrl Pts',(3.57479875549453,1.,-1.37007229485646));
#61098=CARTESIAN_POINT('Ctrl Pts',(3.56782080304554,-1.,-1.36886584973349));
#61099=CARTESIAN_POINT('Ctrl Pts',(3.56782080304554,1.,-1.36886584973349));
#61100=CARTESIAN_POINT('Ctrl Pts',(3.56077662028492,-1.,-1.36754771771174));
#61101=CARTESIAN_POINT('Ctrl Pts',(3.56077662028492,1.,-1.36754771771174));
#61102=CARTESIAN_POINT('Ctrl Pts',(3.55353883995793,-1.,-1.36606145456711));
#61103=CARTESIAN_POINT('Ctrl Pts',(3.55353883995793,1.,-1.36606145456711));
#61104=CARTESIAN_POINT('Ctrl Pts',(3.54602591832893,-1.,-1.36436666257568));
#61105=CARTESIAN_POINT('Ctrl Pts',(3.54602591832893,1.,-1.36436666257568));
#61106=CARTESIAN_POINT('Ctrl Pts',(3.53824396425032,-1.,-1.36245507339334));
#61107=CARTESIAN_POINT('Ctrl Pts',(3.53824396425032,1.,-1.36245507339334));
#61108=CARTESIAN_POINT('Ctrl Pts',(3.53034464961849,-1.,-1.36037259643827));
#61109=CARTESIAN_POINT('Ctrl Pts',(3.53034464961849,1.,-1.36037259643827));
#61110=CARTESIAN_POINT('Ctrl Pts',(3.52261776117121,-1.,-1.35821701528975));
#61111=CARTESIAN_POINT('Ctrl Pts',(3.52261776117121,1.,-1.35821701528975));
#61112=CARTESIAN_POINT('Ctrl Pts',(3.51542230699919,-1.,-1.35611275237288));
#61113=CARTESIAN_POINT('Ctrl Pts',(3.51542230699919,1.,-1.35611275237288));
#61114=CARTESIAN_POINT('Ctrl Pts',(3.50913227060177,-1.,-1.35419113576022));
#61115=CARTESIAN_POINT('Ctrl Pts',(3.50913227060177,1.,-1.35419113576022));
#61116=CARTESIAN_POINT('Ctrl Pts',(3.50408168106113,-1.,-1.3525703284343));
#61117=CARTESIAN_POINT('Ctrl Pts',(3.50408168106113,1.,-1.3525703284343));
#61118=CARTESIAN_POINT('Ctrl Pts',(3.50049707063673,-1.,-1.35133076331065));
#61119=CARTESIAN_POINT('Ctrl Pts',(3.50049707063673,1.,-1.35133076331065));
#61120=CARTESIAN_POINT('Ctrl Pts',(3.49888720256612,-1.,-1.35067437417289));
#61121=CARTESIAN_POINT('Ctrl Pts',(3.49888720256612,1.,-1.35067437417289));
#61122=CARTESIAN_POINT('Ctrl Pts',(3.49840357193384,-1.,-1.35037650302887));
#61123=CARTESIAN_POINT('Ctrl Pts',(3.49840357193384,1.,-1.35037650302887));
#61124=CARTESIAN_POINT('Ctrl Pts',(3.49840260053616,-1.,-1.35026426118352));
#61125=CARTESIAN_POINT('Ctrl Pts',(3.49840260053616,1.,-1.35026426118352));
#61126=CARTESIAN_POINT('Ctrl Pts',(3.49848248301936,-1.,-1.35022972712301));
#61127=CARTESIAN_POINT('Ctrl Pts',(3.49848248301936,1.,-1.35022972712301));
#61128=CARTESIAN_POINT('',(3.97027773754922,1.,-1.36999806084572));
#61129=CARTESIAN_POINT('Ctrl Pts',(3.97027773754922,1.,-1.36999806084572));
#61130=CARTESIAN_POINT('Ctrl Pts',(3.9687184694173,1.,-1.37020239094758));
#61131=CARTESIAN_POINT('Ctrl Pts',(3.96560037975788,1.,-1.37060761746027));
#61132=CARTESIAN_POINT('Ctrl Pts',(3.96092458508407,1.,-1.37120515615663));
#61133=CARTESIAN_POINT('Ctrl Pts',(3.95469287283105,1.,-1.37198126433139));
#61134=CARTESIAN_POINT('Ctrl Pts',(3.94690771786926,1.,-1.37291699203423));
#61135=CARTESIAN_POINT('Ctrl Pts',(3.93912709041791,1.,-1.37381821967499));
#61136=CARTESIAN_POINT('Ctrl Pts',(3.93135106761941,1.,-1.37468482215784));
#61137=CARTESIAN_POINT('Ctrl Pts',(3.92357976987132,1.,-1.37551664448057));
#61138=CARTESIAN_POINT('Ctrl Pts',(3.91581337461825,1.,-1.37631350505516));
#61139=CARTESIAN_POINT('Ctrl Pts',(3.90805209522729,1.,-1.3770751963376));
#61140=CARTESIAN_POINT('Ctrl Pts',(3.90029615196255,1.,-1.3778014851263));
#61141=CARTESIAN_POINT('Ctrl Pts',(3.89254574338385,1.,-1.37849211287981));
#61142=CARTESIAN_POINT('Ctrl Pts',(3.88480102249461,1.,-1.37914679719446));
#61143=CARTESIAN_POINT('Ctrl Pts',(3.87706205830865,1.,-1.37976523097187));
#61144=CARTESIAN_POINT('Ctrl Pts',(3.86932885813403,1.,-1.38034709213129));
#61145=CARTESIAN_POINT('Ctrl Pts',(3.86160143044187,1.,-1.38089205993068));
#61146=CARTESIAN_POINT('Ctrl Pts',(3.85387983979557,1.,-1.38139983115075));
#61147=CARTESIAN_POINT('Ctrl Pts',(3.84616425605705,1.,-1.38187013346089));
#61148=CARTESIAN_POINT('Ctrl Pts',(3.83845502790609,1.,-1.38230274828774));
#61149=CARTESIAN_POINT('Ctrl Pts',(3.83075266982138,1.,-1.38269750245086));
#61150=CARTESIAN_POINT('Ctrl Pts',(3.82305771743715,1.,-1.38305421262724));
#61151=CARTESIAN_POINT('Ctrl Pts',(3.81537060817765,1.,-1.38337263902766));
#61152=CARTESIAN_POINT('Ctrl Pts',(3.80769156398429,1.,-1.38365244046226));
#61153=CARTESIAN_POINT('Ctrl Pts',(3.80002044322169,1.,-1.38389311766701));
#61154=CARTESIAN_POINT('Ctrl Pts',(3.79235669640907,1.,-1.38409399694589));
#61155=CARTESIAN_POINT('Ctrl Pts',(3.78469969805134,1.,-1.38425435883773));
#61156=CARTESIAN_POINT('Ctrl Pts',(3.77704902230441,1.,-1.38437354551435));
#61157=CARTESIAN_POINT('Ctrl Pts',(3.76940473185775,1.,-1.38445107339517));
#61158=CARTESIAN_POINT('Ctrl Pts',(3.76176768271347,1.,-1.38448675253343));
#61159=CARTESIAN_POINT('Ctrl Pts',(3.75413976318727,1.,-1.38448077997155));
#61160=CARTESIAN_POINT('Ctrl Pts',(3.7465231716786,1.,-1.38443344984389));
#61161=CARTESIAN_POINT('Ctrl Pts',(3.73891976418099,1.,-1.38434489156456));
#61162=CARTESIAN_POINT('Ctrl Pts',(3.73133035859283,1.,-1.38421479111531));
#61163=CARTESIAN_POINT('Ctrl Pts',(3.72375409358805,1.,-1.3840421342895));
#61164=CARTESIAN_POINT('Ctrl Pts',(3.7161876605181,1.,-1.38382489984585));
#61165=CARTESIAN_POINT('Ctrl Pts',(3.70862680753343,1.,-1.38356065402122));
#61166=CARTESIAN_POINT('Ctrl Pts',(3.70106792167894,1.,-1.38324717612862));
#61167=CARTESIAN_POINT('Ctrl Pts',(3.69350967899523,1.,-1.38288311171649));
#61168=CARTESIAN_POINT('Ctrl Pts',(3.68595444983844,1.,-1.38246852827185));
#61169=CARTESIAN_POINT('Ctrl Pts',(3.6784103848243,1.,-1.38200574290626));
#61170=CARTESIAN_POINT('Ctrl Pts',(3.67088843112282,1.,-1.38149812653876));
#61171=CARTESIAN_POINT('Ctrl Pts',(3.66339848520874,1.,-1.38094856333558));
#61172=CARTESIAN_POINT('Ctrl Pts',(3.65594554404396,1.,-1.38035791051215));
#61173=CARTESIAN_POINT('Ctrl Pts',(3.64852652756444,1.,-1.37972372481598));
#61174=CARTESIAN_POINT('Ctrl Pts',(3.64112507791112,1.,-1.37903818567347));
#61175=CARTESIAN_POINT('Ctrl Pts',(3.63371727442448,1.,-1.37829035457325));
#61176=CARTESIAN_POINT('Ctrl Pts',(3.62628098665112,1.,-1.37746987919868));
#61177=CARTESIAN_POINT('Ctrl Pts',(3.61880481160408,1.,-1.37657053403102));
#61178=CARTESIAN_POINT('Ctrl Pts',(3.61129546591082,1.,-1.37559314436641));
#61179=CARTESIAN_POINT('Ctrl Pts',(3.60379020124038,1.,-1.37455051379642));
#61180=CARTESIAN_POINT('Ctrl Pts',(3.59634627869117,1.,-1.37346320103184));
#61181=CARTESIAN_POINT('Ctrl Pts',(3.5890185384643,1.,-1.37235053661));
#61182=CARTESIAN_POINT('Ctrl Pts',(3.58183885982745,1.,-1.37122241663073));
#61183=CARTESIAN_POINT('Ctrl Pts',(3.57479875549453,1.,-1.37007229485646));
#61184=CARTESIAN_POINT('Ctrl Pts',(3.56782080304554,1.,-1.36886584973349));
#61185=CARTESIAN_POINT('Ctrl Pts',(3.56077662028492,1.,-1.36754771771174));
#61186=CARTESIAN_POINT('Ctrl Pts',(3.55353883995793,1.,-1.36606145456711));
#61187=CARTESIAN_POINT('Ctrl Pts',(3.54602591832893,1.,-1.36436666257568));
#61188=CARTESIAN_POINT('Ctrl Pts',(3.53824396425032,1.,-1.36245507339334));
#61189=CARTESIAN_POINT('Ctrl Pts',(3.53034464961849,1.,-1.36037259643827));
#61190=CARTESIAN_POINT('Ctrl Pts',(3.52261776117121,1.,-1.35821701528975));
#61191=CARTESIAN_POINT('Ctrl Pts',(3.51542230699919,1.,-1.35611275237288));
#61192=CARTESIAN_POINT('Ctrl Pts',(3.50913227060177,1.,-1.35419113576022));
#61193=CARTESIAN_POINT('Ctrl Pts',(3.50408168106113,1.,-1.3525703284343));
#61194=CARTESIAN_POINT('Ctrl Pts',(3.5007660381658,1.,-1.35142377279535));
#61195=CARTESIAN_POINT('Ctrl Pts',(3.49920025459856,1.,-1.35080045218652));
#61196=CARTESIAN_POINT('Ctrl Pts',(3.49861894124915,1.,-1.35049736560633));
#61197=CARTESIAN_POINT('Ctrl Pts',(3.49847119623841,1.,-1.35036670893102));
#61198=CARTESIAN_POINT('Ctrl Pts',(3.49844575334386,1.,-1.35032489087269));
#61199=CARTESIAN_POINT('',(3.97027773754922,0.,-1.36999806084572));
#61200=CARTESIAN_POINT('Ctrl Pts',(3.62397690409552,-1.,-0.963997613369571));
#61201=CARTESIAN_POINT('Ctrl Pts',(3.62397690409552,1.,-0.963997613369571));
#61202=CARTESIAN_POINT('Ctrl Pts',(3.62393257642191,-1.,-0.963922720982576));
#61203=CARTESIAN_POINT('Ctrl Pts',(3.62393257642191,1.,-0.963922720982576));
#61204=CARTESIAN_POINT('Ctrl Pts',(3.62399933640277,-1.,-0.963832486396056));
#61205=CARTESIAN_POINT('Ctrl Pts',(3.62399933640277,1.,-0.963832486396056));
#61206=CARTESIAN_POINT('Ctrl Pts',(3.62456568607055,-1.,-0.963875774532103));
#61207=CARTESIAN_POINT('Ctrl Pts',(3.62456568607055,1.,-0.963875774532103));
#61208=CARTESIAN_POINT('Ctrl Pts',(3.62625391255277,-1.,-0.964291001274619));
#61209=CARTESIAN_POINT('Ctrl Pts',(3.62625391255277,1.,-0.964291001274619));
#61210=CARTESIAN_POINT('Ctrl Pts',(3.62988252139998,-1.,-0.965395153165716));
#61211=CARTESIAN_POINT('Ctrl Pts',(3.62988252139998,1.,-0.965395153165716));
#61212=CARTESIAN_POINT('Ctrl Pts',(3.6349212208096,-1.,-0.967052554540878));
#61213=CARTESIAN_POINT('Ctrl Pts',(3.6349212208096,1.,-0.967052554540878));
#61214=CARTESIAN_POINT('Ctrl Pts',(3.64113946505393,-1.,-0.969195124674829));
#61215=CARTESIAN_POINT('Ctrl Pts',(3.64113946505393,1.,-0.969195124674829));
#61216=CARTESIAN_POINT('Ctrl Pts',(3.64819756447072,-1.,-0.971722122060278));
#61217=CARTESIAN_POINT('Ctrl Pts',(3.64819756447072,1.,-0.971722122060278));
#61218=CARTESIAN_POINT('Ctrl Pts',(3.6557157673487,-1.,-0.974519971354139));
#61219=CARTESIAN_POINT('Ctrl Pts',(3.6557157673487,1.,-0.974519971354139));
#61220=CARTESIAN_POINT('Ctrl Pts',(3.66333049637403,-1.,-0.977478312751416));
#61221=CARTESIAN_POINT('Ctrl Pts',(3.66333049637403,1.,-0.977478312751416));
#61222=CARTESIAN_POINT('Ctrl Pts',(3.67074983340444,-1.,-0.980505922458495));
#61223=CARTESIAN_POINT('Ctrl Pts',(3.67074983340444,1.,-0.980505922458495));
#61224=CARTESIAN_POINT('Ctrl Pts',(3.67782408841876,-1.,-0.983550791470865));
#61225=CARTESIAN_POINT('Ctrl Pts',(3.67782408841876,1.,-0.983550791470865));
#61226=CARTESIAN_POINT('Ctrl Pts',(3.6845531792623,-1.,-0.986602639864286));
#61227=CARTESIAN_POINT('Ctrl Pts',(3.6845531792623,1.,-0.986602639864286));
#61228=CARTESIAN_POINT('Ctrl Pts',(3.69102682138955,-1.,-0.989676715398859));
#61229=CARTESIAN_POINT('Ctrl Pts',(3.69102682138955,1.,-0.989676715398859));
#61230=CARTESIAN_POINT('Ctrl Pts',(3.69738123415696,-1.,-0.992802218332104));
#61231=CARTESIAN_POINT('Ctrl Pts',(3.69738123415696,1.,-0.992802218332104));
#61232=CARTESIAN_POINT('Ctrl Pts',(3.70375282282107,-1.,-0.996009819772432));
#61233=CARTESIAN_POINT('Ctrl Pts',(3.70375282282107,1.,-0.996009819772432));
#61234=CARTESIAN_POINT('Ctrl Pts',(3.7102243971387,-1.,-0.999317260756345));
#61235=CARTESIAN_POINT('Ctrl Pts',(3.7102243971387,1.,-0.999317260756345));
#61236=CARTESIAN_POINT('Ctrl Pts',(3.71680667125047,-1.,-1.00272423396802));
#61237=CARTESIAN_POINT('Ctrl Pts',(3.71680667125047,1.,-1.00272423396802));
#61238=CARTESIAN_POINT('Ctrl Pts',(3.72346803750544,-1.,-1.00622000735696));
#61239=CARTESIAN_POINT('Ctrl Pts',(3.72346803750544,1.,-1.00622000735696));
#61240=CARTESIAN_POINT('Ctrl Pts',(3.73015276704407,-1.,-1.00978798539491));
#61241=CARTESIAN_POINT('Ctrl Pts',(3.73015276704407,1.,-1.00978798539491));
#61242=CARTESIAN_POINT('Ctrl Pts',(3.73680245055747,-1.,-1.01341114319906));
#61243=CARTESIAN_POINT('Ctrl Pts',(3.73680245055747,1.,-1.01341114319906));
#61244=CARTESIAN_POINT('Ctrl Pts',(3.74337942504993,-1.,-1.01707794311088));
#61245=CARTESIAN_POINT('Ctrl Pts',(3.74337942504993,1.,-1.01707794311088));
#61246=CARTESIAN_POINT('Ctrl Pts',(3.74987777155873,-1.,-1.02078510487439));
#61247=CARTESIAN_POINT('Ctrl Pts',(3.74987777155873,1.,-1.02078510487439));
#61248=CARTESIAN_POINT('Ctrl Pts',(3.75631037456224,-1.,-1.02453429444668));
#61249=CARTESIAN_POINT('Ctrl Pts',(3.75631037456224,1.,-1.02453429444668));
#61250=CARTESIAN_POINT('Ctrl Pts',(3.76270122291245,-1.,-1.02833014458184));
#61251=CARTESIAN_POINT('Ctrl Pts',(3.76270122291245,1.,-1.02833014458184));
#61252=CARTESIAN_POINT('Ctrl Pts',(3.76907609832516,-1.,-1.03217786604919));
#61253=CARTESIAN_POINT('Ctrl Pts',(3.76907609832516,1.,-1.03217786604919));
#61254=CARTESIAN_POINT('Ctrl Pts',(3.77545283140427,-1.,-1.03608074678008));
#61255=CARTESIAN_POINT('Ctrl Pts',(3.77545283140427,1.,-1.03608074678008));
#61256=CARTESIAN_POINT('Ctrl Pts',(3.7818353500817,-1.,-1.04003862055798));
#61257=CARTESIAN_POINT('Ctrl Pts',(3.7818353500817,1.,-1.04003862055798));
#61258=CARTESIAN_POINT('Ctrl Pts',(3.78821910787179,-1.,-1.04404924374422));
#61259=CARTESIAN_POINT('Ctrl Pts',(3.78821910787179,1.,-1.04404924374422));
#61260=CARTESIAN_POINT('Ctrl Pts',(3.79459440308786,-1.,-1.04810913267639));
#61261=CARTESIAN_POINT('Ctrl Pts',(3.79459440308786,1.,-1.04810913267639));
#61262=CARTESIAN_POINT('Ctrl Pts',(3.80095039790681,-1.,-1.05221457990016));
#61263=CARTESIAN_POINT('Ctrl Pts',(3.80095039790681,1.,-1.05221457990016));
#61264=CARTESIAN_POINT('Ctrl Pts',(3.80727913637791,-1.,-1.05636266918644));
#61265=CARTESIAN_POINT('Ctrl Pts',(3.80727913637791,1.,-1.05636266918644));
#61266=CARTESIAN_POINT('Ctrl Pts',(3.8135786611749,-1.,-1.06055206187299));
#61267=CARTESIAN_POINT('Ctrl Pts',(3.8135786611749,1.,-1.06055206187299));
#61268=CARTESIAN_POINT('Ctrl Pts',(3.81985083953012,-1.,-1.0647824403893));
#61269=CARTESIAN_POINT('Ctrl Pts',(3.81985083953012,1.,-1.0647824403893));
#61270=CARTESIAN_POINT('Ctrl Pts',(3.82609989967276,-1.,-1.06905413180359));
#61271=CARTESIAN_POINT('Ctrl Pts',(3.82609989967276,1.,-1.06905413180359));
#61272=CARTESIAN_POINT('Ctrl Pts',(3.83233071195144,-1.,-1.07336766633459));
#61273=CARTESIAN_POINT('Ctrl Pts',(3.83233071195144,1.,-1.07336766633459));
#61274=CARTESIAN_POINT('Ctrl Pts',(3.83854714117491,-1.,-1.07772335353858));
#61275=CARTESIAN_POINT('Ctrl Pts',(3.83854714117491,1.,-1.07772335353858));
#61276=CARTESIAN_POINT('Ctrl Pts',(3.8447504803063,-1.,-1.08212087917991));
#61277=CARTESIAN_POINT('Ctrl Pts',(3.8447504803063,1.,-1.08212087917991));
#61278=CARTESIAN_POINT('Ctrl Pts',(3.85094025222713,-1.,-1.08655950846384));
#61279=CARTESIAN_POINT('Ctrl Pts',(3.85094025222713,1.,-1.08655950846384));
#61280=CARTESIAN_POINT('Ctrl Pts',(3.85711487933931,-1.,-1.09103825516294));
#61281=CARTESIAN_POINT('Ctrl Pts',(3.85711487933931,1.,-1.09103825516294));
#61282=CARTESIAN_POINT('Ctrl Pts',(3.86327241021247,-1.,-1.09555606505013));
#61283=CARTESIAN_POINT('Ctrl Pts',(3.86327241021247,1.,-1.09555606505013));
#61284=CARTESIAN_POINT('Ctrl Pts',(3.86941120134849,-1.,-1.10011198761195));
#61285=CARTESIAN_POINT('Ctrl Pts',(3.86941120134849,1.,-1.10011198761195));
#61286=CARTESIAN_POINT('Ctrl Pts',(3.87553067187514,-1.,-1.10470536603287));
#61287=CARTESIAN_POINT('Ctrl Pts',(3.87553067187514,1.,-1.10470536603287));
#61288=CARTESIAN_POINT('Ctrl Pts',(3.88163105531724,-1.,-1.10933577224008));
#61289=CARTESIAN_POINT('Ctrl Pts',(3.88163105531724,1.,-1.10933577224008));
#61290=CARTESIAN_POINT('Ctrl Pts',(3.88771308285171,-1.,-1.11400292434429));
#61291=CARTESIAN_POINT('Ctrl Pts',(3.88771308285171,1.,-1.11400292434429));
#61292=CARTESIAN_POINT('Ctrl Pts',(3.89377768340344,-1.,-1.11870660794603));
#61293=CARTESIAN_POINT('Ctrl Pts',(3.89377768340344,1.,-1.11870660794603));
#61294=CARTESIAN_POINT('Ctrl Pts',(3.89982569750025,-1.,-1.12344660099043));
#61295=CARTESIAN_POINT('Ctrl Pts',(3.89982569750025,1.,-1.12344660099043));
#61296=CARTESIAN_POINT('Ctrl Pts',(3.90585753318737,-1.,-1.12822258281553));
#61297=CARTESIAN_POINT('Ctrl Pts',(3.90585753318737,1.,-1.12822258281553));
#61298=CARTESIAN_POINT('Ctrl Pts',(3.91187321145649,-1.,-1.13303414693896));
#61299=CARTESIAN_POINT('Ctrl Pts',(3.91187321145649,1.,-1.13303414693896));
#61300=CARTESIAN_POINT('Ctrl Pts',(3.91787251936827,-1.,-1.13788084225554));
#61301=CARTESIAN_POINT('Ctrl Pts',(3.91787251936827,1.,-1.13788084225554));
#61302=CARTESIAN_POINT('Ctrl Pts',(3.92385513133997,-1.,-1.14276220561593));
#61303=CARTESIAN_POINT('Ctrl Pts',(3.92385513133997,1.,-1.14276220561593));
#61304=CARTESIAN_POINT('Ctrl Pts',(3.92982073294257,-1.,-1.14767779451124));
#61305=CARTESIAN_POINT('Ctrl Pts',(3.92982073294257,1.,-1.14767779451124));
#61306=CARTESIAN_POINT('Ctrl Pts',(3.9357691705628,-1.,-1.1526272271632));
#61307=CARTESIAN_POINT('Ctrl Pts',(3.9357691705628,1.,-1.1526272271632));
#61308=CARTESIAN_POINT('Ctrl Pts',(3.94170046685203,-1.,-1.15761018340956));
#61309=CARTESIAN_POINT('Ctrl Pts',(3.94170046685203,1.,-1.15761018340956));
#61310=CARTESIAN_POINT('Ctrl Pts',(3.94761474780583,-1.,-1.16262637999157));
#61311=CARTESIAN_POINT('Ctrl Pts',(3.94761474780583,1.,-1.16262637999157));
#61312=CARTESIAN_POINT('Ctrl Pts',(3.95351219509876,-1.,-1.16767555244438));
#61313=CARTESIAN_POINT('Ctrl Pts',(3.95351219509876,1.,-1.16767555244438));
#61314=CARTESIAN_POINT('Ctrl Pts',(3.95939299213276,-1.,-1.17275743590361));
#61315=CARTESIAN_POINT('Ctrl Pts',(3.95939299213276,1.,-1.17275743590361));
#61316=CARTESIAN_POINT('Ctrl Pts',(3.96525726358159,-1.,-1.17787174135592));
#61317=CARTESIAN_POINT('Ctrl Pts',(3.96525726358159,1.,-1.17787174135592));
#61318=CARTESIAN_POINT('Ctrl Pts',(3.97110505165415,-1.,-1.18301815039831));
#61319=CARTESIAN_POINT('Ctrl Pts',(3.97110505165415,1.,-1.18301815039831));
#61320=CARTESIAN_POINT('Ctrl Pts',(3.97693634767754,-1.,-1.18819633715539));
#61321=CARTESIAN_POINT('Ctrl Pts',(3.97693634767754,1.,-1.18819633715539));
#61322=CARTESIAN_POINT('Ctrl Pts',(3.98275111052561,-1.,-1.19340598349475));
#61323=CARTESIAN_POINT('Ctrl Pts',(3.98275111052561,1.,-1.19340598349475));
#61324=CARTESIAN_POINT('Ctrl Pts',(3.98854928957189,-1.,-1.19864679609566));
#61325=CARTESIAN_POINT('Ctrl Pts',(3.98854928957189,1.,-1.19864679609566));
#61326=CARTESIAN_POINT('Ctrl Pts',(3.99433084799666,-1.,-1.20391852375139));
#61327=CARTESIAN_POINT('Ctrl Pts',(3.99433084799666,1.,-1.20391852375139));
#61328=CARTESIAN_POINT('Ctrl Pts',(4.00009577950721,-1.,-1.20922097029551));
#61329=CARTESIAN_POINT('Ctrl Pts',(4.00009577950721,1.,-1.20922097029551));
#61330=CARTESIAN_POINT('Ctrl Pts',(4.00584409522722,-1.,-1.21455398918133));
#61331=CARTESIAN_POINT('Ctrl Pts',(4.00584409522722,1.,-1.21455398918133));
#61332=CARTESIAN_POINT('Ctrl Pts',(4.01042947140789,-1.,-1.21884478244403));
#61333=CARTESIAN_POINT('Ctrl Pts',(4.01042947140789,1.,-1.21884478244403));
#61334=CARTESIAN_POINT('Ctrl Pts',(4.01386104433519,-1.,-1.22207656455845));
#61335=CARTESIAN_POINT('Ctrl Pts',(4.01386104433519,1.,-1.22207656455845));
#61336=CARTESIAN_POINT('Ctrl Pts',(4.01614544569895,-1.,-1.22423716681317));
#61337=CARTESIAN_POINT('Ctrl Pts',(4.01614544569895,1.,-1.22423716681317));
#61338=CARTESIAN_POINT('Ctrl Pts',(4.01728681790024,-1.,-1.22531898815164));
#61339=CARTESIAN_POINT('Ctrl Pts',(4.01728681790024,1.,-1.22531898815164));
#61340=CARTESIAN_POINT('',(3.62400312501199,1.,-0.963899035118984));
#61341=CARTESIAN_POINT('Ctrl Pts',(3.62400312501199,-1.,-0.963899035118986));
#61342=CARTESIAN_POINT('Ctrl Pts',(3.62400312501199,-0.666666666666667,
-0.963899035118986));
#61343=CARTESIAN_POINT('Ctrl Pts',(3.62400312501199,-0.333333333333333,
-0.963899035118986));
#61344=CARTESIAN_POINT('Ctrl Pts',(3.62400312501199,0.333333333333333,-0.963899035118986));
#61345=CARTESIAN_POINT('Ctrl Pts',(3.62400312501199,0.666666666666667,-0.963899035118986));
#61346=CARTESIAN_POINT('Ctrl Pts',(3.62400312501199,1.,-0.963899035118986));
#61347=CARTESIAN_POINT('',(4.01728681790024,1.,-1.22531898815164));
#61348=CARTESIAN_POINT('',(4.01728681790024,0.,-1.22531898815164));
#61349=CARTESIAN_POINT('Ctrl Pts',(3.62400312501199,1.,-0.963899035118985));
#61350=CARTESIAN_POINT('Ctrl Pts',(3.62404828878374,1.,-0.963880158556713));
#61351=CARTESIAN_POINT('Ctrl Pts',(3.62424461507455,1.,-0.963861297423579));
#61352=CARTESIAN_POINT('Ctrl Pts',(3.62489305727516,1.,-0.96395778264259));
#61353=CARTESIAN_POINT('Ctrl Pts',(3.62652618145252,1.,-0.964373850166082));
#61354=CARTESIAN_POINT('Ctrl Pts',(3.62988252139998,1.,-0.965395153165716));
#61355=CARTESIAN_POINT('Ctrl Pts',(3.6349212208096,1.,-0.967052554540878));
#61356=CARTESIAN_POINT('Ctrl Pts',(3.64113946505393,1.,-0.969195124674829));
#61357=CARTESIAN_POINT('Ctrl Pts',(3.64819756447072,1.,-0.971722122060278));
#61358=CARTESIAN_POINT('Ctrl Pts',(3.6557157673487,1.,-0.974519971354139));
#61359=CARTESIAN_POINT('Ctrl Pts',(3.66333049637403,1.,-0.977478312751416));
#61360=CARTESIAN_POINT('Ctrl Pts',(3.67074983340444,1.,-0.980505922458495));
#61361=CARTESIAN_POINT('Ctrl Pts',(3.67782408841876,1.,-0.983550791470865));
#61362=CARTESIAN_POINT('Ctrl Pts',(3.6845531792623,1.,-0.986602639864286));
#61363=CARTESIAN_POINT('Ctrl Pts',(3.69102682138955,1.,-0.989676715398859));
#61364=CARTESIAN_POINT('Ctrl Pts',(3.69738123415696,1.,-0.992802218332104));
#61365=CARTESIAN_POINT('Ctrl Pts',(3.70375282282107,1.,-0.996009819772432));
#61366=CARTESIAN_POINT('Ctrl Pts',(3.7102243971387,1.,-0.999317260756345));
#61367=CARTESIAN_POINT('Ctrl Pts',(3.71680667125047,1.,-1.00272423396802));
#61368=CARTESIAN_POINT('Ctrl Pts',(3.72346803750544,1.,-1.00622000735696));
#61369=CARTESIAN_POINT('Ctrl Pts',(3.73015276704407,1.,-1.00978798539491));
#61370=CARTESIAN_POINT('Ctrl Pts',(3.73680245055747,1.,-1.01341114319906));
#61371=CARTESIAN_POINT('Ctrl Pts',(3.74337942504993,1.,-1.01707794311088));
#61372=CARTESIAN_POINT('Ctrl Pts',(3.74987777155873,1.,-1.02078510487439));
#61373=CARTESIAN_POINT('Ctrl Pts',(3.75631037456224,1.,-1.02453429444668));
#61374=CARTESIAN_POINT('Ctrl Pts',(3.76270122291245,1.,-1.02833014458184));
#61375=CARTESIAN_POINT('Ctrl Pts',(3.76907609832516,1.,-1.03217786604919));
#61376=CARTESIAN_POINT('Ctrl Pts',(3.77545283140427,1.,-1.03608074678008));
#61377=CARTESIAN_POINT('Ctrl Pts',(3.7818353500817,1.,-1.04003862055798));
#61378=CARTESIAN_POINT('Ctrl Pts',(3.78821910787179,1.,-1.04404924374422));
#61379=CARTESIAN_POINT('Ctrl Pts',(3.79459440308786,1.,-1.04810913267639));
#61380=CARTESIAN_POINT('Ctrl Pts',(3.80095039790681,1.,-1.05221457990016));
#61381=CARTESIAN_POINT('Ctrl Pts',(3.80727913637791,1.,-1.05636266918644));
#61382=CARTESIAN_POINT('Ctrl Pts',(3.8135786611749,1.,-1.06055206187299));
#61383=CARTESIAN_POINT('Ctrl Pts',(3.81985083953012,1.,-1.0647824403893));
#61384=CARTESIAN_POINT('Ctrl Pts',(3.82609989967276,1.,-1.06905413180359));
#61385=CARTESIAN_POINT('Ctrl Pts',(3.83233071195144,1.,-1.07336766633459));
#61386=CARTESIAN_POINT('Ctrl Pts',(3.83854714117491,1.,-1.07772335353858));
#61387=CARTESIAN_POINT('Ctrl Pts',(3.8447504803063,1.,-1.08212087917991));
#61388=CARTESIAN_POINT('Ctrl Pts',(3.85094025222713,1.,-1.08655950846384));
#61389=CARTESIAN_POINT('Ctrl Pts',(3.85711487933931,1.,-1.09103825516294));
#61390=CARTESIAN_POINT('Ctrl Pts',(3.86327241021247,1.,-1.09555606505013));
#61391=CARTESIAN_POINT('Ctrl Pts',(3.86941120134849,1.,-1.10011198761195));
#61392=CARTESIAN_POINT('Ctrl Pts',(3.87553067187514,1.,-1.10470536603287));
#61393=CARTESIAN_POINT('Ctrl Pts',(3.88163105531724,1.,-1.10933577224008));
#61394=CARTESIAN_POINT('Ctrl Pts',(3.88771308285171,1.,-1.11400292434429));
#61395=CARTESIAN_POINT('Ctrl Pts',(3.89377768340344,1.,-1.11870660794603));
#61396=CARTESIAN_POINT('Ctrl Pts',(3.89982569750025,1.,-1.12344660099043));
#61397=CARTESIAN_POINT('Ctrl Pts',(3.90585753318737,1.,-1.12822258281553));
#61398=CARTESIAN_POINT('Ctrl Pts',(3.91187321145649,1.,-1.13303414693896));
#61399=CARTESIAN_POINT('Ctrl Pts',(3.91787251936827,1.,-1.13788084225554));
#61400=CARTESIAN_POINT('Ctrl Pts',(3.92385513133997,1.,-1.14276220561593));
#61401=CARTESIAN_POINT('Ctrl Pts',(3.92982073294257,1.,-1.14767779451124));
#61402=CARTESIAN_POINT('Ctrl Pts',(3.9357691705628,1.,-1.1526272271632));
#61403=CARTESIAN_POINT('Ctrl Pts',(3.94170046685203,1.,-1.15761018340956));
#61404=CARTESIAN_POINT('Ctrl Pts',(3.94761474780583,1.,-1.16262637999157));
#61405=CARTESIAN_POINT('Ctrl Pts',(3.95351219509876,1.,-1.16767555244438));
#61406=CARTESIAN_POINT('Ctrl Pts',(3.95939299213276,1.,-1.17275743590361));
#61407=CARTESIAN_POINT('Ctrl Pts',(3.96525726358159,1.,-1.17787174135592));
#61408=CARTESIAN_POINT('Ctrl Pts',(3.97110505165415,1.,-1.18301815039831));
#61409=CARTESIAN_POINT('Ctrl Pts',(3.97693634767754,1.,-1.18819633715539));
#61410=CARTESIAN_POINT('Ctrl Pts',(3.98275111052561,1.,-1.19340598349475));
#61411=CARTESIAN_POINT('Ctrl Pts',(3.98854928957189,1.,-1.19864679609566));
#61412=CARTESIAN_POINT('Ctrl Pts',(3.99433084799666,1.,-1.20391852375139));
#61413=CARTESIAN_POINT('Ctrl Pts',(4.00009577950721,1.,-1.20922097029551));
#61414=CARTESIAN_POINT('Ctrl Pts',(4.00584409522722,1.,-1.21455398918133));
#61415=CARTESIAN_POINT('Ctrl Pts',(4.01042947140789,1.,-1.21884478244403));
#61416=CARTESIAN_POINT('Ctrl Pts',(4.01386104433519,1.,-1.22207656455845));
#61417=CARTESIAN_POINT('Ctrl Pts',(4.01614544569895,1.,-1.22423716681317));
#61418=CARTESIAN_POINT('Ctrl Pts',(4.01728681790024,1.,-1.22531898815164));
#61419=CARTESIAN_POINT('Origin',(4.01728681790024,0.,-1.22531898815164));
#61420=CARTESIAN_POINT('',(3.97027773754922,1.,-1.36999806084572));
#61421=CARTESIAN_POINT('Origin',(0.,0.,0.));
#61422=CARTESIAN_POINT('',(3.66661143271648,1.,-0.786422660833743));
#61423=CARTESIAN_POINT('Origin',(0.,1.,0.));
#61424=CARTESIAN_POINT('Ctrl Pts',(3.66661143271648,1.,-0.786422660833743));
#61425=CARTESIAN_POINT('Ctrl Pts',(3.66661143271648,0.666666666666667,-0.786422660833743));
#61426=CARTESIAN_POINT('Ctrl Pts',(3.66661143271648,0.333333333333333,-0.786422660833743));
#61427=CARTESIAN_POINT('Ctrl Pts',(3.66661143271648,-0.333333333333333,
-0.786422660833743));
#61428=CARTESIAN_POINT('Ctrl Pts',(3.66661143271648,-0.666666666666667,
-0.786422660833742));
#61429=CARTESIAN_POINT('Ctrl Pts',(3.66661143271648,-1.,-0.786422660833742));
#61430=CARTESIAN_POINT('Ctrl Pts',(4.13571194405636,-1.,-0.73204283740062));
#61431=CARTESIAN_POINT('Ctrl Pts',(4.13571194405636,1.,-0.73204283740062));
#61432=CARTESIAN_POINT('Ctrl Pts',(4.13420383737278,-1.,-0.732488575135926));
#61433=CARTESIAN_POINT('Ctrl Pts',(4.13420383737278,1.,-0.732488575135926));
#61434=CARTESIAN_POINT('Ctrl Pts',(4.13118752796397,-1.,-0.733376589325634));
#61435=CARTESIAN_POINT('Ctrl Pts',(4.13118752796397,1.,-0.733376589325634));
#61436=CARTESIAN_POINT('Ctrl Pts',(4.12666277572794,-1.,-0.734698226767513));
#61437=CARTESIAN_POINT('Ctrl Pts',(4.12666277572794,1.,-0.734698226767513));
#61438=CARTESIAN_POINT('Ctrl Pts',(4.12062919626082,-1.,-0.736439634335347));
#61439=CARTESIAN_POINT('Ctrl Pts',(4.12062919626082,1.,-0.736439634335347));
#61440=CARTESIAN_POINT('Ctrl Pts',(4.11308626953795,-1.,-0.738581708229119));
#61441=CARTESIAN_POINT('Ctrl Pts',(4.11308626953795,1.,-0.738581708229119));
#61442=CARTESIAN_POINT('Ctrl Pts',(4.1055424175856,-1.,-0.740688998555152));
#61443=CARTESIAN_POINT('Ctrl Pts',(4.1055424175856,1.,-0.740688998555152));
#61444=CARTESIAN_POINT('Ctrl Pts',(4.09799769702712,-1.,-0.742761369690018));
#61445=CARTESIAN_POINT('Ctrl Pts',(4.09799769702712,1.,-0.742761369690018));
#61446=CARTESIAN_POINT('Ctrl Pts',(4.09045220253011,-1.,-0.744798649705514));
#61447=CARTESIAN_POINT('Ctrl Pts',(4.09045220253011,1.,-0.744798649705514));
#61448=CARTESIAN_POINT('Ctrl Pts',(4.08290608094789,-1.,-0.746800631490822));
#61449=CARTESIAN_POINT('Ctrl Pts',(4.08290608094789,1.,-0.746800631490822));
#61450=CARTESIAN_POINT('Ctrl Pts',(4.07535951055363,-1.,-0.748767076679177));
#61451=CARTESIAN_POINT('Ctrl Pts',(4.07535951055363,1.,-0.748767076679177));
#61452=CARTESIAN_POINT('Ctrl Pts',(4.06781267241886,-1.,-0.750697720483176));
#61453=CARTESIAN_POINT('Ctrl Pts',(4.06781267241886,1.,-0.750697720483176));
#61454=CARTESIAN_POINT('Ctrl Pts',(4.06026572221399,-1.,-0.752592276482869));
#61455=CARTESIAN_POINT('Ctrl Pts',(4.06026572221399,1.,-0.752592276482869));
#61456=CARTESIAN_POINT('Ctrl Pts',(4.05271876688106,-1.,-0.754450441816412));
#61457=CARTESIAN_POINT('Ctrl Pts',(4.05271876688106,1.,-0.754450441816412));
#61458=CARTESIAN_POINT('Ctrl Pts',(4.04517182654344,-1.,-0.756271902370187));
#61459=CARTESIAN_POINT('Ctrl Pts',(4.04517182654344,1.,-0.756271902370187));
#61460=CARTESIAN_POINT('Ctrl Pts',(4.03762485803468,-1.,-0.758056338885554));
#61461=CARTESIAN_POINT('Ctrl Pts',(4.03762485803468,1.,-0.758056338885554));
#61462=CARTESIAN_POINT('Ctrl Pts',(4.0300778195465,-1.,-0.759803433244166));
#61463=CARTESIAN_POINT('Ctrl Pts',(4.0300778195465,1.,-0.759803433244166));
#61464=CARTESIAN_POINT('Ctrl Pts',(4.02253072741347,-1.,-0.761512875859942));
#61465=CARTESIAN_POINT('Ctrl Pts',(4.02253072741347,1.,-0.761512875859942));
#61466=CARTESIAN_POINT('Ctrl Pts',(4.01498370680434,-1.,-0.763184371182827));
#61467=CARTESIAN_POINT('Ctrl Pts',(4.01498370680434,1.,-0.763184371182827));
#61468=CARTESIAN_POINT('Ctrl Pts',(4.00743706791366,-1.,-0.764817648784947));
#61469=CARTESIAN_POINT('Ctrl Pts',(4.00743706791366,1.,-0.764817648784947));
#61470=CARTESIAN_POINT('Ctrl Pts',(3.99989129179464,-1.,-0.766412457135786));
#61471=CARTESIAN_POINT('Ctrl Pts',(3.99989129179464,1.,-0.766412457135786));
#61472=CARTESIAN_POINT('Ctrl Pts',(3.99234687880892,-1.,-0.767968531377708));
#61473=CARTESIAN_POINT('Ctrl Pts',(3.99234687880892,1.,-0.767968531377708));
#61474=CARTESIAN_POINT('Ctrl Pts',(3.98480422348403,-1.,-0.76948556624546));
#61475=CARTESIAN_POINT('Ctrl Pts',(3.98480422348403,1.,-0.76948556624546));
#61476=CARTESIAN_POINT('Ctrl Pts',(3.97726349165507,-1.,-0.770963190030504));
#61477=CARTESIAN_POINT('Ctrl Pts',(3.97726349165507,1.,-0.770963190030504));
#61478=CARTESIAN_POINT('Ctrl Pts',(3.96972446532832,-1.,-0.772400931772239));
#61479=CARTESIAN_POINT('Ctrl Pts',(3.96972446532832,1.,-0.772400931772239));
#61480=CARTESIAN_POINT('Ctrl Pts',(3.96218649639876,-1.,-0.773798212026683));
#61481=CARTESIAN_POINT('Ctrl Pts',(3.96218649639876,1.,-0.773798212026683));
#61482=CARTESIAN_POINT('Ctrl Pts',(3.95464885452364,-1.,-0.775154418039442));
#61483=CARTESIAN_POINT('Ctrl Pts',(3.95464885452364,1.,-0.775154418039442));
#61484=CARTESIAN_POINT('Ctrl Pts',(3.94711101619471,-1.,-0.77646896669796));
#61485=CARTESIAN_POINT('Ctrl Pts',(3.94711101619471,1.,-0.77646896669796));
#61486=CARTESIAN_POINT('Ctrl Pts',(3.93957296768098,-1.,-0.77774137056855));
#61487=CARTESIAN_POINT('Ctrl Pts',(3.93957296768098,1.,-0.77774137056855));
#61488=CARTESIAN_POINT('Ctrl Pts',(3.93203552473153,-1.,-0.778971308134786));
#61489=CARTESIAN_POINT('Ctrl Pts',(3.93203552473153,1.,-0.778971308134786));
#61490=CARTESIAN_POINT('Ctrl Pts',(3.92450058323799,-1.,-0.780158678615507));
#61491=CARTESIAN_POINT('Ctrl Pts',(3.92450058323799,1.,-0.780158678615507));
#61492=CARTESIAN_POINT('Ctrl Pts',(3.9169703605466,-1.,-0.781303428618344));
#61493=CARTESIAN_POINT('Ctrl Pts',(3.9169703605466,1.,-0.781303428618344));
#61494=CARTESIAN_POINT('Ctrl Pts',(3.90944671004536,-1.,-0.782405395622759));
#61495=CARTESIAN_POINT('Ctrl Pts',(3.90944671004536,1.,-0.782405395622759));
#61496=CARTESIAN_POINT('Ctrl Pts',(3.90193039043971,-1.,-0.783464141529083));
#61497=CARTESIAN_POINT('Ctrl Pts',(3.90193039043971,1.,-0.783464141529083));
#61498=CARTESIAN_POINT('Ctrl Pts',(3.89442039235105,-1.,-0.784478799358336));
#61499=CARTESIAN_POINT('Ctrl Pts',(3.89442039235105,1.,-0.784478799358336));
#61500=CARTESIAN_POINT('Ctrl Pts',(3.88691313167399,-1.,-0.785447890340723));
#61501=CARTESIAN_POINT('Ctrl Pts',(3.88691313167399,1.,-0.785447890340723));
#61502=CARTESIAN_POINT('Ctrl Pts',(3.87940402818186,-1.,-0.786369675812592));
#61503=CARTESIAN_POINT('Ctrl Pts',(3.87940402818186,1.,-0.786369675812592));
#61504=CARTESIAN_POINT('Ctrl Pts',(3.87188916600905,-1.,-0.787242527617981));
#61505=CARTESIAN_POINT('Ctrl Pts',(3.87188916600905,1.,-0.787242527617981));
#61506=CARTESIAN_POINT('Ctrl Pts',(3.86436702561342,-1.,-0.788065315093771));
#61507=CARTESIAN_POINT('Ctrl Pts',(3.86436702561342,1.,-0.788065315093771));
#61508=CARTESIAN_POINT('Ctrl Pts',(3.85683995872536,-1.,-0.788837734090688));
#61509=CARTESIAN_POINT('Ctrl Pts',(3.85683995872536,1.,-0.788837734090688));
#61510=CARTESIAN_POINT('Ctrl Pts',(3.8493163780891,-1.,-0.789560798155619));
#61511=CARTESIAN_POINT('Ctrl Pts',(3.8493163780891,1.,-0.789560798155619));
#61512=CARTESIAN_POINT('Ctrl Pts',(3.84180762342476,-1.,-0.790236124191289));
#61513=CARTESIAN_POINT('Ctrl Pts',(3.84180762342476,1.,-0.790236124191289));
#61514=CARTESIAN_POINT('Ctrl Pts',(3.83432392054804,-1.,-0.79086501270534));
#61515=CARTESIAN_POINT('Ctrl Pts',(3.83432392054804,1.,-0.79086501270534));
#61516=CARTESIAN_POINT('Ctrl Pts',(3.82687033899799,-1.,-0.791447528662381));
#61517=CARTESIAN_POINT('Ctrl Pts',(3.82687033899799,1.,-0.791447528662381));
#61518=CARTESIAN_POINT('Ctrl Pts',(3.81944345442237,-1.,-0.791981740718607));
#61519=CARTESIAN_POINT('Ctrl Pts',(3.81944345442237,1.,-0.791981740718607));
#61520=CARTESIAN_POINT('Ctrl Pts',(3.81202588694726,-1.,-0.792462483517568));
#61521=CARTESIAN_POINT('Ctrl Pts',(3.81202588694726,1.,-0.792462483517568));
#61522=CARTESIAN_POINT('Ctrl Pts',(3.80459229925598,-1.,-0.792882695234693));
#61523=CARTESIAN_POINT('Ctrl Pts',(3.80459229925598,1.,-0.792882695234693));
#61524=CARTESIAN_POINT('Ctrl Pts',(3.79711921389862,-1.,-0.793235612973201));
#61525=CARTESIAN_POINT('Ctrl Pts',(3.79711921389862,1.,-0.793235612973201));
#61526=CARTESIAN_POINT('Ctrl Pts',(3.78959439439222,-1.,-0.793516871680966));
#61527=CARTESIAN_POINT('Ctrl Pts',(3.78959439439222,1.,-0.793516871680966));
#61528=CARTESIAN_POINT('Ctrl Pts',(3.78202460377617,-1.,-0.79372623578134));
#61529=CARTESIAN_POINT('Ctrl Pts',(3.78202460377617,1.,-0.79372623578134));
#61530=CARTESIAN_POINT('Ctrl Pts',(3.77444863801264,-1.,-0.793870523787515));
#61531=CARTESIAN_POINT('Ctrl Pts',(3.77444863801264,1.,-0.793870523787515));
#61532=CARTESIAN_POINT('Ctrl Pts',(3.76692626931184,-1.,-0.793961083689141));
#61533=CARTESIAN_POINT('Ctrl Pts',(3.76692626931184,1.,-0.793961083689141));
#61534=CARTESIAN_POINT('Ctrl Pts',(3.75951468666325,-1.,-0.794008429135047));
#61535=CARTESIAN_POINT('Ctrl Pts',(3.75951468666325,1.,-0.794008429135047));
#61536=CARTESIAN_POINT('Ctrl Pts',(3.75224692493895,-1.,-0.794017347371441));
#61537=CARTESIAN_POINT('Ctrl Pts',(3.75224692493895,1.,-0.794017347371441));
#61538=CARTESIAN_POINT('Ctrl Pts',(3.74511357728827,-1.,-0.79398270045988));
#61539=CARTESIAN_POINT('Ctrl Pts',(3.74511357728827,1.,-0.79398270045988));
#61540=CARTESIAN_POINT('Ctrl Pts',(3.73803280541576,-1.,-0.793882700936791));
#61541=CARTESIAN_POINT('Ctrl Pts',(3.73803280541576,1.,-0.793882700936791));
#61542=CARTESIAN_POINT('Ctrl Pts',(3.7308691469564,-1.,-0.793682750269348));
#61543=CARTESIAN_POINT('Ctrl Pts',(3.7308691469564,1.,-0.793682750269348));
#61544=CARTESIAN_POINT('Ctrl Pts',(3.7234879729357,-1.,-0.793347023783871));
#61545=CARTESIAN_POINT('Ctrl Pts',(3.7234879729357,1.,-0.793347023783871));
#61546=CARTESIAN_POINT('Ctrl Pts',(3.7158024239604,-1.,-0.792848377370116));
#61547=CARTESIAN_POINT('Ctrl Pts',(3.7158024239604,1.,-0.792848377370116));
#61548=CARTESIAN_POINT('Ctrl Pts',(3.70781724021879,-1.,-0.792177688845968));
#61549=CARTESIAN_POINT('Ctrl Pts',(3.70781724021879,1.,-0.792177688845968));
#61550=CARTESIAN_POINT('Ctrl Pts',(3.69968940808982,-1.,-0.791356575696509));
#61551=CARTESIAN_POINT('Ctrl Pts',(3.69968940808982,1.,-0.791356575696509));
#61552=CARTESIAN_POINT('Ctrl Pts',(3.69172044327754,-1.,-0.79043628498958));
#61553=CARTESIAN_POINT('Ctrl Pts',(3.69172044327754,1.,-0.79043628498958));
#61554=CARTESIAN_POINT('Ctrl Pts',(3.68428439784285,-1.,-0.789483546065159));
#61555=CARTESIAN_POINT('Ctrl Pts',(3.68428439784285,1.,-0.789483546065159));
#61556=CARTESIAN_POINT('Ctrl Pts',(3.67777119516438,-1.,-0.788569566220663));
#61557=CARTESIAN_POINT('Ctrl Pts',(3.67777119516438,1.,-0.788569566220663));
#61558=CARTESIAN_POINT('Ctrl Pts',(3.672529236635,-1.,-0.787758799995427));
#61559=CARTESIAN_POINT('Ctrl Pts',(3.672529236635,1.,-0.787758799995427));
#61560=CARTESIAN_POINT('Ctrl Pts',(3.66879484800625,-1.,-0.787095252589508));
#61561=CARTESIAN_POINT('Ctrl Pts',(3.66879484800625,1.,-0.787095252589508));
#61562=CARTESIAN_POINT('Ctrl Pts',(3.66710211819938,-1.,-0.786698783541658));
#61563=CARTESIAN_POINT('Ctrl Pts',(3.66710211819938,1.,-0.786698783541658));
#61564=CARTESIAN_POINT('Ctrl Pts',(3.66657784454965,-1.,-0.786480236184947));
#61565=CARTESIAN_POINT('Ctrl Pts',(3.66657784454965,1.,-0.786480236184947));
#61566=CARTESIAN_POINT('Ctrl Pts',(3.66655932661846,-1.,-0.78636952818304));
#61567=CARTESIAN_POINT('Ctrl Pts',(3.66655932661846,1.,-0.78636952818304));
#61568=CARTESIAN_POINT('Ctrl Pts',(3.66663282329846,-1.,-0.786322922920599));
#61569=CARTESIAN_POINT('Ctrl Pts',(3.66663282329846,1.,-0.786322922920599));
#61570=CARTESIAN_POINT('',(4.13571194405636,1.,-0.73204283740062));
#61571=CARTESIAN_POINT('Ctrl Pts',(4.13571194405636,1.,-0.73204283740062));
#61572=CARTESIAN_POINT('Ctrl Pts',(4.13420383737278,1.,-0.732488575135926));
#61573=CARTESIAN_POINT('Ctrl Pts',(4.13118752796397,1.,-0.733376589325634));
#61574=CARTESIAN_POINT('Ctrl Pts',(4.12666277572794,1.,-0.734698226767513));
#61575=CARTESIAN_POINT('Ctrl Pts',(4.12062919626082,1.,-0.736439634335347));
#61576=CARTESIAN_POINT('Ctrl Pts',(4.11308626953795,1.,-0.738581708229119));
#61577=CARTESIAN_POINT('Ctrl Pts',(4.1055424175856,1.,-0.740688998555152));
#61578=CARTESIAN_POINT('Ctrl Pts',(4.09799769702712,1.,-0.742761369690018));
#61579=CARTESIAN_POINT('Ctrl Pts',(4.09045220253011,1.,-0.744798649705514));
#61580=CARTESIAN_POINT('Ctrl Pts',(4.08290608094789,1.,-0.746800631490822));
#61581=CARTESIAN_POINT('Ctrl Pts',(4.07535951055363,1.,-0.748767076679177));
#61582=CARTESIAN_POINT('Ctrl Pts',(4.06781267241886,1.,-0.750697720483176));
#61583=CARTESIAN_POINT('Ctrl Pts',(4.06026572221399,1.,-0.752592276482869));
#61584=CARTESIAN_POINT('Ctrl Pts',(4.05271876688106,1.,-0.754450441816412));
#61585=CARTESIAN_POINT('Ctrl Pts',(4.04517182654344,1.,-0.756271902370187));
#61586=CARTESIAN_POINT('Ctrl Pts',(4.03762485803468,1.,-0.758056338885554));
#61587=CARTESIAN_POINT('Ctrl Pts',(4.0300778195465,1.,-0.759803433244166));
#61588=CARTESIAN_POINT('Ctrl Pts',(4.02253072741347,1.,-0.761512875859942));
#61589=CARTESIAN_POINT('Ctrl Pts',(4.01498370680434,1.,-0.763184371182827));
#61590=CARTESIAN_POINT('Ctrl Pts',(4.00743706791366,1.,-0.764817648784947));
#61591=CARTESIAN_POINT('Ctrl Pts',(3.99989129179464,1.,-0.766412457135786));
#61592=CARTESIAN_POINT('Ctrl Pts',(3.99234687880892,1.,-0.767968531377708));
#61593=CARTESIAN_POINT('Ctrl Pts',(3.98480422348403,1.,-0.76948556624546));
#61594=CARTESIAN_POINT('Ctrl Pts',(3.97726349165507,1.,-0.770963190030504));
#61595=CARTESIAN_POINT('Ctrl Pts',(3.96972446532832,1.,-0.772400931772239));
#61596=CARTESIAN_POINT('Ctrl Pts',(3.96218649639876,1.,-0.773798212026683));
#61597=CARTESIAN_POINT('Ctrl Pts',(3.95464885452364,1.,-0.775154418039442));
#61598=CARTESIAN_POINT('Ctrl Pts',(3.94711101619471,1.,-0.77646896669796));
#61599=CARTESIAN_POINT('Ctrl Pts',(3.93957296768098,1.,-0.77774137056855));
#61600=CARTESIAN_POINT('Ctrl Pts',(3.93203552473153,1.,-0.778971308134786));
#61601=CARTESIAN_POINT('Ctrl Pts',(3.92450058323799,1.,-0.780158678615507));
#61602=CARTESIAN_POINT('Ctrl Pts',(3.9169703605466,1.,-0.781303428618344));
#61603=CARTESIAN_POINT('Ctrl Pts',(3.90944671004536,1.,-0.782405395622759));
#61604=CARTESIAN_POINT('Ctrl Pts',(3.90193039043971,1.,-0.783464141529083));
#61605=CARTESIAN_POINT('Ctrl Pts',(3.89442039235105,1.,-0.784478799358336));
#61606=CARTESIAN_POINT('Ctrl Pts',(3.88691313167399,1.,-0.785447890340723));
#61607=CARTESIAN_POINT('Ctrl Pts',(3.87940402818186,1.,-0.786369675812592));
#61608=CARTESIAN_POINT('Ctrl Pts',(3.87188916600905,1.,-0.787242527617981));
#61609=CARTESIAN_POINT('Ctrl Pts',(3.86436702561342,1.,-0.788065315093771));
#61610=CARTESIAN_POINT('Ctrl Pts',(3.85683995872536,1.,-0.788837734090688));
#61611=CARTESIAN_POINT('Ctrl Pts',(3.8493163780891,1.,-0.789560798155619));
#61612=CARTESIAN_POINT('Ctrl Pts',(3.84180762342476,1.,-0.790236124191289));
#61613=CARTESIAN_POINT('Ctrl Pts',(3.83432392054804,1.,-0.79086501270534));
#61614=CARTESIAN_POINT('Ctrl Pts',(3.82687033899799,1.,-0.791447528662381));
#61615=CARTESIAN_POINT('Ctrl Pts',(3.81944345442237,1.,-0.791981740718607));
#61616=CARTESIAN_POINT('Ctrl Pts',(3.81202588694726,1.,-0.792462483517568));
#61617=CARTESIAN_POINT('Ctrl Pts',(3.80459229925598,1.,-0.792882695234693));
#61618=CARTESIAN_POINT('Ctrl Pts',(3.79711921389862,1.,-0.793235612973201));
#61619=CARTESIAN_POINT('Ctrl Pts',(3.78959439439222,1.,-0.793516871680966));
#61620=CARTESIAN_POINT('Ctrl Pts',(3.78202460377617,1.,-0.79372623578134));
#61621=CARTESIAN_POINT('Ctrl Pts',(3.77444863801264,1.,-0.793870523787515));
#61622=CARTESIAN_POINT('Ctrl Pts',(3.76692626931184,1.,-0.793961083689141));
#61623=CARTESIAN_POINT('Ctrl Pts',(3.75951468666325,1.,-0.794008429135047));
#61624=CARTESIAN_POINT('Ctrl Pts',(3.75224692493895,1.,-0.794017347371441));
#61625=CARTESIAN_POINT('Ctrl Pts',(3.74511357728827,1.,-0.79398270045988));
#61626=CARTESIAN_POINT('Ctrl Pts',(3.73803280541576,1.,-0.793882700936791));
#61627=CARTESIAN_POINT('Ctrl Pts',(3.7308691469564,1.,-0.793682750269348));
#61628=CARTESIAN_POINT('Ctrl Pts',(3.7234879729357,1.,-0.793347023783871));
#61629=CARTESIAN_POINT('Ctrl Pts',(3.7158024239604,1.,-0.792848377370116));
#61630=CARTESIAN_POINT('Ctrl Pts',(3.70781724021879,1.,-0.792177688845968));
#61631=CARTESIAN_POINT('Ctrl Pts',(3.69968940808982,1.,-0.791356575696509));
#61632=CARTESIAN_POINT('Ctrl Pts',(3.69172044327754,1.,-0.79043628498958));
#61633=CARTESIAN_POINT('Ctrl Pts',(3.68428439784285,1.,-0.789483546065159));
#61634=CARTESIAN_POINT('Ctrl Pts',(3.67777119516438,1.,-0.788569566220663));
#61635=CARTESIAN_POINT('Ctrl Pts',(3.672529236635,1.,-0.787758799995427));
#61636=CARTESIAN_POINT('Ctrl Pts',(3.66907505398769,1.,-0.787145041181589));
#61637=CARTESIAN_POINT('Ctrl Pts',(3.66743103898844,1.,-0.7867743371985));
#61638=CARTESIAN_POINT('Ctrl Pts',(3.66680946938396,1.,-0.78656591955989));
#61639=CARTESIAN_POINT('Ctrl Pts',(3.66664310415236,1.,-0.786459983896781));
#61640=CARTESIAN_POINT('Ctrl Pts',(3.66661143271648,1.,-0.786422660833743));
#61641=CARTESIAN_POINT('',(4.13571194405636,0.,-0.73204283740062));
#61642=CARTESIAN_POINT('Origin',(4.15950947128175,0.,-0.581791163835815));
#61643=CARTESIAN_POINT('',(4.15950947128175,1.,-0.581791163835815));
#61644=CARTESIAN_POINT('',(4.13571194405636,1.,-0.73204283740062));
#61645=CARTESIAN_POINT('',(4.15950947128175,0.,-0.581791163835815));
#61646=CARTESIAN_POINT('Ctrl Pts',(3.73016218570874,-1.,-0.385214314776329));
#61647=CARTESIAN_POINT('Ctrl Pts',(3.73016218570874,1.,-0.385214314776329));
#61648=CARTESIAN_POINT('Ctrl Pts',(3.73010668803185,-1.,-0.385147278814804));
#61649=CARTESIAN_POINT('Ctrl Pts',(3.73010668803185,1.,-0.385147278814804));
#61650=CARTESIAN_POINT('Ctrl Pts',(3.73015851028729,-1.,-0.385047711603887));
#61651=CARTESIAN_POINT('Ctrl Pts',(3.73015851028729,1.,-0.385047711603887));
#61652=CARTESIAN_POINT('Ctrl Pts',(3.73072465900727,-1.,-0.385001870183842));
#61653=CARTESIAN_POINT('Ctrl Pts',(3.73072465900727,1.,-0.385001870183842));
#61654=CARTESIAN_POINT('Ctrl Pts',(3.73245705639337,-1.,-0.385147887989515));
#61655=CARTESIAN_POINT('Ctrl Pts',(3.73245705639337,1.,-0.385147887989515));
#61656=CARTESIAN_POINT('Ctrl Pts',(3.73621371845475,-1.,-0.385670806454744));
#61657=CARTESIAN_POINT('Ctrl Pts',(3.73621371845475,1.,-0.385670806454744));
#61658=CARTESIAN_POINT('Ctrl Pts',(3.74144965781088,-1.,-0.386519576222036));
#61659=CARTESIAN_POINT('Ctrl Pts',(3.74144965781088,1.,-0.386519576222036));
#61660=CARTESIAN_POINT('Ctrl Pts',(3.74792651696269,-1.,-0.387663020050396));
#61661=CARTESIAN_POINT('Ctrl Pts',(3.74792651696269,1.,-0.387663020050396));
#61662=CARTESIAN_POINT('Ctrl Pts',(3.75529302894757,-1.,-0.389054775898251));
#61663=CARTESIAN_POINT('Ctrl Pts',(3.75529302894757,1.,-0.389054775898251));
#61664=CARTESIAN_POINT('Ctrl Pts',(3.76315635032993,-1.,-0.390642072979259));
#61665=CARTESIAN_POINT('Ctrl Pts',(3.76315635032993,1.,-0.390642072979259));
#61666=CARTESIAN_POINT('Ctrl Pts',(3.77114011595892,-1.,-0.392372786223347));
#61667=CARTESIAN_POINT('Ctrl Pts',(3.77114011595892,1.,-0.392372786223347));
#61668=CARTESIAN_POINT('Ctrl Pts',(3.77894173114368,-1.,-0.394202481011595));
#61669=CARTESIAN_POINT('Ctrl Pts',(3.77894173114368,1.,-0.394202481011595));
#61670=CARTESIAN_POINT('Ctrl Pts',(3.78640521279479,-1.,-0.396103205335029));
#61671=CARTESIAN_POINT('Ctrl Pts',(3.78640521279479,1.,-0.396103205335029));
#61672=CARTESIAN_POINT('Ctrl Pts',(3.79352887163457,-1.,-0.398064818684159));
#61673=CARTESIAN_POINT('Ctrl Pts',(3.79352887163457,1.,-0.398064818684159));
#61674=CARTESIAN_POINT('Ctrl Pts',(3.80040370384659,-1.,-0.400088346504727));
#61675=CARTESIAN_POINT('Ctrl Pts',(3.80040370384659,1.,-0.400088346504727));
#61676=CARTESIAN_POINT('Ctrl Pts',(3.80716881962763,-1.,-0.402181320148475));
#61677=CARTESIAN_POINT('Ctrl Pts',(3.80716881962763,1.,-0.402181320148475));
#61678=CARTESIAN_POINT('Ctrl Pts',(3.81396374287762,-1.,-0.404352694628237));
#61679=CARTESIAN_POINT('Ctrl Pts',(3.81396374287762,1.,-0.404352694628237));
#61680=CARTESIAN_POINT('Ctrl Pts',(3.82087303913741,-1.,-0.406607038258907));
#61681=CARTESIAN_POINT('Ctrl Pts',(3.82087303913741,1.,-0.406607038258907));
#61682=CARTESIAN_POINT('Ctrl Pts',(3.82790724256397,-1.,-0.408942371447377));
#61683=CARTESIAN_POINT('Ctrl Pts',(3.82790724256397,1.,-0.408942371447377));
#61684=CARTESIAN_POINT('Ctrl Pts',(3.83503345578645,-1.,-0.41135303879846));
#61685=CARTESIAN_POINT('Ctrl Pts',(3.83503345578645,1.,-0.41135303879846));
#61686=CARTESIAN_POINT('Ctrl Pts',(3.84219403994742,-1.,-0.413831367016727));
#61687=CARTESIAN_POINT('Ctrl Pts',(3.84219403994742,1.,-0.413831367016727));
#61688=CARTESIAN_POINT('Ctrl Pts',(3.8493286415751,-1.,-0.41636967805292));
#61689=CARTESIAN_POINT('Ctrl Pts',(3.8493286415751,1.,-0.41636967805292));
#61690=CARTESIAN_POINT('Ctrl Pts',(3.85639825648031,-1.,-0.41896246808681));
#61691=CARTESIAN_POINT('Ctrl Pts',(3.85639825648031,1.,-0.41896246808681));
#61692=CARTESIAN_POINT('Ctrl Pts',(3.86339652542749,-1.,-0.421607423177576));
#61693=CARTESIAN_POINT('Ctrl Pts',(3.86339652542749,1.,-0.421607423177576));
#61694=CARTESIAN_POINT('Ctrl Pts',(3.87033643487882,-1.,-0.424304173195143));
#61695=CARTESIAN_POINT('Ctrl Pts',(3.87033643487882,1.,-0.424304173195143));
#61696=CARTESIAN_POINT('Ctrl Pts',(3.87724240306609,-1.,-0.427053541173469));
#61697=CARTESIAN_POINT('Ctrl Pts',(3.87724240306609,1.,-0.427053541173469));
#61698=CARTESIAN_POINT('Ctrl Pts',(3.88414070943334,-1.,-0.429856640579734));
#61699=CARTESIAN_POINT('Ctrl Pts',(3.88414070943334,1.,-0.429856640579734));
#61700=CARTESIAN_POINT('Ctrl Pts',(3.89104947940592,-1.,-0.43271392954444));
#61701=CARTESIAN_POINT('Ctrl Pts',(3.89104947940592,1.,-0.43271392954444));
#61702=CARTESIAN_POINT('Ctrl Pts',(3.8979725665544,-1.,-0.435624629433506));
#61703=CARTESIAN_POINT('Ctrl Pts',(3.8979725665544,1.,-0.435624629433506));
#61704=CARTESIAN_POINT('Ctrl Pts',(3.90490512938546,-1.,-0.438587235458234));
#61705=CARTESIAN_POINT('Ctrl Pts',(3.90490512938546,1.,-0.438587235458234));
#61706=CARTESIAN_POINT('Ctrl Pts',(3.91183704069146,-1.,-0.441599824524048));
#61707=CARTESIAN_POINT('Ctrl Pts',(3.91183704069146,1.,-0.441599824524048));
#61708=CARTESIAN_POINT('Ctrl Pts',(3.91875701610721,-1.,-0.444660430230593));
#61709=CARTESIAN_POINT('Ctrl Pts',(3.91875701610721,1.,-0.444660430230593));
#61710=CARTESIAN_POINT('Ctrl Pts',(3.92565674143424,-1.,-0.447767416837297));
#61711=CARTESIAN_POINT('Ctrl Pts',(3.92565674143424,1.,-0.447767416837297));
#61712=CARTESIAN_POINT('Ctrl Pts',(3.93253407403128,-1.,-0.450919768356347));
#61713=CARTESIAN_POINT('Ctrl Pts',(3.93253407403128,1.,-0.450919768356347));
#61714=CARTESIAN_POINT('Ctrl Pts',(3.93939080846298,-1.,-0.454116879027576));
#61715=CARTESIAN_POINT('Ctrl Pts',(3.93939080846298,1.,-0.454116879027576));
#61716=CARTESIAN_POINT('Ctrl Pts',(3.94623117206675,-1.,-0.457358410451674));
#61717=CARTESIAN_POINT('Ctrl Pts',(3.94623117206675,1.,-0.457358410451674));
#61718=CARTESIAN_POINT('Ctrl Pts',(3.95306005817363,-1.,-0.460644124429119));
#61719=CARTESIAN_POINT('Ctrl Pts',(3.95306005817363,1.,-0.460644124429119));
#61720=CARTESIAN_POINT('Ctrl Pts',(3.95988133243543,-1.,-0.463973722115745));
#61721=CARTESIAN_POINT('Ctrl Pts',(3.95988133243543,1.,-0.463973722115745));
#61722=CARTESIAN_POINT('Ctrl Pts',(3.96669622273946,-1.,-0.467346690880672));
#61723=CARTESIAN_POINT('Ctrl Pts',(3.96669622273946,1.,-0.467346690880672));
#61724=CARTESIAN_POINT('Ctrl Pts',(3.97350414289415,-1.,-0.470762379613478));
#61725=CARTESIAN_POINT('Ctrl Pts',(3.97350414289415,1.,-0.470762379613478));
#61726=CARTESIAN_POINT('Ctrl Pts',(3.9803033804443,-1.,-0.474220061019542));
#61727=CARTESIAN_POINT('Ctrl Pts',(3.9803033804443,1.,-0.474220061019542));
#61728=CARTESIAN_POINT('Ctrl Pts',(3.98709184306743,-1.,-0.477718999122033));
#61729=CARTESIAN_POINT('Ctrl Pts',(3.98709184306743,1.,-0.477718999122033));
#61730=CARTESIAN_POINT('Ctrl Pts',(3.99386775880655,-1.,-0.481258512209638));
#61731=CARTESIAN_POINT('Ctrl Pts',(3.99386775880655,1.,-0.481258512209638));
#61732=CARTESIAN_POINT('Ctrl Pts',(4.00063045119234,-1.,-0.484838042421754));
#61733=CARTESIAN_POINT('Ctrl Pts',(4.00063045119234,1.,-0.484838042421754));
#61734=CARTESIAN_POINT('Ctrl Pts',(4.0073800839092,-1.,-0.488457130424531));
#61735=CARTESIAN_POINT('Ctrl Pts',(4.0073800839092,1.,-0.488457130424531));
#61736=CARTESIAN_POINT('Ctrl Pts',(4.01411733503486,-1.,-0.492115383417931));
#61737=CARTESIAN_POINT('Ctrl Pts',(4.01411733503486,1.,-0.492115383417931));
#61738=CARTESIAN_POINT('Ctrl Pts',(4.02084308851813,-1.,-0.495812444326223));
#61739=CARTESIAN_POINT('Ctrl Pts',(4.02084308851813,1.,-0.495812444326223));
#61740=CARTESIAN_POINT('Ctrl Pts',(4.0275581398015,-1.,-0.49954796234089));
#61741=CARTESIAN_POINT('Ctrl Pts',(4.0275581398015,1.,-0.49954796234089));
#61742=CARTESIAN_POINT('Ctrl Pts',(4.0342628417439,-1.,-0.503321556915514));
#61743=CARTESIAN_POINT('Ctrl Pts',(4.0342628417439,1.,-0.503321556915514));
#61744=CARTESIAN_POINT('Ctrl Pts',(4.04095715149074,-1.,-0.507132823288362));
#61745=CARTESIAN_POINT('Ctrl Pts',(4.04095715149074,1.,-0.507132823288362));
#61746=CARTESIAN_POINT('Ctrl Pts',(4.04764078815591,-1.,-0.510981349219174));
#61747=CARTESIAN_POINT('Ctrl Pts',(4.04764078815591,1.,-0.510981349219174));
#61748=CARTESIAN_POINT('Ctrl Pts',(4.05431335771261,-1.,-0.514866728193104));
#61749=CARTESIAN_POINT('Ctrl Pts',(4.05431335771261,1.,-0.514866728193104));
#61750=CARTESIAN_POINT('Ctrl Pts',(4.06097448037934,-1.,-0.51878857233681));
#61751=CARTESIAN_POINT('Ctrl Pts',(4.06097448037934,1.,-0.51878857233681));
#61752=CARTESIAN_POINT('Ctrl Pts',(4.06762394471075,-1.,-0.522746528602768));
#61753=CARTESIAN_POINT('Ctrl Pts',(4.06762394471075,1.,-0.522746528602768));
#61754=CARTESIAN_POINT('Ctrl Pts',(4.07426172299496,-1.,-0.526740277227));
#61755=CARTESIAN_POINT('Ctrl Pts',(4.07426172299496,1.,-0.526740277227));
#61756=CARTESIAN_POINT('Ctrl Pts',(4.08088789536488,-1.,-0.530769518728076));
#61757=CARTESIAN_POINT('Ctrl Pts',(4.08088789536488,1.,-0.530769518728076));
#61758=CARTESIAN_POINT('Ctrl Pts',(4.08750259988693,-1.,-0.534833963477));
#61759=CARTESIAN_POINT('Ctrl Pts',(4.08750259988693,1.,-0.534833963477));
#61760=CARTESIAN_POINT('Ctrl Pts',(4.09410597627116,-1.,-0.538933321179921));
#61761=CARTESIAN_POINT('Ctrl Pts',(4.09410597627116,1.,-0.538933321179921));
#61762=CARTESIAN_POINT('Ctrl Pts',(4.10069810244473,-1.,-0.543067286878457));
#61763=CARTESIAN_POINT('Ctrl Pts',(4.10069810244473,1.,-0.543067286878457));
#61764=CARTESIAN_POINT('Ctrl Pts',(4.1072789702877,-1.,-0.54723553948676));
#61765=CARTESIAN_POINT('Ctrl Pts',(4.1072789702877,1.,-0.54723553948676));
#61766=CARTESIAN_POINT('Ctrl Pts',(4.11384852025578,-1.,-0.551437758498247));
#61767=CARTESIAN_POINT('Ctrl Pts',(4.11384852025578,1.,-0.551437758498247));
#61768=CARTESIAN_POINT('Ctrl Pts',(4.1204066619623,-1.,-0.555673636130778));
#61769=CARTESIAN_POINT('Ctrl Pts',(4.1204066619623,1.,-0.555673636130778));
#61770=CARTESIAN_POINT('Ctrl Pts',(4.12695329951859,-1.,-0.559942890594628));
#61771=CARTESIAN_POINT('Ctrl Pts',(4.12695329951859,1.,-0.559942890594628));
#61772=CARTESIAN_POINT('Ctrl Pts',(4.13348835726086,-1.,-0.564245279535706));
#61773=CARTESIAN_POINT('Ctrl Pts',(4.13348835726086,1.,-0.564245279535706));
#61774=CARTESIAN_POINT('Ctrl Pts',(4.14001179828669,-1.,-0.568580610187116));
#61775=CARTESIAN_POINT('Ctrl Pts',(4.14001179828669,1.,-0.568580610187116));
#61776=CARTESIAN_POINT('Ctrl Pts',(4.14652361065787,-1.,-0.572948736066277));
#61777=CARTESIAN_POINT('Ctrl Pts',(4.14652361065787,1.,-0.572948736066277));
#61778=CARTESIAN_POINT('Ctrl Pts',(4.1517237611974,-1.,-0.576469391673917));
#61779=CARTESIAN_POINT('Ctrl Pts',(4.1517237611974,1.,-0.576469391673917));
#61780=CARTESIAN_POINT('Ctrl Pts',(4.15561864787379,-1.,-0.579124568912544));
#61781=CARTESIAN_POINT('Ctrl Pts',(4.15561864787379,1.,-0.579124568912544));
#61782=CARTESIAN_POINT('Ctrl Pts',(4.15821291712391,-1.,-0.580901211462913));
#61783=CARTESIAN_POINT('Ctrl Pts',(4.15821291712391,1.,-0.580901211462913));
#61784=CARTESIAN_POINT('Ctrl Pts',(4.15950947128175,-1.,-0.581791163835815));
#61785=CARTESIAN_POINT('Ctrl Pts',(4.15950947128175,1.,-0.581791163835815));
#61786=CARTESIAN_POINT('',(3.73017266276632,1.,-0.385112848332548));
#61787=CARTESIAN_POINT('Ctrl Pts',(3.73017266276632,-1.,-0.385112848332549));
#61788=CARTESIAN_POINT('Ctrl Pts',(3.73017266276632,-0.666666666666667,
-0.385112848332549));
#61789=CARTESIAN_POINT('Ctrl Pts',(3.73017266276632,-0.333333333333333,
-0.385112848332549));
#61790=CARTESIAN_POINT('Ctrl Pts',(3.73017266276632,0.333333333333333,-0.385112848332549));
#61791=CARTESIAN_POINT('Ctrl Pts',(3.73017266276632,0.666666666666667,-0.38511284833255));
#61792=CARTESIAN_POINT('Ctrl Pts',(3.73017266276632,1.,-0.38511284833255));
#61793=CARTESIAN_POINT('Ctrl Pts',(3.73017266276632,1.,-0.385112848332549));
#61794=CARTESIAN_POINT('Ctrl Pts',(3.73021431755218,1.,-0.385087139001609));
#61795=CARTESIAN_POINT('Ctrl Pts',(3.73040527620929,1.,-0.385037797882046));
#61796=CARTESIAN_POINT('Ctrl Pts',(3.731060828624,1.,-0.385031656499142));
#61797=CARTESIAN_POINT('Ctrl Pts',(3.73273893363318,1.,-0.385187124633965));
#61798=CARTESIAN_POINT('Ctrl Pts',(3.73621371845475,1.,-0.385670806454744));
#61799=CARTESIAN_POINT('Ctrl Pts',(3.74144965781088,1.,-0.386519576222036));
#61800=CARTESIAN_POINT('Ctrl Pts',(3.74792651696269,1.,-0.387663020050396));
#61801=CARTESIAN_POINT('Ctrl Pts',(3.75529302894757,1.,-0.389054775898251));
#61802=CARTESIAN_POINT('Ctrl Pts',(3.76315635032993,1.,-0.390642072979259));
#61803=CARTESIAN_POINT('Ctrl Pts',(3.77114011595892,1.,-0.392372786223347));
#61804=CARTESIAN_POINT('Ctrl Pts',(3.77894173114368,1.,-0.394202481011595));
#61805=CARTESIAN_POINT('Ctrl Pts',(3.78640521279479,1.,-0.396103205335029));
#61806=CARTESIAN_POINT('Ctrl Pts',(3.79352887163457,1.,-0.398064818684159));
#61807=CARTESIAN_POINT('Ctrl Pts',(3.80040370384659,1.,-0.400088346504727));
#61808=CARTESIAN_POINT('Ctrl Pts',(3.80716881962763,1.,-0.402181320148475));
#61809=CARTESIAN_POINT('Ctrl Pts',(3.81396374287762,1.,-0.404352694628237));
#61810=CARTESIAN_POINT('Ctrl Pts',(3.82087303913741,1.,-0.406607038258907));
#61811=CARTESIAN_POINT('Ctrl Pts',(3.82790724256397,1.,-0.408942371447377));
#61812=CARTESIAN_POINT('Ctrl Pts',(3.83503345578645,1.,-0.41135303879846));
#61813=CARTESIAN_POINT('Ctrl Pts',(3.84219403994742,1.,-0.413831367016727));
#61814=CARTESIAN_POINT('Ctrl Pts',(3.8493286415751,1.,-0.41636967805292));
#61815=CARTESIAN_POINT('Ctrl Pts',(3.85639825648031,1.,-0.41896246808681));
#61816=CARTESIAN_POINT('Ctrl Pts',(3.86339652542749,1.,-0.421607423177576));
#61817=CARTESIAN_POINT('Ctrl Pts',(3.87033643487882,1.,-0.424304173195143));
#61818=CARTESIAN_POINT('Ctrl Pts',(3.87724240306609,1.,-0.427053541173469));
#61819=CARTESIAN_POINT('Ctrl Pts',(3.88414070943334,1.,-0.429856640579734));
#61820=CARTESIAN_POINT('Ctrl Pts',(3.89104947940592,1.,-0.43271392954444));
#61821=CARTESIAN_POINT('Ctrl Pts',(3.8979725665544,1.,-0.435624629433506));
#61822=CARTESIAN_POINT('Ctrl Pts',(3.90490512938546,1.,-0.438587235458234));
#61823=CARTESIAN_POINT('Ctrl Pts',(3.91183704069146,1.,-0.441599824524048));
#61824=CARTESIAN_POINT('Ctrl Pts',(3.91875701610721,1.,-0.444660430230593));
#61825=CARTESIAN_POINT('Ctrl Pts',(3.92565674143424,1.,-0.447767416837297));
#61826=CARTESIAN_POINT('Ctrl Pts',(3.93253407403128,1.,-0.450919768356347));
#61827=CARTESIAN_POINT('Ctrl Pts',(3.93939080846298,1.,-0.454116879027576));
#61828=CARTESIAN_POINT('Ctrl Pts',(3.94623117206675,1.,-0.457358410451674));
#61829=CARTESIAN_POINT('Ctrl Pts',(3.95306005817363,1.,-0.460644124429119));
#61830=CARTESIAN_POINT('Ctrl Pts',(3.95988133243543,1.,-0.463973722115745));
#61831=CARTESIAN_POINT('Ctrl Pts',(3.96669622273946,1.,-0.467346690880672));
#61832=CARTESIAN_POINT('Ctrl Pts',(3.97350414289415,1.,-0.470762379613478));
#61833=CARTESIAN_POINT('Ctrl Pts',(3.9803033804443,1.,-0.474220061019542));
#61834=CARTESIAN_POINT('Ctrl Pts',(3.98709184306743,1.,-0.477718999122033));
#61835=CARTESIAN_POINT('Ctrl Pts',(3.99386775880655,1.,-0.481258512209638));
#61836=CARTESIAN_POINT('Ctrl Pts',(4.00063045119234,1.,-0.484838042421754));
#61837=CARTESIAN_POINT('Ctrl Pts',(4.0073800839092,1.,-0.488457130424531));
#61838=CARTESIAN_POINT('Ctrl Pts',(4.01411733503486,1.,-0.492115383417931));
#61839=CARTESIAN_POINT('Ctrl Pts',(4.02084308851813,1.,-0.495812444326223));
#61840=CARTESIAN_POINT('Ctrl Pts',(4.0275581398015,1.,-0.49954796234089));
#61841=CARTESIAN_POINT('Ctrl Pts',(4.0342628417439,1.,-0.503321556915514));
#61842=CARTESIAN_POINT('Ctrl Pts',(4.04095715149074,1.,-0.507132823288362));
#61843=CARTESIAN_POINT('Ctrl Pts',(4.04764078815591,1.,-0.510981349219174));
#61844=CARTESIAN_POINT('Ctrl Pts',(4.05431335771261,1.,-0.514866728193104));
#61845=CARTESIAN_POINT('Ctrl Pts',(4.06097448037934,1.,-0.51878857233681));
#61846=CARTESIAN_POINT('Ctrl Pts',(4.06762394471075,1.,-0.522746528602768));
#61847=CARTESIAN_POINT('Ctrl Pts',(4.07426172299496,1.,-0.526740277227));
#61848=CARTESIAN_POINT('Ctrl Pts',(4.08088789536488,1.,-0.530769518728076));
#61849=CARTESIAN_POINT('Ctrl Pts',(4.08750259988693,1.,-0.534833963477));
#61850=CARTESIAN_POINT('Ctrl Pts',(4.09410597627116,1.,-0.538933321179921));
#61851=CARTESIAN_POINT('Ctrl Pts',(4.10069810244473,1.,-0.543067286878457));
#61852=CARTESIAN_POINT('Ctrl Pts',(4.1072789702877,1.,-0.54723553948676));
#61853=CARTESIAN_POINT('Ctrl Pts',(4.11384852025578,1.,-0.551437758498247));
#61854=CARTESIAN_POINT('Ctrl Pts',(4.1204066619623,1.,-0.555673636130778));
#61855=CARTESIAN_POINT('Ctrl Pts',(4.12695329951859,1.,-0.559942890594628));
#61856=CARTESIAN_POINT('Ctrl Pts',(4.13348835726086,1.,-0.564245279535706));
#61857=CARTESIAN_POINT('Ctrl Pts',(4.14001179828669,1.,-0.568580610187116));
#61858=CARTESIAN_POINT('Ctrl Pts',(4.14652361065787,1.,-0.572948736066277));
#61859=CARTESIAN_POINT('Ctrl Pts',(4.1517237611974,1.,-0.576469391673917));
#61860=CARTESIAN_POINT('Ctrl Pts',(4.15561864787379,1.,-0.579124568912544));
#61861=CARTESIAN_POINT('Ctrl Pts',(4.15821291712391,1.,-0.580901211462913));
#61862=CARTESIAN_POINT('Ctrl Pts',(4.15950947128175,1.,-0.581791163835815));
#61863=CARTESIAN_POINT('Origin',(0.,0.,0.));
#61864=CARTESIAN_POINT('',(3.74449296982994,1.,-0.203156094897896));
#61865=CARTESIAN_POINT('Origin',(0.,1.,0.));
#61866=CARTESIAN_POINT('Ctrl Pts',(3.74449296982994,1.,-0.203156094897896));
#61867=CARTESIAN_POINT('Ctrl Pts',(3.74449296982994,0.666666666666667,-0.203156094897896));
#61868=CARTESIAN_POINT('Ctrl Pts',(3.74449296982994,0.333333333333333,-0.203156094897896));
#61869=CARTESIAN_POINT('Ctrl Pts',(3.74449296982994,-0.333333333333333,
-0.203156094897896));
#61870=CARTESIAN_POINT('Ctrl Pts',(3.74449296982994,-0.666666666666667,
-0.203156094897895));
#61871=CARTESIAN_POINT('Ctrl Pts',(3.74449296982994,-1.,-0.203156094897895));
#61872=CARTESIAN_POINT('Ctrl Pts',(3.74449849461127,-1.,0.20305423869972));
#61873=CARTESIAN_POINT('Ctrl Pts',(3.74449849461127,1.,0.20305423869972));
#61874=CARTESIAN_POINT('Ctrl Pts',(3.7444331934681,-1.,0.203111767587923));
#61875=CARTESIAN_POINT('Ctrl Pts',(3.7444331934681,1.,0.203111767587923));
#61876=CARTESIAN_POINT('Ctrl Pts',(3.7444688019622,-1.,0.203218215748058));
#61877=CARTESIAN_POINT('Ctrl Pts',(3.7444688019622,1.,0.203218215748058));
#61878=CARTESIAN_POINT('Ctrl Pts',(3.74502080927395,-1.,0.203352057956297));
#61879=CARTESIAN_POINT('Ctrl Pts',(3.74502080927395,1.,0.203352057956297));
#61880=CARTESIAN_POINT('Ctrl Pts',(3.7467547201908,-1.,0.203478844530446));
#61881=CARTESIAN_POINT('Ctrl Pts',(3.7467547201908,1.,0.203478844530446));
#61882=CARTESIAN_POINT('Ctrl Pts',(3.75054693397875,-1.,0.203550035479166));
#61883=CARTESIAN_POINT('Ctrl Pts',(3.75054693397875,1.,0.203550035479166));
#61884=CARTESIAN_POINT('Ctrl Pts',(3.75585118707734,-1.,0.203530796848321));
#61885=CARTESIAN_POINT('Ctrl Pts',(3.75585118707734,1.,0.203530796848321));
#61886=CARTESIAN_POINT('Ctrl Pts',(3.76242717936885,-1.,0.203414634707478));
#61887=CARTESIAN_POINT('Ctrl Pts',(3.76242717936885,1.,0.203414634707478));
#61888=CARTESIAN_POINT('Ctrl Pts',(3.7699207159487,-1.,0.203192390045164));
#61889=CARTESIAN_POINT('Ctrl Pts',(3.7699207159487,1.,0.203192390045164));
#61890=CARTESIAN_POINT('Ctrl Pts',(3.77793553476614,-1.,0.20285472969908));
#61891=CARTESIAN_POINT('Ctrl Pts',(3.77793553476614,1.,0.20285472969908));
#61892=CARTESIAN_POINT('Ctrl Pts',(3.78609175019242,-1.,0.20239426051216));
#61893=CARTESIAN_POINT('Ctrl Pts',(3.78609175019242,1.,0.20239426051216));
#61894=CARTESIAN_POINT('Ctrl Pts',(3.7940835418736,-1.,0.201807533800837));
#61895=CARTESIAN_POINT('Ctrl Pts',(3.7940835418736,1.,0.201807533800837));
#61896=CARTESIAN_POINT('Ctrl Pts',(3.80175247447337,-1.,0.201097756307325));
#61897=CARTESIAN_POINT('Ctrl Pts',(3.80175247447337,1.,0.201097756307325));
#61898=CARTESIAN_POINT('Ctrl Pts',(3.80909529318669,-1.,0.200274679433364));
#61899=CARTESIAN_POINT('Ctrl Pts',(3.80909529318669,1.,0.200274679433364));
#61900=CARTESIAN_POINT('Ctrl Pts',(3.81620203429815,-1.,0.199351525297447));
#61901=CARTESIAN_POINT('Ctrl Pts',(3.81620203429815,1.,0.199351525297447));
#61902=CARTESIAN_POINT('Ctrl Pts',(3.82321127349016,-1.,0.198342616900486));
#61903=CARTESIAN_POINT('Ctrl Pts',(3.82321127349016,1.,0.198342616900486));
#61904=CARTESIAN_POINT('Ctrl Pts',(3.83026221776456,-1.,0.197260935827361));
#61905=CARTESIAN_POINT('Ctrl Pts',(3.83026221776456,1.,0.197260935827361));
#61906=CARTESIAN_POINT('Ctrl Pts',(3.83743910616195,-1.,0.196115198971858));
#61907=CARTESIAN_POINT('Ctrl Pts',(3.83743910616195,1.,0.196115198971858));
#61908=CARTESIAN_POINT('Ctrl Pts',(3.84475203346977,-1.,0.19490900946022));
#61909=CARTESIAN_POINT('Ctrl Pts',(3.84475203346977,1.,0.19490900946022));
#61910=CARTESIAN_POINT('Ctrl Pts',(3.85216762263966,-1.,0.193642806777722));
#61911=CARTESIAN_POINT('Ctrl Pts',(3.85216762263966,1.,0.193642806777722));
#61912=CARTESIAN_POINT('Ctrl Pts',(3.85962774407633,-1.,0.19231515304497));
#61913=CARTESIAN_POINT('Ctrl Pts',(3.85962774407633,1.,0.19231515304497));
#61914=CARTESIAN_POINT('Ctrl Pts',(3.86707158624783,-1.,0.190924190418619));
#61915=CARTESIAN_POINT('Ctrl Pts',(3.86707158624783,1.,0.190924190418619));
#61916=CARTESIAN_POINT('Ctrl Pts',(3.87445976418412,-1.,0.189469253358272));
#61917=CARTESIAN_POINT('Ctrl Pts',(3.87445976418412,1.,0.189469253358272));
#61918=CARTESIAN_POINT('Ctrl Pts',(3.88178563496228,-1.,0.187951632512684));
#61919=CARTESIAN_POINT('Ctrl Pts',(3.88178563496228,1.,0.187951632512684));
#61920=CARTESIAN_POINT('Ctrl Pts',(3.88906196725848,-1.,0.18637372498528));
#61921=CARTESIAN_POINT('Ctrl Pts',(3.88906196725848,1.,0.18637372498528));
#61922=CARTESIAN_POINT('Ctrl Pts',(3.89631300742646,-1.,0.184738537728042));
#61923=CARTESIAN_POINT('Ctrl Pts',(3.89631300742646,1.,0.184738537728042));
#61924=CARTESIAN_POINT('Ctrl Pts',(3.90356488555132,-1.,0.18304908199319));
#61925=CARTESIAN_POINT('Ctrl Pts',(3.90356488555132,1.,0.18304908199319));
#61926=CARTESIAN_POINT('Ctrl Pts',(3.91083557557175,-1.,0.181307740731785));
#61927=CARTESIAN_POINT('Ctrl Pts',(3.91083557557175,1.,0.181307740731785));
#61928=CARTESIAN_POINT('Ctrl Pts',(3.91812876180926,-1.,0.179515885822881));
#61929=CARTESIAN_POINT('Ctrl Pts',(3.91812876180926,1.,0.179515885822881));
#61930=CARTESIAN_POINT('Ctrl Pts',(3.92543942697655,-1.,0.177674246152317));
#61931=CARTESIAN_POINT('Ctrl Pts',(3.92543942697655,1.,0.177674246152317));
#61932=CARTESIAN_POINT('Ctrl Pts',(3.93275726771042,-1.,0.175783136893867));
#61933=CARTESIAN_POINT('Ctrl Pts',(3.93275726771042,1.,0.175783136893867));
#61934=CARTESIAN_POINT('Ctrl Pts',(3.94007083096217,-1.,0.173842734974609));
#61935=CARTESIAN_POINT('Ctrl Pts',(3.94007083096217,1.,0.173842734974609));
#61936=CARTESIAN_POINT('Ctrl Pts',(3.94737164900868,-1.,0.17185335536924));
#61937=CARTESIAN_POINT('Ctrl Pts',(3.94737164900868,1.,0.17185335536924));
#61938=CARTESIAN_POINT('Ctrl Pts',(3.95465744665268,-1.,0.169815666374138));
#61939=CARTESIAN_POINT('Ctrl Pts',(3.95465744665268,1.,0.169815666374138));
#61940=CARTESIAN_POINT('Ctrl Pts',(3.96192990160296,-1.,0.167730547023319));
#61941=CARTESIAN_POINT('Ctrl Pts',(3.96192990160296,1.,0.167730547023319));
#61942=CARTESIAN_POINT('Ctrl Pts',(3.96919313621407,-1.,0.165598992851102));
#61943=CARTESIAN_POINT('Ctrl Pts',(3.96919313621407,1.,0.165598992851102));
#61944=CARTESIAN_POINT('Ctrl Pts',(3.97645194630943,-1.,0.163422004609999));
#61945=CARTESIAN_POINT('Ctrl Pts',(3.97645194630943,1.,0.163422004609999));
#61946=CARTESIAN_POINT('Ctrl Pts',(3.98371010319872,-1.,0.161200482186084));
#61947=CARTESIAN_POINT('Ctrl Pts',(3.98371010319872,1.,0.161200482186084));
#61948=CARTESIAN_POINT('Ctrl Pts',(3.99096873945878,-1.,0.158935123982793));
#61949=CARTESIAN_POINT('Ctrl Pts',(3.99096873945878,1.,0.158935123982793));
#61950=CARTESIAN_POINT('Ctrl Pts',(3.99822717425893,-1.,0.156626481393734));
#61951=CARTESIAN_POINT('Ctrl Pts',(3.99822717425893,1.,0.156626481393734));
#61952=CARTESIAN_POINT('Ctrl Pts',(4.00548360245319,-1.,0.15427500487231));
#61953=CARTESIAN_POINT('Ctrl Pts',(4.00548360245319,1.,0.15427500487231));
#61954=CARTESIAN_POINT('Ctrl Pts',(4.01273584234689,-1.,0.15188109402291));
#61955=CARTESIAN_POINT('Ctrl Pts',(4.01273584234689,1.,0.15188109402291));
#61956=CARTESIAN_POINT('Ctrl Pts',(4.01998203715564,-1.,0.149445144968706));
#61957=CARTESIAN_POINT('Ctrl Pts',(4.01998203715564,1.,0.149445144968706));
#61958=CARTESIAN_POINT('Ctrl Pts',(4.02722143146994,-1.,0.146967602878994));
#61959=CARTESIAN_POINT('Ctrl Pts',(4.02722143146994,1.,0.146967602878994));
#61960=CARTESIAN_POINT('Ctrl Pts',(4.03445411510333,-1.,0.144448947038344));
#61961=CARTESIAN_POINT('Ctrl Pts',(4.03445411510333,1.,0.144448947038344));
#61962=CARTESIAN_POINT('Ctrl Pts',(4.04168069633781,-1.,0.1418896714855));
#61963=CARTESIAN_POINT('Ctrl Pts',(4.04168069633781,1.,0.1418896714855));
#61964=CARTESIAN_POINT('Ctrl Pts',(4.04890199238036,-1.,0.139290267180057));
#61965=CARTESIAN_POINT('Ctrl Pts',(4.04890199238036,1.,0.139290267180057));
#61966=CARTESIAN_POINT('Ctrl Pts',(4.05611873400172,-1.,0.136651205046119));
#61967=CARTESIAN_POINT('Ctrl Pts',(4.05611873400172,1.,0.136651205046119));
#61968=CARTESIAN_POINT('Ctrl Pts',(4.06333121018596,-1.,0.133972916144244));
#61969=CARTESIAN_POINT('Ctrl Pts',(4.06333121018596,1.,0.133972916144244));
#61970=CARTESIAN_POINT('Ctrl Pts',(4.0705393152874,-1.,0.13125579354894));
#61971=CARTESIAN_POINT('Ctrl Pts',(4.0705393152874,1.,0.13125579354894));
#61972=CARTESIAN_POINT('Ctrl Pts',(4.07774270738954,-1.,0.128500200484837));
#61973=CARTESIAN_POINT('Ctrl Pts',(4.07774270738954,1.,0.128500200484837));
#61974=CARTESIAN_POINT('Ctrl Pts',(4.08494093372377,-1.,0.125706476822539));
#61975=CARTESIAN_POINT('Ctrl Pts',(4.08494093372377,1.,0.125706476822539));
#61976=CARTESIAN_POINT('Ctrl Pts',(4.09213355850756,-1.,0.122874946249106));
#61977=CARTESIAN_POINT('Ctrl Pts',(4.09213355850756,1.,0.122874946249106));
#61978=CARTESIAN_POINT('Ctrl Pts',(4.09932031767002,-1.,0.120005924388124));
#61979=CARTESIAN_POINT('Ctrl Pts',(4.09932031767002,1.,0.120005924388124));
#61980=CARTESIAN_POINT('Ctrl Pts',(4.10650113381833,-1.,0.117099722731648));
#61981=CARTESIAN_POINT('Ctrl Pts',(4.10650113381833,1.,0.117099722731648));
#61982=CARTESIAN_POINT('Ctrl Pts',(4.11367603924961,-1.,0.114156649609545));
#61983=CARTESIAN_POINT('Ctrl Pts',(4.11367603924961,1.,0.114156649609545));
#61984=CARTESIAN_POINT('Ctrl Pts',(4.1208451250225,-1.,0.111177012683346));
#61985=CARTESIAN_POINT('Ctrl Pts',(4.1208451250225,1.,0.111177012683346));
#61986=CARTESIAN_POINT('Ctrl Pts',(4.12800848371504,-1.,0.108161120528369));
#61987=CARTESIAN_POINT('Ctrl Pts',(4.12800848371504,1.,0.108161120528369));
#61988=CARTESIAN_POINT('Ctrl Pts',(4.13516614458895,-1.,0.105109286538945));
#61989=CARTESIAN_POINT('Ctrl Pts',(4.13516614458895,1.,0.105109286538945));
#61990=CARTESIAN_POINT('Ctrl Pts',(4.14231804939538,-1.,0.102021826577583));
#61991=CARTESIAN_POINT('Ctrl Pts',(4.14231804939538,1.,0.102021826577583));
#61992=CARTESIAN_POINT('Ctrl Pts',(4.14946408918485,-1.,0.0988990478901221));
#61993=CARTESIAN_POINT('Ctrl Pts',(4.14946408918485,1.,0.0988990478901221));
#61994=CARTESIAN_POINT('Ctrl Pts',(4.15660412653577,-1.,0.0957412403298002));
#61995=CARTESIAN_POINT('Ctrl Pts',(4.15660412653577,1.,0.0957412403298002));
#61996=CARTESIAN_POINT('Ctrl Pts',(4.16373802265839,-1.,0.0925486672167526));
#61997=CARTESIAN_POINT('Ctrl Pts',(4.16373802265839,1.,0.0925486672167526));
#61998=CARTESIAN_POINT('Ctrl Pts',(4.17086566490794,-1.,0.0893215560848644));
#61999=CARTESIAN_POINT('Ctrl Pts',(4.17086566490794,1.,0.0893215560848644));
#62000=CARTESIAN_POINT('Ctrl Pts',(4.17798698668094,-1.,0.0860600915549391));
#62001=CARTESIAN_POINT('Ctrl Pts',(4.17798698668094,1.,0.0860600915549391));
#62002=CARTESIAN_POINT('Ctrl Pts',(4.18510195327123,-1.,0.0827644164385674));
#62003=CARTESIAN_POINT('Ctrl Pts',(4.18510195327123,1.,0.0827644164385674));
#62004=CARTESIAN_POINT('Ctrl Pts',(4.19078883320504,-1.,0.0801005887114315));
#62005=CARTESIAN_POINT('Ctrl Pts',(4.19078883320504,1.,0.0801005887114315));
#62006=CARTESIAN_POINT('Ctrl Pts',(4.19505112859416,-1.,0.0780873956242392));
#62007=CARTESIAN_POINT('Ctrl Pts',(4.19505112859416,1.,0.0780873956242392));
#62008=CARTESIAN_POINT('Ctrl Pts',(4.1978913862118,-1.,0.0767384596141459));
#62009=CARTESIAN_POINT('Ctrl Pts',(4.1978913862118,1.,0.0767384596141459));
#62010=CARTESIAN_POINT('Ctrl Pts',(4.19931119685982,-1.,0.0760622897878241));
#62011=CARTESIAN_POINT('Ctrl Pts',(4.19931119685982,1.,0.0760622897878241));
#62012=CARTESIAN_POINT('',(3.74449296983004,1.,0.2031560948961));
#62013=CARTESIAN_POINT('Ctrl Pts',(3.74449296983004,-1.,0.2031560948961));
#62014=CARTESIAN_POINT('Ctrl Pts',(3.74449296983004,-0.666666666666667,
0.2031560948961));
#62015=CARTESIAN_POINT('Ctrl Pts',(3.74449296983004,-0.333333333333333,
0.2031560948961));
#62016=CARTESIAN_POINT('Ctrl Pts',(3.74449296983004,0.333333333333333,0.2031560948961));
#62017=CARTESIAN_POINT('Ctrl Pts',(3.74449296983004,0.666666666666667,0.2031560948961));
#62018=CARTESIAN_POINT('Ctrl Pts',(3.74449296983004,1.,0.2031560948961));
#62019=CARTESIAN_POINT('',(4.19931119685982,1.,0.0760622897878241));
#62020=CARTESIAN_POINT('',(4.19931119685982,0.,0.0760622897878241));
#62021=CARTESIAN_POINT('Ctrl Pts',(3.74449296983004,1.,0.2031560948961));
#62022=CARTESIAN_POINT('Ctrl Pts',(3.74453008995092,1.,0.203188003946656));
#62023=CARTESIAN_POINT('Ctrl Pts',(3.74471097893845,1.,0.20326661011053));
#62024=CARTESIAN_POINT('Ctrl Pts',(3.74535749969115,1.,0.203375226874121));
#62025=CARTESIAN_POINT('Ctrl Pts',(3.74703926501752,1.,0.203484186269415));
#62026=CARTESIAN_POINT('Ctrl Pts',(3.75054693397875,1.,0.203550035479166));
#62027=CARTESIAN_POINT('Ctrl Pts',(3.75585118707734,1.,0.203530796848321));
#62028=CARTESIAN_POINT('Ctrl Pts',(3.76242717936885,1.,0.203414634707478));
#62029=CARTESIAN_POINT('Ctrl Pts',(3.7699207159487,1.,0.203192390045164));
#62030=CARTESIAN_POINT('Ctrl Pts',(3.77793553476614,1.,0.20285472969908));
#62031=CARTESIAN_POINT('Ctrl Pts',(3.78609175019242,1.,0.20239426051216));
#62032=CARTESIAN_POINT('Ctrl Pts',(3.7940835418736,1.,0.201807533800837));
#62033=CARTESIAN_POINT('Ctrl Pts',(3.80175247447337,1.,0.201097756307325));
#62034=CARTESIAN_POINT('Ctrl Pts',(3.80909529318669,1.,0.200274679433364));
#62035=CARTESIAN_POINT('Ctrl Pts',(3.81620203429815,1.,0.199351525297447));
#62036=CARTESIAN_POINT('Ctrl Pts',(3.82321127349016,1.,0.198342616900486));
#62037=CARTESIAN_POINT('Ctrl Pts',(3.83026221776456,1.,0.197260935827361));
#62038=CARTESIAN_POINT('Ctrl Pts',(3.83743910616195,1.,0.196115198971858));
#62039=CARTESIAN_POINT('Ctrl Pts',(3.84475203346977,1.,0.19490900946022));
#62040=CARTESIAN_POINT('Ctrl Pts',(3.85216762263966,1.,0.193642806777722));
#62041=CARTESIAN_POINT('Ctrl Pts',(3.85962774407633,1.,0.19231515304497));
#62042=CARTESIAN_POINT('Ctrl Pts',(3.86707158624783,1.,0.190924190418619));
#62043=CARTESIAN_POINT('Ctrl Pts',(3.87445976418412,1.,0.189469253358272));
#62044=CARTESIAN_POINT('Ctrl Pts',(3.88178563496228,1.,0.187951632512684));
#62045=CARTESIAN_POINT('Ctrl Pts',(3.88906196725848,1.,0.18637372498528));
#62046=CARTESIAN_POINT('Ctrl Pts',(3.89631300742646,1.,0.184738537728042));
#62047=CARTESIAN_POINT('Ctrl Pts',(3.90356488555132,1.,0.18304908199319));
#62048=CARTESIAN_POINT('Ctrl Pts',(3.91083557557175,1.,0.181307740731785));
#62049=CARTESIAN_POINT('Ctrl Pts',(3.91812876180926,1.,0.179515885822881));
#62050=CARTESIAN_POINT('Ctrl Pts',(3.92543942697655,1.,0.177674246152317));
#62051=CARTESIAN_POINT('Ctrl Pts',(3.93275726771042,1.,0.175783136893867));
#62052=CARTESIAN_POINT('Ctrl Pts',(3.94007083096217,1.,0.173842734974609));
#62053=CARTESIAN_POINT('Ctrl Pts',(3.94737164900868,1.,0.17185335536924));
#62054=CARTESIAN_POINT('Ctrl Pts',(3.95465744665268,1.,0.169815666374138));
#62055=CARTESIAN_POINT('Ctrl Pts',(3.96192990160296,1.,0.167730547023319));
#62056=CARTESIAN_POINT('Ctrl Pts',(3.96919313621407,1.,0.165598992851102));
#62057=CARTESIAN_POINT('Ctrl Pts',(3.97645194630943,1.,0.163422004609999));
#62058=CARTESIAN_POINT('Ctrl Pts',(3.98371010319872,1.,0.161200482186084));
#62059=CARTESIAN_POINT('Ctrl Pts',(3.99096873945878,1.,0.158935123982793));
#62060=CARTESIAN_POINT('Ctrl Pts',(3.99822717425893,1.,0.156626481393734));
#62061=CARTESIAN_POINT('Ctrl Pts',(4.00548360245319,1.,0.15427500487231));
#62062=CARTESIAN_POINT('Ctrl Pts',(4.01273584234689,1.,0.15188109402291));
#62063=CARTESIAN_POINT('Ctrl Pts',(4.01998203715564,1.,0.149445144968706));
#62064=CARTESIAN_POINT('Ctrl Pts',(4.02722143146994,1.,0.146967602878994));
#62065=CARTESIAN_POINT('Ctrl Pts',(4.03445411510333,1.,0.144448947038344));
#62066=CARTESIAN_POINT('Ctrl Pts',(4.04168069633781,1.,0.1418896714855));
#62067=CARTESIAN_POINT('Ctrl Pts',(4.04890199238036,1.,0.139290267180057));
#62068=CARTESIAN_POINT('Ctrl Pts',(4.05611873400172,1.,0.136651205046119));
#62069=CARTESIAN_POINT('Ctrl Pts',(4.06333121018596,1.,0.133972916144244));
#62070=CARTESIAN_POINT('Ctrl Pts',(4.0705393152874,1.,0.13125579354894));
#62071=CARTESIAN_POINT('Ctrl Pts',(4.07774270738954,1.,0.128500200484837));
#62072=CARTESIAN_POINT('Ctrl Pts',(4.08494093372377,1.,0.125706476822539));
#62073=CARTESIAN_POINT('Ctrl Pts',(4.09213355850756,1.,0.122874946249106));
#62074=CARTESIAN_POINT('Ctrl Pts',(4.09932031767002,1.,0.120005924388124));
#62075=CARTESIAN_POINT('Ctrl Pts',(4.10650113381833,1.,0.117099722731648));
#62076=CARTESIAN_POINT('Ctrl Pts',(4.11367603924961,1.,0.114156649609545));
#62077=CARTESIAN_POINT('Ctrl Pts',(4.1208451250225,1.,0.111177012683346));
#62078=CARTESIAN_POINT('Ctrl Pts',(4.12800848371504,1.,0.108161120528369));
#62079=CARTESIAN_POINT('Ctrl Pts',(4.13516614458895,1.,0.105109286538945));
#62080=CARTESIAN_POINT('Ctrl Pts',(4.14231804939538,1.,0.102021826577583));
#62081=CARTESIAN_POINT('Ctrl Pts',(4.14946408918485,1.,0.0988990478901221));
#62082=CARTESIAN_POINT('Ctrl Pts',(4.15660412653577,1.,0.0957412403298002));
#62083=CARTESIAN_POINT('Ctrl Pts',(4.16373802265839,1.,0.0925486672167526));
#62084=CARTESIAN_POINT('Ctrl Pts',(4.17086566490794,1.,0.0893215560848644));
#62085=CARTESIAN_POINT('Ctrl Pts',(4.17798698668094,1.,0.0860600915549391));
#62086=CARTESIAN_POINT('Ctrl Pts',(4.18510195327123,1.,0.0827644164385674));
#62087=CARTESIAN_POINT('Ctrl Pts',(4.19078883320504,1.,0.0801005887114315));
#62088=CARTESIAN_POINT('Ctrl Pts',(4.19505112859416,1.,0.0780873956242392));
#62089=CARTESIAN_POINT('Ctrl Pts',(4.1978913862118,1.,0.0767384596141459));
#62090=CARTESIAN_POINT('Ctrl Pts',(4.19931119685982,1.,0.0760622897878241));
#62091=CARTESIAN_POINT('Ctrl Pts',(4.19931119685982,-1.,-0.0760622897878241));
#62092=CARTESIAN_POINT('Ctrl Pts',(4.19931119685982,1.,-0.0760622897878241));
#62093=CARTESIAN_POINT('Ctrl Pts',(4.19789138621624,-1.,-0.07673845961422));
#62094=CARTESIAN_POINT('Ctrl Pts',(4.19789138621624,1.,-0.07673845961422));
#62095=CARTESIAN_POINT('Ctrl Pts',(4.19505112860624,-1.,-0.0780873956244407));
#62096=CARTESIAN_POINT('Ctrl Pts',(4.19505112860624,1.,-0.0780873956244407));
#62097=CARTESIAN_POINT('Ctrl Pts',(4.19078883322483,-1.,-0.0801005887117608));
#62098=CARTESIAN_POINT('Ctrl Pts',(4.19078883322483,1.,-0.0801005887117608));
#62099=CARTESIAN_POINT('Ctrl Pts',(4.1851019532944,-1.,-0.0827644164389515));
#62100=CARTESIAN_POINT('Ctrl Pts',(4.1851019532944,1.,-0.0827644164389515));
#62101=CARTESIAN_POINT('Ctrl Pts',(4.17798698669991,-1.,-0.086060091555252));
#62102=CARTESIAN_POINT('Ctrl Pts',(4.17798698669991,1.,-0.086060091555252));
#62103=CARTESIAN_POINT('Ctrl Pts',(4.17086566491823,-1.,-0.0893215560850332));
#62104=CARTESIAN_POINT('Ctrl Pts',(4.17086566491823,1.,-0.0893215560850332));
#62105=CARTESIAN_POINT('Ctrl Pts',(4.16373802265942,-1.,-0.0925486672167695));
#62106=CARTESIAN_POINT('Ctrl Pts',(4.16373802265942,1.,-0.0925486672167695));
#62107=CARTESIAN_POINT('Ctrl Pts',(4.15660412653006,-1.,-0.0957412403297072));
#62108=CARTESIAN_POINT('Ctrl Pts',(4.15660412653006,1.,-0.0957412403297072));
#62109=CARTESIAN_POINT('Ctrl Pts',(4.1494640891762,-1.,-0.0988990478899816));
#62110=CARTESIAN_POINT('Ctrl Pts',(4.1494640891762,1.,-0.0988990478899816));
#62111=CARTESIAN_POINT('Ctrl Pts',(4.14231804938737,-1.,-0.102021826577454));
#62112=CARTESIAN_POINT('Ctrl Pts',(4.14231804938737,1.,-0.102021826577454));
#62113=CARTESIAN_POINT('Ctrl Pts',(4.13516614458396,-1.,-0.105109286538864));
#62114=CARTESIAN_POINT('Ctrl Pts',(4.13516614458396,1.,-0.105109286538864));
#62115=CARTESIAN_POINT('Ctrl Pts',(4.12800848371386,-1.,-0.10816112052835));
#62116=CARTESIAN_POINT('Ctrl Pts',(4.12800848371386,1.,-0.10816112052835));
#62117=CARTESIAN_POINT('Ctrl Pts',(4.12084512502444,-1.,-0.111177012683378));
#62118=CARTESIAN_POINT('Ctrl Pts',(4.12084512502444,1.,-0.111177012683378));
#62119=CARTESIAN_POINT('Ctrl Pts',(4.11367603925313,-1.,-0.114156649609602));
#62120=CARTESIAN_POINT('Ctrl Pts',(4.11367603925313,1.,-0.114156649609602));
#62121=CARTESIAN_POINT('Ctrl Pts',(4.10650113382187,-1.,-0.117099722731705));
#62122=CARTESIAN_POINT('Ctrl Pts',(4.10650113382187,1.,-0.117099722731705));
#62123=CARTESIAN_POINT('Ctrl Pts',(4.09932031767243,-1.,-0.120005924388162));
#62124=CARTESIAN_POINT('Ctrl Pts',(4.09932031767243,1.,-0.120005924388162));
#62125=CARTESIAN_POINT('Ctrl Pts',(4.09213355850836,-1.,-0.122874946249119));
#62126=CARTESIAN_POINT('Ctrl Pts',(4.09213355850836,1.,-0.122874946249119));
#62127=CARTESIAN_POINT('Ctrl Pts',(4.08494093372315,-1.,-0.12570647682253));
#62128=CARTESIAN_POINT('Ctrl Pts',(4.08494093372315,1.,-0.12570647682253));
#62129=CARTESIAN_POINT('Ctrl Pts',(4.07774270738809,-1.,-0.128500200484814));
#62130=CARTESIAN_POINT('Ctrl Pts',(4.07774270738809,1.,-0.128500200484814));
#62131=CARTESIAN_POINT('Ctrl Pts',(4.07053931528579,-1.,-0.131255793548914));
#62132=CARTESIAN_POINT('Ctrl Pts',(4.07053931528579,1.,-0.131255793548914));
#62133=CARTESIAN_POINT('Ctrl Pts',(4.06333121018476,-1.,-0.133972916144225));
#62134=CARTESIAN_POINT('Ctrl Pts',(4.06333121018476,1.,-0.133972916144225));
#62135=CARTESIAN_POINT('Ctrl Pts',(4.05611873400122,-1.,-0.136651205046111));
#62136=CARTESIAN_POINT('Ctrl Pts',(4.05611873400122,1.,-0.136651205046111));
#62137=CARTESIAN_POINT('Ctrl Pts',(4.04890199238056,-1.,-0.13929026718006));
#62138=CARTESIAN_POINT('Ctrl Pts',(4.04890199238056,1.,-0.13929026718006));
#62139=CARTESIAN_POINT('Ctrl Pts',(4.04168069633842,-1.,-0.141889671485508));
#62140=CARTESIAN_POINT('Ctrl Pts',(4.04168069633842,1.,-0.141889671485508));
#62141=CARTESIAN_POINT('Ctrl Pts',(4.03445411510403,-1.,-0.144448947038352));
#62142=CARTESIAN_POINT('Ctrl Pts',(4.03445411510403,1.,-0.144448947038352));
#62143=CARTESIAN_POINT('Ctrl Pts',(4.02722143147048,-1.,-0.146967602878999));
#62144=CARTESIAN_POINT('Ctrl Pts',(4.02722143147048,1.,-0.146967602878999));
#62145=CARTESIAN_POINT('Ctrl Pts',(4.01998203715588,-1.,-0.149445144968708));
#62146=CARTESIAN_POINT('Ctrl Pts',(4.01998203715588,1.,-0.149445144968708));
#62147=CARTESIAN_POINT('Ctrl Pts',(4.01273584234684,-1.,-0.151881094022909));
#62148=CARTESIAN_POINT('Ctrl Pts',(4.01273584234684,1.,-0.151881094022909));
#62149=CARTESIAN_POINT('Ctrl Pts',(4.00548360245297,-1.,-0.15427500487231));
#62150=CARTESIAN_POINT('Ctrl Pts',(4.00548360245297,1.,-0.15427500487231));
#62151=CARTESIAN_POINT('Ctrl Pts',(3.99822717425869,-1.,-0.156626481393736));
#62152=CARTESIAN_POINT('Ctrl Pts',(3.99822717425869,1.,-0.156626481393736));
#62153=CARTESIAN_POINT('Ctrl Pts',(3.99096873945862,-1.,-0.158935123982796));
#62154=CARTESIAN_POINT('Ctrl Pts',(3.99096873945862,1.,-0.158935123982796));
#62155=CARTESIAN_POINT('Ctrl Pts',(3.98371010319866,-1.,-0.161200482186088));
#62156=CARTESIAN_POINT('Ctrl Pts',(3.98371010319866,1.,-0.161200482186088));
#62157=CARTESIAN_POINT('Ctrl Pts',(3.97645194630944,-1.,-0.163422004609999));
#62158=CARTESIAN_POINT('Ctrl Pts',(3.97645194630944,1.,-0.163422004609999));
#62159=CARTESIAN_POINT('Ctrl Pts',(3.9691931362141,-1.,-0.165598992851098));
#62160=CARTESIAN_POINT('Ctrl Pts',(3.9691931362141,1.,-0.165598992851098));
#62161=CARTESIAN_POINT('Ctrl Pts',(3.96192990160296,-1.,-0.167730547023312));
#62162=CARTESIAN_POINT('Ctrl Pts',(3.96192990160296,1.,-0.167730547023312));
#62163=CARTESIAN_POINT('Ctrl Pts',(3.95465744665263,-1.,-0.16981566637413));
#62164=CARTESIAN_POINT('Ctrl Pts',(3.95465744665263,1.,-0.16981566637413));
#62165=CARTESIAN_POINT('Ctrl Pts',(3.94737164900861,-1.,-0.171853355369233));
#62166=CARTESIAN_POINT('Ctrl Pts',(3.94737164900861,1.,-0.171853355369233));
#62167=CARTESIAN_POINT('Ctrl Pts',(3.94007083096214,-1.,-0.173842734974608));
#62168=CARTESIAN_POINT('Ctrl Pts',(3.94007083096214,1.,-0.173842734974608));
#62169=CARTESIAN_POINT('Ctrl Pts',(3.93275726771049,-1.,-0.175783136893873));
#62170=CARTESIAN_POINT('Ctrl Pts',(3.93275726771049,1.,-0.175783136893873));
#62171=CARTESIAN_POINT('Ctrl Pts',(3.92543942697672,-1.,-0.177674246152328));
#62172=CARTESIAN_POINT('Ctrl Pts',(3.92543942697672,1.,-0.177674246152328));
#62173=CARTESIAN_POINT('Ctrl Pts',(3.91812876180948,-1.,-0.179515885822895));
#62174=CARTESIAN_POINT('Ctrl Pts',(3.91812876180948,1.,-0.179515885822895));
#62175=CARTESIAN_POINT('Ctrl Pts',(3.91083557557193,-1.,-0.181307740731796));
#62176=CARTESIAN_POINT('Ctrl Pts',(3.91083557557193,1.,-0.181307740731796));
#62177=CARTESIAN_POINT('Ctrl Pts',(3.90356488555138,-1.,-0.183049081993193));
#62178=CARTESIAN_POINT('Ctrl Pts',(3.90356488555138,1.,-0.183049081993193));
#62179=CARTESIAN_POINT('Ctrl Pts',(3.89631300742633,-1.,-0.184738537728035));
#62180=CARTESIAN_POINT('Ctrl Pts',(3.89631300742633,1.,-0.184738537728035));
#62181=CARTESIAN_POINT('Ctrl Pts',(3.88906196725817,-1.,-0.186373724985263));
#62182=CARTESIAN_POINT('Ctrl Pts',(3.88906196725817,1.,-0.186373724985263));
#62183=CARTESIAN_POINT('Ctrl Pts',(3.88178563496187,-1.,-0.187951632512664));
#62184=CARTESIAN_POINT('Ctrl Pts',(3.88178563496187,1.,-0.187951632512664));
#62185=CARTESIAN_POINT('Ctrl Pts',(3.87445976418377,-1.,-0.189469253358255));
#62186=CARTESIAN_POINT('Ctrl Pts',(3.87445976418377,1.,-0.189469253358255));
#62187=CARTESIAN_POINT('Ctrl Pts',(3.8670715862477,-1.,-0.190924190418613));
#62188=CARTESIAN_POINT('Ctrl Pts',(3.8670715862477,1.,-0.190924190418613));
#62189=CARTESIAN_POINT('Ctrl Pts',(3.85962774407652,-1.,-0.19231515304498));
#62190=CARTESIAN_POINT('Ctrl Pts',(3.85962774407652,1.,-0.19231515304498));
#62191=CARTESIAN_POINT('Ctrl Pts',(3.85216762264019,-1.,-0.193642806777748));
#62192=CARTESIAN_POINT('Ctrl Pts',(3.85216762264019,1.,-0.193642806777748));
#62193=CARTESIAN_POINT('Ctrl Pts',(3.84475203347052,-1.,-0.194909009460255));
#62194=CARTESIAN_POINT('Ctrl Pts',(3.84475203347052,1.,-0.194909009460255));
#62195=CARTESIAN_POINT('Ctrl Pts',(3.83743910616265,-1.,-0.19611519897189));
#62196=CARTESIAN_POINT('Ctrl Pts',(3.83743910616265,1.,-0.19611519897189));
#62197=CARTESIAN_POINT('Ctrl Pts',(3.83026221776488,-1.,-0.197260935827375));
#62198=CARTESIAN_POINT('Ctrl Pts',(3.83026221776488,1.,-0.197260935827375));
#62199=CARTESIAN_POINT('Ctrl Pts',(3.82321127348981,-1.,-0.19834261690047));
#62200=CARTESIAN_POINT('Ctrl Pts',(3.82321127348981,1.,-0.19834261690047));
#62201=CARTESIAN_POINT('Ctrl Pts',(3.81620203429702,-1.,-0.199351525297397));
#62202=CARTESIAN_POINT('Ctrl Pts',(3.81620203429702,1.,-0.199351525297397));
#62203=CARTESIAN_POINT('Ctrl Pts',(3.80909529318501,-1.,-0.20027467943329));
#62204=CARTESIAN_POINT('Ctrl Pts',(3.80909529318501,1.,-0.20027467943329));
#62205=CARTESIAN_POINT('Ctrl Pts',(3.80175247447171,-1.,-0.201097756307252));
#62206=CARTESIAN_POINT('Ctrl Pts',(3.80175247447171,1.,-0.201097756307252));
#62207=CARTESIAN_POINT('Ctrl Pts',(3.79408354187274,-1.,-0.201807533800799));
#62208=CARTESIAN_POINT('Ctrl Pts',(3.79408354187274,1.,-0.201807533800799));
#62209=CARTESIAN_POINT('Ctrl Pts',(3.78609175019317,-1.,-0.202394260512193));
#62210=CARTESIAN_POINT('Ctrl Pts',(3.78609175019317,1.,-0.202394260512193));
#62211=CARTESIAN_POINT('Ctrl Pts',(3.77793553476879,-1.,-0.202854729699197));
#62212=CARTESIAN_POINT('Ctrl Pts',(3.77793553476879,1.,-0.202854729699197));
#62213=CARTESIAN_POINT('Ctrl Pts',(3.76992071595267,-1.,-0.203192390045338));
#62214=CARTESIAN_POINT('Ctrl Pts',(3.76992071595267,1.,-0.203192390045338));
#62215=CARTESIAN_POINT('Ctrl Pts',(3.76242717937273,-1.,-0.203414634707647));
#62216=CARTESIAN_POINT('Ctrl Pts',(3.76242717937273,1.,-0.203414634707647));
#62217=CARTESIAN_POINT('Ctrl Pts',(3.75585118707924,-1.,-0.203530796848404));
#62218=CARTESIAN_POINT('Ctrl Pts',(3.75585118707924,1.,-0.203530796848404));
#62219=CARTESIAN_POINT('Ctrl Pts',(3.75054693397716,-1.,-0.203550035479097));
#62220=CARTESIAN_POINT('Ctrl Pts',(3.75054693397716,1.,-0.203550035479097));
#62221=CARTESIAN_POINT('Ctrl Pts',(3.74675472018582,-1.,-0.20347884453023));
#62222=CARTESIAN_POINT('Ctrl Pts',(3.74675472018582,1.,-0.20347884453023));
#62223=CARTESIAN_POINT('Ctrl Pts',(3.7450208092684,-1.,-0.203352057956056));
#62224=CARTESIAN_POINT('Ctrl Pts',(3.7450208092684,1.,-0.203352057956056));
#62225=CARTESIAN_POINT('Ctrl Pts',(3.74446880195845,-1.,-0.203218215747895));
#62226=CARTESIAN_POINT('Ctrl Pts',(3.74446880195845,1.,-0.203218215747895));
#62227=CARTESIAN_POINT('Ctrl Pts',(3.74443319346666,-1.,-0.20311176758786));
#62228=CARTESIAN_POINT('Ctrl Pts',(3.74443319346666,1.,-0.20311176758786));
#62229=CARTESIAN_POINT('Ctrl Pts',(3.74449849461127,-1.,-0.20305423869972));
#62230=CARTESIAN_POINT('Ctrl Pts',(3.74449849461127,1.,-0.20305423869972));
#62231=CARTESIAN_POINT('',(4.19931119685982,1.,-0.0760622897878241));
#62232=CARTESIAN_POINT('Ctrl Pts',(4.19931119685982,1.,-0.0760622897878241));
#62233=CARTESIAN_POINT('Ctrl Pts',(4.19789138621624,1.,-0.07673845961422));
#62234=CARTESIAN_POINT('Ctrl Pts',(4.19505112860624,1.,-0.0780873956244407));
#62235=CARTESIAN_POINT('Ctrl Pts',(4.19078883322483,1.,-0.0801005887117608));
#62236=CARTESIAN_POINT('Ctrl Pts',(4.1851019532944,1.,-0.0827644164389515));
#62237=CARTESIAN_POINT('Ctrl Pts',(4.17798698669991,1.,-0.086060091555252));
#62238=CARTESIAN_POINT('Ctrl Pts',(4.17086566491823,1.,-0.0893215560850332));
#62239=CARTESIAN_POINT('Ctrl Pts',(4.16373802265942,1.,-0.0925486672167695));
#62240=CARTESIAN_POINT('Ctrl Pts',(4.15660412653006,1.,-0.0957412403297072));
#62241=CARTESIAN_POINT('Ctrl Pts',(4.1494640891762,1.,-0.0988990478899816));
#62242=CARTESIAN_POINT('Ctrl Pts',(4.14231804938737,1.,-0.102021826577454));
#62243=CARTESIAN_POINT('Ctrl Pts',(4.13516614458396,1.,-0.105109286538864));
#62244=CARTESIAN_POINT('Ctrl Pts',(4.12800848371386,1.,-0.10816112052835));
#62245=CARTESIAN_POINT('Ctrl Pts',(4.12084512502444,1.,-0.111177012683378));
#62246=CARTESIAN_POINT('Ctrl Pts',(4.11367603925313,1.,-0.114156649609602));
#62247=CARTESIAN_POINT('Ctrl Pts',(4.10650113382187,1.,-0.117099722731705));
#62248=CARTESIAN_POINT('Ctrl Pts',(4.09932031767243,1.,-0.120005924388162));
#62249=CARTESIAN_POINT('Ctrl Pts',(4.09213355850836,1.,-0.122874946249119));
#62250=CARTESIAN_POINT('Ctrl Pts',(4.08494093372315,1.,-0.12570647682253));
#62251=CARTESIAN_POINT('Ctrl Pts',(4.07774270738809,1.,-0.128500200484814));
#62252=CARTESIAN_POINT('Ctrl Pts',(4.07053931528579,1.,-0.131255793548914));
#62253=CARTESIAN_POINT('Ctrl Pts',(4.06333121018476,1.,-0.133972916144225));
#62254=CARTESIAN_POINT('Ctrl Pts',(4.05611873400122,1.,-0.136651205046111));
#62255=CARTESIAN_POINT('Ctrl Pts',(4.04890199238056,1.,-0.13929026718006));
#62256=CARTESIAN_POINT('Ctrl Pts',(4.04168069633842,1.,-0.141889671485508));
#62257=CARTESIAN_POINT('Ctrl Pts',(4.03445411510403,1.,-0.144448947038352));
#62258=CARTESIAN_POINT('Ctrl Pts',(4.02722143147048,1.,-0.146967602878999));
#62259=CARTESIAN_POINT('Ctrl Pts',(4.01998203715588,1.,-0.149445144968708));
#62260=CARTESIAN_POINT('Ctrl Pts',(4.01273584234684,1.,-0.151881094022909));
#62261=CARTESIAN_POINT('Ctrl Pts',(4.00548360245297,1.,-0.15427500487231));
#62262=CARTESIAN_POINT('Ctrl Pts',(3.99822717425869,1.,-0.156626481393736));
#62263=CARTESIAN_POINT('Ctrl Pts',(3.99096873945862,1.,-0.158935123982796));
#62264=CARTESIAN_POINT('Ctrl Pts',(3.98371010319866,1.,-0.161200482186088));
#62265=CARTESIAN_POINT('Ctrl Pts',(3.97645194630944,1.,-0.163422004609999));
#62266=CARTESIAN_POINT('Ctrl Pts',(3.9691931362141,1.,-0.165598992851098));
#62267=CARTESIAN_POINT('Ctrl Pts',(3.96192990160296,1.,-0.167730547023312));
#62268=CARTESIAN_POINT('Ctrl Pts',(3.95465744665263,1.,-0.16981566637413));
#62269=CARTESIAN_POINT('Ctrl Pts',(3.94737164900861,1.,-0.171853355369233));
#62270=CARTESIAN_POINT('Ctrl Pts',(3.94007083096214,1.,-0.173842734974608));
#62271=CARTESIAN_POINT('Ctrl Pts',(3.93275726771049,1.,-0.175783136893873));
#62272=CARTESIAN_POINT('Ctrl Pts',(3.92543942697672,1.,-0.177674246152328));
#62273=CARTESIAN_POINT('Ctrl Pts',(3.91812876180948,1.,-0.179515885822895));
#62274=CARTESIAN_POINT('Ctrl Pts',(3.91083557557193,1.,-0.181307740731796));
#62275=CARTESIAN_POINT('Ctrl Pts',(3.90356488555138,1.,-0.183049081993193));
#62276=CARTESIAN_POINT('Ctrl Pts',(3.89631300742633,1.,-0.184738537728035));
#62277=CARTESIAN_POINT('Ctrl Pts',(3.88906196725817,1.,-0.186373724985263));
#62278=CARTESIAN_POINT('Ctrl Pts',(3.88178563496187,1.,-0.187951632512664));
#62279=CARTESIAN_POINT('Ctrl Pts',(3.87445976418377,1.,-0.189469253358255));
#62280=CARTESIAN_POINT('Ctrl Pts',(3.8670715862477,1.,-0.190924190418613));
#62281=CARTESIAN_POINT('Ctrl Pts',(3.85962774407652,1.,-0.19231515304498));
#62282=CARTESIAN_POINT('Ctrl Pts',(3.85216762264019,1.,-0.193642806777748));
#62283=CARTESIAN_POINT('Ctrl Pts',(3.84475203347052,1.,-0.194909009460255));
#62284=CARTESIAN_POINT('Ctrl Pts',(3.83743910616265,1.,-0.19611519897189));
#62285=CARTESIAN_POINT('Ctrl Pts',(3.83026221776488,1.,-0.197260935827375));
#62286=CARTESIAN_POINT('Ctrl Pts',(3.82321127348981,1.,-0.19834261690047));
#62287=CARTESIAN_POINT('Ctrl Pts',(3.81620203429702,1.,-0.199351525297397));
#62288=CARTESIAN_POINT('Ctrl Pts',(3.80909529318501,1.,-0.20027467943329));
#62289=CARTESIAN_POINT('Ctrl Pts',(3.80175247447171,1.,-0.201097756307252));
#62290=CARTESIAN_POINT('Ctrl Pts',(3.79408354187274,1.,-0.201807533800799));
#62291=CARTESIAN_POINT('Ctrl Pts',(3.78609175019317,1.,-0.202394260512193));
#62292=CARTESIAN_POINT('Ctrl Pts',(3.77793553476879,1.,-0.202854729699197));
#62293=CARTESIAN_POINT('Ctrl Pts',(3.76992071595267,1.,-0.203192390045338));
#62294=CARTESIAN_POINT('Ctrl Pts',(3.76242717937273,1.,-0.203414634707647));
#62295=CARTESIAN_POINT('Ctrl Pts',(3.75585118707924,1.,-0.203530796848404));
#62296=CARTESIAN_POINT('Ctrl Pts',(3.75054693397716,1.,-0.203550035479097));
#62297=CARTESIAN_POINT('Ctrl Pts',(3.74703926501843,1.,-0.203484186269315));
#62298=CARTESIAN_POINT('Ctrl Pts',(3.74535749969262,1.,-0.203375226874332));
#62299=CARTESIAN_POINT('Ctrl Pts',(3.74471097893961,1.,-0.203266610111264));
#62300=CARTESIAN_POINT('Ctrl Pts',(3.74453008995129,1.,-0.203188003947965));
#62301=CARTESIAN_POINT('Ctrl Pts',(3.74449296982994,1.,-0.203156094897896));
#62302=CARTESIAN_POINT('',(4.19931119685982,0.,-0.0760622897878241));
#62303=CARTESIAN_POINT('Origin',(4.19931119685982,0.,0.0760622897878241));
#62304=CARTESIAN_POINT('',(4.19931119685982,1.,-0.0760622897878241));
#62305=CARTESIAN_POINT('Origin',(0.,1.,0.));
#62306=CARTESIAN_POINT('Origin',(0.,1.,0.));
#62307=CARTESIAN_POINT('Origin',(0.,0.,0.));
#62678=UNCERTAINTY_MEASURE_WITH_UNIT(LENGTH_MEASURE(0.001),#62759,
'DISTANCE_ACCURACY_VALUE',
'Maximum model space distance between geometric entities at asserted c
onnectivities');
#62684=UNCERTAINTY_MEASURE_WITH_UNIT(LENGTH_MEASURE(0.001),#62759,
'DISTANCE_ACCURACY_VALUE',
'Maximum model space distance between geometric entities at asserted c
onnectivities');
#62752=(
GEOMETRIC_REPRESENTATION_CONTEXT(3)
GLOBAL_UNCERTAINTY_ASSIGNED_CONTEXT((#62678))
GLOBAL_UNIT_ASSIGNED_CONTEXT((#62759,#62761,#62762))
REPRESENTATION_CONTEXT('','3D')
);
#62758=(
GEOMETRIC_REPRESENTATION_CONTEXT(3)
GLOBAL_UNCERTAINTY_ASSIGNED_CONTEXT((#62684))
GLOBAL_UNIT_ASSIGNED_CONTEXT((#62759,#62761,#62762))
REPRESENTATION_CONTEXT('','3D')
);
#62759=(
LENGTH_UNIT()
NAMED_UNIT(*)
SI_UNIT(.CENTI.,.METRE.)
);
#62761=(
NAMED_UNIT(*)
PLANE_ANGLE_UNIT()
SI_UNIT($,.RADIAN.)
);
#62762=(
NAMED_UNIT(*)
SI_UNIT($,.STERADIAN.)
SOLID_ANGLE_UNIT()
);
#62830=SHAPE_DEFINITION_REPRESENTATION(#62913,#63098);
#62913=PRODUCT_DEFINITION_SHAPE('',$,#63172);
#63098=SHAPE_REPRESENTATION('',(#18482),#62752);
#63104=PRODUCT_DEFINITION_CONTEXT('part definition',#63325,'design');
#63172=PRODUCT_DEFINITION('Spur Gear - Module 2, 40 Teeth, 20 mm Bore',
'Spur Gear - Module 2, 40 Teeth, 20 mm Bore',#63245,#63104);
#63245=PRODUCT_DEFINITION_FORMATION('',$,#63394);
#63325=APPLICATION_CONTEXT(
'Core Data for Automotive Mechanical Design Process');
#63326=PRODUCT_CONTEXT('part definition',#63325,'mechanical');
#63394=PRODUCT('Spur Gear - Module 2, 40 Teeth, 20 mm Bore',
'Spur Gear - Module 2, 40 Teeth, 20 mm Bore',
'Spur Gear - Module 2, 40 Teeth, 20 mm Bore',(#63326));
#63449=COLOUR_RGB('Sky Blue',0.24,0.69,0.87);
#63450=FILL_AREA_STYLE_COLOUR('',#63449);
#63451=FILL_AREA_STYLE('',(#63450));
#63452=SURFACE_STYLE_FILL_AREA(#63451);
#63453=SURFACE_SIDE_STYLE('',(#63452));
#63454=SURFACE_STYLE_USAGE(.BOTH.,#63453);
#63455=PRESENTATION_STYLE_ASSIGNMENT((#63454));
ENDSEC;
END-ISO-10303-21;
